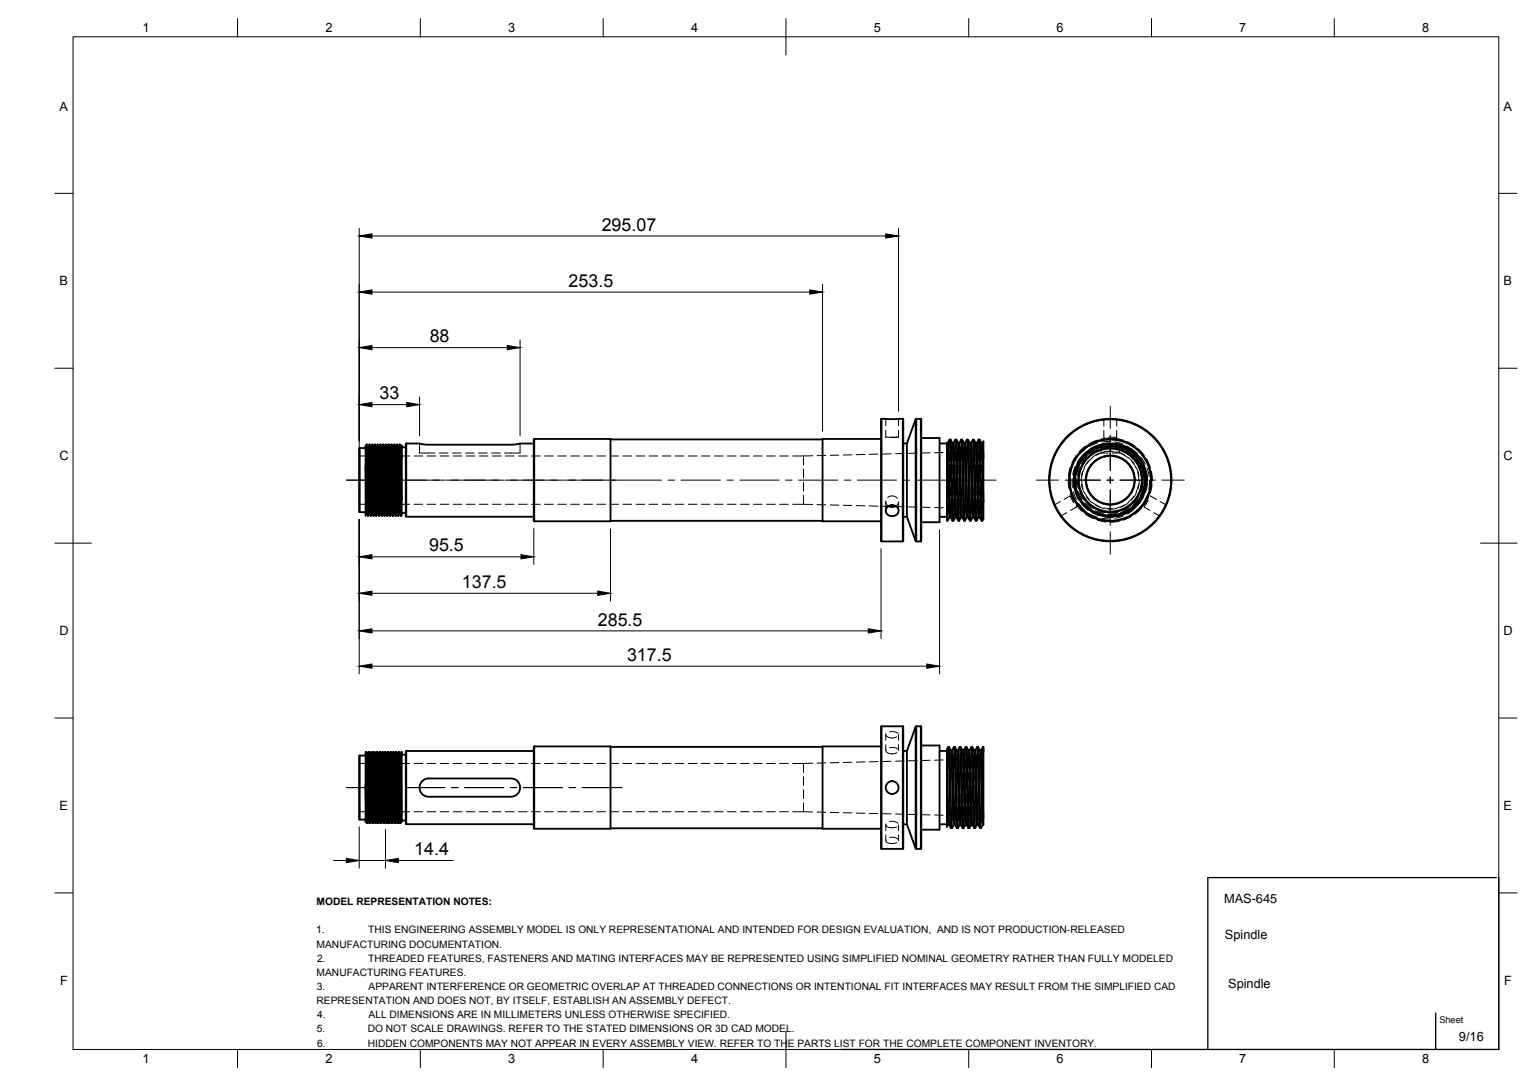
ISO-10303-21;
HEADER;
FILE_DESCRIPTION((''),'2;1');
FILE_NAME('Spindle.step','2026-10-09T10:54:55-07:00',(''),(''),'','','');
FILE_SCHEMA (('AUTOMOTIVE_DESIGN { 1 0 10303 214 3 1 1 }'));
ENDSEC;
DATA;
#10=MECHANICAL_DESIGN_GEOMETRIC_PRESENTATION_REPRESENTATION('',(#600),#63824);
#215=B_SPLINE_SURFACE_WITH_KNOTS('',3,1,((#48544,#48545),(#48546,#48547),
(#48548,#48549),(#48550,#48551),(#48552,#48553),(#48554,#48555),(#48556,
#48557),(#48558,#48559),(#48560,#48561),(#48562,#48563),(#48564,#48565),
(#48566,#48567),(#48568,#48569),(#48570,#48571),(#48572,#48573),(#48574,
#48575),(#48576,#48577),(#48578,#48579),(#48580,#48581),(#48582,#48583),
(#48584,#48585),(#48586,#48587),(#48588,#48589),(#48590,#48591),(#48592,
#48593),(#48594,#48595),(#48596,#48597),(#48598,#48599),(#48600,#48601),
(#48602,#48603),(#48604,#48605),(#48606,#48607),(#48608,#48609),(#48610,
#48611)),.UNSPECIFIED.,.T.,.F.,.F.,(4,2,2,2,2,2,2,2,2,2,2,2,2,2,2,2,4),
(2,2),(0.,0.131943994423176,0.263887988846351,0.395831447701094,0.527774906555838,
0.659718365410582,0.791661824265325,0.9236058186885,1.05554981311168,1.18749380753485,
1.31943780195803,1.45138126081277,1.58332471966751,1.71526817852226,1.847211637377,
1.97915563180018,2.11109962622335),(0.,1.00001320870816),.UNSPECIFIED.) ;
#216=B_SPLINE_SURFACE_WITH_KNOTS('',3,1,((#48671,#48672),(#48673,#48674),
(#48675,#48676),(#48677,#48678),(#48679,#48680),(#48681,#48682),(#48683,
#48684),(#48685,#48686),(#48687,#48688),(#48689,#48690),(#48691,#48692),
(#48693,#48694),(#48695,#48696),(#48697,#48698),(#48699,#48700),(#48701,
#48702),(#48703,#48704),(#48705,#48706),(#48707,#48708),(#48709,#48710),
(#48711,#48712),(#48713,#48714),(#48715,#48716),(#48717,#48718),(#48719,
#48720),(#48721,#48722),(#48723,#48724),(#48725,#48726),(#48727,#48728),
(#48729,#48730),(#48731,#48732),(#48733,#48734),(#48735,#48736),(#48737,
#48738)),.UNSPECIFIED.,.T.,.F.,.F.,(4,2,2,2,2,2,2,2,2,2,2,2,2,2,2,2,4),
(2,2),(0.,0.131943994423175,0.263887988846351,0.395831447701094,0.527774906555838,
0.659718365410582,0.791661824265325,0.923605818688501,1.05554981311168,
1.18749380753485,1.31943780195803,1.45138126081277,1.58332471966751,1.71526817852226,
1.847211637377,1.97915563180018,2.11109962622335),(0.,1.00001320870815),
 .UNSPECIFIED.) ;
#217=B_SPLINE_SURFACE_WITH_KNOTS('',3,1,((#48798,#48799),(#48800,#48801),
(#48802,#48803),(#48804,#48805),(#48806,#48807),(#48808,#48809),(#48810,
#48811),(#48812,#48813),(#48814,#48815),(#48816,#48817),(#48818,#48819),
(#48820,#48821),(#48822,#48823),(#48824,#48825),(#48826,#48827),(#48828,
#48829),(#48830,#48831),(#48832,#48833),(#48834,#48835),(#48836,#48837),
(#48838,#48839),(#48840,#48841),(#48842,#48843),(#48844,#48845),(#48846,
#48847),(#48848,#48849),(#48850,#48851),(#48852,#48853),(#48854,#48855),
(#48856,#48857),(#48858,#48859),(#48860,#48861),(#48862,#48863),(#48864,
#48865)),.UNSPECIFIED.,.T.,.F.,.F.,(4,2,2,2,2,2,2,2,2,2,2,2,2,2,2,2,4),
(2,2),(0.,0.131943994423175,0.26388798884635,0.395831447701094,0.527774906555837,
0.659718365410581,0.791661824265324,0.9236058186885,1.05554981311168,1.18749380753485,
1.31943780195803,1.45138126081277,1.58332471966751,1.71526817852226,1.847211637377,
1.97915563180018,2.11109962622335),(0.,1.00001320870816),.UNSPECIFIED.) ;
#218=B_SPLINE_SURFACE_WITH_KNOTS('',3,3,((#48925,#48926,#48927,#48928,#48929,
#48930,#48931,#48932,#48933,#48934,#48935,#48936,#48937,#48938,#48939,#48940,
#48941,#48942,#48943,#48944,#48945,#48946,#48947,#48948,#48949,#48950,#48951,
#48952,#48953,#48954,#48955,#48956,#48957,#48958,#48959,#48960,#48961,#48962,
#48963,#48964,#48965,#48966,#48967,#48968,#48969,#48970,#48971,#48972,#48973,
#48974,#48975,#48976,#48977,#48978,#48979,#48980,#48981,#48982,#48983,#48984,
#48985,#48986,#48987,#48988,#48989,#48990,#48991,#48992,#48993,#48994,#48995,
#48996,#48997,#48998,#48999,#49000,#49001,#49002,#49003,#49004,#49005,#49006,
#49007,#49008,#49009,#49010,#49011,#49012,#49013,#49014,#49015,#49016,#49017,
#49018,#49019,#49020,#49021,#49022,#49023,#49024,#49025,#49026,#49027,#49028,
#49029,#49030,#49031,#49032,#49033,#49034,#49035,#49036,#49037,#49038,#49039,
#49040,#49041,#49042,#49043,#49044,#49045,#49046,#49047,#49048,#49049,#49050,
#49051,#49052,#49053,#49054,#49055,#49056,#49057,#49058,#49059,#49060,#49061,
#49062,#49063,#49064,#49065,#49066,#49067,#49068,#49069,#49070,#49071,#49072,
#49073,#49074,#49075,#49076,#49077,#49078,#49079,#49080,#49081,#49082,#49083,
#49084,#49085,#49086,#49087,#49088,#49089,#49090,#49091,#49092,#49093,#49094,
#49095,#49096,#49097),(#49098,#49099,#49100,#49101,#49102,#49103,#49104,
#49105,#49106,#49107,#49108,#49109,#49110,#49111,#49112,#49113,#49114,#49115,
#49116,#49117,#49118,#49119,#49120,#49121,#49122,#49123,#49124,#49125,#49126,
#49127,#49128,#49129,#49130,#49131,#49132,#49133,#49134,#49135,#49136,#49137,
#49138,#49139,#49140,#49141,#49142,#49143,#49144,#49145,#49146,#49147,#49148,
#49149,#49150,#49151,#49152,#49153,#49154,#49155,#49156,#49157,#49158,#49159,
#49160,#49161,#49162,#49163,#49164,#49165,#49166,#49167,#49168,#49169,#49170,
#49171,#49172,#49173,#49174,#49175,#49176,#49177,#49178,#49179,#49180,#49181,
#49182,#49183,#49184,#49185,#49186,#49187,#49188,#49189,#49190,#49191,#49192,
#49193,#49194,#49195,#49196,#49197,#49198,#49199,#49200,#49201,#49202,#49203,
#49204,#49205,#49206,#49207,#49208,#49209,#49210,#49211,#49212,#49213,#49214,
#49215,#49216,#49217,#49218,#49219,#49220,#49221,#49222,#49223,#49224,#49225,
#49226,#49227,#49228,#49229,#49230,#49231,#49232,#49233,#49234,#49235,#49236,
#49237,#49238,#49239,#49240,#49241,#49242,#49243,#49244,#49245,#49246,#49247,
#49248,#49249,#49250,#49251,#49252,#49253,#49254,#49255,#49256,#49257,#49258,
#49259,#49260,#49261,#49262,#49263,#49264,#49265,#49266,#49267,#49268,#49269,
#49270),(#49271,#49272,#49273,#49274,#49275,#49276,#49277,#49278,#49279,
#49280,#49281,#49282,#49283,#49284,#49285,#49286,#49287,#49288,#49289,#49290,
#49291,#49292,#49293,#49294,#49295,#49296,#49297,#49298,#49299,#49300,#49301,
#49302,#49303,#49304,#49305,#49306,#49307,#49308,#49309,#49310,#49311,#49312,
#49313,#49314,#49315,#49316,#49317,#49318,#49319,#49320,#49321,#49322,#49323,
#49324,#49325,#49326,#49327,#49328,#49329,#49330,#49331,#49332,#49333,#49334,
#49335,#49336,#49337,#49338,#49339,#49340,#49341,#49342,#49343,#49344,#49345,
#49346,#49347,#49348,#49349,#49350,#49351,#49352,#49353,#49354,#49355,#49356,
#49357,#49358,#49359,#49360,#49361,#49362,#49363,#49364,#49365,#49366,#49367,
#49368,#49369,#49370,#49371,#49372,#49373,#49374,#49375,#49376,#49377,#49378,
#49379,#49380,#49381,#49382,#49383,#49384,#49385,#49386,#49387,#49388,#49389,
#49390,#49391,#49392,#49393,#49394,#49395,#49396,#49397,#49398,#49399,#49400,
#49401,#49402,#49403,#49404,#49405,#49406,#49407,#49408,#49409,#49410,#49411,
#49412,#49413,#49414,#49415,#49416,#49417,#49418,#49419,#49420,#49421,#49422,
#49423,#49424,#49425,#49426,#49427,#49428,#49429,#49430,#49431,#49432,#49433,
#49434,#49435,#49436,#49437,#49438,#49439,#49440,#49441,#49442,#49443),
(#49444,#49445,#49446,#49447,#49448,#49449,#49450,#49451,#49452,#49453,
#49454,#49455,#49456,#49457,#49458,#49459,#49460,#49461,#49462,#49463,#49464,
#49465,#49466,#49467,#49468,#49469,#49470,#49471,#49472,#49473,#49474,#49475,
#49476,#49477,#49478,#49479,#49480,#49481,#49482,#49483,#49484,#49485,#49486,
#49487,#49488,#49489,#49490,#49491,#49492,#49493,#49494,#49495,#49496,#49497,
#49498,#49499,#49500,#49501,#49502,#49503,#49504,#49505,#49506,#49507,#49508,
#49509,#49510,#49511,#49512,#49513,#49514,#49515,#49516,#49517,#49518,#49519,
#49520,#49521,#49522,#49523,#49524,#49525,#49526,#49527,#49528,#49529,#49530,
#49531,#49532,#49533,#49534,#49535,#49536,#49537,#49538,#49539,#49540,#49541,
#49542,#49543,#49544,#49545,#49546,#49547,#49548,#49549,#49550,#49551,#49552,
#49553,#49554,#49555,#49556,#49557,#49558,#49559,#49560,#49561,#49562,#49563,
#49564,#49565,#49566,#49567,#49568,#49569,#49570,#49571,#49572,#49573,#49574,
#49575,#49576,#49577,#49578,#49579,#49580,#49581,#49582,#49583,#49584,#49585,
#49586,#49587,#49588,#49589,#49590,#49591,#49592,#49593,#49594,#49595,#49596,
#49597,#49598,#49599,#49600,#49601,#49602,#49603,#49604,#49605,#49606,#49607,
#49608,#49609,#49610,#49611,#49612,#49613,#49614,#49615,#49616)),
 .UNSPECIFIED.,.F.,.F.,.F.,(4,4),(4,1,1,1,1,1,1,1,1,1,1,1,1,1,1,1,1,1,1,
1,1,1,1,1,1,1,1,1,1,1,1,1,1,1,1,1,1,1,1,1,1,1,1,1,1,1,1,1,1,1,1,1,1,1,1,
1,1,1,1,1,1,1,1,1,1,1,1,1,1,1,1,1,1,1,1,1,1,1,1,1,1,1,1,1,1,1,1,1,1,1,1,
1,1,1,1,1,1,1,1,1,1,1,1,1,1,1,1,1,1,1,1,1,1,1,1,1,1,1,1,1,1,1,1,1,1,1,1,
1,1,1,1,1,1,1,1,1,1,1,1,1,1,1,1,1,1,1,1,1,1,1,1,1,1,1,1,1,1,1,1,1,1,1,1,
1,1,1,1,1,1,1,4),(-0.000231965532648874,0.0996290022117273),(8.29836425792185,
8.79750999747347,9.29636959945186,9.79522920143024,10.2940888034086,10.792948405387,
11.2918080073654,11.7906676093438,12.2895272113222,12.7883868133005,13.2872464152789,
13.7861060172573,14.2849656192357,14.7838252212141,15.2826848231925,15.7815444251708,
16.2804040271492,16.7792636291276,17.278123231106,17.7769828330844,18.2758424350628,
18.7747020370411,19.2735616390195,19.7724212409979,20.2712808429763,20.7701404449547,
21.2690000469331,21.7678596489115,22.2667192508898,22.7655788528682,23.2644384548466,
23.763298056825,24.2621576588034,24.7610172607818,25.2598768627601,25.7587364647385,
26.2575960667169,26.7564556686953,27.2553152706737,27.7541748726521,28.2530344746304,
28.7518940766088,29.2507536785872,29.7496132805656,30.248472882544,30.7473324845224,
31.2461920865007,31.7450516884791,32.2439112904575,32.7427708924359,33.2416304944143,
33.7404900963927,34.239349698371,34.7382093003494,35.2370689023278,35.7359285043062,
36.2347881062846,36.733647708263,37.2325073102413,37.7313669122197,38.2302265141981,
38.7290861161765,39.2279457181549,39.7268053201333,40.2256649221116,40.72452452409,
41.2233841260684,41.7222437280468,42.2211033300252,42.7199629320036,43.218822533982,
43.7176821359603,44.2165417379387,44.7154013399171,45.2142609418955,45.7131205438739,
46.2119801458523,46.7108397478306,47.209699349809,47.7085589517874,48.2074185537658,
48.7062781557442,49.2051377577226,49.7039973597009,50.2028569616793,50.7017165636577,
51.2005761656361,51.6994357676145,52.1982953695929,52.6971549715713,53.1960145735496,
53.694874175528,54.1937337775064,54.6925933794848,55.1914529814632,55.6903125834416,
56.1891721854199,56.6880317873983,57.1868913893767,57.6857509913551,58.1846105933335,
58.6834701953119,59.1823297972902,59.6811893992686,60.180049001247,60.6789086032254,
61.1777682052038,61.6766278071822,62.1754874091605,62.6743470111389,63.1732066131173,
63.6720662150957,64.1709258170741,64.6697854190525,65.1686450210308,65.6675046230092,
66.1663642249876,66.665223826966,67.1640834289444,67.6629430309227,68.1618026329011,
68.6606622348795,69.1595218368579,69.6583814388363,70.1572410408147,70.6561006427931,
71.1549602447714,71.6538198467498,72.1526794487282,72.6515390507066,73.150398652685,
73.6492582546634,74.1481178566417,74.6469774586201,75.1458370605985,75.6446966625769,
76.1435562645553,76.6424158665337,77.141275468512,77.6401350704904,78.1389946724688,
78.6378542744472,79.1367138764256,79.635573478404,80.1344330803824,80.6332926823607,
81.1321522843391,81.6310118863175,82.1298714882959,82.6287310902743,83.1275906922527,
83.626450294231,84.1253098962094,84.6241694981878,85.1230291001662,85.6218887021446,
86.120748304123,86.6196079061014,87.1184675080797,87.6173271100581,88.1161867120365,
88.6150463140149,89.1139059159933,89.6127655179716,90.11162511995,90.6104847219284,
91.1093443239068,91.6082039258852,92.1070635278636,92.605923129842,93.1050146973529),
 .UNSPECIFIED.) ;
#219=B_SPLINE_SURFACE_WITH_KNOTS('',3,3,((#49897,#49898,#49899,#49900,#49901,
#49902,#49903,#49904,#49905,#49906,#49907,#49908,#49909,#49910,#49911,#49912,
#49913,#49914,#49915,#49916,#49917,#49918,#49919,#49920,#49921,#49922,#49923,
#49924,#49925,#49926,#49927,#49928,#49929,#49930,#49931,#49932,#49933,#49934,
#49935,#49936,#49937,#49938,#49939,#49940,#49941,#49942,#49943,#49944,#49945,
#49946,#49947,#49948,#49949,#49950,#49951,#49952,#49953,#49954,#49955,#49956,
#49957,#49958,#49959,#49960,#49961,#49962,#49963,#49964,#49965,#49966,#49967,
#49968,#49969,#49970,#49971,#49972,#49973,#49974,#49975,#49976,#49977,#49978,
#49979,#49980,#49981,#49982,#49983,#49984,#49985,#49986,#49987,#49988,#49989,
#49990,#49991,#49992,#49993,#49994,#49995,#49996,#49997,#49998,#49999,#50000,
#50001,#50002,#50003,#50004,#50005,#50006,#50007,#50008,#50009,#50010,#50011,
#50012,#50013,#50014,#50015,#50016,#50017,#50018,#50019,#50020,#50021,#50022,
#50023,#50024,#50025,#50026,#50027,#50028,#50029,#50030,#50031,#50032,#50033,
#50034,#50035,#50036,#50037,#50038,#50039,#50040,#50041,#50042,#50043,#50044,
#50045,#50046,#50047,#50048,#50049,#50050,#50051,#50052,#50053,#50054,#50055,
#50056,#50057,#50058,#50059,#50060,#50061,#50062,#50063,#50064,#50065,#50066,
#50067,#50068,#50069),(#50070,#50071,#50072,#50073,#50074,#50075,#50076,
#50077,#50078,#50079,#50080,#50081,#50082,#50083,#50084,#50085,#50086,#50087,
#50088,#50089,#50090,#50091,#50092,#50093,#50094,#50095,#50096,#50097,#50098,
#50099,#50100,#50101,#50102,#50103,#50104,#50105,#50106,#50107,#50108,#50109,
#50110,#50111,#50112,#50113,#50114,#50115,#50116,#50117,#50118,#50119,#50120,
#50121,#50122,#50123,#50124,#50125,#50126,#50127,#50128,#50129,#50130,#50131,
#50132,#50133,#50134,#50135,#50136,#50137,#50138,#50139,#50140,#50141,#50142,
#50143,#50144,#50145,#50146,#50147,#50148,#50149,#50150,#50151,#50152,#50153,
#50154,#50155,#50156,#50157,#50158,#50159,#50160,#50161,#50162,#50163,#50164,
#50165,#50166,#50167,#50168,#50169,#50170,#50171,#50172,#50173,#50174,#50175,
#50176,#50177,#50178,#50179,#50180,#50181,#50182,#50183,#50184,#50185,#50186,
#50187,#50188,#50189,#50190,#50191,#50192,#50193,#50194,#50195,#50196,#50197,
#50198,#50199,#50200,#50201,#50202,#50203,#50204,#50205,#50206,#50207,#50208,
#50209,#50210,#50211,#50212,#50213,#50214,#50215,#50216,#50217,#50218,#50219,
#50220,#50221,#50222,#50223,#50224,#50225,#50226,#50227,#50228,#50229,#50230,
#50231,#50232,#50233,#50234,#50235,#50236,#50237,#50238,#50239,#50240,#50241,
#50242),(#50243,#50244,#50245,#50246,#50247,#50248,#50249,#50250,#50251,
#50252,#50253,#50254,#50255,#50256,#50257,#50258,#50259,#50260,#50261,#50262,
#50263,#50264,#50265,#50266,#50267,#50268,#50269,#50270,#50271,#50272,#50273,
#50274,#50275,#50276,#50277,#50278,#50279,#50280,#50281,#50282,#50283,#50284,
#50285,#50286,#50287,#50288,#50289,#50290,#50291,#50292,#50293,#50294,#50295,
#50296,#50297,#50298,#50299,#50300,#50301,#50302,#50303,#50304,#50305,#50306,
#50307,#50308,#50309,#50310,#50311,#50312,#50313,#50314,#50315,#50316,#50317,
#50318,#50319,#50320,#50321,#50322,#50323,#50324,#50325,#50326,#50327,#50328,
#50329,#50330,#50331,#50332,#50333,#50334,#50335,#50336,#50337,#50338,#50339,
#50340,#50341,#50342,#50343,#50344,#50345,#50346,#50347,#50348,#50349,#50350,
#50351,#50352,#50353,#50354,#50355,#50356,#50357,#50358,#50359,#50360,#50361,
#50362,#50363,#50364,#50365,#50366,#50367,#50368,#50369,#50370,#50371,#50372,
#50373,#50374,#50375,#50376,#50377,#50378,#50379,#50380,#50381,#50382,#50383,
#50384,#50385,#50386,#50387,#50388,#50389,#50390,#50391,#50392,#50393,#50394,
#50395,#50396,#50397,#50398,#50399,#50400,#50401,#50402,#50403,#50404,#50405,
#50406,#50407,#50408,#50409,#50410,#50411,#50412,#50413,#50414,#50415),
(#50416,#50417,#50418,#50419,#50420,#50421,#50422,#50423,#50424,#50425,
#50426,#50427,#50428,#50429,#50430,#50431,#50432,#50433,#50434,#50435,#50436,
#50437,#50438,#50439,#50440,#50441,#50442,#50443,#50444,#50445,#50446,#50447,
#50448,#50449,#50450,#50451,#50452,#50453,#50454,#50455,#50456,#50457,#50458,
#50459,#50460,#50461,#50462,#50463,#50464,#50465,#50466,#50467,#50468,#50469,
#50470,#50471,#50472,#50473,#50474,#50475,#50476,#50477,#50478,#50479,#50480,
#50481,#50482,#50483,#50484,#50485,#50486,#50487,#50488,#50489,#50490,#50491,
#50492,#50493,#50494,#50495,#50496,#50497,#50498,#50499,#50500,#50501,#50502,
#50503,#50504,#50505,#50506,#50507,#50508,#50509,#50510,#50511,#50512,#50513,
#50514,#50515,#50516,#50517,#50518,#50519,#50520,#50521,#50522,#50523,#50524,
#50525,#50526,#50527,#50528,#50529,#50530,#50531,#50532,#50533,#50534,#50535,
#50536,#50537,#50538,#50539,#50540,#50541,#50542,#50543,#50544,#50545,#50546,
#50547,#50548,#50549,#50550,#50551,#50552,#50553,#50554,#50555,#50556,#50557,
#50558,#50559,#50560,#50561,#50562,#50563,#50564,#50565,#50566,#50567,#50568,
#50569,#50570,#50571,#50572,#50573,#50574,#50575,#50576,#50577,#50578,#50579,
#50580,#50581,#50582,#50583,#50584,#50585,#50586,#50587,#50588)),
 .UNSPECIFIED.,.F.,.F.,.F.,(4,4),(4,1,1,1,1,1,1,1,1,1,1,1,1,1,1,1,1,1,1,
1,1,1,1,1,1,1,1,1,1,1,1,1,1,1,1,1,1,1,1,1,1,1,1,1,1,1,1,1,1,1,1,1,1,1,1,
1,1,1,1,1,1,1,1,1,1,1,1,1,1,1,1,1,1,1,1,1,1,1,1,1,1,1,1,1,1,1,1,1,1,1,1,
1,1,1,1,1,1,1,1,1,1,1,1,1,1,1,1,1,1,1,1,1,1,1,1,1,1,1,1,1,1,1,1,1,1,1,1,
1,1,1,1,1,1,1,1,1,1,1,1,1,1,1,1,1,1,1,1,1,1,1,1,1,1,1,1,1,1,1,1,1,1,1,1,
1,1,1,1,1,1,1,4),(-0.000434450397776735,0.0994265044407978),(11.614740433148,
12.1138319898177,12.6126915917961,13.1115511937745,13.6104107957528,14.1092703977312,
14.6081299997096,15.106989601688,15.6058492036664,16.1047088056448,16.6035684076232,
17.1024280096015,17.6012876115799,18.1001472135583,18.5990068155367,19.0978664175151,
19.5967260194935,20.0955856214718,20.5944452234502,21.0933048254286,21.592164427407,
22.0910240293854,22.5898836313638,23.0887432333421,23.5876028353205,24.0864624372989,
24.5853220392773,25.0841816412557,25.5830412432341,26.0819008452124,26.5807604471908,
27.0796200491692,27.5784796511476,28.077339253126,28.5761988551044,29.0750584570828,
29.5739180590611,30.0727776610395,30.5716372630179,31.0704968649963,31.5693564669747,
32.0682160689531,32.5670756709314,33.0659352729098,33.5647948748882,34.0636544768666,
34.562514078845,35.0613736808234,35.5602332828017,36.0590928847801,36.5579524867585,
37.0568120887369,37.5556716907153,38.0545312926937,38.553390894672,39.0522504966504,
39.5511100986288,40.0499697006072,40.5488293025856,41.047688904564,41.5465485065424,
42.0454081085207,42.5442677104991,43.0431273124775,43.5419869144559,44.0408465164343,
44.5397061184127,45.038565720391,45.5374253223694,46.0362849243478,46.5351445263262,
47.0340041283046,47.532863730283,48.0317233322614,48.5305829342397,49.0294425362181,
49.5283021381965,50.0271617401749,50.5260213421533,51.0248809441317,51.52374054611,
52.0226001480884,52.5214597500668,53.0203193520452,53.5191789540236,54.018038556002,
54.5168981579803,55.0157577599587,55.5146173619371,56.0134769639155,56.5123365658939,
57.0111961678723,57.5100557698507,58.008915371829,58.5077749738074,59.0066345757858,
59.5054941777642,60.0043537797426,60.503213381721,61.0020729836993,61.5009325856777,
61.9997921876561,62.4986517896345,62.9975113916129,63.4963709935913,63.9952305955696,
64.494090197548,64.9929497995264,65.4918094015048,65.9906690034832,66.4895286054616,
66.98838820744,67.4872478094183,67.9861074113967,68.4849670133751,68.9838266153535,
69.4826862173319,69.9815458193102,70.4804054212886,70.979265023267,71.4781246252454,
71.9769842272238,72.4758438292022,72.9747034311806,73.4735630331589,73.9724226351373,
74.4712822371157,74.9701418390941,75.4690014410725,75.9678610430509,76.4667206450292,
76.9655802470076,77.464439848986,77.9632994509644,78.4621590529428,78.9610186549212,
79.4598782568995,79.9587378588779,80.4575974608563,80.9564570628347,81.4553166648131,
81.9541762667915,82.4530358687698,82.9518954707482,83.4507550727266,83.949614674705,
84.4484742766834,84.9473338786618,85.4461934806401,85.9450530826185,86.4439126845969,
86.9427722865753,87.4416318885537,87.9404914905321,88.4393510925105,88.9382106944888,
89.4370702964672,89.9359298984456,90.434789500424,90.9336491024024,91.4325087043808,
91.9313683063591,92.4302279083375,92.9290875103159,93.4279471122943,93.9268067142727,
94.4256663162511,94.9245259182294,95.4233855202078,95.9222451221862,96.421393347443),
 .UNSPECIFIED.) ;
#220=B_SPLINE_SURFACE_WITH_KNOTS('',3,3,((#50861,#50862,#50863,#50864,#50865,
#50866,#50867,#50868,#50869,#50870,#50871,#50872,#50873,#50874,#50875,#50876,
#50877,#50878,#50879,#50880,#50881,#50882,#50883,#50884,#50885,#50886,#50887,
#50888,#50889,#50890,#50891,#50892,#50893,#50894,#50895,#50896,#50897,#50898,
#50899,#50900,#50901,#50902,#50903,#50904,#50905,#50906,#50907,#50908,#50909,
#50910,#50911,#50912,#50913,#50914,#50915,#50916,#50917,#50918,#50919,#50920,
#50921,#50922,#50923,#50924,#50925,#50926,#50927,#50928,#50929,#50930,#50931,
#50932,#50933,#50934,#50935,#50936,#50937,#50938,#50939,#50940,#50941,#50942,
#50943,#50944,#50945,#50946,#50947),(#50948,#50949,#50950,#50951,#50952,
#50953,#50954,#50955,#50956,#50957,#50958,#50959,#50960,#50961,#50962,#50963,
#50964,#50965,#50966,#50967,#50968,#50969,#50970,#50971,#50972,#50973,#50974,
#50975,#50976,#50977,#50978,#50979,#50980,#50981,#50982,#50983,#50984,#50985,
#50986,#50987,#50988,#50989,#50990,#50991,#50992,#50993,#50994,#50995,#50996,
#50997,#50998,#50999,#51000,#51001,#51002,#51003,#51004,#51005,#51006,#51007,
#51008,#51009,#51010,#51011,#51012,#51013,#51014,#51015,#51016,#51017,#51018,
#51019,#51020,#51021,#51022,#51023,#51024,#51025,#51026,#51027,#51028,#51029,
#51030,#51031,#51032,#51033,#51034),(#51035,#51036,#51037,#51038,#51039,
#51040,#51041,#51042,#51043,#51044,#51045,#51046,#51047,#51048,#51049,#51050,
#51051,#51052,#51053,#51054,#51055,#51056,#51057,#51058,#51059,#51060,#51061,
#51062,#51063,#51064,#51065,#51066,#51067,#51068,#51069,#51070,#51071,#51072,
#51073,#51074,#51075,#51076,#51077,#51078,#51079,#51080,#51081,#51082,#51083,
#51084,#51085,#51086,#51087,#51088,#51089,#51090,#51091,#51092,#51093,#51094,
#51095,#51096,#51097,#51098,#51099,#51100,#51101,#51102,#51103,#51104,#51105,
#51106,#51107,#51108,#51109,#51110,#51111,#51112,#51113,#51114,#51115,#51116,
#51117,#51118,#51119,#51120,#51121),(#51122,#51123,#51124,#51125,#51126,
#51127,#51128,#51129,#51130,#51131,#51132,#51133,#51134,#51135,#51136,#51137,
#51138,#51139,#51140,#51141,#51142,#51143,#51144,#51145,#51146,#51147,#51148,
#51149,#51150,#51151,#51152,#51153,#51154,#51155,#51156,#51157,#51158,#51159,
#51160,#51161,#51162,#51163,#51164,#51165,#51166,#51167,#51168,#51169,#51170,
#51171,#51172,#51173,#51174,#51175,#51176,#51177,#51178,#51179,#51180,#51181,
#51182,#51183,#51184,#51185,#51186,#51187,#51188,#51189,#51190,#51191,#51192,
#51193,#51194,#51195,#51196,#51197,#51198,#51199,#51200,#51201,#51202,#51203,
#51204,#51205,#51206,#51207,#51208)),.UNSPECIFIED.,.F.,.F.,.F.,(4,4),(4,
1,1,1,1,1,1,1,1,1,1,1,1,1,1,1,1,1,1,1,1,1,1,1,1,1,1,1,1,1,1,1,1,1,1,1,1,
1,1,1,1,1,1,1,1,1,1,1,1,1,1,1,1,1,1,1,1,1,1,1,1,1,1,1,1,1,1,1,1,1,1,1,1,
1,1,1,1,1,1,1,1,1,1,1,4),(-0.000240669354260341,0.207692603139416),(8.31441726003343,
8.81032130755511,9.30590986525221,9.8014984229493,10.2970869806464,10.7926755383435,
11.2882640960406,11.7838526537377,12.2794412114348,12.7750297691319,13.270618326829,
13.7662068845261,14.2617954422232,14.7573839999203,15.2529725576174,15.7485611153145,
16.2441496730116,16.7397382307087,17.2353267884057,17.7309153461028,18.2265039037999,
18.722092461497,19.2176810191941,19.7132695768912,20.2088581345883,20.7044466922854,
21.2000352499825,21.6956238076796,22.1912123653767,22.6868009230738,23.1823894807709,
23.677978038468,24.1735665961651,24.6691551538622,25.1647437115593,25.6603322692564,
26.1559208269535,26.6515093846506,27.1470979423477,27.6426865000448,28.1382750577419,
28.633863615439,29.1294521731361,29.6250407308331,30.1206292885302,30.6162178462273,
31.1118064039244,31.6073949616215,32.1029835193186,32.5985720770157,33.0941606347128,
33.5897491924099,34.085337750107,34.5809263078041,35.0765148655012,35.5721034231983,
36.0676919808954,36.5632805385925,37.0588690962896,37.5544576539867,38.0500462116838,
38.5456347693809,39.041223327078,39.5368118847751,40.0324004424722,40.5279890001693,
41.0235775578664,41.5191661155635,42.0147546732606,42.5103432309577,43.0059317886547,
43.5015203463518,43.9971089040489,44.492697461746,44.9882860194431,45.4838745771402,
45.9794631348373,46.4750516925344,46.9706402502315,47.4662288079286,47.9618173656257,
48.4574059233228,48.9529944810199,49.448583038717,49.9444122657684),
 .UNSPECIFIED.) ;
#221=B_SPLINE_SURFACE_WITH_KNOTS('',3,3,((#51336,#51337,#51338,#51339,#51340,
#51341,#51342,#51343,#51344,#51345,#51346,#51347,#51348,#51349,#51350,#51351,
#51352,#51353,#51354,#51355,#51356,#51357,#51358,#51359,#51360,#51361,#51362,
#51363,#51364,#51365,#51366,#51367,#51368,#51369,#51370,#51371,#51372,#51373,
#51374,#51375,#51376,#51377,#51378,#51379,#51380,#51381,#51382,#51383,#51384,
#51385,#51386,#51387,#51388,#51389,#51390,#51391,#51392,#51393,#51394,#51395,
#51396,#51397,#51398,#51399,#51400,#51401,#51402,#51403,#51404,#51405,#51406,
#51407,#51408,#51409,#51410,#51411,#51412,#51413,#51414,#51415,#51416,#51417,
#51418,#51419,#51420,#51421,#51422),(#51423,#51424,#51425,#51426,#51427,
#51428,#51429,#51430,#51431,#51432,#51433,#51434,#51435,#51436,#51437,#51438,
#51439,#51440,#51441,#51442,#51443,#51444,#51445,#51446,#51447,#51448,#51449,
#51450,#51451,#51452,#51453,#51454,#51455,#51456,#51457,#51458,#51459,#51460,
#51461,#51462,#51463,#51464,#51465,#51466,#51467,#51468,#51469,#51470,#51471,
#51472,#51473,#51474,#51475,#51476,#51477,#51478,#51479,#51480,#51481,#51482,
#51483,#51484,#51485,#51486,#51487,#51488,#51489,#51490,#51491,#51492,#51493,
#51494,#51495,#51496,#51497,#51498,#51499,#51500,#51501,#51502,#51503,#51504,
#51505,#51506,#51507,#51508,#51509),(#51510,#51511,#51512,#51513,#51514,
#51515,#51516,#51517,#51518,#51519,#51520,#51521,#51522,#51523,#51524,#51525,
#51526,#51527,#51528,#51529,#51530,#51531,#51532,#51533,#51534,#51535,#51536,
#51537,#51538,#51539,#51540,#51541,#51542,#51543,#51544,#51545,#51546,#51547,
#51548,#51549,#51550,#51551,#51552,#51553,#51554,#51555,#51556,#51557,#51558,
#51559,#51560,#51561,#51562,#51563,#51564,#51565,#51566,#51567,#51568,#51569,
#51570,#51571,#51572,#51573,#51574,#51575,#51576,#51577,#51578,#51579,#51580,
#51581,#51582,#51583,#51584,#51585,#51586,#51587,#51588,#51589,#51590,#51591,
#51592,#51593,#51594,#51595,#51596),(#51597,#51598,#51599,#51600,#51601,
#51602,#51603,#51604,#51605,#51606,#51607,#51608,#51609,#51610,#51611,#51612,
#51613,#51614,#51615,#51616,#51617,#51618,#51619,#51620,#51621,#51622,#51623,
#51624,#51625,#51626,#51627,#51628,#51629,#51630,#51631,#51632,#51633,#51634,
#51635,#51636,#51637,#51638,#51639,#51640,#51641,#51642,#51643,#51644,#51645,
#51646,#51647,#51648,#51649,#51650,#51651,#51652,#51653,#51654,#51655,#51656,
#51657,#51658,#51659,#51660,#51661,#51662,#51663,#51664,#51665,#51666,#51667,
#51668,#51669,#51670,#51671,#51672,#51673,#51674,#51675,#51676,#51677,#51678,
#51679,#51680,#51681,#51682,#51683)),.UNSPECIFIED.,.F.,.F.,.F.,(4,4),(4,
1,1,1,1,1,1,1,1,1,1,1,1,1,1,1,1,1,1,1,1,1,1,1,1,1,1,1,1,1,1,1,1,1,1,1,1,
1,1,1,1,1,1,1,1,1,1,1,1,1,1,1,1,1,1,1,1,1,1,1,1,1,1,1,1,1,1,1,1,1,1,1,1,
1,1,1,1,1,1,1,1,1,1,1,4),(-0.000480856812830276,0.207452754717094),(11.6258564355357,
12.1216855816372,12.6172741393343,13.1128626970314,13.6084512547285,14.1040398124256,
14.5996283701227,15.0952169278198,15.5908054855169,16.086394043214,16.5819826009111,
17.0775711586082,17.5731597163053,18.0687482740024,18.5643368316995,19.0599253893966,
19.5555139470937,20.0511025047908,20.5466910624879,21.042279620185,21.5378681778821,
22.0334567355792,22.5290452932763,23.0246338509733,23.5202224086704,24.0158109663675,
24.5113995240646,25.0069880817617,25.5025766394588,25.9981651971559,26.493753754853,
26.9893423125501,27.4849308702472,27.9805194279443,28.4761079856414,28.9716965433385,
29.4672851010356,29.9628736587327,30.4584622164298,30.9540507741269,31.449639331824,
31.9452278895211,32.4408164472182,32.9364050049153,33.4319935626124,33.9275821203095,
34.4231706780066,34.9187592357037,35.4143477934008,35.9099363510978,36.4055249087949,
36.901113466492,37.3967020241891,37.8922905818862,38.3878791395833,38.8834676972804,
39.3790562549775,39.8746448126746,40.3702333703717,40.8658219280688,41.3614104857659,
41.856999043463,42.3525876011601,42.8481761588572,43.3437647165543,43.8393532742514,
44.3349418319485,44.8305303896456,45.3261189473427,45.8217075050398,46.3172960627369,
46.812884620434,47.3084731781311,47.8040617358281,48.2996502935252,48.7952388512223,
49.2908274089194,49.7864159666165,50.2820045243136,50.7775930820107,51.2731816397078,
51.7687701974049,52.264358755102,52.7599473127991,53.2558559415817),
 .UNSPECIFIED.) ;
#222=B_SPLINE_CURVE_WITH_KNOTS('',3,(#23804,#23805,#23806,#23807,#23808,
#23809,#23810,#23811,#23812,#23813,#23814,#23815,#23816,#23817,#23818,#23819,
#23820,#23821,#23822,#23823,#23824,#23825,#23826,#23827,#23828,#23829,#23830,
#23831,#23832,#23833,#23834,#23835,#23836,#23837,#23838,#23839,#23840,#23841,
#23842,#23843,#23844,#23845,#23846,#23847,#23848,#23849,#23850,#23851,#23852,
#23853,#23854,#23855,#23856,#23857,#23858,#23859,#23860,#23861,#23862,#23863,
#23864,#23865,#23866,#23867,#23868,#23869,#23870,#23871,#23872,#23873,#23874,
#23875,#23876,#23877,#23878,#23879,#23880,#23881,#23882,#23883,#23884,#23885,
#23886,#23887,#23888,#23889,#23890,#23891,#23892,#23893,#23894,#23895,#23896,
#23897,#23898,#23899,#23900,#23901,#23902,#23903,#23904,#23905,#23906,#23907,
#23908,#23909,#23910,#23911,#23912,#23913,#23914,#23915,#23916,#23917,#23918,
#23919,#23920,#23921,#23922,#23923,#23924,#23925,#23926,#23927,#23928,#23929,
#23930,#23931,#23932,#23933,#23934,#23935),.UNSPECIFIED.,.F.,.F.,(4,2,2,
2,2,2,2,2,2,2,2,2,2,2,2,2,2,2,2,2,2,2,2,2,2,2,2,2,2,2,2,2,2,2,2,2,2,2,2,
2,2,2,2,2,2,2,2,2,2,2,2,2,2,2,2,2,2,2,2,2,2,2,2,2,2,4),(-16.1229693507328,
-15.9135799066995,-15.8630188232808,-15.8258339769541,-15.7900643273633,
-15.7493447314678,-15.6804351503378,-15.4438875959545,-15.382716929369,
-15.3511867583258,-15.3490515343236,-15.3474738962906,-15.3462861030307,
-15.3453772206255,-15.3446721805859,-15.3422209639646,-15.3399838267774,
-15.3379087228275,-15.335949913756,-15.3340653838625,-15.3322140707189,
-15.312299721018,-15.2933483093209,-15.2575988936463,-15.1101303960858,
-14.9770661832259,-14.9147347649729,-14.8645510943747,-14.8321428783299,
-14.7941984330884,-14.7474930119732,-14.5824427622385,-14.4236499865968,
-14.3733286233332,-14.3496260871508,-14.3296916779127,-14.3001338022836,
-14.205790025479,-14.1493019577269,-14.0104112561113,-13.9672600709325,
-13.902906436049,-13.8630630143224,-13.8252061120945,-13.7790024342338,
-13.6144737469252,-13.4558833048607,-13.4046920450664,-13.3808187973035,
-13.360892241764,-13.3315240504932,-13.239398973681,-13.112513364983,-12.9674714651803,
-12.9174417478242,-12.8799279430778,-12.838125864583,-12.7648688910664,
-12.7000821654783,-12.5248339492791,-12.4451057288507,-12.4174885325345,
-12.399593032763,-12.3756627482975,-12.3240898597893,-12.2072680143011),
 .UNSPECIFIED.) ;
#223=B_SPLINE_CURVE_WITH_KNOTS('',3,(#23938,#23939,#23940,#23941,#23942,
#23943,#23944,#23945,#23946,#23947,#23948,#23949,#23950,#23951,#23952,#23953,
#23954,#23955,#23956,#23957,#23958,#23959,#23960,#23961,#23962,#23963,#23964,
#23965,#23966,#23967,#23968,#23969,#23970,#23971,#23972,#23973,#23974,#23975,
#23976,#23977,#23978,#23979,#23980,#23981,#23982,#23983,#23984,#23985,#23986,
#23987,#23988,#23989,#23990,#23991,#23992,#23993,#23994,#23995,#23996,#23997,
#23998,#23999,#24000,#24001,#24002,#24003,#24004,#24005,#24006,#24007,#24008,
#24009),.UNSPECIFIED.,.F.,.F.,(4,2,2,2,2,2,2,2,2,2,2,2,2,2,2,2,2,2,2,2,
2,2,2,2,2,2,2,2,2,2,2,2,2,2,2,4),(0.000310445151374366,0.0115408935467113,
0.0246665289368376,0.0621056912317256,0.260884109848728,0.378907191384278,
0.417457177688961,0.45359225385393,0.489222506445489,0.54948956411632,0.725511782450542,
0.865407477841949,0.915570228192533,0.936508372302185,0.957197100440422,
0.975194107826528,0.99626310266181,1.0317648914341,1.16397106478206,1.30320971966519,
1.36670318110169,1.40294750827005,1.41439432286191,1.44931608805952,1.48713481040049,
1.5418368243862,1.75235977753755,1.88243028398069,1.91902241857432,1.94008923532906,
1.9615202035756,1.99897338198793,2.08917556360275,2.10566915491795,2.13232522116834,
2.18817716271853),.UNSPECIFIED.) ;
#224=B_SPLINE_CURVE_WITH_KNOTS('',3,(#24014,#24015,#24016,#24017,#24018,
#24019,#24020,#24021,#24022,#24023,#24024,#24025,#24026,#24027,#24028,#24029,
#24030,#24031,#24032,#24033,#24034,#24035,#24036,#24037,#24038,#24039,#24040,
#24041,#24042,#24043,#24044,#24045,#24046,#24047,#24048,#24049,#24050,#24051,
#24052,#24053,#24054,#24055,#24056,#24057,#24058,#24059,#24060,#24061,#24062,
#24063,#24064,#24065,#24066,#24067,#24068,#24069,#24070,#24071,#24072,#24073,
#24074,#24075,#24076,#24077,#24078,#24079,#24080,#24081,#24082,#24083,#24084,
#24085,#24086,#24087,#24088,#24089,#24090,#24091,#24092,#24093,#24094,#24095,
#24096,#24097,#24098,#24099,#24100,#24101,#24102,#24103,#24104,#24105,#24106,
#24107,#24108,#24109,#24110,#24111,#24112,#24113,#24114,#24115,#24116,#24117,
#24118,#24119,#24120,#24121,#24122,#24123,#24124,#24125,#24126,#24127,#24128,
#24129,#24130,#24131,#24132,#24133,#24134,#24135,#24136,#24137,#24138,#24139,
#24140,#24141,#24142,#24143,#24144,#24145,#24146,#24147,#24148,#24149,#24150,
#24151,#24152,#24153,#24154,#24155,#24156,#24157,#24158,#24159,#24160,#24161,
#24162,#24163,#24164,#24165,#24166,#24167,#24168,#24169,#24170,#24171,#24172,
#24173,#24174,#24175,#24176,#24177,#24178,#24179,#24180,#24181,#24182,#24183,
#24184,#24185,#24186,#24187,#24188,#24189,#24190,#24191,#24192,#24193,#24194,
#24195,#24196,#24197,#24198,#24199,#24200,#24201,#24202,#24203,#24204,#24205,
#24206,#24207,#24208,#24209,#24210,#24211,#24212,#24213,#24214,#24215,#24216,
#24217,#24218,#24219,#24220,#24221,#24222,#24223,#24224,#24225,#24226,#24227,
#24228,#24229,#24230,#24231,#24232,#24233,#24234,#24235,#24236,#24237,#24238,
#24239,#24240,#24241,#24242,#24243,#24244,#24245,#24246,#24247,#24248,#24249,
#24250,#24251,#24252,#24253,#24254,#24255,#24256,#24257,#24258,#24259,#24260,
#24261,#24262,#24263,#24264,#24265,#24266,#24267,#24268,#24269,#24270,#24271,
#24272,#24273,#24274,#24275,#24276,#24277,#24278,#24279,#24280,#24281,#24282,
#24283,#24284,#24285,#24286,#24287,#24288,#24289,#24290,#24291,#24292,#24293,
#24294,#24295,#24296,#24297,#24298,#24299,#24300,#24301,#24302,#24303,#24304,
#24305,#24306,#24307,#24308,#24309,#24310,#24311,#24312,#24313,#24314,#24315,
#24316,#24317,#24318,#24319,#24320,#24321,#24322,#24323,#24324,#24325,#24326,
#24327,#24328,#24329,#24330,#24331,#24332,#24333,#24334,#24335,#24336,#24337,
#24338,#24339,#24340,#24341,#24342,#24343,#24344,#24345,#24346,#24347,#24348,
#24349,#24350,#24351,#24352,#24353,#24354,#24355),.UNSPECIFIED.,.F.,.F.,
(4,2,2,2,2,2,2,2,2,2,2,2,2,2,2,2,2,2,2,2,2,2,2,2,2,2,2,2,2,2,2,2,2,2,2,
2,2,2,2,2,2,2,2,2,2,2,2,2,2,2,2,2,2,2,2,2,2,2,2,2,2,2,2,2,2,2,2,2,2,2,2,
2,2,2,2,2,2,2,2,2,2,2,2,2,2,2,2,2,2,2,2,2,2,2,2,2,2,2,2,2,2,2,2,2,2,2,2,
2,2,2,2,2,2,2,2,2,2,2,2,2,2,2,2,2,2,2,2,2,2,2,2,2,2,2,2,2,2,2,2,2,2,2,2,
2,2,2,2,2,2,2,2,2,2,2,2,2,2,2,2,2,2,2,2,2,2,2,2,2,2,2,4),(-12.2072680143011,
-12.1214316325864,-12.0348137295484,-11.9673727988363,-11.9269792152918,
-11.8889951798646,-11.8354617297945,-11.615155934698,-11.4926371450886,
-11.4567462368015,-11.4357130176028,-11.4169088168123,-11.3819692573798,
-11.2753908522613,-11.0659613648654,-10.9982933482017,-10.9578545775686,
-10.919881999828,-10.866456417054,-10.7484568701481,-10.5837678213848,-10.5450462648772,
-10.4960146050613,-10.4725095334352,-10.4524974952048,-10.4224502327544,
-10.3093369784509,-10.2224431927978,-10.1144447738829,-10.0365217618984,
-9.99428594351171,-9.95687012854156,-9.90853845623905,-9.7794505566006,
-9.61462525448062,-9.57588749294409,-9.52684296406612,-9.50333752228509,
-9.48332735686028,-9.45328875884435,-9.34062140172601,-9.21399657064198,
-9.12730295634282,-9.05982032737858,-9.01941609794039,-8.98143018783511,
-8.93636895026983,-8.80735611467015,-8.64484772170618,-8.60637781831352,
-8.55756026874535,-8.53409283329303,-8.51407078986009,-8.48395034743693,
-8.37518456547857,-8.34399557902459,-8.19873504568114,-8.10613967829615,
-8.06157709065096,-8.02810934960208,-7.98401608757255,-7.89456466392264,
-7.7582671599074,-7.61585865112676,-7.58000855002441,-7.56104370400703,
-7.5401903997776,-7.50523201263521,-7.26025892497224,-7.14755908688535,
-7.09984468888507,-7.06249093535267,-7.01988569946944,-6.93977085594752,
-6.69088410769133,-6.62674460165974,-6.60070971340099,-6.58101006716034,
-6.55508595815767,-6.49001828517347,-6.37409284031265,-6.31557441951567,
-6.18244765878282,-6.13318015851525,-6.09565470845379,-6.05391590447638,
-5.97889669698792,-5.8771619883261,-5.67448067858958,-5.64019149258949,
-5.62150014994861,-5.60031687680764,-5.56367573660035,-5.43426584477831,
-5.22452145485842,-5.16997775976138,-5.13221214200042,-5.0922198482054,
-5.02702365776805,-4.9830435683078,-4.83945447753678,-4.70766533110664,
-4.67208618909627,-4.65316940855279,-4.63226428501289,-4.59703789099837,
-4.42032405949409,-4.34154390172734,-4.23761631495814,-4.19022786076316,
-4.15296687672001,-4.10961863244128,-4.02495046492125,-3.82755257418756,
-3.7266387684387,-3.6970509612286,-3.67710061387468,-3.65336156746934,-3.60294539519532,
-3.44449865278867,-3.27845839873617,-3.23226040626606,-3.19440753104968,
-3.15456903235772,-3.09022638220154,-3.0470830704392,-2.90822062929407,
-2.84901726335752,-2.75694936493455,-2.72759521858757,-2.70767440564304,
-2.68380864659361,-2.63263287327469,-2.47402511406729,-2.30942096653791,
-2.26316889515377,-2.2253042136077,-2.18548599498706,-2.12125537850627,
-2.07822126784755,-1.93996303018653,-1.88739961108352,-1.78860071682233,
-1.75885926938661,-1.73888901059928,-1.71523115206963,-1.66529595529032,
-1.62550000660333,-1.45109008988929,-1.33257085340842,-1.2847708639072,
-1.2474088803859,-1.23704712794801,-1.23271077082133,-1.22810693380001,
-1.18084215915745,-1.12292612799538,-1.00764929421452,-0.825471155663644,
-0.792760620363109,-0.774333300655851,-0.759230550740772,-0.73650450015082,
-0.6598266807045,-0.49922070704633,-0.366888604665163,-0.317766506712928,
-0.280259080447408,-0.245357825619976,-0.203857388925526,-4.21440357605785E-5),
 .UNSPECIFIED.) ;
#225=B_SPLINE_CURVE_WITH_KNOTS('',3,(#24356,#24357,#24358,#24359,#24360,
#24361,#24362,#24363,#24364,#24365,#24366,#24367,#24368,#24369,#24370,#24371,
#24372,#24373,#24374,#24375,#24376,#24377,#24378,#24379,#24380,#24381,#24382,
#24383,#24384,#24385,#24386,#24387,#24388,#24389,#24390,#24391,#24392,#24393,
#24394,#24395,#24396,#24397,#24398,#24399,#24400,#24401,#24402,#24403,#24404,
#24405,#24406,#24407,#24408,#24409,#24410,#24411,#24412,#24413,#24414,#24415,
#24416,#24417,#24418,#24419,#24420,#24421,#24422,#24423,#24424,#24425,#24426,
#24427,#24428,#24429,#24430,#24431,#24432,#24433,#24434,#24435,#24436,#24437,
#24438,#24439,#24440,#24441,#24442,#24443,#24444,#24445,#24446,#24447,#24448,
#24449,#24450,#24451,#24452,#24453,#24454,#24455,#24456,#24457,#24458,#24459,
#24460,#24461,#24462,#24463,#24464,#24465,#24466,#24467,#24468,#24469,#24470,
#24471,#24472,#24473,#24474,#24475,#24476,#24477,#24478,#24479,#24480,#24481,
#24482,#24483,#24484,#24485,#24486,#24487,#24488,#24489,#24490,#24491,#24492,
#24493,#24494,#24495,#24496,#24497,#24498,#24499,#24500,#24501,#24502,#24503,
#24504,#24505,#24506,#24507,#24508,#24509,#24510,#24511,#24512,#24513,#24514,
#24515,#24516,#24517,#24518,#24519,#24520,#24521,#24522,#24523,#24524,#24525,
#24526,#24527,#24528,#24529,#24530,#24531,#24532,#24533,#24534,#24535,#24536,
#24537,#24538,#24539,#24540,#24541,#24542,#24543,#24544,#24545,#24546,#24547,
#24548,#24549,#24550,#24551,#24552,#24553,#24554,#24555,#24556,#24557,#24558,
#24559,#24560,#24561,#24562,#24563,#24564,#24565,#24566,#24567,#24568,#24569,
#24570,#24571,#24572,#24573,#24574,#24575,#24576,#24577,#24578,#24579,#24580,
#24581,#24582,#24583,#24584,#24585,#24586,#24587,#24588,#24589,#24590,#24591,
#24592,#24593,#24594,#24595,#24596,#24597,#24598,#24599,#24600,#24601,#24602,
#24603,#24604,#24605,#24606,#24607,#24608,#24609,#24610,#24611,#24612,#24613,
#24614,#24615,#24616,#24617,#24618,#24619,#24620,#24621,#24622,#24623,#24624,
#24625,#24626,#24627,#24628,#24629,#24630,#24631,#24632,#24633,#24634,#24635,
#24636,#24637,#24638,#24639,#24640,#24641,#24642,#24643,#24644,#24645,#24646,
#24647,#24648,#24649,#24650,#24651,#24652,#24653,#24654,#24655,#24656,#24657,
#24658,#24659,#24660,#24661,#24662,#24663,#24664,#24665,#24666,#24667,#24668,
#24669,#24670,#24671,#24672,#24673,#24674,#24675,#24676,#24677,#24678,#24679,
#24680,#24681,#24682,#24683,#24684,#24685,#24686,#24687,#24688,#24689,#24690,
#24691,#24692,#24693,#24694,#24695,#24696,#24697,#24698,#24699,#24700,#24701,
#24702,#24703,#24704,#24705,#24706,#24707),.UNSPECIFIED.,.F.,.F.,(4,2,2,
2,2,2,2,2,2,2,2,2,2,2,2,2,2,2,2,2,2,2,2,2,2,2,2,2,2,2,2,2,2,2,2,2,2,2,2,
2,2,2,2,2,2,2,2,2,2,2,2,2,2,2,2,2,2,2,2,2,2,2,2,2,2,2,2,2,2,2,2,2,2,2,2,
2,2,2,2,2,2,2,2,2,2,2,2,2,2,2,2,2,2,2,2,2,2,2,2,2,2,2,2,2,2,2,2,2,2,2,2,
2,2,2,2,2,2,2,2,2,2,2,2,2,2,2,2,2,2,2,2,2,2,2,2,2,2,2,2,2,2,2,2,2,2,2,2,
2,2,2,2,2,2,2,2,2,2,2,2,2,2,2,2,2,2,2,2,2,2,2,2,2,2,2,2,4),(2.18817716271853,
2.27258985578313,2.31604363060642,2.38083993956034,2.42101112656157,2.45925672133389,
2.50608966252046,2.67030192185054,2.80070882856306,2.84896253681468,2.88582472444221,
2.90720085914843,2.92594015309928,2.96052122729631,3.13558019513664,3.29691169508635,
3.35412793258946,3.39256123443125,3.42709759077454,3.48388809280466,3.63441718908193,
3.76995307059931,3.84067309963547,3.86719537629394,3.88681756102699,3.9120457363662,
3.96990045621053,4.22743789373958,4.30759701363214,4.35027338084236,4.38772330967091,
4.43562518983659,4.5500003783448,4.72657464056413,4.7665750812795,4.81670405179479,
4.84044726256082,4.86045284261538,4.89026606925306,4.98883636689778,5.18495913352847,
5.2462668736371,5.29914506260869,5.33701066629752,5.37757909946605,5.44608794428359,
5.68485825800973,5.74625569619831,5.78987912174619,5.81239607270393,5.83250681328118,
5.86453556595654,6.0535504441511,6.1656218068973,6.24536847052205,6.28791548716059,
6.32528363131567,6.37310775308717,6.49117238849288,6.66574065634653,6.70554889136079,
6.75549574276886,6.77916055802478,6.79913681140632,6.82889398711347,6.92755915224754,
6.9646146930374,7.07893349649339,7.19783297962598,7.24568051399259,7.28297798784249,
7.32602002229107,7.40877437224083,7.61642909110148,7.71021325152551,7.73974802479294,
7.75969129539594,7.78345667537042,7.83403679037394,7.99229976566751,8.15831221921274,
8.20449621568462,8.24234309080218,8.28218038007358,8.34653217890775,8.38968559157436,
8.52860532650486,8.58521464561437,8.679350844392,8.70891274535028,8.72885850696504,
8.75260920747026,8.80309335979099,8.96146589839134,9.12751138397173,9.17369993230231,
9.21155217066301,9.25139742988831,9.31577013706904,9.35894245804052,9.49796962270571,
9.54934695754393,9.64811878745205,9.67786314318781,9.69783460214745,9.72149243353714,
9.77142886870925,9.81122661178085,9.98565408529672,10.1041854649933,10.1519711614567,
10.189330449529,10.2318884386356,10.3117264710507,10.4240185480195,10.612574726657,
10.644619733548,10.6647404808281,10.6872974545491,10.7310286658147,10.7637600340689,
10.8843189994301,10.9390691633499,11.0698512951672,11.1189664111175,11.1564731071566,
11.1982887945662,11.273753523903,11.3764315412984,11.5759792595209,11.6110296504896,
11.6298532425524,11.6508654825314,11.6866422059215,11.8081309959872,12.030510862482,
12.0836747704508,12.1216061472386,12.1621272563688,12.2302642106318,12.2771873613173,
12.4389310397248,12.5454060943917,12.5803373501216,12.599139745995,12.6201769173334,
12.6560810550213,12.7787069726977,12.9987615041652,13.0523392943701,13.0903327787884,
13.125102134132,13.179271971074,13.2485400062385,13.4155621854189,13.5241216925213,
13.5542315609061,13.573930635645,13.5888938238053,13.5907128182226,13.5925919389256,
13.5945711446099,13.5966932123652,13.5990062508306,13.6015661956319,13.602590316265,
13.6039528520496,13.6336689090568,13.6892734768506,13.8691088931611,13.9813352653587,
14.0289878310402,14.0663352143452,14.1013385267474,14.143671946755,14.3953830185734),
 .UNSPECIFIED.) ;
#226=B_SPLINE_CURVE_WITH_KNOTS('',3,(#24712,#24713,#24714,#24715,#24716,
#24717,#24718,#24719,#24720,#24721,#24722,#24723,#24724,#24725,#24726,#24727,
#24728,#24729,#24730,#24731,#24732,#24733,#24734,#24735,#24736,#24737,#24738,
#24739,#24740,#24741,#24742,#24743,#24744,#24745,#24746,#24747,#24748,#24749,
#24750,#24751,#24752,#24753,#24754,#24755,#24756,#24757,#24758,#24759,#24760,
#24761,#24762,#24763,#24764,#24765,#24766,#24767,#24768,#24769,#24770,#24771,
#24772,#24773,#24774,#24775,#24776,#24777,#24778,#24779,#24780,#24781,#24782,
#24783,#24784,#24785,#24786,#24787,#24788,#24789,#24790,#24791,#24792,#24793,
#24794,#24795,#24796,#24797,#24798,#24799,#24800,#24801,#24802,#24803,#24804,
#24805,#24806,#24807,#24808,#24809,#24810,#24811,#24812,#24813,#24814,#24815,
#24816,#24817,#24818,#24819,#24820,#24821,#24822,#24823,#24824,#24825,#24826,
#24827,#24828,#24829,#24830,#24831,#24832,#24833,#24834,#24835,#24836,#24837,
#24838,#24839,#24840,#24841,#24842,#24843,#24844,#24845,#24846,#24847,#24848,
#24849,#24850,#24851,#24852,#24853,#24854,#24855,#24856,#24857,#24858,#24859,
#24860,#24861,#24862,#24863,#24864,#24865,#24866,#24867,#24868,#24869,#24870,
#24871,#24872,#24873,#24874,#24875,#24876,#24877,#24878,#24879,#24880,#24881,
#24882,#24883,#24884,#24885,#24886,#24887,#24888,#24889,#24890,#24891,#24892,
#24893,#24894,#24895,#24896,#24897,#24898,#24899,#24900,#24901,#24902,#24903,
#24904,#24905,#24906,#24907,#24908,#24909,#24910,#24911,#24912,#24913,#24914,
#24915,#24916,#24917,#24918,#24919,#24920,#24921,#24922,#24923,#24924,#24925,
#24926,#24927,#24928,#24929,#24930,#24931,#24932,#24933,#24934,#24935,#24936,
#24937,#24938,#24939,#24940,#24941,#24942,#24943,#24944,#24945,#24946,#24947,
#24948,#24949,#24950,#24951,#24952,#24953,#24954,#24955,#24956,#24957,#24958,
#24959,#24960,#24961,#24962,#24963,#24964,#24965,#24966,#24967,#24968,#24969,
#24970,#24971,#24972,#24973,#24974,#24975,#24976,#24977,#24978,#24979,#24980,
#24981,#24982,#24983,#24984,#24985,#24986,#24987,#24988,#24989,#24990,#24991,
#24992,#24993,#24994,#24995,#24996,#24997,#24998,#24999,#25000,#25001,#25002,
#25003,#25004,#25005,#25006,#25007,#25008,#25009,#25010,#25011,#25012,#25013,
#25014,#25015),.UNSPECIFIED.,.F.,.F.,(4,3,3,3,3,3,3,3,3,3,3,3,3,3,3,3,3,
3,3,3,3,3,3,3,3,3,3,3,3,3,3,3,3,3,3,3,3,3,3,3,3,3,3,3,3,3,3,3,3,3,3,3,3,
3,3,3,3,3,3,3,3,3,3,3,3,3,3,3,3,3,3,3,3,3,3,3,3,3,3,3,3,3,3,3,3,3,3,3,3,
3,3,3,3,3,3,3,3,3,3,3,3,4),(-16.6593614944316,-16.5954782572781,-16.5289225612824,
-16.4623668652867,-16.4000094150394,-16.3376992006281,-16.2753956730767,
-16.2130959318694,-16.1506987647291,-16.0883926326437,-16.025949947976,
-15.9635072633083,-15.901149813061,-15.8388395986498,-15.7765360710986,
-15.7142363298915,-15.6518391627511,-15.5895330306658,-15.5270903459979,
-15.4646476613299,-15.4022902110826,-15.3399799966714,-15.2776764691201,
-15.2153767279131,-15.1529795607727,-15.0906734286873,-15.0282307440194,
-14.9657880593515,-14.9034306091042,-14.841120394693,-14.7788168671418,
-14.7165171259347,-14.6541199587943,-14.5918138267091,-14.5293711420411,
-14.4669284573731,-14.4045710071258,-14.3422607927144,-14.2799572651628,
-14.2176575239555,-14.1552603568154,-14.0929542247299,-14.0305115400623,
-13.9680688553948,-13.9057114051475,-13.8434011907372,-13.7810976631868,
-13.7187979219806,-13.6564007548396,-13.5940946227552,-13.5316519380858,
-13.4692092534164,-13.4068518031691,-13.3445415887561,-13.282238061203,
-13.2199383199941,-13.1575411528551,-13.0952350207681,-13.0327923361031,
-12.970349651438,-12.9079922011907,-12.8456819867821,-12.7833784592334,
-12.7210787180288,-12.6586815508865,-12.5963754188038,-12.5339327341317,
-12.4714900494596,-12.4091325992123,-12.3468223847994,-12.2845188572466,
-12.2222191160378,-12.1598219488986,-12.0975158168117,-12.0350731321465,
-11.9726304474812,-11.9102729972339,-11.8479627828177,-11.7856592552614,
-11.7233595140491,-11.6609623469126,-11.5986562148222,-11.5362135301625,
-11.4737708455028,-11.4114133952555,-11.3491031808696,-11.2867996533438,
-11.2244999121623,-11.1621027450028,-11.0997966129428,-11.0373539282336,
-10.9749112435245,-10.9125537932772,-10.8502435787957,-10.7879400511739,
-10.7256403098962,-10.6632431428086,-10.6009370106539,-10.5384943261,-10.4760516415461,
-10.4098345567239,-10.3761761872893),.UNSPECIFIED.) ;
#227=B_SPLINE_CURVE_WITH_KNOTS('',3,(#25016,#25017,#25018,#25019,#25020,
#25021,#25022,#25023,#25024,#25025,#25026,#25027,#25028,#25029,#25030,#25031,
#25032,#25033,#25034,#25035,#25036,#25037,#25038,#25039,#25040,#25041,#25042,
#25043,#25044,#25045,#25046,#25047,#25048,#25049,#25050,#25051,#25052,#25053,
#25054,#25055,#25056,#25057,#25058,#25059,#25060,#25061,#25062,#25063,#25064,
#25065,#25066,#25067,#25068,#25069,#25070,#25071,#25072,#25073,#25074,#25075,
#25076,#25077,#25078,#25079,#25080,#25081,#25082,#25083,#25084,#25085,#25086,
#25087,#25088,#25089,#25090,#25091,#25092,#25093,#25094,#25095,#25096,#25097,
#25098,#25099,#25100,#25101,#25102,#25103,#25104,#25105,#25106,#25107,#25108,
#25109,#25110,#25111,#25112,#25113,#25114,#25115,#25116,#25117,#25118,#25119,
#25120,#25121,#25122,#25123,#25124,#25125,#25126,#25127,#25128,#25129,#25130,
#25131,#25132,#25133,#25134,#25135,#25136,#25137,#25138,#25139,#25140,#25141,
#25142,#25143,#25144,#25145,#25146,#25147,#25148,#25149,#25150,#25151,#25152,
#25153,#25154,#25155,#25156,#25157,#25158,#25159,#25160,#25161,#25162,#25163,
#25164,#25165,#25166,#25167,#25168,#25169,#25170,#25171,#25172,#25173,#25174,
#25175,#25176,#25177,#25178,#25179,#25180,#25181,#25182,#25183,#25184,#25185,
#25186,#25187,#25188,#25189,#25190,#25191,#25192,#25193,#25194,#25195,#25196,
#25197,#25198,#25199,#25200,#25201,#25202,#25203,#25204,#25205,#25206,#25207,
#25208,#25209,#25210,#25211,#25212,#25213,#25214,#25215,#25216,#25217,#25218,
#25219,#25220,#25221,#25222,#25223,#25224,#25225,#25226,#25227,#25228,#25229,
#25230,#25231,#25232,#25233,#25234,#25235,#25236,#25237,#25238,#25239,#25240,
#25241,#25242,#25243,#25244,#25245,#25246,#25247,#25248,#25249,#25250,#25251,
#25252,#25253,#25254,#25255,#25256,#25257,#25258,#25259,#25260,#25261,#25262,
#25263,#25264,#25265,#25266,#25267,#25268,#25269,#25270,#25271,#25272,#25273,
#25274,#25275,#25276,#25277,#25278,#25279,#25280,#25281,#25282,#25283,#25284,
#25285,#25286,#25287,#25288,#25289,#25290,#25291,#25292,#25293,#25294,#25295,
#25296,#25297,#25298,#25299,#25300,#25301,#25302,#25303,#25304,#25305,#25306,
#25307,#25308,#25309,#25310,#25311,#25312,#25313,#25314,#25315,#25316,#25317,
#25318,#25319,#25320,#25321,#25322,#25323,#25324,#25325,#25326,#25327,#25328,
#25329,#25330,#25331,#25332,#25333,#25334,#25335,#25336,#25337,#25338,#25339,
#25340,#25341,#25342,#25343,#25344,#25345,#25346,#25347,#25348,#25349,#25350,
#25351,#25352,#25353,#25354,#25355,#25356,#25357,#25358,#25359,#25360,#25361,
#25362,#25363,#25364,#25365,#25366,#25367,#25368,#25369,#25370,#25371,#25372,
#25373,#25374,#25375,#25376,#25377,#25378,#25379,#25380,#25381,#25382,#25383,
#25384,#25385,#25386,#25387,#25388,#25389,#25390,#25391,#25392,#25393,#25394,
#25395,#25396,#25397,#25398,#25399,#25400,#25401,#25402,#25403,#25404,#25405),
 .UNSPECIFIED.,.F.,.F.,(4,2,2,2,2,2,2,2,2,2,2,2,2,2,2,2,2,2,2,2,2,2,2,2,
2,2,2,2,2,2,2,2,2,2,2,2,2,2,2,2,2,2,2,2,2,2,2,2,2,2,2,2,2,2,2,2,2,2,2,2,
2,2,2,2,2,2,2,2,2,2,2,2,2,2,2,2,2,2,2,2,2,2,2,2,2,2,2,2,2,2,2,2,2,2,2,2,
2,2,2,2,2,2,2,2,2,2,2,2,2,2,2,2,2,2,2,2,2,2,2,2,2,2,2,2,2,2,2,2,2,2,2,2,
2,2,2,2,2,2,2,2,2,2,2,2,2,2,2,2,2,2,2,2,2,2,2,2,2,2,2,2,2,2,2,2,2,2,2,2,
2,2,2,2,2,2,2,2,2,2,2,2,2,2,2,2,2,2,2,2,2,2,2,2,2,2,4),(6.54590052552168E-5,
0.0660743354571956,0.103646198129629,0.1252023219725,0.143355746835144,
0.16207812232254,0.196548198026947,0.364599260483942,0.530414938452012,
0.563373596596461,0.589086313045187,0.623967302147303,0.661850038598023,
0.708184547062534,0.96964444084449,1.03777847100332,1.07140718005652,1.09885832328466,
1.11306927385535,1.13190624320692,1.16703366806672,1.33681292915678,1.45677425094401,
1.51591602316336,1.52067111789573,1.52476468859033,1.52832269269611,1.53144559951978,
1.53421362971229,1.53669108928998,1.5389298436005,1.54097205554933,1.54285232749387,
1.54459937456026,1.54623733703716,1.54778681886104,1.54926572133688,1.55068992711668,
1.55207387897404,1.55343109095958,1.55477462589866,1.55611757297875,1.55747356314925,
1.5588573698539,1.59408144255242,1.63209985338781,1.67903832309788,1.84154000799963,
2.00028928923424,2.05155362069965,2.07543402909437,2.09535154223313,2.12467914335601,
2.21652710044626,2.24569141154283,2.4050812360259,2.45164657977742,2.51943120454188,
2.55988944332175,2.59784982310284,2.65120519507239,2.87248814984226,2.99452113975738,
3.03035923015238,3.05138364080831,3.07019711407189,3.10519029423227,3.2124988329447,
3.22937708618387,3.37879241285159,3.42376313105816,3.48995977422986,3.53013228964512,
3.56780382128332,3.62173376307465,3.83971854740559,3.96339735836579,3.99941880927593,
4.0204793111109,4.03926364197498,4.07408997537889,4.17913571272868,4.21352263299063,
4.35297971909989,4.39622995004449,4.46068209329239,4.50054032269965,4.53838163473991,
4.59340962187226,4.7035779351548,4.77050878541039,4.88795941750521,4.95349857385879,
4.97948430158276,4.99918292756109,5.02515497019942,5.08560122530602,5.17513098832738,
5.31957831295779,5.36370711060574,5.42905416069796,5.46907362879258,5.50682450200796,
5.55255303132238,5.6790786642144,5.84209677309376,5.88062597494018,5.92949393068853,
5.95296982544281,5.97298923678071,6.00309139095167,6.1069188961213,6.24168575063817,
6.3286708128752,6.39630705601036,6.43673881669355,6.47471170407527,6.52814902418533,
6.74898021993785,6.87123375025607,6.90709669588237,6.92812608271242,6.94693571741768,
6.98190649947664,7.08890827239652,7.25023590060713,7.29709675142791,7.36517279691773,
7.40568360148085,7.44362079455436,7.49681933001752,7.7190028270069,7.84059300385476,
7.87638152186083,7.89739631457088,7.9162180052221,7.95125752430234,8.1508609250141,
8.25353079054083,8.328992286189,8.37080771702598,8.40831483255875,8.45743136325945,
8.58895408285465,8.64289928696326,8.76350317435513,8.80985943264742,8.84560889744294,
8.86661597948867,8.88544394006687,8.9205194826862,9.10716755185701,9.12225749881739,
9.2236941365127,9.29857174501226,9.3402859599525,9.37781742511362,9.42713395574194,
9.5644409129488,9.72075816499905,9.75848990013041,9.80667613990164,9.83003414494448,
9.85008828593659,9.88043509359002,9.99059322055077,10.156125442796,10.2036112691254,
10.2359891066826,10.2886633017569,10.3265234965363,10.3672152888013,10.4363011155497,
10.6736725170651,10.734943384144,10.7785105700521,10.8010374018716,10.8211737117607,
10.8533063210872,11.0415303876383,11.18253517616,11.2460005498542,11.2856813892659,
11.3236317291432,11.3702673983871,11.533682275802,11.6923778519106,11.743607978469,
11.7674829130203,11.7874019596289,11.8167403325837,11.9086749671978,12.0355647832628,
12.1338726876243,12.2072456703103),.UNSPECIFIED.) ;
#228=B_SPLINE_CURVE_WITH_KNOTS('',3,(#25410,#25411,#25412,#25413,#25414,
#25415,#25416,#25417,#25418,#25419,#25420,#25421,#25422,#25423,#25424,#25425,
#25426,#25427,#25428,#25429,#25430,#25431,#25432,#25433,#25434,#25435,#25436,
#25437,#25438,#25439,#25440,#25441,#25442,#25443,#25444,#25445,#25446,#25447,
#25448,#25449,#25450,#25451,#25452,#25453,#25454,#25455,#25456,#25457,#25458,
#25459,#25460,#25461,#25462,#25463,#25464,#25465,#25466,#25467,#25468,#25469,
#25470,#25471,#25472,#25473,#25474,#25475,#25476,#25477,#25478,#25479,#25480,
#25481,#25482,#25483,#25484,#25485,#25486,#25487,#25488,#25489,#25490,#25491,
#25492,#25493,#25494,#25495,#25496,#25497,#25498,#25499,#25500,#25501,#25502,
#25503,#25504,#25505,#25506,#25507,#25508,#25509,#25510,#25511,#25512,#25513,
#25514,#25515,#25516,#25517,#25518,#25519,#25520,#25521,#25522,#25523,#25524,
#25525,#25526,#25527,#25528,#25529,#25530,#25531,#25532,#25533,#25534,#25535,
#25536,#25537,#25538,#25539,#25540,#25541,#25542,#25543,#25544,#25545,#25546,
#25547,#25548,#25549,#25550,#25551,#25552,#25553,#25554,#25555,#25556,#25557,
#25558,#25559,#25560,#25561,#25562,#25563,#25564,#25565,#25566,#25567,#25568,
#25569,#25570,#25571,#25572,#25573,#25574,#25575,#25576,#25577,#25578,#25579,
#25580,#25581,#25582,#25583,#25584,#25585,#25586,#25587,#25588,#25589,#25590,
#25591,#25592,#25593,#25594,#25595,#25596,#25597,#25598,#25599,#25600,#25601,
#25602,#25603,#25604,#25605,#25606,#25607,#25608,#25609,#25610,#25611,#25612,
#25613,#25614,#25615,#25616,#25617,#25618,#25619,#25620,#25621,#25622,#25623,
#25624,#25625,#25626,#25627,#25628,#25629,#25630,#25631,#25632,#25633,#25634,
#25635,#25636,#25637,#25638,#25639,#25640,#25641,#25642,#25643,#25644,#25645,
#25646,#25647,#25648,#25649,#25650,#25651,#25652,#25653,#25654,#25655,#25656,
#25657,#25658,#25659,#25660,#25661,#25662,#25663,#25664,#25665,#25666,#25667,
#25668,#25669,#25670,#25671,#25672,#25673,#25674,#25675,#25676,#25677,#25678,
#25679,#25680,#25681,#25682,#25683,#25684,#25685,#25686,#25687,#25688,#25689,
#25690,#25691,#25692,#25693,#25694,#25695,#25696,#25697,#25698,#25699,#25700,
#25701,#25702,#25703,#25704,#25705,#25706,#25707,#25708,#25709,#25710,#25711,
#25712,#25713,#25714,#25715,#25716,#25717,#25718,#25719,#25720,#25721,#25722,
#25723,#25724,#25725,#25726,#25727,#25728,#25729,#25730,#25731,#25732,#25733,
#25734,#25735,#25736,#25737,#25738,#25739,#25740,#25741,#25742,#25743,#25744,
#25745,#25746,#25747,#25748,#25749,#25750,#25751,#25752,#25753,#25754,#25755,
#25756,#25757,#25758,#25759,#25760,#25761,#25762,#25763,#25764,#25765,#25766,
#25767,#25768,#25769,#25770,#25771,#25772,#25773,#25774,#25775,#25776,#25777,
#25778,#25779,#25780,#25781,#25782,#25783,#25784,#25785,#25786,#25787,#25788,
#25789,#25790,#25791,#25792,#25793,#25794,#25795,#25796,#25797,#25798,#25799,
#25800,#25801,#25802,#25803,#25804,#25805,#25806,#25807,#25808,#25809,#25810,
#25811,#25812,#25813,#25814,#25815,#25816,#25817,#25818,#25819,#25820,#25821,
#25822,#25823,#25824,#25825,#25826,#25827,#25828,#25829,#25830,#25831,#25832,
#25833,#25834,#25835,#25836,#25837,#25838,#25839,#25840,#25841,#25842,#25843,
#25844,#25845,#25846,#25847,#25848,#25849,#25850,#25851,#25852,#25853,#25854,
#25855,#25856,#25857,#25858,#25859,#25860,#25861,#25862,#25863,#25864,#25865,
#25866,#25867,#25868,#25869,#25870,#25871,#25872,#25873,#25874,#25875,#25876,
#25877,#25878,#25879,#25880,#25881),.UNSPECIFIED.,.F.,.F.,(4,2,2,2,2,2,
2,2,2,2,2,2,2,2,2,2,2,2,2,2,2,2,2,2,2,2,2,2,2,2,2,2,2,2,2,2,2,2,2,2,2,2,
2,2,2,2,2,2,2,2,2,2,2,2,2,2,2,2,2,2,2,2,2,2,2,2,2,2,2,2,2,2,2,2,2,2,2,2,
2,2,2,2,2,2,2,2,2,2,2,2,2,2,2,2,2,2,2,2,2,2,2,2,2,2,2,2,2,2,2,2,2,2,2,2,
2,2,2,2,2,2,2,2,2,2,2,2,2,2,2,2,2,2,2,2,2,2,2,2,2,2,2,2,2,2,2,2,2,2,2,2,
2,2,2,2,2,2,2,2,2,2,2,2,2,2,2,2,2,2,2,2,2,2,2,2,2,2,2,2,2,2,2,2,2,2,2,2,
2,2,2,2,2,2,2,2,2,2,2,2,2,2,2,2,2,2,2,2,2,2,2,2,2,2,2,2,2,2,2,2,2,2,2,2,
2,2,2,2,2,2,2,2,2,2,2,2,2,4),(12.2072906505637,12.2333995230658,12.2998920652981,
12.4204853076344,12.4746294858109,12.6059734111218,12.6550894061824,12.6925963981913,
12.7344119738802,12.8098747078753,12.9125471786017,13.1121343210669,13.1471771244674,
13.1659993677865,13.1870133994815,13.2227982146858,13.3443555734894,13.5666085535278,
13.619795761001,13.6577312089582,13.6982456861688,13.7663425696405,13.8132246011097,
13.9746937416869,14.0815144599795,14.1164717439445,14.1352789917533,14.1563111994805,
14.1921886888268,14.3145723171371,14.5351379620659,14.5886240749683,14.6266042491524,
14.6670199966474,14.7345675613066,14.8213843933541,14.9480065971356,15.0604443260453,
15.0904788517653,15.1104888354367,15.1339980265039,15.18306001687,15.2218179084713,
15.3868202369665,15.5148871547583,15.5635152706309,15.6009650600216,15.6430383627059,
15.7200011187959,15.8258947711875,15.8926597645677,15.9399753637726,16.0312743658349,
16.0605325499453,16.0804416019661,16.1043607935269,16.1558597319316,16.3149858635752,
16.4701698017627,16.5251213385783,16.562950421573,16.6028289716119,16.6673950459589,
16.7107567540235,16.8508379093865,16.8761607749545,16.906370006885,16.9999039644488,
17.0294141907173,17.0493544398992,17.0731346433331,17.1237973782612,17.2819685123973,
17.4479777167766,17.4941531132684,17.5320007288664,17.571847058112,17.6362348917337,
17.6794224762023,17.8185324364809,17.8665906361654,17.9370164162362,17.9846775334201,
18.0079436938594,18.0280262756519,18.0585692200623,18.1838462680258,18.4180055990733,
18.4638778223217,18.501659307889,18.5416213709074,18.6066518327291,18.6504690683125,
18.7931269099642,18.823958030315,18.9278349860858,18.9625848584942,18.9813557107571,
19.0024326816713,19.0385385652653,19.1629850145529,19.3799199640003,19.4339055464632,
19.471585145455,19.5117401022612,19.5778412768407,19.6227172196298,19.7715658839122,
19.8021551667263,19.9062357434439,19.9363309993209,19.9563491777512,19.9798277948077,
20.0287130877471,20.0672630437681,20.2304614994038,20.3560953414037,20.4020660760878,
20.4398687809886,20.4797923610338,20.5446100498309,20.7116044997462,20.7573909757551,
20.865623977585,20.9006842262204,20.9195092636372,20.9405190157294,20.9762835009882,
21.0008894822945,21.1590469701795,21.3248235295797,21.3709615298301,21.4088007590458,
21.4486607337168,21.5131253400588,21.5563880460295,21.695916972558,21.727860631611,
21.8349492965941,21.8699257819381,21.8887361337303,21.9097636543885,21.9456187257387,
22.0678060336367,22.2887686798031,22.3421808380487,22.380149271758,22.4205879504804,
22.4882662660198,22.575331937019,22.7019456534822,22.8139126481655,22.8439389453787,
22.8639474710601,22.8796255428054,22.8798710868697,22.8801208893376,22.8803751977609,
22.8806342700849,22.8808983754389,22.8811677948888,22.8814428223748,22.8817237656049,
22.8820109469831,22.8823047046758,22.882605393669,22.8829133869871,22.8832290768713,
22.8835528761049,22.8838852194455,22.8842265651085,22.8845773963741,22.8849382232655,
22.8853095843748,22.8856920488534,22.8860862184288,22.8864927296133,22.8869122561194,
22.8873455113299,22.8877932510179,22.8882562762144,22.8887354362864,22.8892316322082,
22.8897458200612,22.8902790147546,22.8908322940296,22.8914068027022,22.8920037571857,
22.8926244503446,22.893270256656,22.8939426377042,22.8946431480831,22.8953734416365,
22.8961352781657,22.8963728185666,22.8966383520258,22.8969353318644,22.8972676697636,
22.8976398025119,22.8980567694588,22.8985243020402,22.8990489274648,22.8996380885287,
22.9003002817726,22.901045216305,22.9018839955778,22.9028293242095,22.9038957414864,
22.9050998824483,22.9064607661696,22.9080001089037,22.9097426571472,22.9117165315429,
22.9553119449238,23.0625266937836,23.2514205529398,23.3077527107458,23.3454329646705,
23.3777691992466,23.4269424204246,23.4879482197223,23.5553218510742,23.6819455263177,
23.7834993556504,23.8133239900265,23.8333050193339,23.8519007961556,23.8816510206883,
23.8896786880865,23.9833988046422,24.1196332017496,24.2390329191062,24.2870761464822,
24.3229922517165,24.3578991392153,24.4142930285787),.UNSPECIFIED.) ;
#229=B_SPLINE_CURVE_WITH_KNOTS('',3,(#25882,#25883,#25884,#25885,#25886,
#25887,#25888,#25889,#25890,#25891,#25892,#25893,#25894,#25895,#25896,#25897,
#25898,#25899,#25900,#25901,#25902,#25903,#25904,#25905,#25906,#25907,#25908,
#25909,#25910,#25911,#25912,#25913,#25914,#25915,#25916,#25917,#25918,#25919,
#25920,#25921,#25922,#25923,#25924,#25925,#25926,#25927,#25928,#25929,#25930,
#25931,#25932,#25933,#25934,#25935,#25936,#25937,#25938,#25939,#25940,#25941,
#25942,#25943,#25944,#25945,#25946,#25947,#25948,#25949,#25950,#25951,#25952,
#25953,#25954,#25955,#25956,#25957,#25958,#25959,#25960,#25961,#25962,#25963,
#25964,#25965,#25966,#25967,#25968,#25969,#25970,#25971,#25972,#25973,#25974,
#25975,#25976,#25977,#25978,#25979,#25980,#25981,#25982,#25983,#25984,#25985,
#25986,#25987,#25988,#25989,#25990,#25991,#25992,#25993,#25994,#25995,#25996,
#25997,#25998,#25999,#26000,#26001,#26002,#26003,#26004,#26005,#26006,#26007,
#26008,#26009,#26010,#26011,#26012,#26013,#26014,#26015,#26016,#26017,#26018,
#26019,#26020,#26021,#26022,#26023,#26024,#26025,#26026,#26027,#26028,#26029,
#26030,#26031,#26032,#26033,#26034,#26035,#26036,#26037,#26038,#26039,#26040,
#26041,#26042,#26043,#26044,#26045,#26046,#26047,#26048,#26049,#26050,#26051,
#26052,#26053,#26054,#26055,#26056,#26057,#26058,#26059,#26060,#26061,#26062,
#26063,#26064,#26065,#26066,#26067,#26068,#26069,#26070,#26071,#26072,#26073,
#26074,#26075,#26076,#26077,#26078,#26079,#26080,#26081,#26082,#26083,#26084,
#26085,#26086,#26087,#26088,#26089,#26090,#26091,#26092,#26093,#26094,#26095,
#26096,#26097,#26098,#26099,#26100,#26101,#26102,#26103,#26104,#26105,#26106,
#26107,#26108,#26109,#26110,#26111,#26112,#26113,#26114,#26115,#26116,#26117,
#26118,#26119,#26120,#26121,#26122,#26123,#26124,#26125,#26126,#26127,#26128,
#26129,#26130,#26131,#26132,#26133,#26134,#26135,#26136,#26137,#26138,#26139,
#26140,#26141,#26142,#26143,#26144,#26145,#26146,#26147,#26148,#26149,#26150,
#26151,#26152,#26153,#26154,#26155,#26156,#26157,#26158,#26159,#26160,#26161,
#26162,#26163,#26164,#26165,#26166,#26167,#26168,#26169,#26170,#26171,#26172,
#26173,#26174,#26175,#26176,#26177,#26178,#26179,#26180,#26181,#26182,#26183,
#26184,#26185,#26186,#26187,#26188,#26189,#26190,#26191,#26192,#26193,#26194,
#26195,#26196,#26197,#26198,#26199,#26200,#26201,#26202,#26203,#26204,#26205,
#26206,#26207,#26208,#26209,#26210,#26211,#26212,#26213,#26214,#26215,#26216,
#26217,#26218,#26219,#26220,#26221,#26222,#26223,#26224,#26225,#26226,#26227,
#26228,#26229,#26230,#26231,#26232,#26233,#26234,#26235),.UNSPECIFIED.,
 .F.,.F.,(4,2,2,2,2,2,2,2,2,2,2,2,2,2,2,2,2,2,2,2,2,2,2,2,2,2,2,2,2,2,2,
2,2,2,2,2,2,2,2,2,2,2,2,2,2,2,2,2,2,2,2,2,2,2,2,2,2,2,2,2,2,2,2,2,2,2,2,
2,2,2,2,2,2,2,2,2,2,2,2,2,2,2,2,2,2,2,2,2,2,2,2,2,2,2,2,2,2,2,2,2,2,2,2,
2,2,2,2,2,2,2,2,2,2,2,2,2,2,2,2,2,2,2,2,2,2,2,2,2,2,2,2,2,2,2,2,2,2,2,2,
2,2,2,2,2,2,2,2,2,2,2,2,2,2,2,2,2,2,2,2,2,2,2,2,2,2,2,2,2,2,2,2,2,2,2,2,
2,4),(12.2072456703103,12.2486977382348,12.2862991346331,12.3370675853609,
12.4955056945959,12.6723064111662,12.7165364236069,12.7391860550326,12.7595074682699,
12.7915485636307,12.8314569706321,12.9227553177696,13.1407849364068,13.1947105076481,
13.2323818102843,13.2725564714223,13.3387627942662,13.4561514293095,13.6585370836615,
13.6928946928717,13.7115979590741,13.7327653686174,13.7693258959595,13.8979719074965,
14.108548001842,14.1631311423434,14.2009032660361,14.2408851037059,14.3060212698353,
14.3499419636041,14.4931891857176,14.5541961935573,14.6395264434425,14.6680975226309,
14.6879299393261,14.7122594485561,14.7662943566752,14.8510953181161,15.0865196191968,
15.1323492953002,15.1701221666306,15.2101020929185,15.2752284435875,15.3191395794418,
15.4623325335554,15.4979301920437,15.6054949295739,15.6355678551499,15.6555832804525,
15.6790737572924,15.7280260735791,15.7666545126145,15.9305281011558,16.0528048640956,
16.0997150011174,16.1377272874295,16.1773138358134,16.2402544764528,16.2820392513916,
16.4135664983527,16.4593764288642,16.56517460133,16.6000563850533,16.6188504597195,
16.6398990102012,16.6758594576763,16.7989868423694,17.01802376967,17.0717863210419,
17.1094327589452,17.1496568773599,17.2161392823434,17.30095135273,17.4123212286938,
17.5329590784149,17.5686136285624,17.5875438179729,17.6084343884826,17.6435855486997,
17.6676047878321,17.707172586896,17.8794535122686,17.9648471064293,18.0294516412634,
18.0693374199954,18.107599066136,18.1628843422288,18.2280923016221,18.3740617889961,
18.4108101264105,18.5134536822447,18.5433407488112,18.5633306086471,18.5869139438179,
18.6364094567011,18.6756807452355,18.8452506629214,18.9464257791202,19.0047585507113,
19.039664322051,19.0781107971785,19.13452402533,19.2884483576653,19.4776528089821,
19.5099864957067,19.5301567007405,19.552611715689,19.5957942459034,19.6279335709638,
19.7448230752108,19.8090063387367,19.9357316367902,19.9847596060258,20.0222559995674,
20.0641168322337,20.139841803154,20.2430719388833,20.4191025263796,20.467737281041,
20.491173005453,20.5112040083972,20.5413885849518,20.6574709219083,20.9027636167975,
20.9482081267957,20.9858985819515,21.0260337314445,21.0920226627224,21.1759153590753,
21.2884491584225,21.3908037678933,21.4378195218731,21.4609722025259,21.4810928752659,
21.5118887521058,21.6459575211512,21.8635283825155,21.9175082296144,21.9551873756986,
21.9953448636759,22.0614578718175,22.106345289338,22.2552610128412,22.2839220264468,
22.3903933354499,22.4202267376629,22.4402093140805,22.4638198895315,22.513475814836,
22.5529380950516,22.7242489607561,22.8152070971007,22.8775374852681,22.9170144222158,
22.9555507746083,23.0081366376917,23.2596158863234,23.3598101309815,23.3890076525042,
23.4041051946206,23.4185004054957,23.4390365433674,23.4688488899205,23.5247468046023,
23.706992854538,23.817547422462,23.8652438975169,23.9025270406034,23.9376075996493,
23.9804287313472,24.1651712231583,24.2505805506159,24.3322618369051,24.3577837539985,
24.3775616024521,24.3948373796966,24.414543948155),.UNSPECIFIED.) ;
#230=B_SPLINE_CURVE_WITH_KNOTS('',3,(#26240,#26241,#26242,#26243,#26244,
#26245,#26246,#26247,#26248,#26249,#26250,#26251,#26252,#26253,#26254,#26255,
#26256,#26257,#26258,#26259,#26260,#26261,#26262,#26263,#26264,#26265,#26266,
#26267,#26268,#26269,#26270,#26271,#26272,#26273,#26274,#26275,#26276,#26277,
#26278,#26279,#26280,#26281,#26282,#26283,#26284,#26285,#26286,#26287,#26288,
#26289,#26290,#26291,#26292,#26293,#26294,#26295,#26296,#26297,#26298,#26299,
#26300,#26301,#26302,#26303,#26304,#26305,#26306,#26307,#26308,#26309,#26310,
#26311,#26312,#26313,#26314,#26315,#26316,#26317,#26318,#26319,#26320,#26321,
#26322,#26323,#26324,#26325,#26326,#26327,#26328,#26329,#26330,#26331,#26332,
#26333,#26334,#26335,#26336,#26337,#26338,#26339,#26340,#26341,#26342,#26343,
#26344,#26345,#26346,#26347,#26348,#26349,#26350,#26351,#26352,#26353,#26354,
#26355,#26356,#26357,#26358,#26359,#26360,#26361,#26362,#26363,#26364,#26365,
#26366,#26367,#26368,#26369,#26370,#26371,#26372,#26373,#26374,#26375,#26376,
#26377,#26378,#26379,#26380,#26381,#26382,#26383,#26384,#26385,#26386,#26387,
#26388,#26389,#26390,#26391,#26392,#26393,#26394,#26395,#26396,#26397,#26398,
#26399,#26400,#26401,#26402,#26403,#26404,#26405,#26406,#26407,#26408,#26409,
#26410,#26411,#26412,#26413,#26414,#26415,#26416,#26417,#26418,#26419,#26420,
#26421,#26422,#26423,#26424,#26425,#26426,#26427,#26428,#26429,#26430,#26431,
#26432,#26433,#26434,#26435,#26436,#26437,#26438,#26439,#26440,#26441,#26442,
#26443,#26444,#26445,#26446,#26447,#26448,#26449,#26450,#26451,#26452,#26453,
#26454,#26455,#26456,#26457,#26458,#26459,#26460,#26461,#26462,#26463,#26464,
#26465,#26466,#26467,#26468,#26469,#26470,#26471,#26472,#26473,#26474,#26475,
#26476,#26477,#26478,#26479,#26480,#26481,#26482,#26483,#26484,#26485,#26486,
#26487,#26488,#26489,#26490,#26491,#26492,#26493,#26494,#26495,#26496,#26497,
#26498,#26499,#26500,#26501,#26502,#26503,#26504,#26505,#26506,#26507,#26508,
#26509,#26510,#26511,#26512,#26513,#26514,#26515,#26516,#26517,#26518,#26519,
#26520,#26521,#26522,#26523,#26524,#26525,#26526,#26527,#26528,#26529,#26530,
#26531,#26532,#26533,#26534,#26535,#26536,#26537,#26538,#26539,#26540,#26541,
#26542,#26543,#26544,#26545,#26546,#26547,#26548,#26549,#26550,#26551,#26552,
#26553,#26554,#26555,#26556,#26557,#26558,#26559,#26560,#26561,#26562,#26563,
#26564,#26565,#26566,#26567,#26568,#26569,#26570,#26571,#26572,#26573,#26574,
#26575,#26576,#26577,#26578,#26579,#26580,#26581,#26582,#26583,#26584,#26585,
#26586,#26587,#26588,#26589,#26590,#26591,#26592,#26593,#26594,#26595,#26596,
#26597,#26598,#26599,#26600,#26601,#26602,#26603,#26604,#26605,#26606,#26607,
#26608,#26609,#26610,#26611,#26612,#26613,#26614,#26615,#26616,#26617,#26618,
#26619,#26620,#26621,#26622,#26623,#26624,#26625,#26626,#26627,#26628,#26629,
#26630,#26631,#26632,#26633,#26634,#26635,#26636,#26637,#26638,#26639,#26640,
#26641,#26642,#26643,#26644,#26645,#26646,#26647,#26648,#26649,#26650,#26651,
#26652,#26653),.UNSPECIFIED.,.F.,.F.,(4,2,2,2,2,2,2,2,2,2,2,2,2,2,2,2,2,
2,2,2,2,2,2,2,2,2,2,2,2,2,2,2,2,2,2,2,2,2,2,2,2,2,2,2,2,2,2,2,2,2,2,2,2,
2,2,2,2,2,2,2,2,2,2,2,2,2,2,2,2,2,2,2,2,2,2,2,2,2,2,2,2,2,2,2,2,2,2,2,2,
2,2,2,2,2,2,2,2,2,2,2,2,2,2,2,2,2,2,2,2,2,2,2,2,2,2,2,2,2,2,2,2,2,2,2,2,
2,2,2,2,2,2,2,2,2,2,2,2,2,2,2,2,2,2,2,2,2,2,2,2,2,2,2,2,2,2,2,2,2,2,2,2,
2,2,2,2,2,2,2,2,2,2,2,2,2,2,2,2,2,2,2,2,2,2,2,2,2,2,2,2,2,2,2,2,2,2,2,2,
2,2,2,2,2,2,2,2,2,4),(8.33097403985845E-5,0.037924742923994,0.0723184899431885,
0.108380290041682,0.156714991299736,0.280103304901921,0.417705952640096,
0.420982404833398,0.425206806614123,0.430689472612384,0.454416149801046,
0.52869592538976,0.550033669237741,0.570400687153203,0.592952016895259,
0.636652157922749,0.813935734611086,0.920813221386165,0.97642504527676,
1.02383562632131,1.05434606689617,1.08921156671304,1.1453040955072,1.32097494979816,
1.43620600469129,1.4814893668784,1.48269234458807,1.48354804559005,1.4841557118606,
1.48458676224817,1.48655803406899,1.48830150331304,1.48984406973238,1.4912095796305,
1.49241909838386,1.49349118516626,1.49444215930972,1.49528635161025,1.49603633674722,
1.49670314481816,1.49729645157753,1.49782474777846,1.498295488897,1.49871522661799,
1.49908972385428,1.49942405501724,1.49972269326349,1.49998958623333,1.50022822184291,
1.50096734386075,1.50167606978337,1.52202439888614,1.53644654344062,1.55510281038928,
1.58918819506854,1.75838878910648,1.87988919515148,1.96362838272971,2.00682733499522,
2.04410319658965,2.09170609555358,2.20196652287321,2.21156263283878,2.38645095865376,
2.4262977436429,2.47627536272184,2.49994037767516,2.51990878827355,2.54963638925063,
2.64660470158102,2.70100888497496,2.83927934713902,2.88231565042999,2.94654849259009,
2.98636707769959,3.02423146550515,3.07048235755101,3.2350934482223,3.39369887739012,
3.44487325321878,3.46873876266709,3.48865960655727,3.51801413236063,3.61008539349427,
3.63884740392259,3.79832223152826,3.84490066303349,3.9126982415971,3.95315885195754,
3.9911182407047,4.04446668963585,4.26578912901904,4.38780317245995,4.42363917301473,
4.44466319658567,4.46347704422078,4.4984722576448,4.60580792659009,4.64956654788277,
4.78128857765866,4.84332530544383,4.89666764583297,4.93462618020398,4.97508891347651,
5.04289805390158,5.12067555119254,5.29431532066301,5.3340291652571,5.35811064851171,
5.39332715136781,5.41423032493115,5.43314881398654,5.46873769315376,5.60051985904766,
5.74410091778763,5.78807956191048,5.85327424280867,5.89326621779936,5.9310319155375,
5.98557643098345,6.19521783291394,6.32471181045928,6.36136178221986,6.38254678536875,
6.4012367865757,6.43551841279528,6.63823198419296,6.73995614476405,6.81497027405884,
6.85670810204116,6.89423362662374,6.94350260917837,7.07638563387608,7.13509845021154,
7.29555995338409,7.33130216692823,7.35230776716117,7.37113680573451,7.40621880436233,
7.51474489469923,7.67485389935436,7.72152941057088,7.78942274470131,7.82990053763285,
7.86785210557337,7.92114844542685,8.14276439872491,8.26463458314003,8.30045442391829,
8.32147526494929,8.3402917050924,8.37530177149167,8.48284009898151,8.52633597229078,
8.6580785394766,8.69990422582333,8.76288722725818,8.80248121932488,8.84048811415104,
8.89655058126913,9.00383877176518,9.17237633495223,9.21153292551815,9.26093187098583,
9.28449872510489,9.30449296336996,9.33441247871471,9.43774001426987,9.60883250797868,
9.65711220598767,9.72657348511125,9.76733241057447,9.80516566371884,9.85765296710003,
10.1191234071707,10.1857677606014,10.2319131742954,10.2549109195941,10.2748552302506,
10.3057903605918,10.3801341012346,10.6562804474052,10.710663549089,10.7487816986966,
10.7889203435939,10.8549283417174,10.9369559331857,11.1098303728143,11.1494620486647,
11.1735085210119,11.2086883037301,11.2295844051551,11.2485094706637,11.2841352330492,
11.4158790133166,11.5594414126286,11.6034168628817,11.6686083556248,11.708599831746,
11.7463659613795,11.7921652693021,11.9369634128778,11.967222552164,12.0932113976351,
12.1612847697981,12.1875932308972,12.2072906505637),.UNSPECIFIED.) ;
#231=B_SPLINE_CURVE_WITH_KNOTS('',3,(#26654,#26655,#26656,#26657,#26658,
#26659,#26660,#26661,#26662,#26663,#26664,#26665,#26666,#26667,#26668,#26669,
#26670,#26671,#26672,#26673,#26674,#26675,#26676,#26677,#26678,#26679,#26680,
#26681,#26682,#26683,#26684,#26685,#26686,#26687,#26688,#26689,#26690,#26691,
#26692,#26693,#26694,#26695,#26696,#26697,#26698,#26699,#26700,#26701,#26702,
#26703,#26704,#26705,#26706,#26707,#26708,#26709,#26710,#26711,#26712,#26713,
#26714,#26715,#26716,#26717,#26718,#26719,#26720,#26721,#26722,#26723,#26724,
#26725,#26726,#26727,#26728,#26729,#26730,#26731,#26732,#26733,#26734,#26735,
#26736,#26737,#26738,#26739,#26740,#26741,#26742,#26743,#26744,#26745,#26746,
#26747,#26748,#26749,#26750,#26751,#26752,#26753,#26754,#26755,#26756,#26757,
#26758,#26759,#26760,#26761,#26762,#26763,#26764,#26765,#26766,#26767,#26768,
#26769,#26770,#26771,#26772,#26773,#26774,#26775,#26776,#26777,#26778,#26779,
#26780,#26781,#26782,#26783,#26784,#26785,#26786,#26787,#26788,#26789,#26790,
#26791,#26792,#26793,#26794,#26795,#26796,#26797,#26798,#26799,#26800,#26801,
#26802,#26803,#26804,#26805,#26806,#26807,#26808,#26809,#26810,#26811,#26812,
#26813,#26814,#26815,#26816,#26817,#26818,#26819,#26820,#26821,#26822,#26823,
#26824,#26825,#26826,#26827,#26828,#26829,#26830,#26831,#26832,#26833,#26834,
#26835,#26836,#26837,#26838,#26839,#26840,#26841,#26842,#26843,#26844,#26845,
#26846,#26847,#26848,#26849,#26850,#26851,#26852,#26853,#26854,#26855,#26856,
#26857,#26858,#26859,#26860,#26861,#26862,#26863,#26864,#26865,#26866,#26867,
#26868,#26869,#26870,#26871,#26872,#26873,#26874,#26875,#26876,#26877,#26878,
#26879,#26880,#26881,#26882,#26883,#26884,#26885,#26886,#26887,#26888,#26889,
#26890,#26891,#26892,#26893,#26894,#26895,#26896,#26897,#26898,#26899,#26900,
#26901,#26902,#26903,#26904,#26905,#26906,#26907,#26908,#26909,#26910,#26911,
#26912,#26913,#26914,#26915,#26916,#26917,#26918,#26919,#26920,#26921,#26922,
#26923,#26924,#26925,#26926,#26927,#26928,#26929,#26930,#26931,#26932,#26933,
#26934,#26935,#26936,#26937,#26938,#26939,#26940,#26941,#26942,#26943,#26944,
#26945,#26946,#26947,#26948,#26949,#26950,#26951,#26952,#26953,#26954,#26955,
#26956,#26957,#26958,#26959,#26960,#26961,#26962,#26963,#26964,#26965,#26966,
#26967,#26968,#26969,#26970,#26971,#26972,#26973,#26974,#26975,#26976,#26977,
#26978,#26979,#26980,#26981,#26982,#26983,#26984,#26985,#26986,#26987,#26988,
#26989,#26990,#26991,#26992,#26993,#26994,#26995,#26996,#26997,#26998,#26999,
#27000,#27001,#27002,#27003),.UNSPECIFIED.,.F.,.F.,(4,2,2,2,2,2,2,2,2,2,
2,2,2,2,2,2,2,2,2,2,2,2,2,2,2,2,2,2,2,2,2,2,2,2,2,2,2,2,2,2,2,2,2,2,2,2,
2,2,2,2,2,2,2,2,2,2,2,2,2,2,2,2,2,2,2,2,2,2,2,2,2,2,2,2,2,2,2,2,2,2,2,2,
2,2,2,2,2,2,2,2,2,2,2,2,2,2,2,2,2,2,2,2,2,2,2,2,2,2,2,2,2,2,2,2,2,2,2,2,
2,2,2,2,2,2,2,2,2,2,2,2,2,2,2,2,2,2,2,2,2,2,2,2,2,2,2,2,2,2,2,2,2,2,2,2,
2,2,2,2,2,2,2,2,2,2,2,2,2,2,2,2,2,2,2,2,4),(8.71340497090936E-5,0.0431462393397145,
0.181910412010808,0.302714611116052,0.362072461948706,0.402214388992738,
0.437051944320088,0.474994746927191,0.528233256846255,0.75017799640711,
0.839953070808968,0.879482969901102,0.903609086629516,0.906634849381504,
0.909353999597516,0.912022049628397,0.915012628127877,0.934015672618608,
0.957952767559258,1.00558432627594,1.19433084553241,1.29030967439327,1.34272491498296,
1.38047054742223,1.39814501856307,1.43540911818344,1.48284794697211,1.58893166624209,
1.6654774828848,1.84253608693549,1.87753985098077,1.89840180679442,1.9173582960463,
1.95316163448382,2.08463940622617,2.22815983867,2.27212777975579,2.33731142170937,
2.37730117437565,2.41506759426198,2.46961832702716,2.67980497491144,2.80882575826391,
2.84542549106478,2.86660038316869,2.88529741711737,2.91962055116382,3.11215955905958,
3.21958255490145,3.2972448655286,3.3394372176361,3.37686277535162,3.42527526889042,
3.55407063353732,3.71894157041404,3.75768410043355,3.80673297543037,3.83023980332077,
3.85025024582739,3.88028896781445,3.99296148202705,4.1195876398833,4.20627884229904,
4.27375983542273,4.31416341062241,4.35214883047807,4.40567119924325,4.62603025926647,
4.7485091963076,4.78439713372531,4.80543129520775,4.82423668190984,4.85918389276147,
4.96586967618732,5.12744806913989,5.17434658198585,5.24245946577088,5.28297660984649,
5.32091045160027,5.37408840784635,5.59638784963516,5.71791751129297,5.75369900268019,
5.77471228137251,5.79353487511399,5.82858024712498,6.02815762939676,6.13083354153618,
6.20629762365978,6.24811322208642,6.28561983795941,6.33473477056653,6.46581316357391,
6.62742172267578,6.66578636547734,6.7145141712988,6.73796583700825,6.75799201983952,
6.78814321635514,6.89738942528884,7.06386478617193,7.1114877160055,7.18031033146228,
7.22095481272212,7.25883410989398,7.31164121235167,7.53638617710364,7.62500520997337,
7.66424512477582,7.69588958143311,7.71614459764995,7.73894444327569,7.78399561338899,
7.96463276113703,8.08637008875333,8.15208915214763,8.19217549882729,8.22989065090505,
8.27545264837787,8.51791709249546,8.59875626306783,8.65117096721831,8.67524022380368,
8.69511861441865,8.72411589629726,8.81249850409033,8.87080148252813,9.01319238265485,
9.05696315441157,9.12194654049746,9.16190046891161,9.19968719212972,9.2543668302558,
9.36551960605822,9.53340711272466,9.57249116503908,9.62182896216429,9.64538538638823,
9.66538245307504,9.69532268345045,9.79911773625038,9.99818357310984,10.0794701347149,
10.1222696918792,10.1595951438513,10.2070039239542,10.318236627621,10.3720808854931,
10.5110095745858,10.5606997473462,10.5982860122506,10.6196580071804,10.6382222380849,
10.6717632605593,10.877981421532,10.9785429751086,11.0137461608897,11.0696045947159,
11.1079593650195,11.1429607274567,11.2019041813594,11.3217285549136,11.4755952362156,
11.5276685515026,11.5665353112394,11.5881610618419,11.6065771347512,11.6392174588903,
11.7096407439587,11.9011260415366,12.00661533188,12.0529301905531,12.0865352830313,
12.1292147869275,12.207327736701),.UNSPECIFIED.) ;
#232=B_SPLINE_CURVE_WITH_KNOTS('',3,(#27008,#27009,#27010,#27011,#27012,
#27013,#27014,#27015,#27016,#27017,#27018,#27019,#27020,#27021,#27022,#27023,
#27024,#27025,#27026,#27027,#27028,#27029,#27030,#27031,#27032,#27033,#27034,
#27035,#27036,#27037,#27038,#27039,#27040,#27041,#27042,#27043,#27044,#27045,
#27046,#27047,#27048,#27049,#27050,#27051,#27052,#27053,#27054,#27055,#27056,
#27057,#27058,#27059,#27060,#27061,#27062,#27063,#27064,#27065,#27066,#27067,
#27068,#27069,#27070,#27071,#27072,#27073,#27074,#27075,#27076,#27077,#27078,
#27079,#27080,#27081,#27082,#27083,#27084,#27085,#27086,#27087,#27088,#27089,
#27090,#27091,#27092,#27093,#27094,#27095,#27096,#27097,#27098,#27099,#27100,
#27101,#27102,#27103,#27104,#27105,#27106,#27107,#27108,#27109,#27110,#27111,
#27112,#27113,#27114,#27115,#27116,#27117,#27118,#27119,#27120,#27121,#27122,
#27123,#27124,#27125,#27126,#27127,#27128,#27129,#27130,#27131,#27132,#27133,
#27134,#27135,#27136,#27137,#27138,#27139,#27140,#27141,#27142,#27143,#27144,
#27145,#27146,#27147,#27148,#27149,#27150,#27151,#27152,#27153,#27154,#27155,
#27156,#27157,#27158,#27159,#27160,#27161,#27162,#27163,#27164,#27165,#27166,
#27167,#27168,#27169,#27170,#27171,#27172,#27173,#27174,#27175,#27176,#27177,
#27178,#27179,#27180,#27181,#27182,#27183,#27184,#27185,#27186,#27187,#27188,
#27189,#27190,#27191,#27192,#27193,#27194,#27195,#27196,#27197,#27198,#27199,
#27200,#27201,#27202,#27203,#27204,#27205,#27206,#27207,#27208,#27209,#27210,
#27211,#27212,#27213,#27214,#27215,#27216,#27217,#27218,#27219,#27220,#27221,
#27222,#27223,#27224,#27225,#27226,#27227,#27228,#27229,#27230,#27231,#27232,
#27233,#27234,#27235,#27236,#27237,#27238,#27239,#27240,#27241,#27242,#27243,
#27244,#27245,#27246,#27247,#27248,#27249,#27250,#27251,#27252,#27253,#27254,
#27255,#27256,#27257,#27258,#27259,#27260,#27261,#27262,#27263,#27264,#27265,
#27266,#27267,#27268,#27269,#27270,#27271,#27272,#27273,#27274,#27275,#27276,
#27277,#27278,#27279,#27280,#27281,#27282,#27283,#27284,#27285,#27286,#27287,
#27288,#27289,#27290,#27291,#27292,#27293,#27294,#27295,#27296,#27297,#27298,
#27299,#27300,#27301,#27302,#27303,#27304,#27305,#27306,#27307,#27308,#27309,
#27310,#27311,#27312,#27313,#27314,#27315,#27316,#27317,#27318,#27319,#27320,
#27321,#27322,#27323,#27324,#27325,#27326,#27327,#27328,#27329,#27330,#27331,
#27332,#27333,#27334,#27335,#27336,#27337,#27338,#27339,#27340,#27341,#27342,
#27343,#27344,#27345,#27346,#27347,#27348,#27349,#27350,#27351,#27352,#27353,
#27354,#27355,#27356,#27357,#27358,#27359,#27360,#27361,#27362,#27363,#27364,
#27365,#27366,#27367),.UNSPECIFIED.,.F.,.F.,(4,2,2,2,2,2,2,2,2,2,2,2,2,
2,2,2,2,2,2,2,2,2,2,2,2,2,2,2,2,2,2,2,2,2,2,2,2,2,2,2,2,2,2,2,2,2,2,2,2,
2,2,2,2,2,2,2,2,2,2,2,2,2,2,2,2,2,2,2,2,2,2,2,2,2,2,2,2,2,2,2,2,2,2,2,2,
2,2,2,2,2,2,2,2,2,2,2,2,2,2,2,2,2,2,2,2,2,2,2,2,2,2,2,2,2,2,2,2,2,2,2,2,
2,2,2,2,2,2,2,2,2,2,2,2,2,2,2,2,2,2,2,2,2,2,2,2,2,2,2,2,2,2,2,2,2,2,2,2,
2,2,2,2,2,2,2,2,2,2,2,2,2,2,2,2,2,2,2,2,2,2,4),(12.2075745498797,12.3262656338311,
12.3619799132888,12.3809205220066,12.40179923522,12.4368901463382,12.4608521887084,
12.5002863457929,12.6713410935888,12.7637780156581,12.8255142107852,12.8648847006477,
12.9035025005532,12.9609363993553,13.0297220988503,13.1940375782104,13.3065495849622,
13.3365851096342,13.3565950453348,13.380103289859,13.4291607943439,13.467913616835,
13.6328736557849,13.7611697099932,13.8097291715017,13.8471708606928,13.8892810420357,
13.9664617258692,14.0728304943579,14.2488431086171,14.2938968453501,14.3166970330802,
14.3369516420502,14.3685944472407,14.5180413907856,14.7142330118598,14.7701250277482,
14.8081039637735,14.8477388963176,14.9109518103223,14.9529991818009,15.0859152238612,
15.1049128584893,15.1375766918174,15.2448629786792,15.274923039628,15.2949363417486,
15.3184323560644,15.3674187760068,15.5294021536682,15.6932977991888,15.7397747005401,
15.7776888813061,15.8174246025427,15.8811988808129,15.9610349670388,16.0916551067236,
16.1219689559579,16.2152561674053,16.2447424284249,16.2646794758532,16.2884722309518,
16.3392109897658,16.4972951791983,16.6632894705936,16.7094587940107,16.7473047942463,
16.7871528141012,16.8515516277932,16.8947501342632,17.033921858492,17.0793243534708,
17.1831088277998,17.2132110703781,17.2332301097813,17.2567050186198,17.3055693841273,
17.3440948555309,17.5070834158003,17.6337430137899,17.6794338420895,17.7171759490474,
17.757209060919,17.8226357099702,17.8668435123017,18.0117523825704,18.0534922684096,
18.1530689629708,18.1827909262348,18.2027582911727,18.226425495008,18.2764177677676,
18.316282522179,18.4913421604818,18.510414580487,18.6123123496834,18.659436163935,
18.6966788096134,18.7402145210129,18.8260699123708,18.8931276785117,19.0197420309939,
19.1219162354014,19.1517788528257,19.1717649053111,19.1953594498315,19.2449236235016,
19.2842771920227,19.4545999815899,19.5512977124525,19.6113494801581,19.6465255305553,
19.6847274228018,19.7396467257866,19.905489994391,20.0840613813005,20.1174047867361,
20.1359356258587,20.1573598092236,20.1952103209491,20.2453889442275,20.387243261883,
20.4033374639141,20.5369441268338,20.58941456322,20.6272444503295,20.6680076236605,
20.7374977202671,20.7858078662379,20.9571258856279,21.0601566271548,21.0900615246835,
21.1100532790556,21.1336263041982,21.183064223829,21.2222677242819,21.3912314081192,
21.4959662401701,21.5529624231092,21.5876612035588,21.6263293809405,21.6840624487702,
21.7533530491582,21.9205065892055,22.0288939434272,22.0589958410839,22.0790146702706,
22.1024893564889,22.1513533254384,22.1898785245784,22.3528664700775,22.4795196019357,
22.5252113609124,22.5629533806562,22.602985521628,22.6684083890041,22.7126126667274,
22.8575022074562,22.9004294695854,22.9987949696125,23.028539523143,23.0485097053532,
23.0679043092712,23.0923169440898,23.1326322607895,23.2255946490421,23.4407720122268,
23.4938299072249,23.5312696663016,23.5658907766766,23.6114338851711,23.792588410267,
23.9590681836148,23.9932717857122,24.0119479115602,24.0300697997594,24.0516791077489,
24.0844064158757,24.1495428583943,24.4143137504503),.UNSPECIFIED.) ;
#233=B_SPLINE_CURVE_WITH_KNOTS('',3,(#27368,#27369,#27370,#27371,#27372,
#27373,#27374,#27375,#27376,#27377,#27378,#27379,#27380,#27381,#27382,#27383,
#27384,#27385,#27386,#27387,#27388,#27389,#27390,#27391,#27392,#27393,#27394,
#27395,#27396,#27397,#27398,#27399,#27400,#27401,#27402,#27403,#27404,#27405,
#27406,#27407,#27408,#27409,#27410,#27411,#27412,#27413,#27414,#27415,#27416,
#27417,#27418,#27419,#27420,#27421,#27422,#27423,#27424,#27425,#27426,#27427,
#27428,#27429,#27430,#27431,#27432,#27433,#27434,#27435,#27436,#27437,#27438,
#27439,#27440,#27441,#27442,#27443,#27444,#27445,#27446,#27447,#27448,#27449,
#27450,#27451,#27452,#27453,#27454,#27455,#27456,#27457,#27458,#27459,#27460,
#27461,#27462,#27463,#27464,#27465,#27466,#27467,#27468,#27469,#27470,#27471,
#27472,#27473,#27474,#27475,#27476,#27477,#27478,#27479,#27480,#27481,#27482,
#27483,#27484,#27485,#27486,#27487,#27488,#27489,#27490,#27491,#27492,#27493,
#27494,#27495,#27496,#27497,#27498,#27499,#27500,#27501,#27502,#27503,#27504,
#27505,#27506,#27507,#27508,#27509,#27510,#27511,#27512,#27513,#27514,#27515,
#27516,#27517,#27518,#27519,#27520,#27521,#27522,#27523,#27524,#27525,#27526,
#27527,#27528,#27529,#27530,#27531,#27532,#27533,#27534,#27535,#27536,#27537,
#27538,#27539,#27540,#27541,#27542,#27543,#27544,#27545,#27546,#27547,#27548,
#27549,#27550,#27551,#27552,#27553,#27554,#27555,#27556,#27557,#27558,#27559,
#27560,#27561,#27562,#27563,#27564,#27565,#27566,#27567,#27568,#27569,#27570,
#27571,#27572,#27573,#27574,#27575,#27576,#27577,#27578,#27579,#27580,#27581,
#27582,#27583,#27584,#27585,#27586,#27587,#27588,#27589,#27590,#27591,#27592,
#27593,#27594,#27595,#27596,#27597,#27598,#27599,#27600,#27601,#27602,#27603,
#27604,#27605,#27606,#27607,#27608,#27609,#27610,#27611,#27612,#27613,#27614,
#27615,#27616,#27617,#27618,#27619,#27620,#27621,#27622,#27623,#27624,#27625,
#27626,#27627,#27628,#27629,#27630,#27631,#27632,#27633,#27634,#27635,#27636,
#27637,#27638,#27639,#27640,#27641,#27642,#27643,#27644,#27645,#27646,#27647,
#27648,#27649,#27650,#27651,#27652,#27653,#27654,#27655,#27656,#27657,#27658,
#27659,#27660,#27661,#27662,#27663,#27664,#27665,#27666,#27667,#27668,#27669,
#27670,#27671,#27672,#27673,#27674,#27675,#27676,#27677,#27678,#27679,#27680,
#27681,#27682,#27683,#27684,#27685,#27686,#27687,#27688,#27689,#27690,#27691,
#27692,#27693,#27694,#27695,#27696,#27697,#27698,#27699,#27700,#27701,#27702,
#27703,#27704,#27705,#27706,#27707,#27708,#27709,#27710,#27711,#27712,#27713,
#27714,#27715,#27716,#27717,#27718,#27719,#27720,#27721,#27722,#27723,#27724,
#27725,#27726,#27727,#27728,#27729,#27730,#27731,#27732,#27733),
 .UNSPECIFIED.,.F.,.F.,(4,2,2,2,2,2,2,2,2,2,2,2,2,2,2,2,2,2,2,2,2,2,2,2,
2,2,2,2,2,2,2,2,2,2,2,2,2,2,2,2,2,2,2,2,2,2,2,2,2,2,2,2,2,2,2,2,2,2,2,2,
2,2,2,2,2,2,2,2,2,2,2,2,2,2,2,2,2,2,2,2,2,2,2,2,2,2,2,2,2,2,2,2,2,2,2,2,
2,2,2,2,2,2,2,2,2,2,2,2,2,2,2,2,2,2,2,2,2,2,2,2,2,2,2,2,2,2,2,2,2,2,2,2,
2,2,2,2,2,2,2,2,2,2,2,2,2,2,2,2,2,2,2,2,2,2,2,2,2,2,2,2,2,2,2,2,2,2,2,2,
2,2,2,2,2,2,2,2,2,2,2,2,2,2,4),(12.207327736701,12.3178091535815,12.5100743794467,
12.5418117813965,12.5618825409038,12.5845557468051,12.6289149326578,12.6918105994009,
12.9520503301033,13.0079775049734,13.0459622936337,13.085588895521,13.1487545277891,
13.1907561957183,13.3234292736677,13.3484659519424,13.37024182797,13.4828099779603,
13.5128466304612,13.5328567817399,13.5563646121386,13.6054193728659,13.6441688869385,
13.8090993676656,13.9375679680787,13.9860769341604,14.0235131123492,14.0656514968094,
14.1429969316421,14.2497252201926,14.4266607863629,14.4707378225575,14.4933589249592,
14.5136928400826,14.5458095020569,14.6954878462602,14.8901329126284,14.9461938982554,
14.984200324635,15.0237942440784,15.0867781451114,15.1286048024763,15.2603535862527,
15.3037427392678,15.4113596570535,15.4463751684567,15.4651924629181,15.4862119103093,
15.5220252580706,15.6438389155786,15.8655708085405,15.9188467216112,15.9567949966148,
15.9972790931677,16.0652088532836,16.111921452303,16.2722757918865,16.3804874319662,
16.415546306964,16.4343711876278,16.4553814189954,16.4911478746352,16.6068788644865,
16.8368836909677,16.8892617473599,16.9270789901272,16.9678770350268,17.0375595302559,
17.0860681619753,17.258817442158,17.3025004445771,17.3677833610841,17.3939329753429,
17.4136347980508,17.4394477574176,17.5036765935167,17.6169356864953,17.6615704496211,
17.8084344473779,17.8547379396401,17.8926137546589,17.9324125853187,17.9965368067468,
18.039467367389,18.1771560689096,18.3176876765218,18.3533854613398,18.3723231472201,
18.3932050273094,18.4283122853703,18.6052107732637,18.682904262808,18.7877998404064,
18.8352429535751,18.8725072571318,18.9158161638107,19.0002408803156,19.1234292203653,
19.289575381956,19.3238163707776,19.3424992520199,19.3636936472215,19.40039159649,
19.4484575823164,19.5781284894148,19.6060531490213,19.7475213408503,19.7935510376247,
19.831366781637,19.8712681793573,19.9359616162522,19.9794480723337,20.1202300879615,
20.1576768412232,20.2668746076173,20.2970218335619,20.3170473471543,20.3405006672809,
20.389238701331,20.4276155161417,20.5893276240276,20.720276259877,20.7693910090018,
20.8068973726441,20.8487125732679,20.9241756589133,21.0268497502248,21.2264229268091,
21.2614680033038,21.2802904532003,21.3013035745517,21.3370848289635,21.4586135417284,
21.6809163642699,21.7340937384932,21.7720272702546,21.8125441664727,21.8806569094721,
21.9275554030667,22.0891358617711,22.1958129621524,22.230759234421,22.2495643634196,
22.2705985026272,22.3064868979792,22.4289711190001,22.6493206586609,22.702844768519,
22.7408302258397,22.7812327937582,22.7825642676513,22.7839416949544,22.7853787528071,
22.7868907252314,22.7884950545104,22.790212008366,22.7920655063888,22.7940841609254,
22.7963026032125,22.8443807907027,22.9266898391829,23.0405125053488,23.0594391175267,
23.165137508115,23.2000113966874,23.2188038453493,23.2330053580524,23.2596792309956,
23.3346895057409,23.4944949105014,23.6274693338759,23.6767372189328,23.714262211541,
23.7520563198239,23.7760108174523,23.8855779476864,24.1118905529006,24.1596988100813,
24.1832773027337,24.2025205472974,24.2228626976231,24.2521404093967,24.4143563453461),
 .UNSPECIFIED.) ;
#234=B_SPLINE_CURVE_WITH_KNOTS('',3,(#27738,#27739,#27740,#27741,#27742,
#27743,#27744,#27745,#27746,#27747,#27748,#27749,#27750,#27751,#27752,#27753,
#27754,#27755,#27756,#27757,#27758,#27759,#27760,#27761,#27762,#27763,#27764,
#27765,#27766,#27767,#27768,#27769,#27770,#27771,#27772,#27773,#27774,#27775,
#27776,#27777,#27778,#27779,#27780,#27781,#27782,#27783,#27784,#27785,#27786,
#27787,#27788,#27789,#27790,#27791,#27792,#27793,#27794,#27795,#27796,#27797,
#27798,#27799,#27800,#27801,#27802,#27803,#27804,#27805,#27806,#27807,#27808,
#27809,#27810,#27811,#27812,#27813,#27814,#27815,#27816,#27817,#27818,#27819,
#27820,#27821,#27822,#27823,#27824,#27825,#27826,#27827,#27828,#27829,#27830,
#27831,#27832,#27833,#27834,#27835,#27836,#27837,#27838,#27839,#27840,#27841,
#27842,#27843,#27844,#27845,#27846,#27847,#27848,#27849,#27850,#27851,#27852,
#27853,#27854,#27855,#27856,#27857,#27858,#27859,#27860,#27861,#27862,#27863,
#27864,#27865,#27866,#27867,#27868,#27869,#27870,#27871,#27872,#27873,#27874,
#27875,#27876,#27877,#27878,#27879,#27880,#27881,#27882,#27883,#27884,#27885,
#27886,#27887,#27888,#27889,#27890,#27891,#27892,#27893,#27894,#27895,#27896,
#27897,#27898,#27899,#27900,#27901,#27902,#27903,#27904,#27905,#27906,#27907,
#27908,#27909,#27910,#27911,#27912,#27913,#27914,#27915,#27916,#27917,#27918,
#27919,#27920,#27921,#27922,#27923,#27924,#27925,#27926,#27927,#27928,#27929,
#27930,#27931,#27932,#27933,#27934,#27935,#27936,#27937,#27938,#27939,#27940,
#27941,#27942,#27943,#27944,#27945,#27946,#27947,#27948,#27949,#27950,#27951,
#27952,#27953,#27954,#27955,#27956,#27957,#27958,#27959,#27960,#27961,#27962,
#27963,#27964,#27965,#27966,#27967,#27968,#27969,#27970,#27971,#27972,#27973,
#27974,#27975,#27976,#27977,#27978,#27979,#27980,#27981,#27982,#27983,#27984,
#27985,#27986,#27987,#27988,#27989,#27990,#27991,#27992,#27993,#27994,#27995,
#27996,#27997,#27998,#27999,#28000,#28001,#28002,#28003,#28004,#28005,#28006,
#28007,#28008,#28009,#28010,#28011,#28012,#28013,#28014,#28015,#28016,#28017,
#28018,#28019,#28020,#28021,#28022,#28023,#28024,#28025,#28026,#28027,#28028,
#28029,#28030,#28031,#28032,#28033,#28034,#28035,#28036,#28037,#28038,#28039,
#28040,#28041,#28042,#28043,#28044,#28045,#28046,#28047,#28048,#28049,#28050,
#28051,#28052,#28053,#28054,#28055,#28056,#28057,#28058,#28059,#28060,#28061,
#28062,#28063,#28064,#28065,#28066,#28067,#28068,#28069,#28070,#28071,#28072,
#28073,#28074,#28075,#28076,#28077),.UNSPECIFIED.,.F.,.F.,(4,2,2,2,2,2,
2,2,2,2,2,2,2,2,2,2,2,2,2,2,2,2,2,2,2,2,2,2,2,2,2,2,2,2,2,2,2,2,2,2,2,2,
2,2,2,2,2,2,2,2,2,2,2,2,2,2,2,2,2,2,2,2,2,2,2,2,2,2,2,2,2,2,2,2,2,2,2,2,
2,2,2,2,2,2,2,2,2,2,2,2,2,2,2,2,2,2,2,2,2,2,2,2,2,2,2,2,2,2,2,2,2,2,2,2,
2,2,2,2,2,2,2,2,2,2,2,2,2,2,2,2,2,2,2,2,2,2,2,2,2,2,2,2,2,2,2,2,2,2,2,2,
2,2,2,2,2,2,2,2,2,2,2,2,2,2,2,2,2,2,2,4),(0.000300129334749554,0.170465605201082,
0.214637287488896,0.249980507413532,0.283690260726543,0.327926523715331,
0.418325202517395,0.625914115324944,0.710601461913576,0.734601505583537,
0.75288144025282,0.771791205841507,0.807331235707942,0.922372580218292,
1.07735723027461,1.14439175336905,1.19718502406728,1.23119397558456,1.26885562888494,
1.32272110109602,1.5663565353341,1.64165365566064,1.66583171542758,1.70114944642875,
1.72207220203394,1.74097283993035,1.77646121213289,1.89073012681927,2.06011175954378,
2.10136034790645,2.16374171685343,2.20322772394761,2.24130902597476,2.29782783579101,
2.44545568475422,2.58202574778774,2.63131319296772,2.66868035420441,2.69000854808319,
2.70860064223467,2.74230781710601,2.94717425486887,3.04830685954465,3.08364420536323,
3.13965165022443,3.17803074202575,3.21300556545503,3.27178104262712,3.42241596180073,
3.55322533087405,3.60149741138596,3.63830885096753,3.65952591970968,3.67819284370369,
3.71234052207645,3.91564545314322,4.03249736151204,4.09870746168942,4.1388821666574,
4.17655212825755,4.23047331559905,4.44721933963644,4.57194332415861,4.60807974270388,
4.62916280319412,4.65063485526444,4.68872480648082,4.92902139295812,5.00763059519555,
5.07072319130099,5.11033650613542,5.14832968813457,5.20430984495815,5.40572489476059,
5.54326374723279,5.57826773895211,5.59912968855381,5.61808604561732,5.65388889218677,
5.78536681143262,5.92888681078269,5.9728546110497,6.03803803799565,6.07802765170954,
6.11579393536218,6.17034446111403,6.37968776190185,6.50941613108775,6.54609055206226,
6.56728025879866,6.58596647804041,6.62022697135088,6.82302906606593,6.92472319746984,
6.99972276014687,7.04145772361579,7.07898338791301,7.12825652116853,7.2634165000218,
7.42149409749689,7.45943896159524,7.50780792108265,7.53119743466352,7.55124167182216,
7.58152106393081,7.69155709053772,7.8572732465834,7.90478559705969,7.97350007778487,
8.01412496788776,8.05201203658566,8.1048739416702,8.22460674778463,8.25994604508097,
8.39706702613442,8.44644900246894,8.48386757826114,8.50520594649681,8.52379124003589,
8.55745857534416,8.76303535135153,8.87912816591802,8.94501396227604,8.98513011922795,
9.02282939732705,9.06831763163212,9.20844413813766,9.23043327241713,9.3665852366911,
9.41580029743774,9.45312790975155,9.47444807492814,9.4930450945367,9.52678216465161,
9.70430907774216,9.86525919965067,9.92256964739479,9.96116636547169,10.0005632205022,
10.0624478544322,10.1545107458112,10.3256265502277,10.3650670819695,10.3890318007783,
10.4241255136066,10.4450047085898,10.4639446937056,10.4996558087116,10.618226283471,
10.7705657941295,10.8370779122678,10.8931514127444,10.9315410977742,10.9712236694182,
11.0347024647697,11.122825319912,11.2946224940449,11.3341372028636,11.3838368902229,
11.4074546806538,11.4274349945917,11.457253245552,11.5634988816045,11.7326325700872,
11.7806363762068,11.8498296065167,11.890540121213,11.9283917584273,11.9810105037408,
12.2075745498797),.UNSPECIFIED.) ;
#235=B_SPLINE_CURVE_WITH_KNOTS('',3,(#28078,#28079,#28080,#28081,#28082,
#28083,#28084,#28085,#28086,#28087,#28088,#28089,#28090,#28091,#28092,#28093,
#28094,#28095,#28096,#28097,#28098,#28099,#28100,#28101,#28102,#28103,#28104,
#28105,#28106,#28107,#28108,#28109,#28110,#28111,#28112,#28113,#28114,#28115,
#28116,#28117,#28118,#28119,#28120,#28121,#28122,#28123,#28124,#28125,#28126,
#28127,#28128,#28129,#28130,#28131,#28132,#28133,#28134,#28135,#28136,#28137,
#28138,#28139,#28140,#28141,#28142,#28143,#28144,#28145,#28146,#28147,#28148,
#28149,#28150,#28151,#28152,#28153,#28154,#28155,#28156,#28157,#28158,#28159,
#28160,#28161,#28162,#28163,#28164,#28165,#28166,#28167,#28168,#28169,#28170,
#28171,#28172,#28173,#28174,#28175,#28176,#28177,#28178,#28179,#28180,#28181,
#28182,#28183,#28184,#28185,#28186,#28187,#28188,#28189,#28190,#28191,#28192,
#28193,#28194,#28195,#28196,#28197,#28198,#28199,#28200,#28201,#28202,#28203,
#28204,#28205,#28206,#28207,#28208,#28209,#28210,#28211,#28212,#28213,#28214,
#28215,#28216,#28217,#28218,#28219,#28220,#28221,#28222,#28223,#28224,#28225,
#28226,#28227,#28228,#28229,#28230,#28231,#28232,#28233,#28234,#28235,#28236,
#28237,#28238,#28239,#28240,#28241,#28242,#28243,#28244,#28245,#28246,#28247,
#28248,#28249,#28250,#28251,#28252,#28253,#28254,#28255,#28256,#28257,#28258,
#28259,#28260,#28261,#28262,#28263,#28264,#28265,#28266,#28267,#28268,#28269,
#28270,#28271,#28272,#28273,#28274,#28275,#28276,#28277,#28278,#28279,#28280,
#28281,#28282,#28283,#28284,#28285,#28286,#28287,#28288,#28289,#28290,#28291,
#28292,#28293,#28294,#28295,#28296,#28297,#28298,#28299,#28300,#28301,#28302,
#28303,#28304,#28305,#28306,#28307,#28308,#28309,#28310,#28311,#28312,#28313,
#28314,#28315,#28316,#28317,#28318,#28319,#28320,#28321,#28322,#28323,#28324,
#28325,#28326,#28327,#28328,#28329,#28330,#28331,#28332,#28333,#28334,#28335,
#28336,#28337,#28338,#28339,#28340,#28341,#28342,#28343,#28344,#28345,#28346,
#28347,#28348,#28349,#28350,#28351,#28352,#28353,#28354,#28355,#28356,#28357,
#28358,#28359,#28360,#28361,#28362,#28363,#28364,#28365,#28366,#28367,#28368,
#28369,#28370,#28371,#28372,#28373,#28374,#28375,#28376,#28377,#28378,#28379,
#28380,#28381,#28382,#28383,#28384,#28385,#28386,#28387,#28388,#28389,#28390,
#28391,#28392,#28393,#28394,#28395,#28396,#28397,#28398,#28399,#28400,#28401,
#28402,#28403,#28404,#28405,#28406,#28407,#28408,#28409,#28410,#28411,#28412,
#28413,#28414,#28415,#28416,#28417,#28418,#28419,#28420,#28421,#28422,#28423,
#28424,#28425,#28426,#28427,#28428,#28429,#28430,#28431,#28432,#28433,#28434,
#28435,#28436,#28437,#28438,#28439),.UNSPECIFIED.,.F.,.F.,(4,2,2,2,2,2,
2,2,2,2,2,2,2,2,2,2,2,2,2,2,2,2,2,2,2,2,2,2,2,2,2,2,2,2,2,2,2,2,2,2,2,2,
2,2,2,2,2,2,2,2,2,2,2,2,2,2,2,2,2,2,2,2,2,2,2,2,2,2,2,2,2,2,2,2,2,2,2,2,
2,2,2,2,2,2,2,2,2,2,2,2,2,2,2,2,2,2,2,2,2,2,2,2,2,2,2,2,2,2,2,2,2,2,2,2,
2,2,2,2,2,2,2,2,2,2,2,2,2,2,2,2,2,2,2,2,2,2,2,2,2,2,2,2,2,2,2,2,2,2,2,2,
2,2,2,2,2,2,2,2,2,2,2,2,2,2,2,2,2,2,2,2,2,2,2,2,2,2,2,2,2,2,4),(4.23208308298446E-5,
0.125359044082082,0.188807359086395,0.226619635936491,0.261894632939479,
0.301516669984305,0.364656721856589,0.61174494231358,0.701792257972909,
0.726120374666445,0.7443308594801,0.763137486151525,0.798091618841933,0.904870341165865,
1.06637480891283,1.1346478809672,1.18801517880547,1.22249963161744,1.26051544834448,
1.31423745572013,1.55868437822124,1.63369005301111,1.68361916086748,1.7072760983078,
1.72724677703,1.75699053571378,1.85474710861021,1.87800506345815,1.92125906900328,
2.08751035155991,2.1528800725541,2.19290369839278,2.23065248806155,2.27637097063721,
2.41948400187062,2.56957920845577,2.62107711579589,2.65963718064942,2.68120248947268,
2.69965185280298,2.73249751267298,2.91344854070258,3.07305960022707,3.13020302263844,
3.16877198440148,3.20820629324407,3.27029768947247,3.36184935782567,3.53305642683296,
3.57250728691684,3.59647654667502,3.63157520846381,3.65245561014531,3.67139515469671,
3.70710253008245,3.84781568567189,3.98538126159972,4.02828973948332,4.09239148125162,
4.13218662328738,4.17006543016343,4.21638090087466,4.36464709054382,4.40849224309567,
4.52130023446569,4.58538569184048,4.6111797275287,4.6308823001479,4.65705252053155,
4.72247211276768,4.79779163748163,4.91060303536709,4.99420300781514,5.0600341082905,
5.10014084484866,5.13784586064497,5.18335914962703,5.42701725234172,5.50720117219997,
5.55934285500671,5.58336772698827,5.60325506408137,5.63232890046331,5.72125832396878,
5.84828674542808,5.94848543588946,5.98360317020306,6.03936667202018,6.07770613764213,
6.1174675128258,6.18138062525257,6.26844950686896,6.44043502187367,6.47997068112303,
6.52968833490125,6.55330954558013,6.57328960624022,6.60310304900225,6.70924258213049,
6.76838856406456,6.89762208222835,6.93896693259228,7.00144919678329,7.04095371300572,
7.07902292296772,7.13546531115045,7.24171428897968,7.30926201508716,7.42686290205341,
7.45911835407648,7.47987746782347,7.51151874063607,7.53177340356168,7.55457489041168,
7.59963416754486,7.77566893744542,7.92260413226695,7.97807940928382,8.01637185866739,
8.05620748142914,8.12053330743185,8.20659960122973,8.37876032725485,8.41831494587016,
8.46804846269441,8.49167234136789,8.51165166613299,8.54145979676041,8.64720944667967,
8.66543450543302,8.6900939667173,8.83004828358448,8.87338770827212,8.93793126485065,
8.97780620088743,9.01563831209363,9.06174053721773,9.17318043634505,9.34743776759368,
9.38721780003057,9.43713997440076,9.46079587793659,9.48076705789845,9.5105134961185,
9.60872403283247,9.63158564408396,9.67396915947893,9.80444882423844,9.86619223250518,
9.91935329872147,9.95728516743988,9.99780902479776,10.0659565583404,10.1195530796605,
10.3124948241768,10.3954032270064,10.4233305459428,10.4431037317468,10.4678643137253,
10.5246840232667,10.7851174757713,10.8650978148507,10.907680974549,10.9450386874909,
10.9927901013387,11.1112053664767,11.2858111189896,11.3256282138407,11.3755813085676,
11.3992424135982,11.419212220799,11.4489485073966,11.5462389152137,11.5902958510401,
11.7351763810448,11.7793800795842,11.8448032398245,11.8848367095948,11.9225806732416,
11.9682756484446,12.2073821909332),.UNSPECIFIED.) ;
#236=B_SPLINE_CURVE_WITH_KNOTS('',3,(#28444,#28445,#28446,#28447,#28448,
#28449,#28450,#28451,#28452,#28453,#28454,#28455,#28456,#28457,#28458,#28459,
#28460,#28461,#28462,#28463,#28464,#28465,#28466,#28467,#28468,#28469,#28470,
#28471,#28472,#28473,#28474,#28475,#28476,#28477,#28478,#28479,#28480,#28481,
#28482,#28483,#28484,#28485,#28486,#28487,#28488,#28489,#28490,#28491,#28492,
#28493,#28494,#28495,#28496,#28497,#28498,#28499,#28500,#28501,#28502,#28503,
#28504,#28505,#28506,#28507,#28508,#28509,#28510,#28511,#28512,#28513,#28514,
#28515,#28516,#28517,#28518,#28519,#28520,#28521,#28522,#28523,#28524,#28525,
#28526,#28527,#28528,#28529,#28530,#28531,#28532,#28533,#28534,#28535,#28536,
#28537,#28538,#28539,#28540,#28541,#28542,#28543,#28544,#28545,#28546,#28547,
#28548,#28549,#28550,#28551,#28552,#28553,#28554,#28555,#28556,#28557,#28558,
#28559,#28560,#28561,#28562,#28563,#28564,#28565,#28566,#28567,#28568,#28569,
#28570,#28571,#28572,#28573,#28574,#28575,#28576,#28577,#28578,#28579,#28580,
#28581,#28582,#28583,#28584,#28585,#28586,#28587,#28588,#28589,#28590,#28591,
#28592,#28593,#28594,#28595,#28596,#28597,#28598,#28599,#28600,#28601,#28602,
#28603,#28604,#28605,#28606,#28607,#28608,#28609,#28610,#28611,#28612,#28613,
#28614,#28615,#28616,#28617,#28618,#28619,#28620,#28621,#28622,#28623,#28624,
#28625,#28626,#28627,#28628,#28629,#28630,#28631,#28632,#28633,#28634,#28635,
#28636,#28637,#28638,#28639,#28640,#28641,#28642,#28643,#28644,#28645,#28646,
#28647,#28648,#28649,#28650,#28651,#28652,#28653,#28654,#28655,#28656,#28657,
#28658,#28659,#28660,#28661,#28662,#28663,#28664,#28665,#28666,#28667,#28668,
#28669,#28670,#28671,#28672,#28673,#28674,#28675,#28676,#28677,#28678,#28679,
#28680,#28681,#28682,#28683,#28684,#28685,#28686,#28687,#28688,#28689,#28690,
#28691,#28692,#28693,#28694,#28695,#28696,#28697,#28698,#28699,#28700,#28701,
#28702,#28703,#28704,#28705,#28706,#28707,#28708,#28709,#28710,#28711,#28712,
#28713,#28714,#28715,#28716,#28717,#28718,#28719,#28720,#28721,#28722,#28723,
#28724,#28725,#28726,#28727,#28728,#28729,#28730,#28731,#28732,#28733,#28734,
#28735,#28736,#28737,#28738,#28739,#28740,#28741,#28742,#28743,#28744,#28745,
#28746,#28747),.UNSPECIFIED.,.F.,.F.,(4,3,3,3,3,3,3,3,3,3,3,3,3,3,3,3,3,
3,3,3,3,3,3,3,3,3,3,3,3,3,3,3,3,3,3,3,3,3,3,3,3,3,3,3,3,3,3,3,3,3,3,3,3,
3,3,3,3,3,3,3,3,3,3,3,3,3,3,3,3,3,3,3,3,3,3,3,3,3,3,3,3,3,3,3,3,3,3,3,3,
3,3,3,3,3,3,3,3,3,3,3,3,4),(-48.0752879938944,-48.0111765274951,-47.9470448098061,
-47.8905217899249,-47.8281643396776,-47.7658541252663,-47.7035505977148,
-47.6412508565077,-47.5788536893674,-47.5165475572819,-47.4541048726142,
-47.3916621879465,-47.3293047376992,-47.266994523288,-47.2046909957368,
-47.1423912545299,-47.0799940873895,-47.0176879553043,-46.9552452706362,
-46.8928025859681,-46.8304451357208,-46.7681349213095,-46.7058313937583,
-46.643531652551,-46.5811344854107,-46.5188283533254,-46.4563856686576,
-46.3939429839897,-46.3315855337424,-46.2692753193313,-46.2069717917801,
-46.144672050573,-46.0822748834326,-46.0199687513474,-45.9575260666794,
-45.8950833820114,-45.8327259317641,-45.7704157173528,-45.7081121898015,
-45.6458124485943,-45.583415281454,-45.5211091493687,-45.4586664647008,
-45.396223780033,-45.3338663297857,-45.2715561153745,-45.2092525878232,
-45.1469528466161,-45.0845556794757,-45.0222495473905,-44.9598068627226,
-44.8973641780546,-44.8350067278073,-44.7726965133961,-44.7103929858449,
-44.6480932446378,-44.5856960774974,-44.5233899454122,-44.4609472607442,
-44.3985045760762,-44.3361471258289,-44.2738369114177,-44.2115333838663,
-44.1492336426592,-44.0868364755189,-44.0245303434336,-43.9620876587657,
-43.8996449740978,-43.8372875238505,-43.7749773094393,-43.712673781888,
-43.6503740406809,-43.5879768735405,-43.5256707414552,-43.4632280567873,
-43.4007853721194,-43.3384279218721,-43.2761177074608,-43.2138141799096,
-43.1515144387025,-43.0891172715621,-43.0268111394768,-42.9643684548089,
-42.901925770141,-42.8395683198937,-42.7772581054827,-42.7149545779317,
-42.6526548367248,-42.5902576695843,-42.527951537499,-42.4655088528309,
-42.4030661681627,-42.3407087179154,-42.2783985035042,-42.2160949759529,
-42.153795234746,-42.0913980676056,-42.0290919355203,-41.9666492508523,
-41.9042065661843,-41.8383523791251,-41.7921027231872),.UNSPECIFIED.) ;
#237=B_SPLINE_CURVE_WITH_KNOTS('',3,(#28748,#28749,#28750,#28751,#28752,
#28753,#28754,#28755,#28756,#28757,#28758,#28759,#28760,#28761,#28762,#28763,
#28764,#28765,#28766,#28767,#28768,#28769,#28770,#28771,#28772,#28773,#28774,
#28775,#28776,#28777,#28778,#28779,#28780,#28781,#28782,#28783,#28784,#28785,
#28786,#28787,#28788,#28789,#28790,#28791,#28792,#28793,#28794,#28795,#28796,
#28797,#28798,#28799,#28800,#28801,#28802,#28803,#28804,#28805,#28806,#28807,
#28808,#28809,#28810,#28811,#28812,#28813,#28814,#28815,#28816,#28817,#28818,
#28819,#28820,#28821,#28822,#28823,#28824,#28825,#28826,#28827,#28828,#28829,
#28830,#28831,#28832,#28833,#28834,#28835,#28836,#28837,#28838,#28839,#28840,
#28841,#28842,#28843,#28844,#28845,#28846,#28847,#28848,#28849,#28850,#28851,
#28852,#28853,#28854,#28855,#28856,#28857,#28858,#28859,#28860,#28861,#28862,
#28863,#28864,#28865,#28866,#28867,#28868,#28869,#28870,#28871,#28872,#28873,
#28874,#28875,#28876,#28877,#28878,#28879,#28880,#28881,#28882,#28883,#28884,
#28885,#28886,#28887,#28888,#28889,#28890,#28891,#28892,#28893,#28894,#28895,
#28896,#28897,#28898,#28899,#28900,#28901,#28902,#28903,#28904,#28905,#28906,
#28907,#28908,#28909,#28910,#28911,#28912,#28913,#28914,#28915,#28916,#28917,
#28918,#28919,#28920,#28921,#28922,#28923,#28924,#28925,#28926,#28927,#28928,
#28929,#28930,#28931,#28932,#28933,#28934,#28935,#28936,#28937,#28938,#28939,
#28940,#28941,#28942,#28943,#28944,#28945,#28946,#28947,#28948,#28949,#28950,
#28951,#28952,#28953,#28954,#28955,#28956,#28957,#28958,#28959,#28960,#28961,
#28962,#28963,#28964,#28965,#28966,#28967,#28968,#28969,#28970,#28971,#28972,
#28973,#28974,#28975,#28976,#28977,#28978,#28979,#28980,#28981,#28982,#28983,
#28984,#28985,#28986,#28987,#28988,#28989,#28990,#28991,#28992,#28993,#28994,
#28995,#28996,#28997,#28998,#28999,#29000,#29001,#29002,#29003,#29004,#29005,
#29006,#29007,#29008,#29009,#29010,#29011,#29012,#29013,#29014,#29015,#29016,
#29017,#29018,#29019,#29020,#29021,#29022,#29023,#29024,#29025,#29026,#29027,
#29028,#29029,#29030,#29031,#29032,#29033,#29034,#29035,#29036,#29037,#29038,
#29039,#29040,#29041,#29042,#29043,#29044,#29045,#29046,#29047,#29048,#29049,
#29050,#29051,#29052,#29053,#29054,#29055,#29056,#29057,#29058,#29059,#29060,
#29061,#29062,#29063,#29064,#29065,#29066,#29067,#29068,#29069,#29070,#29071,
#29072,#29073,#29074,#29075,#29076,#29077,#29078,#29079,#29080,#29081,#29082,
#29083,#29084,#29085,#29086,#29087,#29088,#29089,#29090,#29091,#29092,#29093,
#29094,#29095,#29096,#29097,#29098,#29099,#29100,#29101,#29102,#29103,#29104,
#29105,#29106,#29107),.UNSPECIFIED.,.F.,.F.,(4,2,2,2,2,2,2,2,2,2,2,2,2,
2,2,2,2,2,2,2,2,2,2,2,2,2,2,2,2,2,2,2,2,2,2,2,2,2,2,2,2,2,2,2,2,2,2,2,2,
2,2,2,2,2,2,2,2,2,2,2,2,2,2,2,2,2,2,2,2,2,2,2,2,2,2,2,2,2,2,2,2,2,2,2,2,
2,2,2,2,2,2,2,2,2,2,2,2,2,2,2,2,2,2,2,2,2,2,2,2,2,2,2,2,2,2,2,2,2,2,2,2,
2,2,2,2,2,2,2,2,2,2,2,2,2,2,2,2,2,2,2,2,2,2,2,2,2,2,2,2,2,2,2,2,2,2,2,2,
2,2,2,2,2,2,2,2,2,2,2,2,2,2,2,2,2,2,2,2,2,2,4),(12.2073821909332,12.2335108175185,
12.3299598799027,12.359669725321,12.379636103873,12.4033111185916,12.4533462044853,
12.4932615289407,12.66879152795,12.6866512872709,12.7890113437492,12.8362015980871,
12.8734497250337,12.9169400247124,13.0025007637647,13.1285337363769,13.2892804868801,
13.3239529316366,13.3427106131057,13.3638055097289,13.4000005239578,13.6698456745913,
13.763805228594,13.8091048954636,13.846284188843,13.8913684087509,13.9875932290115,
14.1440986993087,14.1602490901029,14.2676653884496,14.2977332044632,14.3177478629965,
14.3412407243228,14.3902072356886,14.4288524664773,14.592872378819,14.7144029361213,
14.7666914242695,14.8044963844781,14.8453284056641,14.9151990047304,14.9639021863386,
15.1380718922427,15.2375839381707,15.2673088456427,15.2872770337817,15.3109437657025,
15.3609308073712,15.4007887503178,15.5757787134379,15.5801640021051,15.6932087792408,
15.7411479955948,15.7785240519513,15.8209922723131,15.9002867660881,16.0113452242571,
16.2016950323066,16.233895139588,16.2540426958676,16.2765450004068,16.3199810428799,
16.3523932020669,16.4709609251633,16.5407207889432,16.6301590977717,16.6931043977956,
16.7326916193452,16.7711479806587,16.8276208164989,16.9820013316163,17.1710067511695,
17.2031455466139,17.2232827939903,17.2458071437963,17.2893615554697,17.3506067208589,
17.5876451688366,17.6569439452046,17.6976736459204,17.735518169528,17.7880852689427,
17.9692824278461,18.1363571134062,18.1705080951362,18.1891756527205,18.210392060249,
18.247199862594,18.2954653410335,18.4262365426923,18.5742167558884,18.6343215100856,
18.6695067476063,18.7077031839726,18.7625828700015,18.7969096618638,18.8937932623165,
19.0205917530423,19.1147345320124,19.1442990317169,19.164246283408,19.1879975186905,
19.2384868622976,19.3968527023198,19.5628872508156,19.6090775458069,19.6469285652457,
19.6867696000186,19.7511273021494,19.7942853784863,19.9332309222493,19.9885447352403,
20.0837452695773,20.1133884240324,20.1333457652756,20.1570550352196,20.2072950257437,
20.2474569200636,20.4253465244089,20.5393278456696,20.5872168681035,20.624587592034,
20.6670854383346,20.7465582805782,20.8058214030132,20.9189734423972,20.952383185187,
21.0528086576659,21.0824986058953,21.1024619896055,21.1261464813385,21.1762398477189,
21.2162255841325,21.3924288319422,21.4236285255905,21.5174088990174,21.5626807125665,
21.5998592239767,21.6449692039608,21.7413815390771,21.8985009085148,21.9281635907577,
22.0222563778361,22.0518164267903,22.0717629267108,22.0955160994496,22.1460180188203,
22.3043673793578,22.4703984770611,22.5165870426842,22.5544373713324,22.5942784111169,
22.6586379002873,22.7017979415561,22.8407555262912,22.8954534513049,22.9911796912393,
23.0208541392432,23.0408153794863,23.0574552138452,23.0807058927684,23.1178562351819,
23.1984496194167,23.4275355100229,23.4830345879557,23.5208986404524,23.5544995671929,
23.6090937621864,23.6741041743715,23.8191415988856,23.8541325148862,23.9600830243459,
23.9898913709594,24.0098702272613,24.0284682795909,24.0524962523772,24.0917586445026,
24.1804682782649,24.3558152153503,24.41439747201),.UNSPECIFIED.) ;
#238=B_SPLINE_CURVE_WITH_KNOTS('',3,(#29112,#29113,#29114,#29115,#29116,
#29117,#29118,#29119,#29120,#29121,#29122,#29123,#29124,#29125,#29126,#29127,
#29128,#29129,#29130,#29131,#29132,#29133,#29134,#29135,#29136,#29137,#29138,
#29139,#29140,#29141,#29142,#29143,#29144,#29145,#29146,#29147,#29148,#29149,
#29150,#29151,#29152,#29153,#29154,#29155,#29156,#29157,#29158,#29159,#29160,
#29161,#29162,#29163,#29164,#29165,#29166,#29167,#29168,#29169,#29170,#29171,
#29172,#29173,#29174,#29175,#29176,#29177,#29178,#29179,#29180,#29181,#29182,
#29183,#29184,#29185,#29186,#29187,#29188,#29189,#29190,#29191,#29192,#29193,
#29194,#29195,#29196,#29197,#29198,#29199,#29200,#29201,#29202,#29203,#29204,
#29205,#29206,#29207,#29208,#29209,#29210,#29211,#29212,#29213,#29214,#29215,
#29216,#29217,#29218,#29219,#29220,#29221,#29222,#29223,#29224,#29225,#29226,
#29227,#29228,#29229,#29230,#29231,#29232,#29233,#29234,#29235,#29236,#29237,
#29238,#29239,#29240,#29241,#29242,#29243,#29244,#29245,#29246,#29247,#29248,
#29249,#29250,#29251,#29252,#29253,#29254,#29255,#29256,#29257,#29258,#29259,
#29260,#29261,#29262,#29263,#29264,#29265,#29266,#29267,#29268,#29269,#29270,
#29271,#29272,#29273,#29274,#29275,#29276,#29277,#29278,#29279,#29280,#29281,
#29282,#29283,#29284,#29285,#29286,#29287,#29288,#29289,#29290,#29291,#29292,
#29293,#29294,#29295,#29296,#29297,#29298,#29299,#29300,#29301,#29302,#29303,
#29304,#29305,#29306,#29307,#29308,#29309,#29310,#29311,#29312,#29313,#29314,
#29315,#29316,#29317,#29318,#29319,#29320,#29321,#29322,#29323,#29324,#29325,
#29326,#29327,#29328,#29329,#29330,#29331,#29332,#29333,#29334,#29335,#29336,
#29337,#29338,#29339,#29340,#29341,#29342,#29343,#29344,#29345,#29346,#29347,
#29348,#29349,#29350,#29351,#29352,#29353,#29354,#29355,#29356,#29357,#29358,
#29359,#29360,#29361,#29362,#29363,#29364,#29365,#29366,#29367,#29368,#29369,
#29370,#29371,#29372,#29373,#29374,#29375,#29376,#29377,#29378,#29379,#29380,
#29381,#29382,#29383,#29384,#29385,#29386,#29387,#29388,#29389,#29390,#29391,
#29392,#29393,#29394,#29395,#29396,#29397,#29398,#29399,#29400,#29401,#29402,
#29403,#29404,#29405,#29406,#29407,#29408,#29409,#29410,#29411,#29412,#29413,
#29414,#29415),.UNSPECIFIED.,.F.,.F.,(4,3,3,3,3,3,3,3,3,3,3,3,3,3,3,3,3,
3,3,3,3,3,3,3,3,3,3,3,3,3,3,3,3,3,3,3,3,3,3,3,3,3,3,3,3,3,3,3,3,3,3,3,3,
3,3,3,3,3,3,3,3,3,3,3,3,3,3,3,3,3,3,3,3,3,3,3,3,3,3,3,3,3,3,3,3,3,3,3,3,
3,3,3,3,3,3,3,3,3,3,3,3,4),(-54.3584733375017,-54.2962473358395,-54.2340310509242,
-54.1718213867751,-54.1096152496348,-54.0474030002711,-53.9851897965479,
-53.9229636429728,-53.8768370136655,-53.8144795634182,-53.752169349007,
-53.6898658214558,-53.6275660802489,-53.5651689131085,-53.5028627810232,
-53.4404200963551,-53.3779774116871,-53.3156199614398,-53.2533097470287,
-53.1910062194775,-53.1287064782702,-53.0663093111299,-53.0040031790443,
-52.9415604943765,-52.8791178097087,-52.8167603594614,-52.7544501450502,
-52.6921466174993,-52.6298468762923,-52.5674497091518,-52.5051435770666,
-52.4427008923984,-52.3802582077303,-52.317900757483,-52.2555905430719,
-52.1932870155204,-52.1309872743138,-52.0685901071733,-52.0062839750878,
-51.9438412904198,-51.8813986057519,-51.8190411555046,-51.7567309410938,
-51.6944274135426,-51.6321276723354,-51.569730505195,-51.5074243731099,
-51.4449816884418,-51.3825390037736,-51.3201815535263,-51.2578713391152,
-51.1955678115636,-51.1332680703565,-51.0708709032162,-51.0085647711309,
-50.9461220864631,-50.8836794017952,-50.8213219515479,-50.7590117371368,
-50.6967082095859,-50.6344084683787,-50.5720113012383,-50.5097051691533,
-50.447262484485,-50.3848197998168,-50.3224623495695,-50.2601521351584,
-50.1978486076073,-50.1355488664007,-50.0731516992601,-50.0108455671745,
-49.9484028825064,-49.8859601978384,-49.8236027475911,-49.7612925331797,
-49.6989890056283,-49.6366892644216,-49.5742920972812,-49.5119859651957,
-49.4495432805279,-49.38710059586,-49.3247431456127,-49.2624329312014,-49.2001294036503,
-49.1378296624429,-49.0754324953026,-49.0131263632179,-48.9506836785498,
-48.8882409938817,-48.8258835436344,-48.7635733292232,-48.7012698016721,
-48.6389700604652,-48.5765728933247,-48.5142667612395,-48.4518240765714,
-48.3893813919033,-48.3269379190192,-48.264025446856,-48.2015992973433,
-48.138443663855,-48.0752880303667),.UNSPECIFIED.) ;
#239=B_SPLINE_CURVE_WITH_KNOTS('',3,(#29416,#29417,#29418,#29419,#29420,
#29421,#29422,#29423,#29424,#29425,#29426,#29427,#29428,#29429,#29430,#29431,
#29432,#29433,#29434,#29435,#29436,#29437,#29438,#29439,#29440,#29441,#29442,
#29443,#29444,#29445,#29446,#29447,#29448,#29449,#29450,#29451,#29452,#29453,
#29454,#29455,#29456,#29457,#29458,#29459,#29460,#29461,#29462,#29463,#29464,
#29465,#29466,#29467,#29468,#29469,#29470,#29471,#29472,#29473,#29474,#29475,
#29476,#29477,#29478,#29479,#29480,#29481,#29482,#29483,#29484,#29485,#29486,
#29487,#29488,#29489,#29490,#29491,#29492,#29493,#29494,#29495,#29496,#29497,
#29498,#29499,#29500,#29501,#29502,#29503,#29504,#29505,#29506,#29507,#29508,
#29509,#29510,#29511,#29512,#29513,#29514,#29515,#29516,#29517,#29518,#29519,
#29520,#29521,#29522,#29523,#29524,#29525,#29526,#29527,#29528,#29529,#29530,
#29531,#29532,#29533,#29534,#29535,#29536,#29537,#29538,#29539,#29540,#29541,
#29542,#29543,#29544,#29545,#29546,#29547,#29548,#29549,#29550,#29551,#29552,
#29553,#29554,#29555,#29556,#29557,#29558,#29559,#29560,#29561,#29562,#29563,
#29564,#29565,#29566,#29567,#29568,#29569,#29570,#29571,#29572,#29573,#29574,
#29575,#29576,#29577,#29578,#29579,#29580,#29581,#29582,#29583,#29584,#29585,
#29586,#29587,#29588,#29589,#29590,#29591,#29592,#29593,#29594,#29595,#29596,
#29597,#29598,#29599,#29600,#29601,#29602,#29603,#29604,#29605,#29606,#29607,
#29608,#29609,#29610,#29611,#29612,#29613,#29614,#29615,#29616,#29617,#29618,
#29619,#29620,#29621,#29622,#29623,#29624,#29625,#29626,#29627,#29628,#29629,
#29630,#29631,#29632,#29633,#29634,#29635,#29636,#29637,#29638,#29639,#29640,
#29641,#29642,#29643,#29644,#29645,#29646,#29647,#29648,#29649,#29650,#29651,
#29652,#29653,#29654,#29655,#29656,#29657,#29658,#29659,#29660,#29661,#29662,
#29663,#29664,#29665,#29666,#29667,#29668,#29669,#29670,#29671,#29672,#29673,
#29674,#29675,#29676,#29677,#29678,#29679,#29680,#29681,#29682,#29683,#29684,
#29685,#29686,#29687,#29688,#29689,#29690,#29691,#29692,#29693,#29694,#29695,
#29696,#29697,#29698,#29699,#29700,#29701,#29702,#29703,#29704,#29705,#29706,
#29707,#29708,#29709,#29710,#29711,#29712,#29713,#29714,#29715,#29716,#29717,
#29718,#29719,#29720,#29721,#29722,#29723,#29724,#29725,#29726,#29727,#29728,
#29729,#29730,#29731,#29732,#29733,#29734,#29735,#29736,#29737,#29738,#29739,
#29740,#29741,#29742,#29743,#29744,#29745,#29746,#29747,#29748,#29749,#29750,
#29751,#29752,#29753,#29754,#29755,#29756,#29757,#29758,#29759,#29760,#29761,
#29762,#29763,#29764,#29765,#29766,#29767,#29768,#29769,#29770,#29771,#29772,
#29773,#29774,#29775,#29776,#29777,#29778,#29779,#29780,#29781,#29782,#29783,
#29784,#29785,#29786,#29787,#29788,#29789,#29790,#29791,#29792,#29793,#29794,
#29795,#29796,#29797,#29798,#29799,#29800,#29801,#29802,#29803,#29804,#29805,
#29806,#29807,#29808,#29809),.UNSPECIFIED.,.F.,.F.,(4,2,2,2,2,2,2,2,2,2,
2,2,2,2,2,2,2,2,2,2,2,2,2,2,2,2,2,2,2,2,2,2,2,2,2,2,2,2,2,2,2,2,2,2,2,2,
2,2,2,2,2,2,2,2,2,2,2,2,2,2,2,2,2,2,2,2,2,2,2,2,2,2,2,2,2,2,2,2,2,2,2,2,
2,2,2,2,2,2,2,2,2,2,2,2,2,2,2,2,2,2,2,2,2,2,2,2,2,2,2,2,2,2,2,2,2,2,2,2,
2,2,2,2,2,2,2,2,2,2,2,2,2,2,2,2,2,2,2,2,2,2,2,2,2,2,2,2,2,2,2,2,2,2,2,2,
2,2,2,2,2,2,2,2,2,2,2,2,2,2,2,2,2,2,2,2,2,2,2,2,2,2,2,2,2,2,2,2,2,2,2,2,
2,2,2,2,2,2,4),(8.42914463236037E-5,0.0379717091092616,0.0736004856464233,
0.111473526474535,0.167020001785984,0.317233552160938,0.505139405702036,
0.534949880889817,0.55357464234073,0.573529591958853,0.603153569578424,
0.698067353575928,0.824841874188393,0.921254879414346,0.973802149138873,
1.01159198463408,1.04328096525734,1.08124253197859,1.13727922809431,1.31362105569038,
1.42846726630663,1.47367222863448,1.475123949699,1.47616049958101,1.47826043255324,
1.48011910574621,1.48176445634631,1.48322140215602,1.48451207107788,1.4856560462315,
1.48667061299986,1.48757099891463,1.48837060052546,1.48908119374871,1.48971312584074,
1.49027548848422,1.49077627235489,1.49122250407503,1.49162036687352,1.49197530637639,
1.4922921231375,1.49257505325408,1.49282783861581,1.49356172595305,1.49426540413618,
1.51454008506316,1.52896115409072,1.54771820193755,1.58238781940073,1.743496899363,
1.92963920949245,1.98222828653364,2.02007603697584,2.06079794993105,2.13005292476935,
2.36715764379405,2.42840755269984,2.47196437793416,2.49448920784632,2.51462629013244,
2.54676395544301,2.73577335762321,2.89015668344801,2.94663001587642,2.98508651664267,
3.02467371278034,3.0876186215798,3.17705649078552,3.34862863024698,3.38811925433987,
3.43779904785868,3.46141373843161,3.48139534210748,3.51122103003068,3.61278413786048,
3.81457167343543,3.89570451511808,3.93847874779858,3.9758077862152,4.02325584262599,
4.13461652018255,4.14179323143894,4.31696781496736,4.35684517903941,4.40684849789668,
4.43051802538501,4.45048558308685,4.48020536235353,4.57988215993593,4.630397590054,
4.76945331042978,4.81263152939806,4.87701005759037,4.91685518757331,4.95470452532019,
5.0008856662727,5.16690394656811,5.32514240431074,5.37574589160291,5.3995164322811,
5.41945938440006,5.44898877434882,5.54272584624629,5.59981405266092,5.73872353145172,
5.78187549420257,5.84622720775365,5.88606762328978,5.92391998744518,5.97011438487237,
6.13615207424831,6.29455448153151,6.3450121274628,6.36875828692691,6.38870716422874,
6.41828234765136,6.51254958461194,6.56898841175525,6.7079126232618,6.75106731360748,
6.81542190354679,6.85526295200383,6.89311519239849,6.93930851464101,7.10534542211121,
7.2637337335032,7.28812340851755,7.3236626930908,7.34462883399883,7.36349196989876,
7.39876669505061,7.59746873301997,7.70040152346541,7.77598702393112,7.81782410906911,
7.85532652117246,7.90440190090633,8.03097055259366,8.19623428326075,8.23502212293775,
8.28410973392786,8.30762352669691,8.32763259646727,8.35765893967885,8.46955534934651,
8.59617419100339,8.68328405047701,8.75098629434154,8.79143024598732,8.82939818498459,
8.88280028053755,9.10383230051427,9.22599132024928,9.26184394033772,9.28287146140896,
9.30168304254138,9.33666410090269,9.44380113818884,9.60502335128768,9.65186851590099,
9.71992938011551,9.76043778765256,9.79837669551035,9.85158440980379,10.0737203701549,
10.1953370549295,10.2311288128344,10.2521444038105,10.2709658545005,10.3060031643562,
10.5056190625521,10.6082871429532,10.6837481119395,10.7255637860518,10.7630713946087,
10.812188969959,10.9438134631646,11.1049940917399,11.1433088797067,11.1919945336148,
11.2154392507245,11.235468013524,11.2656351550321,11.3750567230316,11.4127992358692,
11.553222914681,11.5966462616358,11.6612757849033,11.7011664832244,11.7389900921116,
11.7850521901086,11.9269428949954,12.0772646034911,12.1287980077517,12.1673772153281,
12.1889465269692,12.2073941385125),.UNSPECIFIED.) ;
#240=B_SPLINE_CURVE_WITH_KNOTS('',3,(#29814,#29815,#29816,#29817,#29818,
#29819,#29820,#29821,#29822,#29823,#29824,#29825,#29826,#29827,#29828,#29829,
#29830,#29831,#29832,#29833,#29834,#29835,#29836,#29837,#29838,#29839,#29840,
#29841,#29842,#29843,#29844,#29845,#29846,#29847,#29848,#29849,#29850,#29851,
#29852,#29853,#29854,#29855,#29856,#29857,#29858,#29859,#29860,#29861,#29862,
#29863,#29864,#29865,#29866,#29867,#29868,#29869,#29870,#29871,#29872,#29873,
#29874,#29875,#29876,#29877,#29878,#29879,#29880,#29881,#29882,#29883,#29884,
#29885,#29886,#29887,#29888,#29889,#29890,#29891,#29892,#29893,#29894,#29895,
#29896,#29897,#29898,#29899,#29900,#29901,#29902,#29903,#29904,#29905,#29906,
#29907,#29908,#29909,#29910,#29911,#29912,#29913,#29914,#29915,#29916,#29917,
#29918,#29919,#29920,#29921,#29922,#29923,#29924,#29925,#29926,#29927,#29928,
#29929,#29930,#29931,#29932,#29933,#29934,#29935,#29936,#29937,#29938,#29939,
#29940,#29941,#29942,#29943,#29944,#29945,#29946,#29947,#29948,#29949,#29950,
#29951,#29952,#29953,#29954,#29955,#29956,#29957,#29958,#29959,#29960,#29961,
#29962,#29963,#29964,#29965,#29966,#29967,#29968,#29969,#29970,#29971,#29972,
#29973,#29974,#29975,#29976,#29977,#29978,#29979,#29980,#29981,#29982,#29983,
#29984,#29985,#29986,#29987,#29988,#29989,#29990,#29991,#29992,#29993,#29994,
#29995,#29996,#29997,#29998,#29999,#30000,#30001,#30002,#30003,#30004,#30005,
#30006,#30007,#30008,#30009,#30010,#30011,#30012,#30013,#30014,#30015,#30016,
#30017,#30018,#30019,#30020,#30021,#30022,#30023,#30024,#30025,#30026,#30027,
#30028,#30029,#30030,#30031,#30032,#30033,#30034,#30035,#30036,#30037,#30038,
#30039,#30040,#30041,#30042,#30043,#30044,#30045,#30046,#30047,#30048,#30049,
#30050,#30051,#30052,#30053,#30054,#30055,#30056,#30057,#30058,#30059,#30060,
#30061,#30062,#30063,#30064,#30065,#30066,#30067,#30068,#30069,#30070,#30071,
#30072,#30073,#30074,#30075,#30076,#30077,#30078,#30079,#30080,#30081,#30082,
#30083,#30084,#30085,#30086,#30087,#30088,#30089,#30090,#30091,#30092,#30093,
#30094,#30095,#30096,#30097,#30098,#30099,#30100,#30101,#30102,#30103,#30104,
#30105,#30106,#30107,#30108,#30109,#30110,#30111,#30112,#30113,#30114,#30115,
#30116,#30117,#30118,#30119,#30120,#30121,#30122,#30123,#30124,#30125,#30126,
#30127,#30128,#30129,#30130,#30131,#30132,#30133,#30134,#30135,#30136,#30137,
#30138,#30139,#30140,#30141,#30142,#30143,#30144,#30145,#30146,#30147,#30148,
#30149,#30150,#30151,#30152,#30153,#30154,#30155,#30156,#30157,#30158,#30159,
#30160,#30161,#30162,#30163,#30164,#30165,#30166,#30167,#30168,#30169,#30170,
#30171,#30172,#30173,#30174,#30175,#30176,#30177,#30178,#30179,#30180,#30181,
#30182,#30183,#30184,#30185,#30186,#30187,#30188,#30189,#30190,#30191),
 .UNSPECIFIED.,.F.,.F.,(4,2,2,2,2,2,2,2,2,2,2,2,2,2,2,2,2,2,2,2,2,2,2,2,
2,2,2,2,2,2,2,2,2,2,2,2,2,2,2,2,2,2,2,2,2,2,2,2,2,2,2,2,2,2,2,2,2,2,2,2,
2,2,2,2,2,2,2,2,2,2,2,2,2,2,2,2,2,2,2,2,2,2,2,2,2,2,2,2,2,2,2,2,2,2,2,2,
2,2,2,2,2,2,2,2,2,2,2,2,2,2,2,2,2,2,2,2,2,2,2,2,2,2,2,2,2,2,2,2,2,2,2,2,
2,2,2,2,2,2,2,2,2,2,2,2,2,2,2,2,2,2,2,2,2,2,2,2,2,2,2,2,2,2,2,2,2,2,2,2,
2,2,2,2,2,2,2,2,2,2,2,2,2,2,2,2,2,2,2,2,4),(12.2074643523629,12.2510803881761,
12.2883180320074,12.3353371243011,12.4466774321583,12.6682126897982,12.7204788088286,
12.7445241480605,12.7624004881259,12.7898456193121,12.8678923586911,13.0347194994456,
13.1521854717311,13.2047004583025,13.2425381103645,13.2832878345502,13.3526954514402,
13.4009193969484,13.5716118896449,13.6758492046428,13.7056014738285,13.72557350327,
13.7492265568158,13.7991314627909,13.8388907598491,14.0129509107426,14.0976376388995,
14.1614522369843,14.2011960752979,14.2395472969524,14.2953814613993,14.3305625597964,
14.4310296607404,14.637522630409,14.6710105909773,14.6895661291709,14.7109526919714,
14.7486110615429,14.7984339371305,14.9381464093486,15.0815732664283,15.1381033189386,
15.1761870585934,15.2156715395401,15.2780412003025,15.3553589401022,15.5816945830979,
15.6294915144264,15.6530683724527,15.6730604222033,15.7029616079101,15.813172166321,
16.054776135241,16.1095205494218,16.1473178936361,16.1872547210646,16.252140473882,
16.295814959929,16.437656944076,16.5719371037958,16.6075966722555,16.6265279426321,
16.6474179656736,16.682565196325,16.7065805514402,16.7461389990475,16.9183306199123,
17.0042489247897,17.0686379592868,17.1084853493193,17.1467713642115,17.2022045788382,
17.2370257813654,17.5022201977551,17.5612904440889,17.5870846028357,17.6067822251668,
17.6329485882213,17.6998887355955,17.8219833864515,17.8374754768821,17.9940003069029,
18.0484104745623,18.0861561469217,18.1261879729017,18.1915998603211,18.2357920985166,
18.3806051357199,18.4299954355254,18.5227153760692,18.5521439148391,18.5720743712274,
18.5959001827515,18.6468333446375,18.805055771765,18.9707261747319,19.0168654435275,
19.0547059901497,19.0945676323238,19.1590356171313,19.202300884865,19.341840284446,
19.3736248368375,19.4808515432485,19.5158392026574,19.5346519865175,19.5556781893222,
19.5915238804521,19.7136200462538,19.9347883507604,19.9881669652328,20.0261314839503,
20.0665833334768,20.1343290372588,20.2215211384079,20.3481368979375,20.4573827572483,
20.488607745454,20.5085968812826,20.531473449926,20.5769455195891,20.6421622662813,
20.8944472580128,20.9521848115145,20.9869984733818,21.0255408652821,21.0825251729922,
21.2408749872914,21.4235403121264,21.4563279828499,21.4747680524404,21.4963505854128,
21.5349972264426,21.5866571617766,21.737799702797,21.8788098486998,21.9248047933719,
21.9626135807268,22.0025295478043,22.0673003824412,22.1108622458796,22.2520671713703,
22.2707721174684,22.3881315118216,22.4233417510973,22.4421935090534,22.4631728105367,
22.4987796572793,22.52323410308,22.6814825622351,22.847505797266,22.8936874985564,
22.9315371282327,22.9669806785719,22.9685774877449,22.9702809011894,22.9721163437289,
22.9741135066938,22.976307552976,22.978740559645,22.9814632409231,22.9845369755012,
22.9880361193795,22.9920504992698,22.996687822658,22.9987967732181,23.0019792913726,
23.1299912527637,23.237551300046,23.3568775224537,23.3916479673123,23.406909112261,
23.4214491618102,23.4406719877125,23.4667344349675,23.5116352457113,23.6250013681698,
23.6699341512628,23.8162833611432,23.8626152147707,23.9004979981165,23.9353795627966,
23.974761624626,24.1173917648754,24.3050605783251,24.3522425303142,24.3759138015097,
24.3947801408357,24.4149503713271),.UNSPECIFIED.) ;
#241=B_SPLINE_CURVE_WITH_KNOTS('',3,(#30192,#30193,#30194,#30195,#30196,
#30197,#30198,#30199,#30200,#30201,#30202,#30203,#30204,#30205,#30206,#30207,
#30208,#30209,#30210,#30211,#30212,#30213,#30214,#30215,#30216,#30217,#30218,
#30219,#30220,#30221,#30222,#30223,#30224,#30225,#30226,#30227,#30228,#30229,
#30230,#30231,#30232,#30233,#30234,#30235,#30236,#30237,#30238,#30239,#30240,
#30241,#30242,#30243,#30244,#30245,#30246,#30247,#30248,#30249,#30250,#30251,
#30252,#30253,#30254,#30255,#30256,#30257,#30258,#30259,#30260,#30261,#30262,
#30263,#30264,#30265,#30266,#30267,#30268,#30269,#30270,#30271,#30272,#30273,
#30274,#30275,#30276,#30277,#30278,#30279,#30280,#30281,#30282,#30283,#30284,
#30285,#30286,#30287,#30288,#30289,#30290,#30291,#30292,#30293,#30294,#30295,
#30296,#30297,#30298,#30299,#30300,#30301,#30302,#30303,#30304,#30305,#30306,
#30307,#30308,#30309,#30310,#30311,#30312,#30313,#30314,#30315,#30316,#30317,
#30318,#30319,#30320,#30321,#30322,#30323,#30324,#30325,#30326,#30327,#30328,
#30329,#30330,#30331,#30332,#30333,#30334,#30335,#30336,#30337,#30338,#30339,
#30340,#30341,#30342,#30343,#30344,#30345,#30346,#30347,#30348,#30349,#30350,
#30351,#30352,#30353,#30354,#30355,#30356,#30357,#30358,#30359,#30360,#30361,
#30362,#30363,#30364,#30365,#30366,#30367,#30368,#30369,#30370,#30371,#30372,
#30373,#30374,#30375,#30376,#30377,#30378,#30379,#30380,#30381,#30382,#30383,
#30384,#30385,#30386,#30387,#30388,#30389,#30390,#30391,#30392,#30393,#30394,
#30395,#30396,#30397,#30398,#30399,#30400,#30401,#30402,#30403,#30404,#30405,
#30406,#30407,#30408,#30409,#30410,#30411,#30412,#30413,#30414,#30415,#30416,
#30417,#30418,#30419,#30420,#30421,#30422,#30423,#30424,#30425,#30426,#30427,
#30428,#30429,#30430,#30431,#30432,#30433,#30434,#30435,#30436,#30437,#30438,
#30439,#30440,#30441,#30442,#30443,#30444,#30445,#30446,#30447,#30448,#30449,
#30450,#30451,#30452,#30453,#30454,#30455,#30456,#30457,#30458,#30459,#30460,
#30461,#30462,#30463,#30464,#30465,#30466,#30467,#30468,#30469,#30470,#30471,
#30472,#30473,#30474,#30475,#30476,#30477,#30478,#30479,#30480,#30481,#30482,
#30483,#30484,#30485,#30486,#30487,#30488,#30489,#30490,#30491,#30492,#30493,
#30494,#30495,#30496,#30497,#30498,#30499,#30500,#30501,#30502,#30503,#30504,
#30505,#30506,#30507,#30508,#30509,#30510,#30511,#30512,#30513,#30514,#30515,
#30516,#30517,#30518,#30519,#30520,#30521,#30522,#30523,#30524,#30525,#30526,
#30527,#30528,#30529,#30530,#30531,#30532,#30533,#30534,#30535,#30536,#30537,
#30538,#30539,#30540,#30541,#30542,#30543,#30544,#30545,#30546,#30547,#30548,
#30549,#30550,#30551,#30552,#30553,#30554,#30555,#30556,#30557,#30558,#30559,
#30560,#30561,#30562,#30563,#30564,#30565,#30566,#30567,#30568,#30569,#30570,
#30571,#30572,#30573,#30574,#30575,#30576,#30577,#30578,#30579,#30580,#30581,
#30582,#30583,#30584,#30585,#30586,#30587,#30588,#30589,#30590,#30591,#30592,
#30593,#30594,#30595),.UNSPECIFIED.,.F.,.F.,(4,2,2,2,2,2,2,2,2,2,2,2,2,
2,2,2,2,2,2,2,2,2,2,2,2,2,2,2,2,2,2,2,2,2,2,2,2,2,2,2,2,2,2,2,2,2,2,2,2,
2,2,2,2,2,2,2,2,2,2,2,2,2,2,2,2,2,2,2,2,2,2,2,2,2,2,2,2,2,2,2,2,2,2,2,2,
2,2,2,2,2,2,2,2,2,2,2,2,2,2,2,2,2,2,2,2,2,2,2,2,2,2,2,2,2,2,2,2,2,2,2,2,
2,2,2,2,2,2,2,2,2,2,2,2,2,2,2,2,2,2,2,2,2,2,2,2,2,2,2,2,2,2,2,2,2,2,2,2,
2,2,2,2,2,2,2,2,2,2,2,2,2,2,2,2,2,2,2,2,2,2,2,2,2,2,2,2,2,2,2,2,2,2,2,2,
2,2,2,2,2,2,2,2,4),(12.2073941385125,12.2402277463726,12.2620763310274,
12.3272670935593,12.5802781988266,12.6376944261202,12.672458709584,12.7110554746234,
12.7683607958391,12.929260864507,13.1070412498584,13.1406838558017,13.1592653645263,
13.1806110691908,13.2180644095471,13.2675098091101,13.4049956667988,13.4603376119083,
13.5718096540163,13.6192907211529,13.6566232879607,13.6993774303379,13.7803859555984,
13.985102861166,14.0841261389353,14.1138642469289,14.133834455417,14.1574949936934,
14.2074438455509,14.2472556898354,14.4218081857704,14.5402824015585,14.5880396880502,
14.6253982920502,14.6679785308719,14.7479397534326,15.0101718030228,15.0650846189291,
15.0898977721188,15.1094767154397,15.1371860434586,15.2178389622492,15.3979808805493,
15.5099669470672,15.557576848642,15.5949215325385,15.637594074765,15.7181090672836,
15.8319512896149,16.0170989026736,16.0495351425806,16.0697231547625,16.0921431083163,
16.1351367198853,16.1952448931677,16.4184621045062,16.4961897031074,16.5388011696546,
16.5724162675553,16.6188316749206,16.7251238282469,16.9202378288812,16.9373526937547,
16.9997737458706,17.0257826125564,17.0454821922326,17.0714327270402,17.1366993754574,
17.2532640785524,17.3156173902785,17.4401716471949,17.4864430803509,17.5243127165114,
17.5641251944169,17.6283200941376,17.6713188645151,17.8093800675466,17.8327271117422,
17.9498780016721,17.9852861878183,18.0041729606285,18.0251123281562,18.0605137665094,
18.0847715613042,18.1248997809032,18.3024587782809,18.4169858554173,18.4648290923152,
18.5021962697318,18.544724127103,18.6243709266633,18.6838364470958,18.8196312704273,
18.9292916969126,18.9594869148141,18.9795196804231,19.0029508627655,19.0515578999591,
19.0897805304463,19.2501783583851,19.3827794571685,19.4319061182526,19.4694148995634,
19.5112260819638,19.5866607633317,19.6892728136684,19.8890747185072,19.9240638087518,
19.9428768412877,19.9639027354199,19.9997468652963,20.1218291408583,20.3430258769336,
20.396399366038,20.4343631114911,20.4748166376966,20.5425716953716,20.6297815788976,
20.756396931293,20.8659003903521,20.8969824554747,20.9169494013343,20.9398852354991,
20.9856854428877,21.051595639326,21.2372716604169,21.3338551891554,21.3789900859218,
21.4161695752109,21.4614187244392,21.5588225609816,21.7192223136479,21.8273847351294,
21.8624407136265,21.8812654043188,21.902276959806,21.9380483773288,21.9626607089466,
22.1208406636643,22.2865907302731,22.3327294816639,22.3705697553468,22.4104312634578,
22.4748994070042,22.5181649442971,22.6577064435626,22.6894020266327,22.7967023059467,
22.8316952164351,22.8505088468344,22.8647992054061,22.8839837746901,22.8845685791001,
22.8851763591001,22.8858084486113,22.8864662668027,22.8871513239457,22.8878652276767,
22.8886096896721,22.8893865327876,22.8896415311894,22.8899266823925,22.8902457310949,
22.8906029244097,22.8910030861364,22.89145170288,22.8919550240197,22.8925201774645,
22.8931553036475,22.8938697102046,22.8946740498672,22.8955805241163,22.8966031147916,
22.8977578452999,22.8990630721213,22.9005398055998,22.9022120567559,22.9041072032384,
22.947517097388,23.0538776382587,23.2440538574769,23.3003757495573,23.3384253462907,
23.3709547725524,23.4205897152378,23.4823122802948,23.6127045873432,23.6546966511943,
23.6758343404169,23.7764285743187,23.8061122741945,23.8260752302238,23.8446917280693,
23.8747983291818,23.8838035469633,23.9768535759189,24.1132601416553,24.2318215601649,
24.2798122853754,24.3157026486367,24.3506131919194,24.4148629559983),
 .UNSPECIFIED.) ;
#242=B_SPLINE_CURVE_WITH_KNOTS('',3,(#30600,#30601,#30602,#30603,#30604,
#30605,#30606,#30607,#30608,#30609,#30610,#30611,#30612,#30613,#30614,#30615,
#30616,#30617,#30618,#30619,#30620,#30621,#30622,#30623,#30624,#30625,#30626,
#30627,#30628,#30629,#30630,#30631,#30632,#30633,#30634,#30635,#30636,#30637,
#30638,#30639,#30640,#30641,#30642,#30643,#30644,#30645,#30646,#30647,#30648,
#30649,#30650,#30651,#30652,#30653,#30654,#30655,#30656,#30657,#30658,#30659,
#30660,#30661,#30662,#30663,#30664,#30665,#30666,#30667,#30668,#30669,#30670,
#30671,#30672,#30673,#30674,#30675,#30676,#30677,#30678,#30679,#30680,#30681,
#30682,#30683,#30684,#30685,#30686,#30687,#30688,#30689,#30690,#30691,#30692,
#30693,#30694,#30695,#30696,#30697,#30698,#30699,#30700,#30701,#30702,#30703,
#30704,#30705,#30706,#30707,#30708,#30709,#30710,#30711,#30712,#30713,#30714,
#30715,#30716,#30717,#30718,#30719,#30720,#30721,#30722,#30723,#30724,#30725,
#30726,#30727,#30728,#30729,#30730,#30731,#30732,#30733,#30734,#30735,#30736,
#30737,#30738,#30739,#30740,#30741,#30742,#30743,#30744,#30745,#30746,#30747,
#30748,#30749,#30750,#30751,#30752,#30753,#30754,#30755,#30756,#30757,#30758,
#30759,#30760,#30761,#30762,#30763,#30764,#30765,#30766,#30767,#30768,#30769,
#30770,#30771,#30772,#30773,#30774,#30775,#30776,#30777,#30778,#30779,#30780,
#30781,#30782,#30783,#30784,#30785,#30786,#30787,#30788,#30789,#30790,#30791,
#30792,#30793,#30794,#30795,#30796,#30797,#30798,#30799,#30800,#30801,#30802,
#30803,#30804,#30805,#30806,#30807,#30808,#30809,#30810,#30811,#30812,#30813,
#30814,#30815,#30816,#30817,#30818,#30819,#30820,#30821,#30822,#30823,#30824,
#30825,#30826,#30827,#30828,#30829,#30830,#30831,#30832,#30833,#30834,#30835,
#30836,#30837,#30838,#30839,#30840,#30841,#30842,#30843,#30844,#30845,#30846,
#30847,#30848,#30849,#30850,#30851,#30852,#30853,#30854,#30855,#30856,#30857,
#30858,#30859,#30860,#30861,#30862,#30863,#30864,#30865,#30866,#30867,#30868,
#30869,#30870,#30871,#30872,#30873,#30874,#30875,#30876,#30877,#30878,#30879,
#30880,#30881,#30882,#30883,#30884,#30885,#30886,#30887,#30888,#30889,#30890,
#30891,#30892,#30893,#30894,#30895,#30896,#30897,#30898,#30899,#30900,#30901,
#30902,#30903,#30904,#30905,#30906,#30907,#30908,#30909,#30910,#30911,#30912,
#30913,#30914,#30915,#30916,#30917,#30918,#30919,#30920,#30921,#30922,#30923,
#30924,#30925,#30926,#30927,#30928,#30929,#30930,#30931,#30932,#30933,#30934,
#30935,#30936,#30937,#30938,#30939,#30940,#30941,#30942,#30943,#30944,#30945,
#30946,#30947,#30948,#30949,#30950,#30951,#30952,#30953,#30954,#30955,#30956,
#30957,#30958,#30959,#30960,#30961,#30962,#30963,#30964,#30965,#30966,#30967,
#30968,#30969,#30970,#30971,#30972,#30973,#30974,#30975,#30976,#30977,#30978,
#30979,#30980,#30981,#30982,#30983,#30984,#30985,#30986,#30987,#30988,#30989,
#30990,#30991,#30992,#30993,#30994,#30995,#30996,#30997,#30998,#30999,#31000,
#31001),.UNSPECIFIED.,.F.,.F.,(4,2,2,2,2,2,2,2,2,2,2,2,2,2,2,2,2,2,2,2,
2,2,2,2,2,2,2,2,2,2,2,2,2,2,2,2,2,2,2,2,2,2,2,2,2,2,2,2,2,2,2,2,2,2,2,2,
2,2,2,2,2,2,2,2,2,2,2,2,2,2,2,2,2,2,2,2,2,2,2,2,2,2,2,2,2,2,2,2,2,2,2,2,
2,2,2,2,2,2,2,2,2,2,2,2,2,2,2,2,2,2,2,2,2,2,2,2,2,2,2,2,2,2,2,2,2,2,2,2,
2,2,2,2,2,2,2,2,2,2,2,2,2,2,2,2,2,2,2,2,2,2,2,2,2,2,2,2,2,2,2,2,2,2,2,2,
2,2,2,2,2,2,2,2,2,2,2,2,2,2,2,2,2,2,2,2,2,2,2,2,2,2,2,2,2,2,2,2,2,2,2,2,
4),(0.000300064236370683,0.0723647523763316,0.111708964416556,0.133287846849445,
0.151427998569037,0.17013081821157,0.204487533123056,0.373915727662253,
0.537245797439023,0.570889420460193,0.596385588041295,0.631244919618651,
0.668999717700598,0.714747735427124,0.952409100978459,1.03593112393576,
1.07385966190513,1.10398883900008,1.11932044457847,1.13772612486928,1.17030222790595,
1.35876937254578,1.47049448971958,1.52745299964897,1.53168771270016,1.53535849172675,
1.53857162794452,1.54141187276103,1.5439470340794,1.54623167307539,1.54831002122938,
1.55021826097559,1.55198630429099,1.55363918342455,1.55519814630363,1.55668153004232,
1.55810547054093,1.559484494541,1.56083203232386,1.56216088437471,1.56348367356664,
1.56481331618967,1.56616355164705,1.60155322785786,1.63946693853557,1.68594048847265,
1.94848653822088,2.01577373849035,2.06221959112931,2.08527095315853,2.10519629497473,
2.13084457801574,2.21445944474567,2.23554690278583,2.3621746902663,2.42952807234498,
2.47051079859878,2.53261391621636,2.57205030529448,2.61016783628193,2.66690564154787,
2.81677996189875,2.97663844412068,3.0285960169111,3.05259073381019,3.07248411879497,
3.10161000549298,3.1919375061799,3.23252290104051,3.38535656667436,3.45196785765083,
3.50810142678944,3.54650165838166,3.58617065584388,3.64957052680161,3.73789184711398,
3.80749417098868,3.92634500745432,3.95880285775157,4.00228136249625,4.02479165207644,
4.04493560566148,4.07711391642218,4.26440509197348,4.40632405735721,4.46975103458349,
4.50942489693709,4.54737955021244,4.59403475245416,4.75738974052942,4.91941144723466,
4.96841971448581,4.99191978946321,5.01193249829625,5.04198595384655,5.14906647062526,
5.18878183592139,5.32960245465832,5.39370579429852,5.44831832084239,5.48647268635229,
5.52171219460949,5.58215554063168,5.67786011361571,5.84835696426342,5.88773025204314,
5.91166638340001,5.94673027626426,5.96760405128236,5.98655002035884,6.02229310404073,
6.16357791017453,6.16860445723978,6.30251128132899,6.34474497558316,6.40815118598117,
6.44782139163533,6.48577857146016,6.53244468854559,6.69576748855268,6.85779174181329,
6.90680135080787,6.93030169649483,6.95031440070281,6.98036751682532,7.08733849819573,
7.11498834189863,7.12643693941062,7.26773736289183,7.33194569648429,7.38662239240289,
7.42478697794578,7.46484105145289,7.53037852391577,7.61353026912302,7.78620615773346,
7.82581658647806,7.84985405055683,7.88502445212145,7.90591884726129,7.92484577643522,
7.96048149047412,8.09221411801463,8.23577394466106,8.27974909469319,8.34494044159996,
8.38493211014731,8.42269859623056,8.47724622664784,8.68674670184714,8.8163574987617,
8.85302003660045,8.8742076859909,8.89289613642419,8.92716796190361,9.09303206713614,
9.1304372160529,9.23185397379078,9.30672239106383,9.34843529249482,9.38596755269279,
9.4352880210662,9.57271885683992,9.59274033742292,9.73358572025248,9.78359783189059,
9.82135874652594,9.84276566457034,9.86130838133924,9.89471999765144,10.1016103456568,
10.201940253525,10.2370889597033,10.2928869478137,10.3312320888182,10.3709847738933,
10.4348494268077,10.522036558219,10.6940016560854,10.7335351245911,10.7832509602547,
10.8068718782516,10.8268520418335,10.8566661305089,10.9628188449026,10.9918644932046,
11.1407696282762,11.1856556229305,11.2517673867061,11.2919249703653,11.3296047038382,
11.3835863047801,11.6004953681049,11.7249773570164,11.7610876730576,11.7821658752364,
11.8009366502485,11.8356842599261,11.9930366547178,12.1211061577448,12.2074643523629),
 .UNSPECIFIED.) ;
#243=B_SPLINE_CURVE_WITH_KNOTS('',3,(#31002,#31003,#31004,#31005,#31006,
#31007,#31008,#31009,#31010,#31011,#31012,#31013,#31014,#31015,#31016,#31017,
#31018,#31019,#31020,#31021,#31022,#31023,#31024,#31025,#31026,#31027,#31028,
#31029,#31030,#31031,#31032,#31033,#31034,#31035,#31036,#31037,#31038,#31039,
#31040,#31041,#31042,#31043,#31044,#31045,#31046,#31047,#31048,#31049,#31050,
#31051,#31052,#31053,#31054,#31055,#31056,#31057,#31058,#31059,#31060,#31061,
#31062,#31063,#31064,#31065,#31066,#31067,#31068,#31069,#31070,#31071,#31072,
#31073,#31074,#31075,#31076,#31077,#31078,#31079,#31080,#31081,#31082,#31083,
#31084,#31085,#31086,#31087,#31088,#31089,#31090,#31091,#31092,#31093,#31094,
#31095,#31096,#31097,#31098,#31099,#31100,#31101,#31102,#31103,#31104,#31105,
#31106,#31107,#31108,#31109,#31110,#31111,#31112,#31113,#31114,#31115,#31116,
#31117,#31118,#31119,#31120,#31121,#31122,#31123,#31124,#31125,#31126,#31127,
#31128,#31129,#31130,#31131,#31132,#31133,#31134,#31135,#31136,#31137,#31138,
#31139,#31140,#31141,#31142,#31143,#31144,#31145,#31146,#31147,#31148,#31149,
#31150,#31151,#31152,#31153,#31154,#31155,#31156,#31157,#31158,#31159,#31160,
#31161,#31162,#31163,#31164,#31165,#31166,#31167,#31168,#31169,#31170,#31171,
#31172,#31173,#31174,#31175,#31176,#31177,#31178,#31179,#31180,#31181,#31182,
#31183,#31184,#31185,#31186,#31187,#31188,#31189,#31190,#31191,#31192,#31193,
#31194,#31195,#31196,#31197,#31198,#31199,#31200,#31201,#31202,#31203,#31204,
#31205,#31206,#31207,#31208,#31209,#31210,#31211,#31212,#31213,#31214,#31215,
#31216,#31217,#31218,#31219,#31220,#31221,#31222,#31223,#31224,#31225,#31226,
#31227,#31228,#31229,#31230,#31231,#31232,#31233,#31234,#31235,#31236,#31237,
#31238,#31239,#31240,#31241,#31242,#31243,#31244,#31245,#31246,#31247,#31248,
#31249,#31250,#31251,#31252,#31253,#31254,#31255,#31256,#31257,#31258,#31259,
#31260,#31261,#31262,#31263,#31264,#31265,#31266,#31267,#31268,#31269,#31270,
#31271,#31272,#31273,#31274,#31275,#31276,#31277,#31278,#31279,#31280,#31281,
#31282,#31283,#31284,#31285,#31286,#31287,#31288,#31289,#31290,#31291,#31292,
#31293,#31294,#31295,#31296,#31297,#31298,#31299,#31300,#31301,#31302,#31303,
#31304,#31305,#31306,#31307,#31308,#31309,#31310,#31311,#31312,#31313,#31314,
#31315,#31316,#31317,#31318,#31319,#31320,#31321,#31322,#31323,#31324,#31325,
#31326,#31327,#31328,#31329,#31330,#31331,#31332,#31333,#31334,#31335,#31336,
#31337,#31338,#31339,#31340,#31341,#31342,#31343,#31344,#31345,#31346,#31347,
#31348,#31349,#31350,#31351,#31352,#31353,#31354,#31355,#31356,#31357,#31358,
#31359,#31360,#31361,#31362,#31363,#31364,#31365,#31366,#31367,#31368,#31369,
#31370,#31371,#31372,#31373),.UNSPECIFIED.,.F.,.F.,(4,2,2,2,2,2,2,2,2,2,
2,2,2,2,2,2,2,2,2,2,2,2,2,2,2,2,2,2,2,2,2,2,2,2,2,2,2,2,2,2,2,2,2,2,2,2,
2,2,2,2,2,2,2,2,2,2,2,2,2,2,2,2,2,2,2,2,2,2,2,2,2,2,2,2,2,2,2,2,2,2,2,2,
2,2,2,2,2,2,2,2,2,2,2,2,2,2,2,2,2,2,2,2,2,2,2,2,2,2,2,2,2,2,2,2,2,2,2,2,
2,2,2,2,2,2,2,2,2,2,2,2,2,2,2,2,2,2,2,2,2,2,2,2,2,2,2,2,2,2,2,2,2,2,2,2,
2,2,2,2,2,2,2,2,2,2,2,2,2,2,2,2,2,2,2,2,2,2,2,2,2,2,2,2,2,2,2,4),(7.92263036594461E-5,
0.285439410797672,0.325676368230994,0.350060823789353,0.368760547286798,
0.388654969438788,0.417789629828308,0.507173101801483,0.689783397735617,
0.761619798396612,0.806150156115514,0.827146881759627,0.861764633508179,
0.896566139823352,0.954226345151844,1.13569588276715,1.24609044475653,1.29036866305543,
1.32257183830718,1.32300963011027,1.32346132062348,1.3239268511748,1.3244061461291,
1.32489911478138,1.32540565331693,1.32592564675978,1.32613706685496,1.32638366586913,
1.32667045895257,1.32700290726294,1.34528641022483,1.36420141855042,1.39977043093359,
1.51981062658116,1.62960186208969,1.71559627827994,1.7827085910791,1.82304611173117,
1.86106343668104,1.91479418490189,2.13400773413672,2.25704484647675,2.2929952128078,
2.31404178075911,2.3328374434696,2.36772835947233,2.47364901716055,2.50518289537555,
2.64586136325104,2.68932978949199,2.75400507063272,2.7939036207803,2.83172188411034,
2.87776125777176,3.01935189475744,3.07313293165803,3.18418266974929,3.22859936087,
3.26325525692269,3.28405066236122,3.30588196070914,3.34579788186677,3.4662822281287,
3.47076102233836,3.6138137466388,3.65770040213656,3.72280170143627,3.76277694874762,
3.80055202583491,3.85515631618018,4.06586733540959,4.16094638922756,4.20177335680755,
4.23435557358773,4.25477000579239,4.27722637779772,4.32041608244396,4.50351224128716,
4.60756120622037,4.68366923759432,4.7255960500385,4.76307743179355,4.8119789307011,
4.92772763216422,5.10200867745599,5.14179105332943,5.16590172698441,5.20114885299746,
5.22205796169431,5.24097105199415,5.27652947274814,5.39645726740062,5.50594777158999,
5.59216120249817,5.65938958444144,5.69974789728489,5.73775505200043,5.79141963594927,
6.01100098193801,6.1338570920963,6.16978724043466,6.19082978590478,6.20962858270671,
6.24453766784338,6.35070530251803,6.51270087106321,6.61057590871916,6.65588980040333,
6.69306901824452,6.73813895419844,6.83426310658243,7.03479453419374,7.1189348794266,
7.14697721537695,7.16675976898853,7.1914391192938,7.24772529496063,7.50892187453285,
7.58889300767342,7.63147429440938,7.66883179318164,7.71658489294355,7.83401819784822,
8.00940902891725,8.04930912411433,8.07346985049825,8.10876940680438,8.12968861911999,
8.14859240034251,8.18409860511552,8.378267319018,8.48350894297163,8.56017071346663,
8.60219237603552,8.63965275564109,8.68837534228286,8.81611979692329,8.98117508921895,
9.01993874606655,9.06900556021672,9.09251549839319,9.11252513281466,9.14255775762738,
9.25488838855663,9.38151021911214,9.46838523109454,9.53596328585282,9.57638437438618,
9.61436176961882,9.66783051638161,9.88848482264557,10.0108220173771,10.0466941582192,
10.0677252465313,10.0865332200554,10.121495054378,10.2283782003239,10.2589239251033,
10.3995307482353,10.4429863047724,10.5076483007207,10.5475442572115,10.5853635758931,
10.6314086883711,10.7730793282653,10.9235986574593,10.9606072834236,11.0081686762797,
11.0314174879324,11.0515059445415,11.0820875706546,11.1922514526446,11.3574293215483,
11.4263707271137,11.4838971873268,11.5225310618414,11.5572614879215,11.6144595637865,
11.7972060660193,11.9073918645691,11.9516257385787,11.9861775610999,12.0069530834011,
12.0259950927627,12.0622764357232,12.2072718274533),.UNSPECIFIED.) ;
#244=B_SPLINE_CURVE_WITH_KNOTS('',3,(#31378,#31379,#31380,#31381,#31382,
#31383,#31384,#31385,#31386,#31387,#31388,#31389,#31390,#31391,#31392,#31393,
#31394,#31395,#31396,#31397,#31398,#31399,#31400,#31401,#31402,#31403,#31404,
#31405,#31406,#31407,#31408,#31409,#31410,#31411,#31412,#31413,#31414,#31415,
#31416,#31417,#31418,#31419,#31420,#31421,#31422,#31423,#31424,#31425,#31426,
#31427,#31428,#31429,#31430,#31431,#31432,#31433,#31434,#31435,#31436,#31437,
#31438,#31439,#31440,#31441,#31442,#31443,#31444,#31445,#31446,#31447,#31448,
#31449,#31450,#31451,#31452,#31453,#31454,#31455,#31456,#31457,#31458,#31459,
#31460,#31461,#31462,#31463,#31464,#31465,#31466,#31467,#31468,#31469,#31470,
#31471,#31472,#31473,#31474,#31475,#31476,#31477,#31478,#31479,#31480,#31481,
#31482,#31483,#31484,#31485,#31486,#31487,#31488,#31489,#31490,#31491,#31492,
#31493,#31494,#31495,#31496,#31497,#31498,#31499,#31500,#31501,#31502,#31503,
#31504,#31505,#31506,#31507,#31508,#31509,#31510,#31511,#31512,#31513,#31514,
#31515,#31516,#31517,#31518,#31519,#31520,#31521,#31522,#31523,#31524,#31525,
#31526,#31527,#31528,#31529,#31530,#31531,#31532,#31533,#31534,#31535,#31536,
#31537,#31538,#31539,#31540,#31541,#31542,#31543,#31544,#31545,#31546,#31547,
#31548,#31549,#31550,#31551,#31552,#31553,#31554,#31555,#31556,#31557,#31558,
#31559,#31560,#31561,#31562,#31563,#31564,#31565,#31566,#31567,#31568,#31569,
#31570,#31571,#31572,#31573,#31574,#31575,#31576,#31577,#31578,#31579,#31580,
#31581,#31582,#31583,#31584,#31585,#31586,#31587,#31588,#31589,#31590,#31591,
#31592,#31593,#31594,#31595,#31596,#31597,#31598,#31599,#31600,#31601,#31602,
#31603,#31604,#31605,#31606,#31607,#31608,#31609,#31610,#31611,#31612,#31613,
#31614,#31615,#31616,#31617,#31618,#31619,#31620,#31621,#31622,#31623,#31624,
#31625,#31626,#31627,#31628,#31629,#31630,#31631,#31632,#31633,#31634,#31635,
#31636,#31637,#31638,#31639,#31640,#31641,#31642,#31643,#31644,#31645,#31646,
#31647,#31648,#31649,#31650,#31651,#31652,#31653,#31654,#31655,#31656,#31657,
#31658,#31659,#31660,#31661,#31662,#31663,#31664,#31665,#31666,#31667,#31668,
#31669,#31670,#31671,#31672,#31673,#31674,#31675,#31676,#31677,#31678,#31679,
#31680,#31681),.UNSPECIFIED.,.F.,.F.,(4,3,3,3,3,3,3,3,3,3,3,3,3,3,3,3,3,
3,3,3,3,3,3,3,3,3,3,3,3,3,3,3,3,3,3,3,3,3,3,3,3,3,3,3,3,3,3,3,3,3,3,3,3,
3,3,3,3,3,3,3,3,3,3,3,3,3,3,3,3,3,3,3,3,3,3,3,3,3,3,3,3,3,3,3,3,3,3,3,3,
3,3,3,3,3,3,3,3,3,3,3,3,4),(-73.2080292590851,-73.1459143162487,-73.083804333767,
-73.0212287225363,-72.9591134095751,-72.8963076492096,-72.8335018888441,
-72.7711444385968,-72.7088342241839,-72.6465306966311,-72.5842309554224,
-72.5218337882832,-72.4595276561961,-72.3970849715309,-72.3346422868657,
-72.2722848366184,-72.2099746222097,-72.147671094661,-72.0853713534566,
-72.0229741863143,-71.9606680542315,-71.8982253695594,-71.8357826848873,
-71.77342523464,-71.711115020227,-71.6488114926738,-71.5865117514652,-71.5241145843261,
-71.4618084522392,-71.399365767574,-71.3369230829089,-71.2745656326616,
-71.2122554182513,-71.1499518907003,-71.0876521494938,-71.025254982353,
-70.9629488502689,-70.9005061655997,-70.8380634809305,-70.7757060306832,
-70.7133958162715,-70.6510922887201,-70.5887925475126,-70.5263953803724,
-70.4640892482871,-70.4016465636196,-70.3392038789521,-70.2768464287048,
-70.2145362142939,-70.1522326867427,-70.0899329455366,-70.0275357783959,
-69.9652296463107,-69.9027869616422,-69.8403442769738,-69.7779868267265,
-69.7156766123153,-69.6533730847636,-69.5910733435567,-69.5286761764164,
-69.4663700443315,-69.4039273596635,-69.3414846749954,-69.2791272247481,
-69.2168170103367,-69.1545134827852,-69.0922137415786,-69.0298165744382,
-68.9675104423528,-68.9050677576849,-68.842625073017,-68.7802676227697,
-68.7179574083583,-68.6556538808074,-68.5933541396007,-68.5309569724601,
-68.4686508403746,-68.4062081557066,-68.3437654710386,-68.2814080207913,
-68.2190978063795,-68.1567942788276,-68.09449453762,-68.0320973704801,-67.9697912383952,
-67.9073485537277,-67.8449058690602,-67.7825484188129,-67.7202382044018,
-67.6579346768496,-67.5956349356414,-67.5332377685015,-67.4709316364168,
-67.4084889517493,-67.3460462670818,-67.2839762765568,-67.2219166211779,
-67.1598638956407,-67.0978094185812,-67.0357563242646,-66.9736929977926,
-66.9248439817473),.UNSPECIFIED.) ;
#245=B_SPLINE_CURVE_WITH_KNOTS('',3,(#31682,#31683,#31684,#31685,#31686,
#31687,#31688,#31689,#31690,#31691,#31692,#31693,#31694,#31695,#31696,#31697,
#31698,#31699,#31700,#31701,#31702,#31703,#31704,#31705,#31706,#31707,#31708,
#31709,#31710,#31711,#31712,#31713,#31714,#31715,#31716,#31717,#31718,#31719,
#31720,#31721,#31722,#31723,#31724,#31725,#31726,#31727,#31728,#31729,#31730,
#31731,#31732,#31733,#31734,#31735,#31736,#31737,#31738,#31739,#31740,#31741,
#31742,#31743,#31744,#31745,#31746,#31747,#31748,#31749,#31750,#31751,#31752,
#31753,#31754,#31755,#31756,#31757,#31758,#31759,#31760,#31761,#31762,#31763,
#31764,#31765,#31766,#31767,#31768,#31769,#31770,#31771,#31772,#31773,#31774,
#31775,#31776,#31777,#31778,#31779,#31780,#31781,#31782,#31783,#31784,#31785,
#31786,#31787,#31788,#31789,#31790,#31791,#31792,#31793,#31794,#31795,#31796,
#31797,#31798,#31799,#31800,#31801,#31802,#31803,#31804,#31805,#31806,#31807,
#31808,#31809,#31810,#31811,#31812,#31813,#31814,#31815,#31816,#31817,#31818,
#31819,#31820,#31821,#31822,#31823,#31824,#31825,#31826,#31827,#31828,#31829,
#31830,#31831,#31832,#31833,#31834,#31835,#31836,#31837,#31838,#31839,#31840,
#31841,#31842,#31843,#31844,#31845,#31846,#31847,#31848,#31849,#31850,#31851,
#31852,#31853,#31854,#31855,#31856,#31857,#31858,#31859,#31860,#31861,#31862,
#31863,#31864,#31865,#31866,#31867,#31868,#31869,#31870,#31871,#31872,#31873,
#31874,#31875,#31876,#31877,#31878,#31879,#31880,#31881,#31882,#31883,#31884,
#31885,#31886,#31887,#31888,#31889,#31890,#31891,#31892,#31893,#31894,#31895,
#31896,#31897,#31898,#31899,#31900,#31901,#31902,#31903,#31904,#31905,#31906,
#31907,#31908,#31909,#31910,#31911,#31912,#31913,#31914,#31915,#31916,#31917,
#31918,#31919,#31920,#31921,#31922,#31923,#31924,#31925,#31926,#31927,#31928,
#31929,#31930,#31931,#31932,#31933,#31934,#31935,#31936,#31937,#31938,#31939,
#31940,#31941,#31942,#31943,#31944,#31945,#31946,#31947,#31948,#31949,#31950,
#31951,#31952,#31953,#31954,#31955,#31956,#31957,#31958,#31959,#31960,#31961,
#31962,#31963,#31964,#31965,#31966,#31967,#31968,#31969,#31970,#31971,#31972,
#31973,#31974,#31975,#31976,#31977,#31978,#31979,#31980,#31981,#31982,#31983,
#31984,#31985,#31986,#31987,#31988,#31989,#31990,#31991,#31992,#31993,#31994,
#31995,#31996,#31997,#31998,#31999,#32000,#32001,#32002,#32003,#32004,#32005,
#32006,#32007,#32008,#32009,#32010,#32011,#32012,#32013,#32014,#32015,#32016,
#32017,#32018,#32019,#32020,#32021,#32022,#32023,#32024,#32025,#32026,#32027,
#32028,#32029,#32030,#32031,#32032,#32033,#32034,#32035,#32036,#32037,#32038,
#32039,#32040,#32041,#32042,#32043,#32044,#32045,#32046,#32047,#32048,#32049,
#32050,#32051),.UNSPECIFIED.,.F.,.F.,(4,2,2,2,2,2,2,2,2,2,2,2,2,2,2,2,2,
2,2,2,2,2,2,2,2,2,2,2,2,2,2,2,2,2,2,2,2,2,2,2,2,2,2,2,2,2,2,2,2,2,2,2,2,
2,2,2,2,2,2,2,2,2,2,2,2,2,2,2,2,2,2,2,2,2,2,2,2,2,2,2,2,2,2,2,2,2,2,2,2,
2,2,2,2,2,2,2,2,2,2,2,2,2,2,2,2,2,2,2,2,2,2,2,2,2,2,2,2,2,2,2,2,2,2,2,2,
2,2,2,2,2,2,2,2,2,2,2,2,2,2,2,2,2,2,2,2,2,2,2,2,2,2,2,2,2,2,2,2,2,2,2,2,
2,2,2,2,2,2,2,2,2,2,2,2,2,2,2,2,2,2,2,2,2,2,2,4),(12.2072718274533,12.3977497167711,
12.4542601641789,12.492340157742,12.5318281998818,12.5942206404381,12.6354797337976,
12.8330913798462,12.9304389954081,12.9601760835259,12.9801458178146,13.0038060585305,
13.0537550543852,13.0935674945261,13.2681298160631,13.3865875607127,13.4343428119366,
13.4717005257048,13.5142804954632,13.5942438157573,13.8561141395262,13.906722921667,
13.9307678299505,13.9506034283396,13.9749116314301,14.0288133857135,14.1132843107081,
14.345980084663,14.3930210529472,14.4310628889466,14.4706052945446,14.5333012545417,
14.5748511353524,14.7051500962768,14.7469377194739,14.768758474474,14.8689820838145,
14.8986805456691,14.9186451485686,14.9423254319356,14.9923932900624,15.0323482812315,
15.2082579481845,15.2554131694779,15.3399116421206,15.3832324915028,15.4204957737368,
15.467922240178,15.5828877701329,15.815116838862,15.8573604795725,15.8796388035456,
15.9001484229358,15.9332670072165,16.0831770575733,16.2749317396433,16.3313129842835,
16.369371793282,16.4088898500396,16.4714498617669,16.549106901566,16.7789207200217,
16.8245616193987,16.8474685011202,16.8676799806685,16.8990561683132,16.9195755448626,
16.9793178593975,17.1984043708695,17.2800333779453,17.3228892807793,17.3564722659033,
17.4025394623861,17.5060744367043,17.6892054292528,17.7780476655874,17.807109446059,
17.8269953075165,17.8510269814867,17.9032107517015,17.9834956909541,18.2269717953508,
18.2724926696637,18.3101991603103,18.3503025013178,18.4161155464988,18.4996820679835,
18.6125184861236,18.6843704966532,18.7523022276742,18.7765449539403,18.7964094801789,
18.8205513045987,18.8734142187059,18.9553366890172,19.1958506793755,19.2414905949628,
19.279222241373,19.3192767259005,19.3848195962123,19.4291419028953,19.5747160340016,
19.6135170462254,19.707978132078,19.7411832809283,19.7596914432612,19.7811542150584,
19.8191975518346,19.8697330190019,20.0137621064173,20.1632170884288,20.2095196347705,
20.247395277952,20.2871945323048,20.3513208955801,20.3942535155513,20.531953412779,
20.6724696534244,20.7081667428062,20.7271043221114,20.7479863724557,20.7830944133269,
20.9599919924138,21.0376929821642,21.1425816252534,21.1900246095976,21.2272889499342,
21.2705980495207,21.3550237204654,21.4782143097203,21.6443564483648,21.6785979390088,
21.6972809236204,21.7184752379256,21.7551726872479,21.8032377402809,21.9329033386672,
21.9602240229548,22.1031732687599,22.1488840141077,22.1866308273941,22.2266568842223,
22.2920419213765,22.3362083313097,22.4808751952126,22.5437265258313,22.625444393919,
22.6510891019342,22.6710135673878,22.6940667156398,22.7405233697114,22.7762714348927,
22.9172470237126,22.9361918323935,23.0744560047225,23.1238018227702,23.1613365295802,
23.1999601848588,23.2691837177158,23.3602921810928,23.4629378081837,23.5046776914714,
23.5932273095291,23.6222480465391,23.642128924908,23.6590527974992,23.660973926847,
23.6630216957833,23.6652412710208,23.6676848669956,23.6682091844828,23.6688922373065,
23.6697911582846,23.6709889349966,23.6726089671795,23.6748389801266,23.7445416256931,
23.8828363914229,23.946311966082,24.0502159880961,24.0976017790855,24.1348620029846,
24.1699782283782,24.2130079824613,24.4145864482893),.UNSPECIFIED.) ;
#246=B_SPLINE_CURVE_WITH_KNOTS('',3,(#32056,#32057,#32058,#32059,#32060,
#32061,#32062,#32063,#32064,#32065,#32066,#32067,#32068,#32069,#32070,#32071,
#32072,#32073,#32074,#32075,#32076,#32077,#32078,#32079,#32080,#32081,#32082,
#32083,#32084,#32085,#32086,#32087,#32088,#32089,#32090,#32091,#32092,#32093,
#32094,#32095,#32096,#32097,#32098,#32099,#32100,#32101,#32102,#32103,#32104,
#32105,#32106,#32107,#32108,#32109,#32110,#32111,#32112,#32113,#32114,#32115,
#32116,#32117,#32118,#32119,#32120,#32121,#32122,#32123,#32124,#32125,#32126,
#32127,#32128,#32129,#32130,#32131,#32132,#32133,#32134,#32135,#32136,#32137,
#32138,#32139,#32140,#32141,#32142,#32143,#32144,#32145,#32146,#32147,#32148,
#32149,#32150,#32151,#32152,#32153,#32154,#32155,#32156,#32157,#32158,#32159,
#32160,#32161,#32162,#32163,#32164,#32165,#32166,#32167,#32168,#32169,#32170,
#32171,#32172,#32173,#32174,#32175,#32176,#32177,#32178,#32179,#32180,#32181,
#32182,#32183,#32184,#32185,#32186,#32187,#32188,#32189,#32190,#32191,#32192,
#32193,#32194,#32195,#32196,#32197,#32198,#32199,#32200,#32201,#32202,#32203,
#32204,#32205,#32206,#32207,#32208,#32209,#32210,#32211,#32212,#32213,#32214,
#32215,#32216,#32217,#32218,#32219,#32220,#32221,#32222,#32223,#32224,#32225,
#32226,#32227,#32228,#32229,#32230,#32231,#32232,#32233,#32234,#32235,#32236,
#32237,#32238,#32239,#32240,#32241,#32242,#32243,#32244,#32245,#32246,#32247,
#32248,#32249,#32250,#32251,#32252,#32253,#32254,#32255,#32256,#32257,#32258,
#32259,#32260,#32261,#32262,#32263,#32264,#32265,#32266,#32267,#32268,#32269,
#32270,#32271,#32272,#32273,#32274,#32275,#32276,#32277,#32278,#32279,#32280,
#32281,#32282,#32283,#32284,#32285,#32286,#32287,#32288,#32289,#32290,#32291,
#32292,#32293,#32294,#32295,#32296,#32297,#32298,#32299,#32300,#32301,#32302,
#32303,#32304,#32305,#32306,#32307,#32308,#32309,#32310,#32311,#32312,#32313,
#32314,#32315,#32316,#32317,#32318,#32319,#32320,#32321,#32322,#32323,#32324,
#32325,#32326,#32327,#32328,#32329,#32330,#32331,#32332,#32333,#32334,#32335,
#32336,#32337,#32338,#32339,#32340,#32341,#32342,#32343,#32344,#32345,#32346,
#32347,#32348,#32349,#32350,#32351,#32352,#32353,#32354,#32355,#32356,#32357,
#32358,#32359),.UNSPECIFIED.,.F.,.F.,(4,3,3,3,3,3,3,3,3,3,3,3,3,3,3,3,3,
3,3,3,3,3,3,3,3,3,3,3,3,3,3,3,3,3,3,3,3,3,3,3,3,3,3,3,3,3,3,3,3,3,3,3,3,
3,3,3,3,3,3,3,3,3,3,3,3,3,3,3,3,3,3,3,3,3,3,3,3,3,3,3,3,3,3,3,3,3,3,3,3,
3,3,3,3,3,3,3,3,3,3,3,3,4),(-79.4912145612532,-79.4268580816011,-79.3624817745964,
-79.3186767145631,-79.2563192643158,-79.194009049235,-79.1317055211391,
-79.0694057795137,-79.0070086127814,-78.9447024805901,-78.8822597965874,
-78.8198171125847,-78.7574596623374,-78.6951494239939,-78.6328458722586,
-78.5705461066667,-78.5081489576516,-78.445842800927,-78.3834001557667,
-78.3209575106063,-78.258600060359,-78.1962898663862,-78.1339863594574,
-78.0716866390136,-78.0092894564172,-77.9469833452384,-77.8845406269331,
-77.8220979086279,-77.7597404583806,-77.6974302322208,-77.6351266928235,
-77.5728269396977,-77.5104297814357,-77.44812363737,-77.3856809720097,-77.3232383066495,
-77.2608808564022,-77.1985706471886,-77.1362671248746,-77.0739673889335,
-77.0115702178679,-76.9492640910678,-76.8868213978695,-76.8243787046712,
-76.7620212544239,-76.6997110383436,-76.6374075091123,-76.5751077662177,
-76.5127106003365,-76.4504044665619,-76.3879617846274,-76.3255191026928,
-76.2631616524455,-76.2008514382385,-76.1385479108915,-76.0762481698883,
-76.0138510025948,-75.9515448707106,-75.8891021857125,-75.8266595007144,
-75.7643020504671,-75.7019918362715,-75.6396883089383,-75.5773885679514,
-75.5149914006475,-75.4526852687853,-75.3902425837607,-75.327799898736,
-75.2654424484887,-75.2031322338472,-75.1408287060635,-75.0785289646224,
-75.0161317976562,-74.9538256653351,-74.8913829810463,-74.8289402967576,
-74.7665828465103,-74.704272632244,-74.641969104839,-74.5796693637792,-74.5172721965292,
-74.454966064592,-74.3925233796856,-74.3300806947792,-74.2677232445319,
-74.2054130300514,-74.1431095024306,-74.0808097611533,-74.0184125940652,
-73.9561064619095,-73.8936637773551,-73.8312210928008,-73.7688636425535,
-73.7065534281674,-73.6442499006414,-73.5819501594596,-73.5195529923003,
-73.4572468602403,-73.3948041755314,-73.3323614908225,-73.2668472050594,
-73.2080292600168),.UNSPECIFIED.) ;
#247=B_SPLINE_CURVE_WITH_KNOTS('',3,(#32360,#32361,#32362,#32363,#32364,
#32365,#32366,#32367,#32368,#32369,#32370,#32371,#32372,#32373,#32374,#32375,
#32376,#32377,#32378,#32379,#32380,#32381,#32382,#32383,#32384,#32385,#32386,
#32387,#32388,#32389,#32390,#32391,#32392,#32393,#32394,#32395,#32396,#32397,
#32398,#32399,#32400,#32401,#32402,#32403,#32404,#32405,#32406,#32407,#32408,
#32409,#32410,#32411,#32412,#32413,#32414,#32415,#32416,#32417,#32418,#32419,
#32420,#32421,#32422,#32423,#32424,#32425,#32426,#32427,#32428,#32429,#32430,
#32431,#32432,#32433,#32434,#32435,#32436,#32437,#32438,#32439,#32440,#32441,
#32442,#32443,#32444,#32445,#32446,#32447,#32448,#32449,#32450,#32451,#32452,
#32453,#32454,#32455,#32456,#32457,#32458,#32459,#32460,#32461,#32462,#32463,
#32464,#32465,#32466,#32467,#32468,#32469,#32470,#32471,#32472,#32473,#32474,
#32475,#32476,#32477,#32478,#32479,#32480,#32481,#32482,#32483,#32484,#32485,
#32486,#32487,#32488,#32489,#32490,#32491,#32492,#32493,#32494,#32495,#32496,
#32497,#32498,#32499,#32500,#32501,#32502,#32503,#32504,#32505,#32506,#32507,
#32508,#32509,#32510,#32511,#32512,#32513,#32514,#32515,#32516,#32517,#32518,
#32519,#32520,#32521,#32522,#32523,#32524,#32525,#32526,#32527,#32528,#32529,
#32530,#32531,#32532,#32533,#32534,#32535,#32536,#32537,#32538,#32539,#32540,
#32541,#32542,#32543,#32544,#32545,#32546,#32547,#32548,#32549,#32550,#32551,
#32552,#32553,#32554,#32555,#32556,#32557,#32558,#32559,#32560,#32561,#32562,
#32563,#32564,#32565,#32566,#32567,#32568,#32569,#32570,#32571,#32572,#32573,
#32574,#32575,#32576,#32577,#32578,#32579,#32580,#32581,#32582,#32583,#32584,
#32585,#32586,#32587,#32588,#32589,#32590,#32591,#32592,#32593,#32594,#32595,
#32596,#32597,#32598,#32599,#32600,#32601,#32602,#32603,#32604,#32605,#32606,
#32607,#32608,#32609,#32610,#32611,#32612,#32613,#32614,#32615,#32616,#32617,
#32618,#32619,#32620,#32621,#32622,#32623,#32624,#32625,#32626,#32627,#32628,
#32629,#32630,#32631,#32632,#32633,#32634,#32635,#32636,#32637,#32638,#32639,
#32640,#32641,#32642,#32643,#32644,#32645,#32646,#32647,#32648,#32649,#32650,
#32651,#32652,#32653,#32654,#32655,#32656,#32657,#32658,#32659,#32660,#32661,
#32662,#32663,#32664,#32665,#32666,#32667,#32668,#32669,#32670,#32671,#32672,
#32673,#32674,#32675,#32676,#32677,#32678,#32679,#32680,#32681,#32682,#32683,
#32684,#32685,#32686,#32687,#32688,#32689,#32690,#32691,#32692,#32693,#32694,
#32695,#32696,#32697,#32698,#32699,#32700,#32701,#32702,#32703,#32704,#32705,
#32706,#32707,#32708,#32709,#32710,#32711,#32712,#32713,#32714,#32715,#32716,
#32717,#32718,#32719,#32720,#32721,#32722,#32723,#32724,#32725,#32726,#32727,
#32728,#32729,#32730,#32731,#32732,#32733,#32734,#32735,#32736,#32737,#32738,
#32739,#32740,#32741,#32742,#32743),.UNSPECIFIED.,.F.,.F.,(4,2,2,2,2,2,
2,2,2,2,2,2,2,2,2,2,2,2,2,2,2,2,2,2,2,2,2,2,2,2,2,2,2,2,2,2,2,2,2,2,2,2,
2,2,2,2,2,2,2,2,2,2,2,2,2,2,2,2,2,2,2,2,2,2,2,2,2,2,2,2,2,2,2,2,2,2,2,2,
2,2,2,2,2,2,2,2,2,2,2,2,2,2,2,2,2,2,2,2,2,2,2,2,2,2,2,2,2,2,2,2,2,2,2,2,
2,2,2,2,2,2,2,2,2,2,2,2,2,2,2,2,2,2,2,2,2,2,2,2,2,2,2,2,2,2,2,2,2,2,2,2,
2,2,2,2,2,2,2,2,2,2,2,2,2,2,2,2,2,2,2,2,2,2,2,2,2,2,2,2,2,2,2,2,2,2,2,2,
2,2,2,2,2,4),(5.2387363187429E-5,0.1405308078795,0.165124190737373,0.183885119107637,
0.203738040115377,0.232506750144318,0.319290774131082,0.371642125817686,
0.519414229923385,0.60985617636824,0.636520703677487,0.671400516008268,
0.709276099436823,0.75557745570598,0.902321740580871,0.949174461745862,
1.06096782730526,1.12291765042536,1.14829962710164,1.14917706987226,1.14954701645056,
1.15025320562604,1.15158559594079,1.15271509751055,1.16637849569789,1.19067113203141,
1.2444751441704,1.42807348775699,1.52295990086329,1.57504189836203,1.57808789692835,
1.58078667485465,1.58320080112759,1.58538064790428,1.58736709006859,1.5891936032842,
1.59088789389522,1.59247317004041,1.59396914073202,1.5953928107427,1.59675912418272,
1.5980814985439,1.59937228309313,1.60064317046535,1.60190558840903,1.63800769101212,
1.67595402831942,1.72921571476367,1.95102839234152,2.07280111762692,2.10860996914406,
2.12962862765459,2.14844680189936,2.18346689838626,2.29114286070091,2.45192942298535,
2.4987081052802,2.56670309223246,2.60719912377983,2.64514246625316,2.69838384251997,
2.92031401043612,3.04202877521207,3.07783113743871,3.09884853868992,3.11766779297178,
3.15269396899841,3.26045260830269,3.4211734331033,3.46794215432795,3.53592735543642,
3.57642166201242,3.61436584012224,3.66761258984043,3.88951236659545,4.01124248192391,
4.04704659527464,4.0680643562044,4.08688335485402,4.12190798922611,4.22964512057845,
4.39038340247107,4.43715480200092,4.50514266638918,4.54563748378574,4.58358149785494,
4.63682691619637,4.8587349765706,4.98046124868621,5.01626495545068,5.03728265270326,
5.05610174569895,5.0911268348381,5.19886975695654,5.35960369772108,5.40637446330416,
5.47436172849374,5.51485647088167,5.5528005831335,5.60604642787711,5.86649630065179,
5.93270562666728,5.97864667804191,6.00160770838509,6.0215651460436,6.05258644346674,
6.16219854515578,6.2888140889046,6.37603201315851,6.44379098055487,6.48424491503088,
6.52220786735582,6.57557823168696,6.69375388075133,6.85842528766969,6.89714530466782,
6.9461753718782,6.96967923000966,6.98969095468523,7.01973698793249,7.13275354873733,
7.25938679694259,7.34589523015528,7.41328000525393,7.45366675955542,7.49166104476944,
7.53676175779244,7.6753807065217,7.70864742204927,7.83836787042646,7.88644321797574,
7.92314659309218,7.9443423614454,7.96302496087448,7.99726278780776,8.16345188463413,
8.28662582603297,8.3710454478524,8.41435417208961,8.45161934510122,8.49906496438502,
8.60403012089681,8.68165096613729,8.85855072499019,8.89365876266852,8.91454108634465,
8.93347914361499,8.96917759230719,9.10970932898925,9.2474057180307,9.29033812857189,
9.35446460887873,9.39426442675673,9.43214090035472,9.47844483613853,9.64443274742685,
9.80554922683034,9.85403831555512,9.87744897776189,9.89748754233686,9.92772462730858,
10.0376180736525,10.1732045969089,10.232623032307,10.3122293422575,10.3547501960325,
10.3921181337826,10.4399718695478,10.5584051231605,10.732774186249,10.7725662042014,
10.8224984500119,10.8461561121503,10.8661269329768,10.8958702435779,10.994578182696,
11.0460476076368,11.1850829479737,11.2282576846174,11.2926328486577,11.3324776536624,
11.3703277908964,11.4165113183186,11.5825345314837,11.7408001323303,11.7913812512808,
11.8151482008142,11.835092272962,11.8598176811538,11.9309094264544,12.1305249554991,
12.2072423730149),.UNSPECIFIED.) ;
#248=B_SPLINE_CURVE_WITH_KNOTS('',3,(#32749,#32750,#32751,#32752,#32753,
#32754,#32755,#32756,#32757,#32758,#32759,#32760,#32761,#32762,#32763,#32764,
#32765,#32766,#32767,#32768,#32769,#32770,#32771,#32772,#32773,#32774,#32775,
#32776,#32777,#32778,#32779,#32780,#32781,#32782,#32783,#32784,#32785,#32786,
#32787,#32788,#32789,#32790,#32791,#32792,#32793,#32794,#32795,#32796,#32797,
#32798),.UNSPECIFIED.,.F.,.F.,(4,2,2,2,2,2,2,2,2,2,2,2,2,2,2,2,2,2,2,2,
2,2,2,2,4),(41.7287185600906,41.8375642754602,41.9723397523482,42.0760090490107,
42.223976254466,42.4899520935777,42.6571500039819,42.8888759482191,43.0565538258593,
43.1530925035041,43.4139782595738,43.6194950036453,43.7994553691564,44.0331432752365,
44.1674373114751,44.271451812564,44.4207260572351,44.6841181869952,44.8508350319949,
45.0843043610434,45.2522594766109,45.3495974165661,45.7530389442282,45.906737536888,
46.2267394719888),.UNSPECIFIED.) ;
#249=B_SPLINE_CURVE_WITH_KNOTS('',3,(#32801,#32802,#32803,#32804,#32805,
#32806,#32807,#32808,#32809,#32810,#32811,#32812,#32813,#32814,#32815,#32816,
#32817,#32818,#32819,#32820,#32821,#32822,#32823,#32824,#32825,#32826,#32827,
#32828,#32829,#32830,#32831,#32832),.UNSPECIFIED.,.F.,.F.,(4,2,2,2,2,2,
2,2,2,2,2,2,2,2,2,4),(0.000341622627806292,0.0673400657444466,0.227847209082467,
0.411559779210653,0.57815132892849,0.812417356253106,1.04496426355356,1.13432835898471,
1.33790194751096,1.52715641261998,1.69498193634874,1.96835421119834,2.11155443311271,
2.21386703158126,2.42160026776052,2.45788151536469),.UNSPECIFIED.) ;
#250=B_SPLINE_CURVE_WITH_KNOTS('',3,(#32837,#32838,#32839,#32840,#32841,
#32842,#32843,#32844,#32845,#32846,#32847,#32848,#32849,#32850,#32851,#32852,
#32853,#32854,#32855,#32856,#32857,#32858,#32859,#32860,#32861,#32862,#32863,
#32864,#32865,#32866,#32867,#32868,#32869,#32870,#32871,#32872,#32873,#32874,
#32875,#32876,#32877,#32878,#32879,#32880,#32881,#32882,#32883,#32884,#32885,
#32886,#32887,#32888,#32889,#32890,#32891,#32892,#32893,#32894,#32895,#32896,
#32897,#32898,#32899,#32900,#32901,#32902,#32903,#32904,#32905,#32906,#32907,
#32908,#32909,#32910,#32911,#32912,#32913,#32914,#32915,#32916,#32917,#32918,
#32919,#32920,#32921,#32922,#32923,#32924,#32925,#32926,#32927,#32928,#32929,
#32930,#32931,#32932,#32933,#32934,#32935,#32936,#32937,#32938,#32939,#32940,
#32941,#32942,#32943,#32944,#32945,#32946,#32947,#32948,#32949,#32950,#32951,
#32952,#32953,#32954,#32955,#32956,#32957,#32958,#32959,#32960,#32961,#32962,
#32963,#32964,#32965,#32966,#32967,#32968,#32969,#32970,#32971,#32972,#32973,
#32974,#32975,#32976,#32977,#32978,#32979,#32980,#32981,#32982,#32983,#32984,
#32985,#32986,#32987,#32988,#32989,#32990),.UNSPECIFIED.,.F.,.F.,(4,2,2,
2,2,2,2,2,2,2,2,2,2,2,2,2,2,2,2,2,2,2,2,2,2,2,2,2,2,2,2,2,2,2,2,2,2,2,2,
2,2,2,2,2,2,2,2,2,2,2,2,2,2,2,2,2,2,2,2,2,2,2,2,2,2,2,2,2,2,2,2,2,2,2,2,
2,4),(27.8190516686995,28.0540235284573,28.2596408606393,28.4393565434381,
28.6723158521103,28.8069846106989,28.9108641731384,29.0595232512103,29.3239631514734,
29.4910804091608,29.7230468328308,29.8906690727476,29.9870524844356,30.2446291280341,
30.4523398010245,30.6312239858078,30.8610367252987,31.0025169158246,31.1075312692734,
31.2598656914219,31.5169605627561,31.6838216517124,31.9173531199209,32.0850718077781,
32.1815366645503,32.4423589581098,32.6479885134352,32.8277093378174,33.0606711957569,
33.1953481304821,33.299225384594,33.4478701785114,33.7123598734217,33.8794843925669,
34.1114512397397,34.2790790990271,34.375465620232,34.633051245024,34.840771283573,
35.0196619820374,35.2494823254115,35.3909693236478,35.4959885973176,35.6483316549986,
35.9054290247319,36.0722964432488,36.3058352920589,36.4735590354038,36.570023962846,
36.8308511488704,37.0364974251052,37.2162166432378,37.4491597061846,37.5838559375489,
37.687721235687,37.8363163400969,38.1009267038591,38.2680694397395,38.4999965555923,
38.6676240359239,38.7639977290439,39.0215672768671,39.2293360539831,39.4081912845709,
39.637886369621,39.7795604418841,39.8845711602258,40.0368694462086,40.294084744372,
40.4609885606339,40.69445452348,40.8621804866196,40.958636438836,41.2194417914166,
41.4251129111561,41.6047817746195,41.7287185600906),.UNSPECIFIED.) ;
#251=B_SPLINE_CURVE_WITH_KNOTS('',3,(#32991,#32992,#32993,#32994,#32995,
#32996,#32997,#32998,#32999,#33000,#33001,#33002,#33003,#33004,#33005,#33006,
#33007,#33008,#33009,#33010,#33011,#33012,#33013,#33014,#33015,#33016,#33017,
#33018,#33019,#33020,#33021,#33022,#33023,#33024,#33025,#33026,#33027,#33028,
#33029,#33030,#33031,#33032,#33033,#33034,#33035,#33036,#33037,#33038,#33039,
#33040,#33041,#33042,#33043,#33044,#33045,#33046,#33047,#33048,#33049,#33050,
#33051,#33052,#33053,#33054,#33055,#33056,#33057,#33058,#33059,#33060,#33061,
#33062,#33063,#33064,#33065,#33066,#33067,#33068,#33069,#33070,#33071,#33072,
#33073,#33074,#33075,#33076,#33077,#33078,#33079,#33080,#33081,#33082,#33083,
#33084,#33085,#33086,#33087,#33088,#33089,#33090,#33091,#33092,#33093,#33094,
#33095,#33096,#33097,#33098,#33099,#33100,#33101,#33102,#33103,#33104,#33105,
#33106,#33107,#33108,#33109,#33110,#33111,#33112,#33113,#33114,#33115,#33116,
#33117,#33118,#33119,#33120,#33121,#33122,#33123,#33124,#33125,#33126,#33127,
#33128,#33129,#33130,#33131,#33132,#33133,#33134,#33135,#33136,#33137,#33138,
#33139,#33140,#33141,#33142),.UNSPECIFIED.,.F.,.F.,(4,2,2,2,2,2,2,2,2,2,
2,2,2,2,2,2,2,2,2,2,2,2,2,2,2,2,2,2,2,2,2,2,2,2,2,2,2,2,2,2,2,2,2,2,2,2,
2,2,2,2,2,2,2,2,2,2,2,2,2,2,2,2,2,2,2,2,2,2,2,2,2,2,2,2,2,4),(2.45788151536469,
2.61572539621936,2.78598388195183,3.08078171023571,3.21465083221518,3.31432199203162,
3.46437731498878,3.68336366443902,3.85866608787174,4.06937792176419,4.32664895588177,
4.42141259903627,4.58806490653788,4.81302279923895,4.98186528234662,5.2643125384097,
5.40439542228602,5.5058086928236,5.63875899112841,5.86989141345836,6.04899095963599,
6.25466890087166,6.51329933433767,6.61027514846681,6.79807166592806,6.99695763716408,
7.16745943789951,7.47298648500569,7.60501576704184,7.70392271308596,7.92851927930397,
8.18428585977036,8.35194201046475,8.58095157831059,8.74838260263357,8.84457212200991,
9.10183145747964,9.31016312720026,9.48877639729143,9.71759798271826,9.8605031233545,
9.96525293206253,10.1167206115351,10.3755787449451,10.5425322324869,10.7756652500631,
10.9433779405392,11.0398442315285,11.3006610830669,11.506319792173,11.6860162797535,
11.9188817453385,12.0536204870947,12.157383004324,12.3056508006402,12.5709461774572,
12.7381165289833,12.9699010332766,13.1375293398637,13.2339189450469,13.4915109933954,
13.6992538133391,13.8781451816648,14.1079472058251,14.249486161008,14.3544968433405,
14.5068036390699,14.76400349011,14.9308824549095,15.1644181044631,15.332151221201,
15.428624657939,15.6894701986197,15.8951196283019,16.0475649733886,16.3682710977173),
 .UNSPECIFIED.) ;
#252=B_SPLINE_CURVE_WITH_KNOTS('',3,(#33147,#33148,#33149,#33150,#33151,
#33152,#33153,#33154,#33155,#33156,#33157,#33158,#33159,#33160,#33161,#33162,
#33163,#33164,#33165,#33166,#33167,#33168,#33169,#33170,#33171,#33172,#33173,
#33174,#33175,#33176,#33177,#33178,#33179,#33180,#33181,#33182,#33183,#33184,
#33185,#33186,#33187,#33188,#33189,#33190,#33191,#33192,#33193,#33194,#33195,
#33196,#33197,#33198,#33199,#33200,#33201,#33202,#33203,#33204,#33205,#33206,
#33207,#33208,#33209,#33210,#33211,#33212,#33213,#33214,#33215,#33216,#33217,
#33218,#33219,#33220,#33221,#33222,#33223,#33224,#33225,#33226,#33227,#33228,
#33229,#33230,#33231,#33232,#33233,#33234,#33235,#33236,#33237,#33238,#33239,
#33240,#33241,#33242,#33243,#33244,#33245,#33246,#33247,#33248,#33249,#33250,
#33251,#33252,#33253,#33254,#33255,#33256,#33257,#33258,#33259,#33260,#33261,
#33262,#33263,#33264,#33265,#33266,#33267,#33268,#33269,#33270,#33271,#33272,
#33273,#33274,#33275,#33276,#33277,#33278,#33279,#33280,#33281,#33282,#33283,
#33284,#33285,#33286,#33287,#33288,#33289,#33290,#33291,#33292,#33293,#33294,
#33295,#33296,#33297,#33298,#33299,#33300,#33301,#33302),.UNSPECIFIED.,
 .F.,.F.,(4,2,2,2,2,2,2,2,2,2,2,2,2,2,2,2,2,2,2,2,2,2,2,2,2,2,2,2,2,2,2,
2,2,2,2,2,2,2,2,2,2,2,2,2,2,2,2,2,2,2,2,2,2,2,2,2,2,2,2,2,2,2,2,2,2,2,2,
2,2,2,2,2,2,2,2,2,2,4),(13.9103642396951,14.059290140731,14.3237983625056,
14.4724210040941,14.5762901521091,14.7109677686707,14.943922753552,15.123638578108,
15.329262085377,15.5900705656506,15.6865317966044,15.8542477597018,16.0877656548719,
16.2546245954422,16.511761847043,16.6640612199289,16.7690634207516,16.9105862528965,
17.1403657262307,17.3192378820909,17.5269617415358,17.7845148316813,17.8808886684624,
18.048500856383,18.2803347085067,18.4474698768279,18.7124781184351,18.8608450506072,
18.9646331944916,19.0993477918314,19.3322130954862,19.511900790291,19.7175675247081,
19.978338496364,20.0747801450231,20.242471329193,20.4756670603556,20.6425710537004,
20.9012441620136,21.0527546018228,21.1575112070697,21.3003433500153,21.5291973969586,
21.7078186505762,21.9161865574636,22.1733999212904,22.2695732864486,22.4369325533377,
22.6649689996637,22.8327644295761,23.1136426005817,23.3162890235833,23.4164490753815,
23.5528962226204,23.8237852586347,23.9883724044378,24.0776389286475,24.4097814047875,
24.5080062088504,24.6377712884637,24.9354426049739,25.1024882127116,25.3348355091553,
25.5024751812084,25.598874840555,25.8564748147422,26.0641135164308,26.2430155267256,
26.4729116887741,26.6142560450411,26.7192918204235,26.871702545449,27.1286270367516,
27.2954768834071,27.529031415055,27.6967457248573,27.7932084143236,27.8190516686995),
 .UNSPECIFIED.) ;
#253=B_SPLINE_CURVE_WITH_KNOTS('',3,(#33303,#33304,#33305,#33306,#33307,
#33308,#33309,#33310,#33311,#33312,#33313,#33314,#33315,#33316,#33317,#33318,
#33319,#33320,#33321,#33322,#33323,#33324,#33325,#33326,#33327,#33328,#33329,
#33330,#33331,#33332,#33333,#33334,#33335,#33336,#33337,#33338,#33339,#33340,
#33341,#33342,#33343,#33344,#33345,#33346,#33347,#33348,#33349,#33350,#33351,
#33352,#33353,#33354,#33355,#33356,#33357,#33358,#33359,#33360,#33361,#33362,
#33363,#33364,#33365,#33366,#33367,#33368,#33369,#33370,#33371,#33372,#33373,
#33374,#33375,#33376,#33377,#33378,#33379,#33380,#33381,#33382,#33383,#33384,
#33385,#33386,#33387,#33388,#33389,#33390,#33391,#33392,#33393,#33394,#33395,
#33396,#33397,#33398,#33399,#33400,#33401,#33402,#33403,#33404,#33405,#33406,
#33407,#33408,#33409,#33410,#33411,#33412,#33413,#33414,#33415,#33416,#33417,
#33418,#33419,#33420,#33421,#33422,#33423,#33424,#33425,#33426,#33427,#33428,
#33429,#33430,#33431,#33432,#33433,#33434,#33435,#33436,#33437,#33438,#33439,
#33440,#33441,#33442,#33443,#33444,#33445,#33446,#33447,#33448,#33449,#33450,
#33451,#33452,#33453,#33454,#33455,#33456,#33457,#33458),.UNSPECIFIED.,
 .F.,.F.,(4,2,2,2,2,2,2,2,2,2,2,2,2,2,2,2,2,2,2,2,2,2,2,2,2,2,2,2,2,2,2,
2,2,2,2,2,2,2,2,2,2,2,2,2,2,2,2,2,2,2,2,2,2,2,2,2,2,2,2,2,2,2,2,2,2,2,2,
2,2,2,2,2,2,2,2,2,2,4),(8.88234718024114E-5,0.0601731981236326,0.110544207433153,
0.280019453746977,0.526557105931961,0.686420100604339,0.94582691662437,
1.0970123777365,1.2016778533486,1.34515029285172,1.573614889418,1.75215096620334,
1.96086205048697,2.21796096889079,2.31405837721316,2.48132234554296,2.71655350383365,
2.88303392076658,3.12529198286448,3.28553078281349,3.39298102298311,3.53575118406741,
3.76636756107163,3.94547424543211,4.15265776878262,4.41052553945569,4.50708440246902,
4.6749158123924,4.91021311217619,5.07680440524432,5.32415911551499,5.48160075826832,
5.58819192173581,5.73025418571335,5.96076037630328,6.13983557684914,6.34708723007708,
6.60491304823191,6.70144736191669,6.86925036137248,7.10409881782883,7.27075703608349,
7.52082435426871,7.67681151042562,7.78295420614849,7.92462507781732,8.15507438766519,
8.33413226772008,8.54141594843493,8.79921842941794,8.89573962148368,9.06352678642508,
9.29814912360071,9.46483942112775,9.71618375185056,9.87149161696981,9.97742405377179,
10.1189058542712,10.3493268332367,10.5283749724368,10.7356711879939,10.9934603611286,
11.0899745710014,11.257752759487,11.4922692505847,11.6589725815367,11.910884678648,
12.0658891807724,12.1717270734666,12.3052477517957,12.5402382400976,12.7204909057877,
12.9248764487335,13.1863693694132,13.2832324775336,13.4935240406713,13.7449391001076,
13.9098688392401),.UNSPECIFIED.) ;
#254=B_SPLINE_CURVE_WITH_KNOTS('',3,(#33463,#33464,#33465,#33466,#33467,
#33468,#33469,#33470,#33471,#33472,#33473,#33474,#33475,#33476,#33477,#33478,
#33479,#33480,#33481,#33482,#33483,#33484,#33485,#33486,#33487,#33488,#33489,
#33490,#33491,#33492,#33493,#33494,#33495,#33496,#33497,#33498,#33499,#33500,
#33501,#33502,#33503,#33504,#33505,#33506,#33507,#33508,#33509,#33510,#33511,
#33512,#33513,#33514,#33515,#33516,#33517,#33518,#33519,#33520,#33521,#33522,
#33523,#33524,#33525,#33526,#33527,#33528,#33529,#33530,#33531,#33532,#33533,
#33534,#33535,#33536,#33537,#33538,#33539,#33540,#33541,#33542,#33543,#33544,
#33545,#33546,#33547,#33548,#33549,#33550,#33551,#33552,#33553,#33554,#33555,
#33556,#33557,#33558,#33559,#33560,#33561,#33562,#33563,#33564,#33565,#33566,
#33567,#33568,#33569,#33570,#33571,#33572,#33573,#33574,#33575,#33576,#33577,
#33578,#33579,#33580,#33581,#33582,#33583,#33584,#33585,#33586,#33587,#33588,
#33589,#33590,#33591,#33592,#33593,#33594,#33595,#33596,#33597,#33598,#33599,
#33600,#33601,#33602,#33603,#33604,#33605,#33606,#33607,#33608,#33609,#33610,
#33611,#33612,#33613,#33614,#33615,#33616,#33617,#33618),.UNSPECIFIED.,
 .F.,.F.,(4,2,2,2,2,2,2,2,2,2,2,2,2,2,2,2,2,2,2,2,2,2,2,2,2,2,2,2,2,2,2,
2,2,2,2,2,2,2,2,2,2,2,2,2,2,2,2,2,2,2,2,2,2,2,2,2,2,2,2,2,2,2,2,2,2,2,2,
2,2,2,2,2,2,2,2,2,2,4),(0.000358256576057275,0.228881878662184,0.285883905039836,
0.392988116828161,0.733898218813132,0.893503238773272,1.15802559996168,
1.3066728138271,1.41055610600951,1.54524765423352,1.77823150756874,1.95796833075757,
2.16361352921898,2.42445237999845,2.52092502082217,2.68866053278439,2.92221456396537,
3.08909080129259,3.34620855128427,3.49854988914389,3.60357160178668,3.7450705602412,
3.97490407266984,4.15380392840545,4.36153168449772,4.61912391930075,4.71551468909243,
4.88315305759357,5.11513116765748,5.28226528591404,5.54677768360417,5.69541928404525,
5.79929865587834,5.93398512494897,6.16696018842095,6.34669023172362,6.55232767503622,
6.81315668675464,6.90962568839495,7.07735487321628,7.31090008676587,7.47777003123677,
7.73487812554999,7.88721369588314,7.99223144067999,8.13372509674368,8.36354991594576,
8.54244301745753,8.75016295551668,9.00774546577109,9.1041325946582,9.27176463391636,
9.5037338916022,9.67086172323557,9.93536460275411,10.084000371521,10.1878757558121,
10.3225571827991,10.5555233861152,10.735246631149,10.9408763640544,11.2016955129446,
11.2981608616184,11.4658837034878,11.6994198261313,11.8662835226502,12.1233833316115,
12.2757124374329,12.3807259994421,12.5222154765817,12.7520308131936,12.9309169506701,
13.1386296230641,13.396202127569,13.4925854459245,13.6602109532714,13.8921680337048,
13.9103642396951),.UNSPECIFIED.) ;
#255=B_SPLINE_CURVE_WITH_KNOTS('',3,(#33619,#33620,#33621,#33622,#33623,
#33624,#33625,#33626,#33627,#33628,#33629,#33630,#33631,#33632,#33633,#33634,
#33635,#33636,#33637,#33638,#33639,#33640,#33641,#33642,#33643,#33644,#33645,
#33646,#33647,#33648,#33649,#33650,#33651,#33652,#33653,#33654,#33655,#33656,
#33657,#33658,#33659,#33660,#33661,#33662,#33663,#33664,#33665,#33666,#33667,
#33668,#33669,#33670,#33671,#33672,#33673,#33674,#33675,#33676,#33677,#33678,
#33679,#33680,#33681,#33682,#33683,#33684,#33685,#33686,#33687,#33688,#33689,
#33690,#33691,#33692,#33693,#33694,#33695,#33696,#33697,#33698,#33699,#33700,
#33701,#33702,#33703,#33704,#33705,#33706,#33707,#33708,#33709,#33710,#33711,
#33712,#33713,#33714,#33715,#33716,#33717,#33718,#33719,#33720,#33721,#33722,
#33723,#33724,#33725,#33726,#33727,#33728,#33729,#33730,#33731,#33732,#33733,
#33734,#33735,#33736,#33737,#33738,#33739,#33740,#33741,#33742,#33743,#33744,
#33745,#33746,#33747,#33748,#33749,#33750,#33751,#33752,#33753,#33754,#33755,
#33756,#33757,#33758,#33759,#33760,#33761,#33762,#33763,#33764,#33765,#33766,
#33767,#33768,#33769,#33770,#33771,#33772),.UNSPECIFIED.,.F.,.F.,(4,2,2,
2,2,2,2,2,2,2,2,2,2,2,2,2,2,2,2,2,2,2,2,2,2,2,2,2,2,2,2,2,2,2,2,2,2,2,2,
2,2,2,2,2,2,2,2,2,2,2,2,2,2,2,2,2,2,2,2,2,2,2,2,2,2,2,2,2,2,2,2,2,2,2,2,
2,4),(13.9098688392401,14.1556640945556,14.3228458792463,14.4188879587625,
14.6758880360635,14.8847408681272,15.0632003858644,15.2914213689572,15.4351943825689,
15.5397975605937,15.6907999063745,15.9505284316708,16.1174774019243,16.3504696402124,
16.5181559164659,16.6145926296687,16.8753658706323,17.0810835460594,17.2607658518236,
17.4935838069903,17.6283345220276,17.7320751647221,17.8802772177466,18.1456688450993,
18.3128274245213,18.5445902888266,18.7122051875404,18.8085807795861,19.0661478292541,
19.2739013729509,19.4527775282826,19.6825454438916,19.8241052324821,19.9291087000797,
20.0814014988205,20.3385969942852,20.5054666418987,20.7389878885708,20.9067110744443,
21.0031778248,21.264006667204,21.4696471635165,21.6493715566429,21.882332452245,
22.0170184957055,22.1208909453636,22.269513722124,22.5340676516857,22.7012001115818,
22.933162201478,23.100794947581,23.1971838319584,23.4547765389269,23.6625060379139,
23.8414008388903,24.0712225297513,24.2127230657623,24.3177427228717,24.4700810655704,
24.7272075613882,24.8940807985462,25.1276263420014,25.2953566309189,25.3918277354045,
25.6526675765619,25.858313103886,26.0380451905918,26.2710187231217,26.4057076175683,
26.5095877573895,26.6582285391607,26.9227667038272,27.082368010658,27.4239759561574,
27.5307307926211,27.585780009175,27.8196846114232),.UNSPECIFIED.) ;
#256=B_SPLINE_CURVE_WITH_KNOTS('',3,(#33777,#33778,#33779,#33780,#33781,
#33782,#33783,#33784,#33785,#33786,#33787,#33788,#33789,#33790,#33791,#33792,
#33793,#33794,#33795,#33796,#33797,#33798,#33799,#33800,#33801,#33802,#33803,
#33804,#33805,#33806,#33807,#33808,#33809,#33810,#33811,#33812,#33813,#33814,
#33815,#33816,#33817,#33818,#33819,#33820,#33821,#33822,#33823,#33824,#33825,
#33826,#33827,#33828,#33829,#33830,#33831,#33832,#33833,#33834,#33835,#33836,
#33837,#33838,#33839,#33840,#33841,#33842,#33843,#33844,#33845,#33846,#33847,
#33848,#33849,#33850,#33851,#33852,#33853,#33854,#33855,#33856,#33857,#33858,
#33859,#33860,#33861,#33862,#33863,#33864,#33865,#33866,#33867,#33868,#33869,
#33870,#33871,#33872,#33873,#33874,#33875,#33876,#33877,#33878,#33879,#33880,
#33881,#33882,#33883,#33884,#33885,#33886,#33887,#33888,#33889,#33890,#33891,
#33892,#33893,#33894,#33895,#33896,#33897,#33898,#33899,#33900,#33901,#33902,
#33903,#33904,#33905,#33906,#33907,#33908,#33909,#33910,#33911,#33912,#33913,
#33914,#33915,#33916,#33917,#33918,#33919,#33920,#33921,#33922,#33923,#33924,
#33925,#33926,#33927,#33928,#33929,#33930,#33931,#33932,#33933,#33934,#33935,
#33936,#33937,#33938,#33939,#33940,#33941,#33942,#33943,#33944,#33945,#33946,
#33947,#33948,#33949,#33950,#33951,#33952,#33953,#33954,#33955,#33956,#33957,
#33958,#33959,#33960,#33961,#33962,#33963,#33964,#33965,#33966,#33967,#33968,
#33969,#33970,#33971,#33972,#33973,#33974,#33975,#33976,#33977,#33978,#33979,
#33980,#33981,#33982,#33983,#33984,#33985,#33986,#33987,#33988,#33989,#33990,
#33991,#33992,#33993,#33994,#33995,#33996,#33997,#33998,#33999,#34000,#34001,
#34002,#34003,#34004,#34005,#34006,#34007,#34008,#34009,#34010,#34011,#34012,
#34013,#34014,#34015,#34016,#34017,#34018,#34019,#34020,#34021,#34022,#34023,
#34024,#34025,#34026,#34027,#34028,#34029,#34030,#34031,#34032,#34033,#34034,
#34035,#34036,#34037,#34038,#34039,#34040,#34041,#34042,#34043,#34044,#34045,
#34046,#34047,#34048,#34049,#34050,#34051,#34052,#34053,#34054,#34055,#34056,
#34057,#34058,#34059,#34060,#34061,#34062,#34063,#34064,#34065,#34066,#34067,
#34068,#34069,#34070,#34071,#34072,#34073,#34074,#34075,#34076,#34077,#34078,
#34079,#34080,#34081,#34082,#34083,#34084,#34085,#34086,#34087,#34088,#34089,
#34090,#34091,#34092,#34093,#34094,#34095,#34096,#34097,#34098,#34099,#34100,
#34101,#34102,#34103,#34104,#34105,#34106,#34107,#34108,#34109,#34110,#34111,
#34112,#34113,#34114,#34115,#34116),.UNSPECIFIED.,.F.,.F.,(4,3,3,3,3,3,
3,3,3,3,3,3,3,3,3,3,3,3,3,3,3,3,3,3,3,3,3,3,3,3,3,3,3,3,3,3,3,3,3,3,3,3,
3,3,3,3,3,3,3,3,3,3,3,3,3,3,3,3,3,3,3,3,3,3,3,3,3,3,3,3,3,3,3,3,3,3,3,3,
3,3,3,3,3,3,3,3,3,3,3,3,3,3,3,3,3,3,3,3,3,3,3,3,3,3,3,3,3,3,3,3,3,3,3,4),
(-29.2146074456426,-29.1543978565729,-29.0941972193378,-29.034002687827,
-28.9738114178698,-28.9136143857649,-28.8534164946886,-28.7932062199675,
-28.7441363464316,-28.6821877767195,-28.6218625733065,-28.5615435728776,
-28.501228171081,-28.4380580754944,-28.3777368279562,-28.317412879575,-28.2570789068001,
-28.2485477887345,-28.1865992190224,-28.126274015621,-28.065955015204,-28.0056396134189,
-27.9424695178235,-27.8821482702971,-27.8218243219273,-27.7614903491642,
-27.7529592310374,-27.6910106613253,-27.630685457917,-27.5703664574931,
-27.5100510557013,-27.4468809601111,-27.3865597125778,-27.3262357642009,
-27.2659017914312,-27.2573706733403,-27.1954221036282,-27.1350969002231,
-27.0747778998024,-27.0144624980132,-26.9512924024207,-26.8909711548904,
-26.8306472065173,-26.7703132337501,-26.7617821156432,-26.6998335459311,
-26.639508342525,-26.5791893421032,-26.5188739403131,-26.4557038447214,
-26.3953825971904,-26.3350586488164,-26.2747246760482,-26.2661935579461,
-26.204244988234,-26.1439197848279,-26.0836007844062,-26.0232853826161,
-25.9601152870243,-25.8997940394931,-25.83947009112,-25.7791361183522,-25.770605000249,
-25.7086564305369,-25.6483312271311,-25.5880122267092,-25.5276968249196,
-25.4645267293277,-25.4042054817964,-25.3438815334227,-25.2835475606549,
-25.2750164425519,-25.2130678728398,-25.1527426694337,-25.0924236690117,
-25.0321082672212,-24.9689381716296,-24.9086169240982,-24.8482929757248,
-24.7879590029576,-24.7794278848548,-24.7174793151427,-24.6571541117367,
-24.5968351113151,-24.536519709526,-24.4733496139339,-24.4130283664028,
-24.3527044180278,-24.292370445261,-24.2838393271577,-24.2218907574456,
-24.1615655540396,-24.101246553618,-24.0409311518278,-23.977761056236,-23.9174398087045,
-23.8571158603309,-23.7967818875636,-23.7882507694606,-23.7263021997485,
-23.6659769963423,-23.6056579959201,-23.5453425941303,-23.4821724985386,
-23.4218512510077,-23.361527302633,-23.3011933298654,-23.2926622117635,
-23.2324753090154,-23.1722980607319,-23.1120790869358,-23.0519100205918,
-22.9916660930697,-22.9314221655476),.UNSPECIFIED.) ;
#257=B_SPLINE_CURVE_WITH_KNOTS('',3,(#34117,#34118,#34119,#34120,#34121,
#34122,#34123,#34124,#34125,#34126,#34127,#34128,#34129,#34130,#34131,#34132,
#34133,#34134,#34135,#34136,#34137,#34138,#34139,#34140,#34141,#34142,#34143,
#34144,#34145,#34146,#34147,#34148,#34149,#34150,#34151,#34152,#34153,#34154,
#34155,#34156,#34157,#34158,#34159,#34160,#34161,#34162,#34163,#34164,#34165,
#34166,#34167,#34168,#34169,#34170,#34171,#34172,#34173,#34174,#34175,#34176,
#34177,#34178,#34179,#34180,#34181,#34182,#34183,#34184,#34185,#34186,#34187,
#34188,#34189,#34190,#34191,#34192,#34193,#34194,#34195,#34196,#34197,#34198,
#34199,#34200,#34201,#34202,#34203,#34204,#34205,#34206,#34207,#34208,#34209,
#34210,#34211,#34212,#34213,#34214,#34215,#34216,#34217,#34218,#34219,#34220,
#34221,#34222,#34223,#34224,#34225,#34226,#34227,#34228,#34229,#34230,#34231,
#34232,#34233,#34234,#34235,#34236,#34237,#34238,#34239,#34240,#34241,#34242,
#34243,#34244,#34245,#34246,#34247,#34248,#34249,#34250,#34251,#34252,#34253,
#34254,#34255,#34256,#34257,#34258,#34259,#34260,#34261,#34262,#34263,#34264,
#34265,#34266,#34267,#34268,#34269,#34270,#34271,#34272,#34273,#34274,#34275,
#34276,#34277,#34278,#34279,#34280,#34281,#34282,#34283,#34284,#34285,#34286,
#34287,#34288,#34289,#34290,#34291,#34292,#34293,#34294,#34295,#34296,#34297,
#34298,#34299,#34300,#34301,#34302,#34303,#34304,#34305,#34306,#34307,#34308,
#34309,#34310,#34311,#34312,#34313,#34314,#34315,#34316,#34317,#34318,#34319,
#34320,#34321,#34322,#34323,#34324,#34325,#34326,#34327,#34328,#34329,#34330,
#34331,#34332,#34333,#34334,#34335,#34336,#34337,#34338,#34339,#34340,#34341,
#34342,#34343,#34344,#34345,#34346,#34347,#34348,#34349,#34350,#34351,#34352,
#34353,#34354,#34355,#34356,#34357,#34358,#34359,#34360,#34361,#34362,#34363,
#34364,#34365,#34366,#34367,#34368,#34369,#34370,#34371,#34372,#34373,#34374,
#34375,#34376,#34377,#34378,#34379,#34380,#34381,#34382,#34383,#34384,#34385,
#34386,#34387,#34388,#34389,#34390,#34391,#34392,#34393,#34394,#34395,#34396,
#34397,#34398,#34399,#34400,#34401,#34402,#34403,#34404,#34405,#34406,#34407,
#34408,#34409,#34410,#34411,#34412,#34413,#34414,#34415,#34416,#34417,#34418,
#34419,#34420,#34421,#34422,#34423,#34424,#34425,#34426,#34427,#34428,#34429,
#34430,#34431,#34432,#34433,#34434,#34435,#34436,#34437,#34438,#34439,#34440,
#34441,#34442,#34443,#34444,#34445,#34446,#34447,#34448,#34449,#34450,#34451,
#34452,#34453,#34454,#34455,#34456),.UNSPECIFIED.,.F.,.F.,(4,3,3,3,3,3,
3,3,3,3,3,3,3,3,3,3,3,3,3,3,3,3,3,3,3,3,3,3,3,3,3,3,3,3,3,3,3,3,3,3,3,3,
3,3,3,3,3,3,3,3,3,3,3,3,3,3,3,3,3,3,3,3,3,3,3,3,3,3,3,3,3,3,3,3,3,3,3,3,
3,3,3,3,3,3,3,3,3,3,3,3,3,3,3,3,3,3,3,3,3,3,3,3,3,3,3,3,3,3,3,3,3,3,3,4),
(19.9596011324501,20.0197790710957,20.079953312403,20.1401332122979,20.2003136007354,
20.2605071303629,20.3191308655809,20.381079435293,20.4414046386991,20.5017236391209,
20.5620390409103,20.6252091365022,20.6855303840333,20.7458543324078,20.8061883051758,
20.814719423278,20.8766679929901,20.9369931963961,20.9973121968177,21.0576275986076,
21.1207976941995,21.1811189417305,21.2414428901052,21.301776862873,21.3103079809751,
21.3722565506872,21.4325817540933,21.492900754515,21.5532161563048,21.6163862518967,
21.6767074994277,21.7370314478021,21.7973654205698,21.8058965386722,21.8678451083843,
21.9281703117903,21.988489312212,22.0488047140018,22.1119748095937,22.1722960571249,
22.2326200054995,22.292953978267,22.3014850963693,22.3634336660814,22.4237588694873,
22.4840778699091,22.5443932716994,22.6075633672911,22.6678846148225,22.7282085631966,
22.7885425359647,22.7970736540664,22.8590222237785,22.9193474271845,22.9796664276061,
23.0399818293961,23.103151924988,23.1634731725189,23.2237971208939,23.2841310936618,
23.2926622117635,23.3546107814756,23.4149359848817,23.4752549853033,23.5355703870933,
23.5987404826852,23.6590617302163,23.7193856785906,23.7797196513582,23.7882507694606,
23.8501993391727,23.9105245425788,23.9708435430002,24.0311589447903,24.0943290403821,
24.1546502879132,24.2149742362876,24.2753082090551,24.2838393271577,24.3457878968698,
24.4061131002758,24.4664321006976,24.5267475024869,24.5899175980789,24.6502388456092,
24.7105627939837,24.7708967667503,24.7794278848548,24.8413764545669,24.9017016579728,
24.9620206583941,25.0223360601837,25.0855061557758,25.145827403307,25.2061513516832,
25.2664853244505,25.2750164425519,25.336965012264,25.3972902156699,25.4576092160917,
25.517924617882,25.5810947134737,25.6414159610052,25.7017399093814,25.7620738821499,
25.770605000249,25.8308224790742,25.8910307598749,25.9512326757154,26.0114310576459,
26.0716348337217,26.1318391994483,26.1920557052503,26.2427864138602),
 .UNSPECIFIED.) ;
#258=B_SPLINE_CURVE_WITH_KNOTS('',3,(#34461,#34462,#34463,#34464,#34465,
#34466,#34467,#34468,#34469,#34470,#34471,#34472,#34473,#34474,#34475,#34476,
#34477,#34478,#34479,#34480,#34481,#34482,#34483,#34484,#34485,#34486,#34487,
#34488,#34489,#34490,#34491,#34492,#34493,#34494,#34495,#34496,#34497,#34498,
#34499,#34500,#34501,#34502,#34503,#34504,#34505,#34506,#34507,#34508,#34509,
#34510,#34511,#34512,#34513,#34514,#34515,#34516,#34517,#34518,#34519,#34520,
#34521,#34522,#34523,#34524,#34525,#34526,#34527,#34528,#34529,#34530,#34531,
#34532,#34533,#34534,#34535,#34536,#34537,#34538,#34539,#34540,#34541,#34542,
#34543,#34544,#34545,#34546,#34547,#34548,#34549,#34550,#34551,#34552,#34553,
#34554,#34555,#34556,#34557,#34558,#34559,#34560,#34561,#34562,#34563,#34564,
#34565,#34566,#34567,#34568,#34569,#34570,#34571,#34572,#34573,#34574,#34575,
#34576,#34577,#34578,#34579,#34580,#34581,#34582,#34583,#34584,#34585,#34586,
#34587,#34588,#34589,#34590,#34591,#34592,#34593,#34594,#34595,#34596,#34597,
#34598,#34599,#34600,#34601,#34602,#34603,#34604,#34605,#34606,#34607,#34608,
#34609,#34610,#34611,#34612,#34613,#34614,#34615,#34616,#34617,#34618,#34619,
#34620,#34621,#34622,#34623,#34624,#34625,#34626,#34627,#34628,#34629,#34630,
#34631,#34632,#34633,#34634,#34635,#34636,#34637,#34638,#34639,#34640,#34641,
#34642,#34643,#34644,#34645,#34646,#34647,#34648,#34649,#34650,#34651,#34652,
#34653,#34654,#34655,#34656,#34657,#34658,#34659,#34660,#34661,#34662,#34663,
#34664,#34665,#34666,#34667,#34668,#34669,#34670,#34671,#34672,#34673,#34674,
#34675,#34676,#34677,#34678,#34679,#34680,#34681,#34682,#34683,#34684,#34685,
#34686,#34687,#34688,#34689,#34690,#34691,#34692,#34693,#34694,#34695,#34696,
#34697,#34698,#34699,#34700,#34701,#34702,#34703,#34704,#34705,#34706,#34707,
#34708,#34709,#34710,#34711,#34712,#34713,#34714,#34715,#34716,#34717,#34718,
#34719,#34720,#34721,#34722,#34723,#34724,#34725,#34726,#34727,#34728,#34729,
#34730,#34731,#34732,#34733,#34734,#34735,#34736,#34737,#34738,#34739,#34740,
#34741,#34742,#34743,#34744,#34745,#34746,#34747,#34748,#34749,#34750,#34751,
#34752,#34753,#34754,#34755,#34756,#34757,#34758,#34759,#34760,#34761,#34762,
#34763,#34764,#34765,#34766,#34767,#34768,#34769,#34770,#34771,#34772,#34773,
#34774,#34775,#34776,#34777,#34778,#34779,#34780,#34781,#34782,#34783,#34784,
#34785,#34786,#34787,#34788,#34789,#34790,#34791,#34792,#34793,#34794,#34795,
#34796,#34797,#34798,#34799,#34800,#34801,#34802,#34803,#34804,#34805,#34806),
 .UNSPECIFIED.,.F.,.F.,(4,3,3,3,3,3,3,3,3,3,3,3,3,3,3,3,3,3,3,3,3,3,3,3,
3,3,3,3,3,3,3,3,3,3,3,3,3,3,3,3,3,3,3,3,3,3,3,3,3,3,3,3,3,3,3,3,3,3,3,3,
3,3,3,3,3,3,3,3,3,3,3,3,3,3,3,3,3,3,3,3,3,3,3,3,3,3,3,3,3,3,3,3,3,3,3,3,
3,3,3,3,3,3,3,3,3,3,3,3,3,3,3,3,3,3,3,4),(-35.4977927799067,-35.4373549022818,
-35.3747130758348,-35.314266582531,-35.2538167087216,-35.1933564437769,
-35.1867875964938,-35.1248390267817,-35.0645138625596,-35.0041949016703,
-34.9438795396833,-34.8807094144617,-34.8203882070317,-34.7600642987708,
-34.699730365999,-34.6911990387967,-34.6292504690846,-34.5689252380228,
-34.5086062097224,-34.4482907798863,-34.3851207051896,-34.3247994294596,
-34.2644754528975,-34.2041414520523,-34.1956104810996,-34.1336619113875,
-34.0733367226025,-34.0130177369113,-33.9527023499317,-33.8895322432994,
-33.8292110106377,-33.7688870771199,-33.7085531191401,-33.7000219234025,
-33.6380733536904,-33.577748144358,-33.5174291379697,-33.4571137301851,
-33.3939436390652,-33.3336223855255,-33.2732984311522,-33.2129644524189,
-33.2044333657054,-33.1424847959933,-33.0821595941034,-33.0218405952054,
-32.9615251949437,-32.8983550982098,-32.8380338522037,-32.7777099053508,
-32.7173759340923,-32.7088448080083,-32.6468962382962,-32.5865710350704,
-32.5262520348324,-32.4659366332302,-32.4027665375005,-32.3424452901631,
-32.2821213419845,-32.2217873694142,-32.2132562503113,-32.1513076805991,
-32.0909824766373,-32.0306634756543,-31.9703480732994,-31.9071779781281,
-31.8468567300272,-31.7865327810836,-31.7261988077471,-31.7176676926141,
-31.655719122902,-31.5953939199476,-31.5350749199809,-31.4747595186488,
-31.4115894227158,-31.3512681756456,-31.2909442277319,-31.2306102554234,
-31.2220791349171,-31.160130565205,-31.0998053615387,-31.0394863608549,
-30.9791709588018,-30.9160008634064,-30.8556796156103,-30.7953556669706,
-30.7350216939395,-30.72649057722,-30.6645420075079,-30.604216804218,-30.5438978039128,
-30.4835824022401,-30.4204123065608,-30.3600910591481,-30.2997671108904,
-30.2394331382394,-30.2309020195229,-30.1689534498108,-30.108628246368,
-30.0483092459097,-29.9879938440825,-29.9248237485183,-29.8645025009507,
-29.8041785525403,-29.7438445797366,-29.7353134618258,-29.6733648921137,
-29.6130396887101,-29.5527206882902,-29.4924052865024,-29.429235190909,
-29.36891394338,-29.3085899950081,-29.2482560222431,-29.2397249041287,-29.2146074727272),
 .UNSPECIFIED.) ;
#259=B_SPLINE_CURVE_WITH_KNOTS('',3,(#34807,#34808,#34809,#34810,#34811,
#34812,#34813,#34814,#34815,#34816,#34817,#34818,#34819,#34820,#34821,#34822,
#34823,#34824,#34825,#34826,#34827,#34828,#34829,#34830,#34831,#34832,#34833,
#34834,#34835,#34836,#34837,#34838,#34839,#34840,#34841,#34842,#34843,#34844,
#34845,#34846,#34847,#34848,#34849,#34850,#34851,#34852,#34853,#34854,#34855,
#34856,#34857,#34858,#34859,#34860,#34861,#34862,#34863,#34864,#34865,#34866,
#34867,#34868,#34869,#34870,#34871,#34872,#34873,#34874,#34875,#34876,#34877,
#34878,#34879,#34880,#34881,#34882,#34883,#34884,#34885,#34886,#34887,#34888,
#34889,#34890,#34891,#34892,#34893,#34894,#34895,#34896,#34897,#34898,#34899,
#34900,#34901,#34902,#34903,#34904,#34905,#34906,#34907,#34908,#34909,#34910,
#34911,#34912,#34913,#34914,#34915,#34916,#34917,#34918,#34919,#34920,#34921,
#34922,#34923,#34924,#34925,#34926,#34927,#34928,#34929,#34930,#34931,#34932,
#34933,#34934,#34935,#34936,#34937,#34938,#34939,#34940,#34941,#34942,#34943,
#34944,#34945,#34946,#34947,#34948,#34949,#34950,#34951,#34952,#34953,#34954,
#34955,#34956,#34957,#34958,#34959,#34960,#34961,#34962,#34963,#34964,#34965,
#34966,#34967,#34968,#34969,#34970,#34971,#34972,#34973,#34974,#34975,#34976,
#34977,#34978,#34979,#34980,#34981,#34982,#34983,#34984,#34985,#34986,#34987,
#34988,#34989,#34990,#34991,#34992,#34993,#34994,#34995,#34996,#34997,#34998,
#34999,#35000,#35001,#35002,#35003,#35004,#35005,#35006,#35007,#35008,#35009,
#35010,#35011,#35012,#35013,#35014,#35015,#35016,#35017,#35018,#35019,#35020,
#35021,#35022,#35023,#35024,#35025,#35026,#35027,#35028,#35029,#35030,#35031,
#35032,#35033,#35034,#35035,#35036,#35037,#35038,#35039,#35040,#35041,#35042,
#35043,#35044,#35045,#35046,#35047,#35048,#35049,#35050,#35051,#35052,#35053,
#35054,#35055,#35056,#35057,#35058,#35059,#35060,#35061,#35062,#35063,#35064,
#35065,#35066,#35067,#35068,#35069,#35070,#35071,#35072,#35073,#35074,#35075,
#35076,#35077,#35078,#35079,#35080,#35081,#35082,#35083,#35084,#35085,#35086,
#35087,#35088,#35089,#35090,#35091,#35092,#35093,#35094,#35095,#35096,#35097,
#35098,#35099,#35100,#35101,#35102,#35103,#35104,#35105,#35106,#35107,#35108,
#35109,#35110,#35111,#35112,#35113,#35114,#35115,#35116,#35117,#35118,#35119,
#35120,#35121,#35122,#35123,#35124,#35125,#35126,#35127,#35128,#35129,#35130,
#35131,#35132,#35133,#35134,#35135,#35136,#35137,#35138,#35139,#35140,#35141,
#35142,#35143,#35144,#35145,#35146,#35147,#35148,#35149,#35150,#35151,#35152),
 .UNSPECIFIED.,.F.,.F.,(4,3,3,3,3,3,3,3,3,3,3,3,3,3,3,3,3,3,3,3,3,3,3,3,
3,3,3,3,3,3,3,3,3,3,3,3,3,3,3,3,3,3,3,3,3,3,3,3,3,3,3,3,3,3,3,3,3,3,3,3,
3,3,3,3,3,3,3,3,3,3,3,3,3,3,3,3,3,3,3,3,3,3,3,3,3,3,3,3,3,3,3,3,3,3,3,3,
3,3,3,3,3,3,3,3,3,3,3,3,3,3,3,3,3,3,3,4),(26.2427864396297,26.2661935579461,
26.3281421276582,26.388467331065,26.4487863314875,26.509101733278,26.5722718288693,
26.6325930764013,26.6929170247759,26.7532509975444,26.7617821156432,26.8237306853553,
26.8840558887602,26.9443748891806,27.0046902909692,27.067860386562,27.128181634092,
27.1885055824644,27.2488395552309,27.2573706733403,27.3193192430524,27.3796444464606,
27.4399634468845,27.5002788486765,27.5634489442667,27.6237701918,27.6840941401761,
27.744428112946,27.7529592310374,27.8149078007495,27.875233004151,27.9355520045683,
27.9958674063536,28.0590375019488,28.1193587494755,28.1796826978451,28.2400166706085,
28.2485477887345,28.3104963584466,28.3708215618596,28.4311405622883,28.4914559640852,
28.5546260596718,28.6149473072098,28.6752712555904,28.735605228365,28.7441363464316,
28.8060849161437,28.8664101195424,28.9267291199569,28.9870445217396,29.0502146173369,
29.1105358648609,29.1708598132279,29.2311937859887,29.2397249041287,29.3016734738408,
29.3619986772444,29.4223176776636,29.482633079451,29.5458031750447,29.6061244225732,
29.6664483709447,29.7267823437097,29.7353134618258,29.7972620315379,29.8575872349799,
29.9179062354377,29.9782216372637,30.0413917328285,30.1017129803954,30.1620369288052,
30.2223709016083,30.2309020195229,30.292850589235,30.3531757925255,30.4134947928316,
30.4738101945057,30.5369802901843,30.597301537601,30.6576254858612,30.7179594585165,
30.72649057722,30.7884391469321,30.848764350598,30.9090833512799,30.9693987533295,
31.0325688487264,31.0928900965141,31.1532140451428,31.2135480181622,31.2220791349171,
31.2840277046292,31.3443529075824,31.4046719075513,31.4649873088892,31.5281574048204,
31.5884786519057,31.6488025998371,31.709136572168,31.7176676926141,31.7796162623263,
31.839941466294,31.9002604672771,31.9605758696268,32.0237459647979,32.0840672128796,
32.1443911617988,32.2047251351045,32.2132562503113,32.2737037987142,32.336770785738,
32.397202128338,32.457628314494,32.5180533031214,32.5259717468093),
 .UNSPECIFIED.) ;
#260=B_SPLINE_CURVE_WITH_KNOTS('',3,(#35159,#35160,#35161,#35162,#35163,
#35164,#35165,#35166,#35167,#35168,#35169,#35170,#35171,#35172,#35173,#35174,
#35175,#35176,#35177,#35178,#35179,#35180,#35181,#35182,#35183,#35184,#35185,
#35186,#35187,#35188,#35189,#35190,#35191,#35192,#35193,#35194,#35195,#35196,
#35197,#35198,#35199,#35200,#35201,#35202,#35203,#35204,#35205,#35206,#35207,
#35208,#35209,#35210,#35211,#35212,#35213,#35214,#35215,#35216,#35217,#35218,
#35219,#35220,#35221,#35222,#35223,#35224,#35225,#35226,#35227,#35228,#35229,
#35230,#35231,#35232,#35233,#35234,#35235,#35236,#35237,#35238,#35239,#35240,
#35241,#35242,#35243,#35244,#35245,#35246,#35247,#35248,#35249,#35250,#35251,
#35252,#35253,#35254,#35255,#35256,#35257,#35258,#35259,#35260,#35261,#35262,
#35263,#35264,#35265,#35266,#35267,#35268,#35269,#35270,#35271,#35272,#35273,
#35274,#35275,#35276,#35277,#35278,#35279,#35280,#35281,#35282,#35283,#35284,
#35285,#35286,#35287,#35288,#35289,#35290,#35291,#35292,#35293,#35294,#35295,
#35296,#35297,#35298,#35299,#35300,#35301,#35302,#35303,#35304,#35305,#35306,
#35307,#35308,#35309,#35310,#35311,#35312,#35313,#35314,#35315,#35316,#35317,
#35318,#35319,#35320,#35321,#35322,#35323,#35324,#35325,#35326,#35327,#35328,
#35329,#35330,#35331,#35332,#35333,#35334,#35335,#35336,#35337,#35338,#35339,
#35340,#35341,#35342,#35343,#35344,#35345,#35346,#35347,#35348,#35349,#35350,
#35351,#35352,#35353,#35354,#35355,#35356,#35357,#35358,#35359,#35360,#35361,
#35362,#35363,#35364,#35365,#35366,#35367,#35368,#35369,#35370,#35371,#35372,
#35373,#35374,#35375,#35376,#35377,#35378,#35379,#35380,#35381,#35382,#35383,
#35384,#35385,#35386,#35387,#35388,#35389,#35390,#35391,#35392,#35393,#35394,
#35395,#35396,#35397,#35398,#35399,#35400,#35401,#35402,#35403,#35404,#35405,
#35406,#35407,#35408,#35409,#35410,#35411,#35412,#35413,#35414,#35415,#35416,
#35417,#35418,#35419,#35420,#35421,#35422,#35423,#35424,#35425,#35426,#35427,
#35428,#35429,#35430,#35431,#35432,#35433,#35434,#35435,#35436,#35437,#35438,
#35439,#35440,#35441,#35442,#35443,#35444,#35445,#35446,#35447,#35448,#35449,
#35450,#35451,#35452,#35453,#35454,#35455,#35456,#35457,#35458,#35459,#35460,
#35461,#35462,#35463,#35464,#35465,#35466,#35467,#35468,#35469,#35470,#35471,
#35472,#35473,#35474,#35475,#35476,#35477,#35478,#35479,#35480,#35481,#35482,
#35483,#35484,#35485,#35486,#35487,#35488,#35489,#35490,#35491,#35492),
 .UNSPECIFIED.,.F.,.F.,(4,3,3,3,3,3,3,3,3,3,3,3,3,3,3,3,3,3,3,3,3,3,3,3,
3,3,3,3,3,3,3,3,3,3,3,3,3,3,3,3,3,3,3,3,3,3,3,3,3,3,3,3,3,3,3,3,3,3,3,3,
3,3,3,3,3,3,3,3,3,3,3,3,3,3,3,3,3,3,3,3,3,3,3,3,3,3,3,3,3,3,3,3,3,3,3,3,
3,3,3,3,3,3,3,3,3,3,3,3,3,3,3,4),(-41.6294388465561,-41.567490276844,-41.5068129036286,
-41.4461373909485,-41.3854619060442,-41.3225590017479,-41.2618724615581,
-41.2011823182609,-41.1404821935598,-41.133850288859,-41.0719017191469,
-41.0117574354034,-40.9516209847975,-40.8914894119347,-40.8313597630322,
-40.7712239022798,-40.7110856043998,-40.650936698952,-40.6382617311619,
-40.5763131614498,-40.5158900890388,-40.4554724366547,-40.3950577994203,
-40.3319616429314,-40.2715406611331,-40.2111170377586,-40.1506838110237,
-40.1426731734648,-40.0807246037527,-40.0204417302746,-39.9601653570302,
-39.8998927959327,-39.8366907508915,-39.7764124738498,-39.7161314439029,
-39.6558401732367,-39.6470846157677,-39.5851360460556,-39.5247976669795,
-39.4644654135086,-39.4041367076079,-39.3409765452236,-39.2806419927029,
-39.2203047694599,-39.1599576085501,-39.1514960580706,-39.0895474883585,
-39.0292231358422,-38.968904978419,-38.9085904100647,-38.8454196826419,
-38.7850992366082,-38.7247760768171,-38.6644428719227,-38.6559075003735,
-38.5939589306614,-38.5336363799959,-38.4733200593599,-38.4130073590988,
-38.3498352549932,-38.2895167377735,-38.2291955234812,-38.1688642808967,
-38.1603189426764,-38.0983703729643,-38.038042569437,-37.9777209466698,
-37.9174029055051,-37.8542347753736,-37.7939108709406,-37.7335842656406,
-37.6732476448322,-37.6647303849793,-37.6027818152672,-37.5424582539623,
-37.4821409085262,-37.4218271713306,-37.3586558353185,-37.2983362606098,
-37.2380139841017,-37.1776816762533,-37.1691418272822,-37.1071932575701,
-37.0468672569077,-36.9865474534408,-36.9262312444077,-36.863061750702,
-36.8027396930987,-36.7424149355172,-36.6820801574679,-36.6735532695851,
-36.611604699873,-36.551279784747,-36.4909610744466,-36.4306459640453,-36.367475651006,
-36.3071546952618,-36.2468310381478,-36.1864973549261,-36.177964711888,
-36.1160161421759,-36.0556908873698,-35.9953718354003,-35.9350563820169,
-35.8718863250604,-35.811565026313,-35.7512410269701,-35.6909070037518,
-35.6823761541909,-35.6203299863175,-35.5582978922954,-35.4977928149021),
 .UNSPECIFIED.) ;
#261=B_SPLINE_CURVE_WITH_KNOTS('',3,(#35493,#35494,#35495,#35496,#35497,
#35498,#35499,#35500,#35501,#35502,#35503,#35504,#35505,#35506,#35507,#35508,
#35509,#35510,#35511,#35512,#35513,#35514,#35515,#35516,#35517,#35518,#35519,
#35520,#35521,#35522,#35523,#35524,#35525,#35526,#35527,#35528,#35529,#35530,
#35531,#35532,#35533,#35534,#35535,#35536,#35537,#35538,#35539,#35540,#35541,
#35542,#35543,#35544,#35545,#35546,#35547,#35548,#35549,#35550,#35551,#35552,
#35553,#35554,#35555,#35556,#35557,#35558,#35559,#35560,#35561,#35562,#35563,
#35564,#35565,#35566,#35567,#35568,#35569,#35570,#35571,#35572,#35573,#35574,
#35575,#35576,#35577,#35578,#35579,#35580,#35581,#35582,#35583,#35584,#35585,
#35586,#35587,#35588,#35589,#35590,#35591,#35592,#35593,#35594,#35595,#35596,
#35597,#35598,#35599,#35600,#35601,#35602,#35603,#35604,#35605,#35606,#35607,
#35608,#35609,#35610,#35611,#35612,#35613,#35614,#35615,#35616,#35617,#35618,
#35619,#35620,#35621,#35622,#35623,#35624,#35625,#35626,#35627,#35628,#35629,
#35630,#35631,#35632,#35633,#35634,#35635,#35636,#35637,#35638,#35639,#35640,
#35641,#35642,#35643,#35644,#35645,#35646,#35647,#35648,#35649,#35650,#35651,
#35652,#35653,#35654,#35655,#35656,#35657,#35658,#35659,#35660,#35661,#35662,
#35663,#35664,#35665,#35666,#35667,#35668,#35669,#35670,#35671,#35672,#35673,
#35674,#35675,#35676,#35677,#35678,#35679,#35680,#35681,#35682,#35683,#35684,
#35685,#35686,#35687,#35688,#35689,#35690,#35691,#35692,#35693,#35694,#35695,
#35696,#35697,#35698,#35699,#35700,#35701,#35702,#35703,#35704,#35705,#35706,
#35707,#35708,#35709,#35710,#35711,#35712,#35713,#35714,#35715,#35716,#35717,
#35718,#35719,#35720,#35721,#35722,#35723,#35724,#35725,#35726,#35727,#35728,
#35729,#35730,#35731,#35732,#35733,#35734,#35735,#35736,#35737,#35738,#35739,
#35740,#35741,#35742,#35743,#35744,#35745,#35746,#35747,#35748,#35749,#35750,
#35751,#35752,#35753,#35754,#35755,#35756,#35757,#35758,#35759,#35760,#35761,
#35762,#35763,#35764,#35765,#35766,#35767,#35768,#35769,#35770,#35771,#35772,
#35773,#35774,#35775,#35776,#35777,#35778,#35779,#35780,#35781,#35782,#35783,
#35784,#35785,#35786,#35787,#35788,#35789,#35790,#35791,#35792,#35793,#35794,
#35795,#35796,#35797,#35798,#35799,#35800,#35801,#35802,#35803,#35804,#35805,
#35806,#35807,#35808,#35809,#35810,#35811,#35812,#35813,#35814,#35815,#35816,
#35817,#35818,#35819,#35820,#35821,#35822,#35823,#35824,#35825,#35826,#35827,
#35828,#35829,#35830,#35831,#35832,#35833,#35834,#35835),.UNSPECIFIED.,
 .F.,.F.,(4,3,3,3,3,3,3,3,3,3,3,3,3,3,3,3,3,3,3,3,3,3,3,3,3,3,3,3,3,3,3,
3,3,3,3,3,3,3,3,3,3,3,3,3,3,3,3,3,3,3,3,3,3,3,3,3,3,3,3,3,3,3,3,3,3,3,3,
3,3,3,3,3,3,3,3,3,3,3,3,3,3,3,3,3,3,3,3,3,3,3,3,3,3,3,3,3,3,3,3,3,3,3,3,
3,3,3,3,3,3,3,3,3,3,3,4),(32.5259717819584,32.588029893979,32.6501070318688,
32.7088448080084,32.7707933777205,32.8311185796354,32.8914375785607,32.951752978852,
33.0149230755653,33.0752443216065,33.1355682684968,33.1959022397947,33.2044333657054,
33.2663819354175,33.3267071447261,33.3870261510605,33.4473415587615,33.5105116499217,
33.5708329033046,33.6311568574965,33.6914908360153,33.7000219234025,33.7619704931146,
33.8222956818779,33.8826146676421,33.9429300547883,34.0061001613661,34.066421394426,
34.1267453284214,34.1870792869874,34.1956104810996,34.2575590508117,34.3178842820452,
34.3782033103068,34.4385187398944,34.50168881462,34.5620100895816,34.6223340651971,
34.6826680648513,34.6911990387967,34.7531476085088,34.8134727722351,34.8737917329921,
34.9341070952092,34.9972772205304,35.0575984290914,35.1179223387918,35.1782562734283,
35.1867875964938,35.2487361662059,35.3090613994056,35.369380429522,35.4296958608503,
35.4928659341855,35.5531872105891,35.6135111875406,35.6738451883794,35.6823761541909,
35.744324723903,35.8046499773561,35.8649690281093,35.9252844804149,35.9884545382831,
36.0487758363077,36.1090998350517,36.1694338578468,36.177964711888,36.2399132816001,
36.300238197271,36.3605569093567,36.4208720227762,36.4840423344784,36.5443632962832,
36.6046869604949,36.6650206522349,36.6735532695851,36.7355018392972,36.7958278437611,
36.8561476462205,36.9164638494562,36.9796333439127,37.0399553838398,37.1002801196819,
37.1606148704077,37.1691418272822,37.2310903969943,37.291413942665,37.3517312842844,
37.4120450294478,37.4752163683307,37.5355359802912,37.5958583040811,37.6561906730196,
37.6647303849793,37.7266789546914,37.7870067972581,37.8473284367508,37.9076464723714,
37.9708145899476,38.031138433411,38.0914649587342,38.1518014733698,38.1603189426764,
38.2222675123885,38.2825899914703,38.3429062719906,38.4032189635737,38.4663910977737,
38.5267096847223,38.5870309956665,38.6473623720695,38.6559075003735,38.7185947802169,
38.7812660984336,38.8091570245189),.UNSPECIFIED.) ;
#262=B_SPLINE_CURVE_WITH_KNOTS('',3,(#35841,#35842,#35843,#35844,#35845,
#35846,#35847,#35848,#35849,#35850,#35851,#35852,#35853,#35854,#35855,#35856,
#35857,#35858,#35859,#35860,#35861,#35862,#35863,#35864,#35865,#35866,#35867,
#35868,#35869,#35870,#35871,#35872,#35873,#35874,#35875,#35876,#35877,#35878,
#35879,#35880,#35881,#35882,#35883,#35884,#35885,#35886,#35887,#35888,#35889,
#35890,#35891,#35892,#35893,#35894,#35895,#35896,#35897,#35898,#35899,#35900,
#35901,#35902,#35903,#35904,#35905,#35906,#35907,#35908,#35909,#35910,#35911,
#35912,#35913,#35914,#35915,#35916,#35917,#35918,#35919,#35920,#35921,#35922,
#35923,#35924,#35925,#35926,#35927,#35928,#35929,#35930,#35931,#35932,#35933,
#35934,#35935,#35936,#35937,#35938),.UNSPECIFIED.,.F.,.F.,(4,2,2,2,2,2,
2,2,2,2,2,2,2,2,2,2,2,2,2,2,2,2,2,2,2,2,2,2,2,2,2,2,2,2,2,2,2,2,2,2,2,2,
2,2,2,2,2,2,4),(-8.6283049271654,-8.44563511642056,-8.26252267487022,-8.09546352263789,
-7.93482896054982,-7.81992734806337,-7.62625451933204,-7.42468926409441,
-7.23019569314527,-6.99118982362461,-6.89161836480484,-6.7080558318219,
-6.44464309997694,-6.27048108699121,-6.05333123482325,-5.92170915794646,
-5.81119227905867,-5.63452184767797,-5.42175995687018,-5.23923964233179,
-5.11200558695375,-4.92271658910161,-4.82048727563227,-4.67440773777088,
-4.43080365520216,-4.25778980550549,-4.04526002899663,-3.90739432205506,
-3.79929099426129,-3.63162373705064,-3.42044304635338,-3.24652543009668,
-3.03042830592731,-2.89736788090823,-2.78721938360196,-2.61200305571173,
-2.39899408459298,-2.21760220863657,-1.97106907021256,-1.8636225674043,
-1.67308020303453,-1.4019990020959,-1.22784167090017,-1.01012824950624,
-0.871498618028422,-0.746912125939072,-0.403443808576563,-0.30289397028493,
-1.00000000635703E-6),.UNSPECIFIED.) ;
#263=B_SPLINE_CURVE_WITH_KNOTS('',3,(#35941,#35942,#35943,#35944,#35945,
#35946,#35947,#35948,#35949,#35950,#35951,#35952,#35953,#35954,#35955,#35956,
#35957,#35958,#35959,#35960,#35961,#35962,#35963,#35964,#35965,#35966,#35967,
#35968,#35969,#35970,#35971,#35972,#35973,#35974,#35975,#35976,#35977,#35978,
#35979,#35980,#35981,#35982,#35983,#35984,#35985,#35986,#35987,#35988,#35989,
#35990,#35991,#35992,#35993,#35994,#35995,#35996,#35997,#35998,#35999,#36000,
#36001,#36002,#36003,#36004,#36005,#36006,#36007,#36008,#36009,#36010,#36011,
#36012),.UNSPECIFIED.,.F.,.F.,(4,2,2,2,2,2,2,2,2,2,2,2,2,2,2,2,2,2,2,2,
2,2,2,2,2,2,2,2,2,2,2,2,2,2,2,4),(-80.5246266814036,-80.1666400655345,-80.0053224599515,
-79.7602571484243,-79.6065532257719,-79.5034892892416,-79.3649560014289,
-79.149023933939,-78.9752478356705,-78.7288342161045,-78.5853061673665,
-78.4835684711015,-78.3013460459308,-78.1711839038137,-77.986351085049,
-77.7720026203175,-77.5968503405372,-77.4864799335814,-77.3241970195642,
-77.124749503217,-76.9556934438728,-76.6796488708706,-76.5012330945668,
-76.3898224188898,-76.1560480763953,-75.9710887556106,-75.7582801102011,
-75.5807809927086,-75.4699172140184,-75.3359737020451,-75.1206153925808,
-74.9470295109835,-74.7403046328623,-74.569427574836,-74.4605084889714,
-74.4589523653195),.UNSPECIFIED.) ;
#264=B_SPLINE_CURVE_WITH_KNOTS('',3,(#36017,#36018,#36019,#36020,#36021,
#36022,#36023,#36024,#36025,#36026,#36027,#36028,#36029,#36030,#36031,#36032,
#36033,#36034,#36035,#36036,#36037,#36038,#36039,#36040,#36041,#36042,#36043,
#36044,#36045,#36046,#36047,#36048,#36049,#36050,#36051,#36052,#36053,#36054,
#36055,#36056,#36057,#36058,#36059,#36060,#36061,#36062,#36063,#36064,#36065,
#36066,#36067,#36068,#36069,#36070,#36071,#36072,#36073,#36074,#36075,#36076,
#36077,#36078,#36079,#36080,#36081,#36082,#36083,#36084,#36085,#36086,#36087,
#36088,#36089,#36090,#36091,#36092,#36093,#36094,#36095,#36096,#36097,#36098,
#36099,#36100,#36101,#36102,#36103,#36104,#36105,#36106,#36107,#36108,#36109,
#36110,#36111,#36112,#36113,#36114,#36115,#36116,#36117,#36118,#36119,#36120,
#36121,#36122,#36123,#36124,#36125,#36126,#36127,#36128,#36129,#36130,#36131,
#36132,#36133,#36134,#36135,#36136,#36137,#36138,#36139,#36140,#36141,#36142,
#36143,#36144,#36145,#36146,#36147,#36148,#36149,#36150,#36151,#36152,#36153,
#36154,#36155,#36156,#36157,#36158,#36159,#36160),.UNSPECIFIED.,.F.,.F.,
(4,2,2,2,2,2,2,2,2,2,2,2,2,2,2,2,2,2,2,2,2,2,2,2,2,2,2,2,2,2,2,2,2,2,2,
2,2,2,2,2,2,2,2,2,2,2,2,2,2,2,2,2,2,2,2,2,2,2,2,2,2,2,2,2,2,2,2,2,2,2,2,
4),(-21.4112482236887,-21.395018839335,-21.1786168465405,-21.0460115238846,
-20.9359359568184,-20.7609107582667,-20.5479128146165,-20.3669372388779,
-20.1219005459217,-20.01212254847,-19.8210807003159,-19.5511547240092,-19.3765640904682,
-19.1576946106882,-19.0206800954041,-18.8974475163927,-18.5178607380296,
-18.3260088901507,-18.0897196278096,-17.9872267539132,-17.7957545253425,
-17.5358887773981,-17.3619377606238,-17.1456460818616,-17.0129023635293,
-16.9028860341006,-16.7280790286043,-16.5150805001345,-16.3343156219491,
-16.0901169990782,-15.9796193960046,-15.7901984333427,-15.517685168774,
-15.3429409300139,-15.1234403336084,-14.9873344434116,-14.8636672269134,
-14.4862875752506,-14.2959466369376,-14.0612755975542,-13.9567916457698,
-13.7788983270654,-13.5003576759277,-13.3252913165706,-13.10447614829,-12.9775670876658,
-12.8648511184702,-12.6797428835252,-12.4739818922446,-12.2873174175172,
-11.9780281867481,-11.8741210996828,-11.7218506369985,-11.489466218588,
-11.3168413061589,-11.105915354737,-10.9663548850042,-10.8594637224488,
-10.6962625606892,-10.4804969704791,-10.3075555629212,-10.0953574493798,
-9.95702541736544,-9.84903262735902,-9.68177387436709,-9.47012502269245,
-9.29625963443787,-9.08033275022843,-8.94708756555045,-8.83727055637995,
-8.66321978929217,-8.6283049271654),.UNSPECIFIED.) ;
#265=B_SPLINE_CURVE_WITH_KNOTS('',3,(#36161,#36162,#36163,#36164,#36165,
#36166,#36167,#36168,#36169,#36170,#36171,#36172,#36173,#36174,#36175,#36176,
#36177,#36178,#36179,#36180,#36181,#36182,#36183,#36184,#36185,#36186,#36187,
#36188,#36189,#36190,#36191,#36192,#36193,#36194,#36195,#36196,#36197,#36198,
#36199,#36200,#36201,#36202,#36203,#36204,#36205,#36206,#36207,#36208,#36209,
#36210,#36211,#36212,#36213,#36214,#36215,#36216,#36217,#36218,#36219,#36220,
#36221,#36222,#36223,#36224,#36225,#36226,#36227,#36228,#36229,#36230,#36231,
#36232,#36233,#36234,#36235,#36236,#36237,#36238,#36239,#36240,#36241,#36242,
#36243,#36244,#36245,#36246,#36247,#36248,#36249,#36250,#36251,#36252,#36253,
#36254,#36255,#36256,#36257,#36258,#36259,#36260,#36261,#36262,#36263,#36264,
#36265,#36266,#36267,#36268,#36269,#36270,#36271,#36272,#36273,#36274,#36275,
#36276,#36277,#36278,#36279,#36280,#36281,#36282,#36283,#36284,#36285,#36286,
#36287,#36288,#36289,#36290,#36291,#36292,#36293,#36294,#36295,#36296,#36297,
#36298,#36299,#36300,#36301,#36302,#36303,#36304,#36305,#36306,#36307,#36308,
#36309,#36310,#36311,#36312),.UNSPECIFIED.,.F.,.F.,(4,2,2,2,2,2,2,2,2,2,
2,2,2,2,2,2,2,2,2,2,2,2,2,2,2,2,2,2,2,2,2,2,2,2,2,2,2,2,2,2,2,2,2,2,2,2,
2,2,2,2,2,2,2,2,2,2,2,2,2,2,2,2,2,2,2,2,2,2,2,2,2,2,2,2,2,4),(-74.4589523653195,
-74.3265007778098,-74.1110963267903,-73.9373025312386,-73.7347057927969,
-73.561860568035,-73.4523376858543,-73.3176312089985,-73.1027395663676,
-72.9291097723617,-72.726632241673,-72.5536717587562,-72.4441399440812,
-72.3004543074962,-72.0903185907499,-71.9178862184339,-71.6982031634796,
-71.5382433967428,-71.4322305051113,-71.292424008278,-71.0820984090018,
-70.9095934273694,-70.6889884263145,-70.5295921806519,-70.4237274826831,
-70.2838865719299,-70.0737103989504,-69.9012631469297,-69.6810805418431,
-69.5214303218753,-69.41550305007,-69.2756816129106,-69.0654273530361,-68.8929521476015,
-68.6726317279836,-68.5130705959056,-68.4071647676874,-68.2673383955658,
-68.0571217499896,-67.884661524328,-67.6645673682827,-67.5048663734266,
-67.3989249106178,-67.2591098422661,-67.0488598611346,-66.8763918770729,
-66.658651669558,-66.4974507682909,-66.3911002858384,-66.2513826672066,
-66.0408439496718,-65.8683060418149,-65.6401772541515,-65.4309829879885,
-65.3350553589436,-65.0929076908778,-64.8950377985158,-64.6972644760291,
-64.4491847467691,-64.4060739836119,-64.2986816063683,-64.0508943899226,
-63.8691274930506,-63.6561956981757,-63.4803176045911,-63.3700110952462,
-63.2379366317503,-63.0211171077155,-62.8470246104173,-62.6395444686835,
-62.4692160690279,-62.3603925705269,-62.2244718845535,-62.0105182173817,
-61.8371361301002,-61.6753285154585),.UNSPECIFIED.) ;
#266=B_SPLINE_CURVE_WITH_KNOTS('',3,(#36317,#36318,#36319,#36320,#36321,
#36322,#36323,#36324,#36325,#36326,#36327,#36328,#36329,#36330,#36331,#36332,
#36333,#36334,#36335,#36336,#36337,#36338,#36339,#36340,#36341,#36342,#36343,
#36344,#36345,#36346,#36347,#36348,#36349,#36350,#36351,#36352,#36353,#36354,
#36355,#36356,#36357,#36358,#36359,#36360,#36361,#36362,#36363,#36364,#36365,
#36366,#36367,#36368,#36369,#36370,#36371,#36372,#36373,#36374,#36375,#36376,
#36377,#36378,#36379,#36380,#36381,#36382,#36383,#36384,#36385,#36386,#36387,
#36388,#36389,#36390,#36391,#36392,#36393,#36394,#36395,#36396,#36397,#36398,
#36399,#36400,#36401,#36402,#36403,#36404,#36405,#36406,#36407,#36408,#36409,
#36410,#36411,#36412,#36413,#36414,#36415,#36416,#36417,#36418,#36419,#36420,
#36421,#36422,#36423,#36424,#36425,#36426,#36427,#36428,#36429,#36430,#36431,
#36432,#36433,#36434,#36435,#36436,#36437,#36438,#36439,#36440,#36441,#36442,
#36443,#36444,#36445,#36446,#36447,#36448,#36449,#36450,#36451,#36452,#36453,
#36454,#36455,#36456,#36457,#36458,#36459,#36460,#36461,#36462,#36463,#36464),
 .UNSPECIFIED.,.F.,.F.,(4,2,2,2,2,2,2,2,2,2,2,2,2,2,2,2,2,2,2,2,2,2,2,2,
2,2,2,2,2,2,2,2,2,2,2,2,2,2,2,2,2,2,2,2,2,2,2,2,2,2,2,2,2,2,2,2,2,2,2,2,
2,2,2,2,2,2,2,2,2,2,2,2,2,4),(-34.1936391063407,-34.1526970834958,-34.0424813560459,
-33.8669170704365,-33.6539735846087,-33.4724917747383,-33.2253958642913,
-33.1173551327557,-32.9264081971104,-32.6582814268131,-32.483810603873,
-32.265402438362,-32.1277449105955,-32.0048155318769,-31.62374016017,-31.4308157047062,
-31.1934125312668,-31.0922100941797,-31.046804554797,-30.9172170606046,
-30.640647352708,-30.4656834280484,-30.2452703249294,-30.1184391905269,
-30.0066984351524,-29.825338795797,-29.6181078581474,-29.4345881974818,
-29.1783538943782,-29.0766484422157,-29.0314901472356,-28.903181133213,
-28.6240155892456,-28.4489244570544,-28.2279958106869,-28.101300372818,
-27.9885874062051,-27.8034838329686,-27.5977287160442,-27.4110695718176,
-27.1017882629211,-26.9978834700024,-26.8456153892239,-26.6132401534391,
-26.4406194907526,-26.2296982363399,-26.090141922616,-25.9832525168262,
-25.8200514725944,-25.6042957006854,-25.4313581532595,-25.2191616273762,
-25.0808395456631,-24.9728489461978,-24.8055916252599,-24.5939515075186,
-24.4200907745686,-24.2041691860031,-24.0709281545374,-23.9611090447325,
-23.7870453902097,-23.569558169572,-23.3864923558574,-23.2164704392175,
-23.0586180687099,-22.9436096408969,-22.7495001276715,-22.5483067922997,
-22.353543415325,-22.1142890470351,-22.0149792499618,-21.8292879644468,
-21.568999457946,-21.4112482236887),.UNSPECIFIED.) ;
#267=B_SPLINE_CURVE_WITH_KNOTS('',3,(#36465,#36466,#36467,#36468,#36469,
#36470,#36471,#36472,#36473,#36474,#36475,#36476,#36477,#36478,#36479,#36480,
#36481,#36482,#36483,#36484,#36485,#36486,#36487,#36488,#36489,#36490,#36491,
#36492,#36493,#36494,#36495,#36496,#36497,#36498,#36499,#36500,#36501,#36502,
#36503,#36504,#36505,#36506,#36507,#36508,#36509,#36510,#36511,#36512,#36513,
#36514,#36515,#36516,#36517,#36518,#36519,#36520,#36521,#36522,#36523,#36524,
#36525,#36526,#36527,#36528,#36529,#36530,#36531,#36532,#36533,#36534,#36535,
#36536,#36537,#36538,#36539,#36540,#36541,#36542,#36543,#36544,#36545,#36546,
#36547,#36548,#36549,#36550,#36551,#36552,#36553,#36554,#36555,#36556,#36557,
#36558,#36559,#36560,#36561,#36562,#36563,#36564,#36565,#36566,#36567,#36568,
#36569,#36570,#36571,#36572,#36573,#36574,#36575,#36576,#36577,#36578,#36579,
#36580,#36581,#36582,#36583,#36584,#36585,#36586,#36587,#36588,#36589,#36590,
#36591,#36592,#36593,#36594,#36595,#36596,#36597,#36598,#36599,#36600,#36601,
#36602,#36603,#36604,#36605,#36606,#36607,#36608,#36609,#36610,#36611,#36612),
 .UNSPECIFIED.,.F.,.F.,(4,2,2,2,2,2,2,2,2,2,2,2,2,2,2,2,2,2,2,2,2,2,2,2,
2,2,2,2,2,2,2,2,2,2,2,2,2,2,2,2,2,2,2,2,2,2,2,2,2,2,2,2,2,2,2,2,2,2,2,2,
2,2,2,2,2,2,2,2,2,2,2,2,2,4),(-61.6753285154585,-61.6228359350141,-61.4580058246525,
-61.3506687888318,-61.2112613683406,-60.9999976335177,-60.82728245136,-60.6109254773445,
-60.4484481206533,-60.3417516253654,-60.202128704269,-59.9913443765748,
-59.8187492239848,-59.6021458502637,-59.4400166941392,-59.333415823976,
-59.1937688820631,-58.9830552850426,-58.8104791396269,-58.5801878127834,
-58.4266935186611,-58.3224509856121,-58.0123777319399,-57.8258717399889,
-57.6200037585776,-57.4350862756363,-57.3224177640415,-57.1958753725372,
-56.9748722836351,-56.7997560142291,-56.5202163191938,-56.3431495648183,
-56.2386178812058,-56.0039804817052,-55.8136681421047,-55.4363229335071,
-55.3126407866901,-55.1765513551912,-54.9570357797179,-54.7822842467627,
-54.5097109125687,-54.3222211715738,-54.2137989371203,-53.9671522627128,
-53.7857752745581,-53.5728020054108,-53.3973461293979,-53.2871555118113,
-53.1548254634903,-52.9382182238007,-52.7641853742159,-52.5549825616221,
-52.3858738418835,-52.2773823413023,-52.1405410142872,-51.9272766375091,
-51.7540723281387,-51.5071681601972,-51.3121195888342,-51.2138263409947,
-50.973471975645,-50.7775697538017,-50.5777247821068,-50.3307160871589,
-50.2881713296445,-50.1786052451498,-49.9333229491322,-49.7522852299641,
-49.5392844508873,-49.3641886634143,-49.2540937423335,-49.1215300736148,
-48.9050993610572,-48.8923243137223),.UNSPECIFIED.) ;
#268=B_SPLINE_CURVE_WITH_KNOTS('',3,(#36617,#36618,#36619,#36620,#36621,
#36622,#36623,#36624,#36625,#36626,#36627,#36628,#36629,#36630,#36631,#36632,
#36633,#36634,#36635,#36636,#36637,#36638,#36639,#36640,#36641,#36642,#36643,
#36644,#36645,#36646,#36647,#36648,#36649,#36650,#36651,#36652,#36653,#36654,
#36655,#36656,#36657,#36658,#36659,#36660,#36661,#36662,#36663,#36664,#36665,
#36666,#36667,#36668,#36669,#36670,#36671,#36672,#36673,#36674,#36675,#36676,
#36677,#36678,#36679,#36680,#36681,#36682,#36683,#36684,#36685,#36686,#36687,
#36688,#36689,#36690,#36691,#36692,#36693,#36694,#36695,#36696,#36697,#36698,
#36699,#36700,#36701,#36702,#36703,#36704,#36705,#36706,#36707,#36708,#36709,
#36710,#36711,#36712,#36713,#36714,#36715,#36716,#36717,#36718,#36719,#36720,
#36721,#36722,#36723,#36724,#36725,#36726,#36727,#36728,#36729,#36730,#36731,
#36732,#36733,#36734,#36735,#36736,#36737,#36738,#36739,#36740,#36741,#36742,
#36743,#36744,#36745,#36746,#36747,#36748,#36749,#36750,#36751,#36752,#36753,
#36754,#36755,#36756),.UNSPECIFIED.,.F.,.F.,(4,2,2,2,2,2,2,2,2,2,2,2,2,
2,2,2,2,2,2,2,2,2,2,2,2,2,2,2,2,2,2,2,2,2,2,2,2,2,2,2,2,2,2,2,2,2,2,2,2,
2,2,2,2,2,2,2,2,2,2,2,2,2,2,2,2,2,2,2,2,4),(-46.9761112544596,-46.887959319714,
-46.7131715474143,-46.4396544303016,-46.2630271782697,-46.1624606952762,
-45.924487784234,-45.7310006255373,-45.3491627751212,-45.2263888687142,
-45.0883949216917,-44.8702369915205,-44.6958328063143,-44.4286423908784,
-44.2476883150171,-44.1477658417111,-43.9091656490518,-43.7150557229674,
-43.3323905629399,-43.2097750395941,-43.0714067915801,-42.8534998994136,
-42.6791555505541,-42.41295365977,-42.2267415181231,-42.1241220332522,-41.8879612904891,
-41.6962270516749,-41.3168066906816,-41.1935489113774,-41.0566066379994,
-40.8377084040195,-40.6631167026597,-40.3930248956316,-40.2602686457487,
-40.1614948136577,-39.9712357283276,-39.717589879487,-39.5440241228471,
-39.3292689229644,-39.1944821485798,-39.0852649836751,-38.9134417067484,
-38.7085802334176,-38.5346327441269,-38.3183406707748,-38.1856101147548,
-38.0755933914421,-37.9007777221915,-37.6877856691828,-37.507012703818,
-37.2627670479032,-37.1523202854762,-37.1099843269924,-36.8628889891071,
-36.6625531933715,-36.4670986898819,-36.2271740881804,-36.128511827087,
-35.9372096831459,-35.6850548715227,-35.5115749896293,-35.2971675371291,
-35.1619082853902,-35.0528651788837,-34.8816915200588,-34.6756393220112,
-34.5016007066658,-34.2849409728589,-34.1936391063407),.UNSPECIFIED.) ;
#269=B_SPLINE_CURVE_WITH_KNOTS('',3,(#36757,#36758,#36759,#36760,#36761,
#36762,#36763,#36764,#36765,#36766,#36767,#36768,#36769,#36770,#36771,#36772,
#36773,#36774,#36775,#36776,#36777,#36778,#36779,#36780,#36781,#36782,#36783,
#36784,#36785,#36786,#36787,#36788,#36789,#36790,#36791,#36792,#36793,#36794,
#36795,#36796,#36797,#36798,#36799,#36800,#36801,#36802,#36803,#36804,#36805,
#36806,#36807,#36808,#36809,#36810,#36811,#36812,#36813,#36814,#36815,#36816,
#36817,#36818,#36819,#36820,#36821,#36822,#36823,#36824,#36825,#36826,#36827,
#36828,#36829,#36830,#36831,#36832,#36833,#36834,#36835,#36836,#36837,#36838,
#36839,#36840,#36841,#36842,#36843,#36844,#36845,#36846,#36847,#36848,#36849,
#36850,#36851,#36852,#36853,#36854,#36855,#36856,#36857,#36858,#36859,#36860,
#36861,#36862,#36863,#36864,#36865,#36866,#36867,#36868,#36869,#36870,#36871,
#36872,#36873,#36874,#36875,#36876,#36877,#36878,#36879,#36880,#36881,#36882,
#36883,#36884,#36885,#36886,#36887,#36888,#36889,#36890,#36891,#36892,#36893,
#36894,#36895,#36896,#36897,#36898,#36899,#36900,#36901,#36902),
 .UNSPECIFIED.,.F.,.F.,(4,2,2,2,2,2,2,2,2,2,2,2,2,2,2,2,2,2,2,2,2,2,2,2,
2,2,2,2,2,2,2,2,2,2,2,2,2,2,2,2,2,2,2,2,2,2,2,2,2,2,2,2,2,2,2,2,2,2,2,2,
2,2,2,2,2,2,2,2,2,2,2,2,4),(-48.8923243137223,-48.7311102437702,-48.4706971753778,
-48.2850805924847,-48.1857596435972,-47.9465181468345,-47.7517652195359,
-47.5505532007241,-47.3564530917116,-47.2414462242878,-47.0837073368052,
-46.9138544860948,-46.7306722642033,-46.518172647404,-46.3406619295693,
-46.2299276804503,-46.0988870050805,-45.881301830456,-45.7070281233357,
-45.4421203801134,-45.2492795993685,-45.1421281434426,-44.8938617393175,
-44.7121152693629,-44.4991963054057,-44.3233385544006,-44.2130416958794,
-44.0809711977412,-43.8641696370465,-43.6900895105923,-43.4824272948797,
-43.3122402199191,-43.2034588723095,-43.0674485332026,-42.8535811826038,
-42.680228459931,-42.3945193861139,-42.271790433139,-42.2277299954773,-42.1233538359875,
-41.8885949478744,-41.6981709741039,-41.3206583063989,-41.197009222143,
-41.060852538196,-40.8413838659923,-40.6666437124145,-40.3942671157565,
-40.2626060616138,-40.1640932887395,-39.9712757348543,-39.7212425122708,
-39.5478712057474,-39.3339324865582,-39.1980079905828,-39.0891951193058,
-38.918893231552,-38.711410109376,-38.5373264214066,-38.3205144570587,-38.1884461808277,
-38.0781473211432,-37.9022844381012,-37.6893683189646,-37.5076112921277,
-37.2597770807576,-37.1524168668946,-36.9755748468808,-36.6921066358992,
-36.5167312594253,-36.294688310285,-36.1710739584292,-36.1093811124386),
 .UNSPECIFIED.) ;
#270=B_SPLINE_CURVE_WITH_KNOTS('',3,(#36907,#36908,#36909,#36910,#36911,
#36912,#36913,#36914,#36915,#36916,#36917,#36918,#36919,#36920,#36921,#36922,
#36923,#36924,#36925,#36926,#36927,#36928,#36929,#36930,#36931,#36932,#36933,
#36934,#36935,#36936,#36937,#36938,#36939,#36940,#36941,#36942,#36943,#36944,
#36945,#36946,#36947,#36948,#36949,#36950,#36951,#36952,#36953,#36954,#36955,
#36956,#36957,#36958,#36959,#36960,#36961,#36962,#36963,#36964,#36965,#36966,
#36967,#36968,#36969,#36970,#36971,#36972,#36973,#36974,#36975,#36976,#36977,
#36978,#36979,#36980,#36981,#36982,#36983,#36984,#36985,#36986,#36987,#36988,
#36989,#36990,#36991,#36992,#36993,#36994,#36995,#36996,#36997,#36998,#36999,
#37000,#37001,#37002,#37003,#37004,#37005,#37006,#37007,#37008,#37009,#37010,
#37011,#37012,#37013,#37014,#37015,#37016,#37017,#37018,#37019,#37020,#37021,
#37022,#37023,#37024,#37025,#37026,#37027,#37028,#37029,#37030,#37031,#37032,
#37033,#37034,#37035,#37036,#37037,#37038,#37039,#37040,#37041,#37042,#37043,
#37044,#37045,#37046,#37047,#37048,#37049,#37050,#37051,#37052,#37053,#37054,
#37055,#37056),.UNSPECIFIED.,.F.,.F.,(4,2,2,2,2,2,2,2,2,2,2,2,2,2,2,2,2,
2,2,2,2,2,2,2,2,2,2,2,2,2,2,2,2,2,2,2,2,2,2,2,2,2,2,2,2,2,2,2,2,2,2,2,2,
2,2,2,2,2,2,2,2,2,2,2,2,2,2,2,2,2,2,2,2,2,4),(-59.7576642542407,-59.5933744459689,
-59.4338184624438,-59.3279219508154,-59.188111664293,-58.9779089966092,
-58.8054641205551,-58.5851882669472,-58.4256344828241,-58.3197393690206,
-58.1799308625549,-57.9697309211142,-57.7972882660943,-57.577015372777,
-57.4174635456083,-57.3115697652949,-57.1717630540937,-56.9615657795836,
-56.7891253229855,-56.5688551907947,-56.4093054418243,-56.3034130257952,
-56.1636081016588,-55.9534135298879,-55.7809752851254,-55.5607079879421,
-55.4011602717046,-55.2952692091105,-55.1554660753708,-54.9452741896308,
-54.7728381505053,-54.5525736959291,-54.3930280076242,-54.2871382963303,
-54.1473369529504,-53.9371477560825,-53.7647139239242,-53.5444513981186,
-53.3849083145396,-53.279020112319,-53.1392205235918,-52.9290341279034,
-52.7566025303904,-52.5363804760838,-52.3768156488363,-52.2709223086606,
-52.1311259868732,-51.9209375912665,-51.7485070421084,-51.5295534196106,
-51.3691865786828,-51.2630751521756,-51.1233310020683,-50.9129874194926,
-50.7405200698919,-50.5147898879696,-50.3072521043426,-50.2112007438594,
-49.9432253358134,-49.7565323181416,-49.5508157270068,-49.3656601613506,
-49.2529377922316,-49.1261477278738,-48.9052897136255,-48.7302234356747,
-48.4513591565083,-48.2728065805656,-48.1675160513685,-47.9334953291543,
-47.7437434841282,-47.3672580888974,-47.2434274595821,-47.1076791434906,
-46.9761112544596),.UNSPECIFIED.) ;
#271=B_SPLINE_CURVE_WITH_KNOTS('',3,(#37057,#37058,#37059,#37060,#37061,
#37062,#37063,#37064,#37065,#37066,#37067,#37068,#37069,#37070,#37071,#37072,
#37073,#37074,#37075,#37076,#37077,#37078,#37079,#37080,#37081,#37082,#37083,
#37084,#37085,#37086,#37087,#37088,#37089,#37090,#37091,#37092,#37093,#37094,
#37095,#37096,#37097,#37098,#37099,#37100,#37101,#37102,#37103,#37104,#37105,
#37106,#37107,#37108,#37109,#37110,#37111,#37112,#37113,#37114,#37115,#37116,
#37117,#37118,#37119,#37120,#37121,#37122,#37123,#37124,#37125,#37126,#37127,
#37128,#37129,#37130,#37131,#37132,#37133,#37134,#37135,#37136,#37137,#37138,
#37139,#37140,#37141,#37142,#37143,#37144,#37145,#37146,#37147,#37148,#37149,
#37150,#37151,#37152,#37153,#37154,#37155,#37156,#37157,#37158,#37159,#37160,
#37161,#37162,#37163,#37164,#37165,#37166,#37167,#37168,#37169,#37170,#37171,
#37172,#37173,#37174,#37175,#37176,#37177,#37178,#37179,#37180,#37181,#37182,
#37183,#37184,#37185,#37186,#37187,#37188,#37189,#37190,#37191,#37192,#37193,
#37194,#37195,#37196,#37197,#37198,#37199,#37200,#37201,#37202),
 .UNSPECIFIED.,.F.,.F.,(4,2,2,2,2,2,2,2,2,2,2,2,2,2,2,2,2,2,2,2,2,2,2,2,
2,2,2,2,2,2,2,2,2,2,2,2,2,2,2,2,2,2,2,2,2,2,2,2,2,2,2,2,2,2,2,2,2,2,2,2,
2,2,2,2,2,2,2,2,2,2,2,2,4),(-36.1093811124386,-36.059797019336,-35.8802277972535,
-35.6828168746143,-35.5069094314293,-35.2827111342303,-35.151117375553,
-35.0190731635707,-34.6470151800124,-34.4493600629226,-34.2073681631372,
-34.1113225917796,-33.9041369981001,-33.6734984391581,-33.5009153618648,
-33.2901659340044,-33.1505319122536,-33.0438858079697,-32.8815878157741,
-32.6651157479579,-32.492461697318,-32.2814314033653,-32.1419106931438,
-32.0348828588114,-31.8711850728226,-31.6558375621578,-31.4827493038765,
-31.2699695197905,-31.1324358815375,-31.0241753827991,-30.8559313620608,
-30.645560686355,-30.4715926842249,-30.2552634409984,-30.1225430663045,
-30.0125066105907,-29.8376391204446,-29.6246274794085,-29.4438028008348,
-29.1993945104597,-29.0890593822841,-28.8990471431737,-28.6273506283001,
-28.4526447571417,-28.2333306667098,-28.0969315775383,-27.9733961740721,
-27.5952916723206,-27.4044669019083,-27.1692706080269,-27.0654291954941,
-26.8759947765048,-26.6115868538986,-26.4373403468686,-26.2198756063967,
-26.088660565147,-25.9779984966219,-25.8007665613539,-25.5881753882271,
-25.4052207109607,-25.277012342567,-25.0908300755658,-24.9892704444479,
-24.845701269077,-24.5972924815534,-24.4240009379411,-24.2104076248183,
-24.0739894173798,-23.9653435726816,-23.7956737648866,-23.5872421169101,
-23.4131668872054,-23.3261135788128),.UNSPECIFIED.) ;
#272=B_SPLINE_CURVE_WITH_KNOTS('',3,(#37207,#37208,#37209,#37210,#37211,
#37212,#37213,#37214,#37215,#37216,#37217,#37218,#37219,#37220,#37221,#37222,
#37223,#37224,#37225,#37226,#37227,#37228,#37229,#37230,#37231,#37232,#37233,
#37234,#37235,#37236,#37237,#37238,#37239,#37240,#37241,#37242,#37243,#37244,
#37245,#37246,#37247,#37248,#37249,#37250,#37251,#37252,#37253,#37254,#37255,
#37256,#37257,#37258,#37259,#37260,#37261,#37262,#37263,#37264,#37265,#37266,
#37267,#37268,#37269,#37270,#37271,#37272,#37273,#37274,#37275,#37276,#37277,
#37278,#37279,#37280,#37281,#37282,#37283,#37284,#37285,#37286,#37287,#37288,
#37289,#37290,#37291,#37292,#37293,#37294,#37295,#37296,#37297,#37298,#37299,
#37300,#37301,#37302,#37303,#37304,#37305,#37306,#37307,#37308,#37309,#37310,
#37311,#37312,#37313,#37314,#37315,#37316,#37317,#37318,#37319,#37320,#37321,
#37322,#37323,#37324,#37325,#37326,#37327,#37328,#37329,#37330,#37331,#37332,
#37333,#37334,#37335,#37336,#37337,#37338,#37339,#37340,#37341,#37342,#37343,
#37344,#37345,#37346,#37347,#37348,#37349,#37350,#37351,#37352,#37353,#37354,
#37355,#37356,#37357,#37358,#37359,#37360,#37361,#37362),.UNSPECIFIED.,
 .F.,.F.,(4,2,2,2,2,2,2,2,2,2,2,2,2,2,2,2,2,2,2,2,2,2,2,2,2,2,2,2,2,2,2,
2,2,2,2,2,2,2,2,2,2,2,2,2,2,2,2,2,2,2,2,2,2,2,2,2,2,2,2,2,2,2,2,2,2,2,2,
2,2,2,2,2,2,2,2,2,2,4),(-72.5408068653678,-72.4391534491535,-72.2954642163267,
-72.0853270421682,-71.9128932356433,-71.6931951744418,-71.5332421280119,
-71.4272305392111,-71.2874223100186,-71.077096347533,-70.9045903798868,
-70.6839783638239,-70.5245839584325,-70.4187192648185,-70.2788769277484,
-70.0686992119904,-69.8962505191355,-69.676056586719,-69.5164108517257,
-69.4104842553953,-69.2706612128027,-69.0604062046357,-68.8879298574234,
-68.6676033055693,-68.5080433944154,-68.4021373891409,-68.262309628792,
-68.05209139734,-67.8796297739851,-67.659319606616,-67.4997525201673,-67.393847081321,
-67.25402236401,-67.0437970512951,-66.8713341719612,-66.6510498184925,-66.4914713007699,
-66.3855629356491,-66.2457405650643,-66.0355178602222,-65.8630570459642,
-65.6427513883988,-65.4831893790932,-65.3772864117109,-65.2374650056748,
-65.0272476019066,-64.8547900216135,-64.6345028319881,-64.474933400994,
-64.3690292788099,-64.2292102574205,-64.0189932278641,-63.8465369725667,
-63.6262448370045,-63.4666821782468,-63.3607806131091,-63.2209630624664,
-63.0107501229198,-62.8382965998372,-62.6180101833715,-62.4584477843913,
-62.3525471496183,-62.2127315202632,-62.0025206188915,-61.8300690621381,
-61.6097848819375,-61.4502248961111,-61.3443256863569,-61.2045118116099,
-60.994303823011,-60.8218545537725,-60.6015729642054,-60.4420151511489,
-60.3361173450703,-60.1963052573786,-59.9860999300074,-59.8136528590843,
-59.7576642542407),.UNSPECIFIED.) ;
#273=B_SPLINE_CURVE_WITH_KNOTS('',3,(#37363,#37364,#37365,#37366,#37367,
#37368,#37369,#37370,#37371,#37372,#37373,#37374,#37375,#37376,#37377,#37378,
#37379,#37380,#37381,#37382,#37383,#37384,#37385,#37386,#37387,#37388,#37389,
#37390,#37391,#37392,#37393,#37394,#37395,#37396,#37397,#37398,#37399,#37400,
#37401,#37402,#37403,#37404,#37405,#37406,#37407,#37408,#37409,#37410,#37411,
#37412,#37413,#37414,#37415,#37416,#37417,#37418,#37419,#37420,#37421,#37422,
#37423,#37424,#37425,#37426,#37427,#37428,#37429,#37430,#37431,#37432,#37433,
#37434,#37435,#37436,#37437,#37438,#37439,#37440,#37441,#37442,#37443,#37444,
#37445,#37446,#37447,#37448,#37449,#37450,#37451,#37452,#37453,#37454,#37455,
#37456,#37457,#37458,#37459,#37460,#37461,#37462,#37463,#37464,#37465,#37466,
#37467,#37468,#37469,#37470,#37471,#37472,#37473,#37474,#37475,#37476,#37477,
#37478,#37479,#37480,#37481,#37482,#37483,#37484,#37485,#37486,#37487,#37488,
#37489,#37490,#37491,#37492,#37493,#37494,#37495,#37496,#37497,#37498,#37499,
#37500,#37501,#37502,#37503,#37504,#37505,#37506,#37507,#37508),
 .UNSPECIFIED.,.F.,.F.,(4,2,2,2,2,2,2,2,2,2,2,2,2,2,2,2,2,2,2,2,2,2,2,2,
2,2,2,2,2,2,2,2,2,2,2,2,2,2,2,2,2,2,2,2,2,2,2,2,2,2,2,2,2,2,2,2,2,2,2,2,
2,2,2,2,2,2,2,2,2,2,2,2,4),(-23.3261135788128,-23.1964122101452,-23.0642484493351,
-22.9539813882199,-22.778249740813,-22.5653025552382,-22.3836641930565,
-22.1282235208404,-22.0242491936684,-21.8369835871211,-21.5698412106102,
-21.3954151573718,-21.1772412301014,-21.0391945576416,-20.9164167373402,
-20.5344605856882,-20.3408935159719,-20.1028309733555,-20.0023019437154,
-19.8253186808675,-19.5522518367965,-19.3774650802196,-19.1578223420381,
-19.0218904733213,-18.8981241350163,-18.5211803167825,-18.3311315652274,
-18.0967783795858,-17.9918572842245,-17.8015295407976,-17.5365947175085,
-17.3623149656535,-17.1447146028426,-17.0136779253518,-16.9029390390793,
-16.7254157304334,-16.5129199959725,-16.3297211405915,-16.1459749552859,
-16.0078912622961,-15.8998137655918,-15.7322476667436,-15.5209855844207,
-15.3470836956579,-15.1310224393778,-14.9979448674968,-14.8880515511446,
-14.7137223485656,-14.4976288883751,-14.3152746440806,-14.1883830381326,
-13.9980150996916,-13.8955256353688,-13.7484955119404,-13.5066310847622,
-13.3336531396858,-13.1213377043073,-12.9831420011226,-12.8750953885095,
-12.7076522530855,-12.4962138280885,-12.3223183804109,-12.1063015828812,
-11.9731491078745,-11.8632801018285,-11.6890507397833,-11.4723357756697,
-11.2896572000988,-11.1620685942577,-10.9738931175874,-10.8718966904332,
-10.7267076612704,-10.5425049368748),.UNSPECIFIED.) ;
#274=B_SPLINE_CURVE_WITH_KNOTS('',3,(#37514,#37515,#37516,#37517,#37518,
#37519,#37520,#37521,#37522,#37523,#37524,#37525,#37526,#37527,#37528,#37529,
#37530,#37531,#37532,#37533,#37534,#37535,#37536,#37537,#37538,#37539,#37540,
#37541,#37542,#37543,#37544,#37545,#37546,#37547,#37548,#37549,#37550,#37551,
#37552,#37553,#37554,#37555,#37556,#37557,#37558,#37559,#37560,#37561,#37562,
#37563,#37564,#37565,#37566,#37567,#37568,#37569,#37570,#37571,#37572,#37573,
#37574,#37575,#37576,#37577,#37578,#37579,#37580,#37581,#37582,#37583,#37584,
#37585,#37586,#37587,#37588,#37589,#37590,#37591,#37592,#37593,#37594,#37595,
#37596,#37597,#37598,#37599,#37600,#37601,#37602,#37603,#37604,#37605,#37606,
#37607,#37608,#37609,#37610,#37611,#37612,#37613,#37614,#37615,#37616,#37617,
#37618,#37619,#37620,#37621,#37622,#37623,#37624,#37625,#37626,#37627,#37628,
#37629,#37630,#37631,#37632,#37633,#37634,#37635,#37636,#37637,#37638,#37639,
#37640,#37641,#37642,#37643,#37644,#37645,#37646,#37647,#37648,#37649,#37650,
#37651,#37652,#37653,#37654,#37655,#37656,#37657,#37658,#37659,#37660,#37661,
#37662,#37663,#37664,#37665,#37666,#37667,#37668,#37669,#37670,#37671,#37672,
#37673,#37674,#37675,#37676,#37677,#37678,#37679,#37680,#37681,#37682,#37683,
#37684,#37685,#37686,#37687,#37688,#37689,#37690,#37691,#37692,#37693,#37694,
#37695,#37696,#37697,#37698,#37699,#37700,#37701,#37702,#37703,#37704,#37705,
#37706,#37707,#37708,#37709,#37710,#37711,#37712,#37713,#37714,#37715,#37716,
#37717,#37718,#37719,#37720,#37721,#37722,#37723,#37724,#37725,#37726,#37727,
#37728,#37729,#37730,#37731,#37732,#37733,#37734,#37735,#37736,#37737,#37738,
#37739,#37740,#37741,#37742,#37743,#37744,#37745,#37746,#37747,#37748,#37749,
#37750,#37751,#37752,#37753),.UNSPECIFIED.,.F.,.F.,(4,2,2,2,2,2,2,2,2,2,
2,2,2,2,2,2,2,2,2,2,2,2,2,2,2,2,2,2,2,2,2,2,2,2,2,2,2,2,2,2,2,2,2,2,2,2,
2,2,2,2,2,2,2,2,2,2,2,2,2,2,2,2,2,2,2,2,2,2,2,2,2,2,2,2,2,2,2,2,2,2,2,2,
2,2,2,2,2,2,2,2,2,2,2,2,2,2,2,2,2,2,2,2,2,2,2,2,2,2,2,2,2,2,2,2,2,2,2,2,
2,4),(-7.07001074019559,-6.97214799296548,-6.86257413286767,-6.815076472517,
-6.77781127057839,-6.73435011765435,-6.64787909076555,-6.51661040762408,
-6.38274658248721,-6.34808760339101,-6.32936344415715,-6.30808846045213,
-6.27074207319299,-6.2211598558415,-6.07834832333788,-5.94288381481757,
-5.89779633375777,-5.85982903394297,-5.81931476283132,-5.75073449114823,
-5.70297785800585,-5.52925430061811,-5.44364308355816,-5.41803276265346,
-5.39792813650759,-5.37448251943844,-5.32533346674813,-5.17375247153273,
-5.01651467495703,-4.97144238528326,-4.9334755870355,-4.89294824119181,
-4.82430744727727,-4.77648907560603,-4.60228634462766,-4.51736172903062,
-4.49173201521265,-4.47162424844343,-4.44819645774043,-4.39913656527529,
-4.247686484259,-4.10327612770059,-4.04763579703826,-4.00973399465062,-3.96992400695954,
-3.9053390477792,-3.8233409502829,-3.71812616332203,-3.68973805571307,-3.59319124604815,
-3.56382019913162,-3.5439000307015,-3.51973495493247,-3.46614699626435,
-3.38120386675306,-3.16800726161808,-3.12137332113153,-3.08345076694654,
-3.04365603404235,-2.97918496125071,-2.89740332700571,-2.79191626716292,
-2.77546374061009,-2.67591475821705,-2.64203033053413,-2.62343344176577,
-2.60194884328964,-2.56356273770187,-2.51202638466183,-2.35598119717274,
-2.26681982957397,-2.20328757294974,-2.16365752688015,-2.12518099839849,
-2.06837297332616,-2.00026103662752,-1.83338532789489,-1.73975551249685,
-1.71080075654854,-1.69093948456169,-1.66657999711708,-1.61159897970373,
-1.52303217123091,-1.31734880043544,-1.26458886979624,-1.22676414386914,
-1.1914426910813,-1.13499811808568,-1.06156327628703,-0.855608151594484,
-0.801459131626637,-0.777206119362864,-0.758416903670133,-0.7559933625668,
-0.754383203189016,-0.753152784062996,-0.752131919506535,-0.751234637396342,
-0.750409970413967,-0.749623510843456,-0.748848986992787,-0.748063705107264,
-0.747245569367162,-0.746370635723716,-0.74541057345217,-0.744329492112801,
-0.743079473345434,-0.741593827743262,-0.739776504427147,-0.737485107454084,
-0.734503627617138,-0.730500059700828,-0.696818098040978,-0.627882540733976,
-0.390114315027872,-0.343393722788442,-0.305390732344919,-0.270426232424303,
-0.230894996292773,-1.96849127237957E-5),.UNSPECIFIED.) ;
#275=B_SPLINE_CURVE_WITH_KNOTS('',3,(#37756,#37757,#37758,#37759,#37760,
#37761,#37762,#37763,#37764,#37765,#37766,#37767,#37768,#37769,#37770,#37771,
#37772,#37773,#37774,#37775,#37776,#37777,#37778,#37779,#37780,#37781,#37782,
#37783,#37784,#37785,#37786,#37787,#37788,#37789,#37790,#37791,#37792,#37793,
#37794,#37795,#37796,#37797,#37798,#37799,#37800,#37801,#37802,#37803,#37804,
#37805,#37806,#37807,#37808,#37809,#37810,#37811,#37812,#37813,#37814,#37815,
#37816,#37817,#37818,#37819,#37820,#37821,#37822,#37823,#37824,#37825,#37826,
#37827,#37828,#37829,#37830,#37831,#37832,#37833,#37834,#37835,#37836,#37837,
#37838,#37839,#37840,#37841,#37842,#37843,#37844,#37845,#37846,#37847,#37848,
#37849,#37850,#37851,#37852,#37853,#37854,#37855,#37856,#37857,#37858,#37859,
#37860,#37861,#37862,#37863,#37864,#37865,#37866,#37867,#37868,#37869,#37870,
#37871,#37872,#37873,#37874,#37875,#37876,#37877,#37878,#37879,#37880,#37881,
#37882,#37883,#37884,#37885,#37886,#37887,#37888,#37889,#37890,#37891,#37892,
#37893,#37894,#37895,#37896,#37897,#37898,#37899,#37900,#37901,#37902,#37903),
 .UNSPECIFIED.,.F.,.F.,(4,2,2,2,2,2,2,2,2,2,2,2,2,2,2,2,2,2,2,2,2,2,2,2,
2,2,2,2,2,2,2,2,2,2,2,2,2,2,2,2,2,2,2,2,2,2,2,2,2,2,2,2,2,2,2,2,2,2,2,2,
2,2,2,2,2,2,2,2,2,2,2,2,2,4),(-30.9360917508779,-30.9172686061639,-30.8923525799296,
-30.7520148786595,-30.5902087215969,-30.5487737722513,-30.5131684200696,
-30.4746533000097,-30.4207200076829,-30.1401595208009,-30.0752894875511,
-30.0431710704356,-30.034244148993,-30.030559360134,-30.0270253893342,-30.0247930648611,
-30.0234480796277,-30.0056381873835,-29.9849208811472,-29.9509450339346,
-29.8001616461514,-29.6825535715349,-29.6247809295708,-29.5852819125843,
-29.5503343290935,-29.5123662271205,-29.4565029910238,-29.2798001519611,
-29.127372093649,-29.0970176100024,-29.0770243913552,-29.0533768770667,
-29.0035447573524,-28.8098233148861,-28.7273054275376,-28.6623184632453,
-28.6221834204209,-28.5838750031023,-28.5273482769931,-28.4143021457096,
-28.2673071730302,-28.2170454955267,-28.1792760863907,-28.1577694941432,
-28.1390211672174,-28.1042164905962,-27.983621445643,-27.8440240607279,
-27.8013736683322,-27.7379011213654,-27.6984264085651,-27.6606470540911,
-27.6140179451516,-27.399599766512,-27.3142149514903,-27.2604789252421,
-27.2363937886926,-27.2165494279139,-27.1874346688687,-27.0921926598196,
-26.9605183436304,-26.8764532442066,-26.8107295661752,-26.7706516210622,
-26.7327487215632,-26.6864909734428,-26.4362394890791,-26.3900300566055,
-26.3353779971005,-26.3109960011018,-26.2910617730222,-26.2618384231154,
-26.1649960376261,-26.1634755787047),.UNSPECIFIED.) ;
#276=B_SPLINE_CURVE_WITH_KNOTS('',3,(#37906,#37907,#37908,#37909,#37910,
#37911,#37912,#37913,#37914,#37915,#37916,#37917,#37918,#37919,#37920,#37921,
#37922,#37923,#37924,#37925,#37926,#37927,#37928,#37929,#37930,#37931,#37932,
#37933,#37934,#37935,#37936,#37937,#37938,#37939,#37940,#37941,#37942,#37943,
#37944,#37945,#37946,#37947,#37948,#37949,#37950,#37951,#37952,#37953,#37954,
#37955,#37956,#37957,#37958,#37959,#37960,#37961,#37962,#37963,#37964,#37965,
#37966,#37967,#37968,#37969,#37970,#37971,#37972,#37973,#37974,#37975,#37976,
#37977,#37978,#37979,#37980,#37981,#37982,#37983,#37984,#37985,#37986,#37987,
#37988,#37989,#37990,#37991,#37992,#37993,#37994,#37995,#37996,#37997,#37998,
#37999,#38000,#38001,#38002,#38003,#38004,#38005,#38006,#38007,#38008,#38009,
#38010,#38011,#38012,#38013,#38014,#38015,#38016,#38017,#38018,#38019,#38020,
#38021,#38022,#38023,#38024,#38025,#38026,#38027,#38028,#38029,#38030,#38031,
#38032,#38033,#38034,#38035,#38036,#38037,#38038,#38039,#38040,#38041,#38042,
#38043,#38044,#38045,#38046,#38047,#38048,#38049,#38050,#38051,#38052,#38053,
#38054,#38055,#38056,#38057,#38058,#38059,#38060,#38061,#38062,#38063,#38064,
#38065,#38066,#38067,#38068,#38069,#38070,#38071,#38072,#38073,#38074,#38075,
#38076,#38077,#38078,#38079,#38080,#38081,#38082,#38083,#38084,#38085,#38086,
#38087,#38088,#38089,#38090,#38091,#38092,#38093,#38094,#38095,#38096,#38097,
#38098,#38099,#38100,#38101,#38102,#38103,#38104,#38105,#38106,#38107,#38108,
#38109,#38110,#38111,#38112,#38113,#38114,#38115,#38116,#38117,#38118,#38119,
#38120,#38121,#38122,#38123,#38124,#38125,#38126,#38127,#38128,#38129,#38130,
#38131,#38132,#38133,#38134,#38135,#38136,#38137,#38138,#38139,#38140,#38141,
#38142,#38143,#38144,#38145,#38146,#38147,#38148,#38149,#38150,#38151,#38152,
#38153,#38154,#38155,#38156,#38157,#38158,#38159,#38160,#38161,#38162,#38163,
#38164,#38165,#38166,#38167,#38168,#38169,#38170,#38171,#38172,#38173,#38174,
#38175,#38176,#38177,#38178,#38179,#38180,#38181,#38182,#38183,#38184,#38185,
#38186,#38187,#38188,#38189,#38190,#38191,#38192,#38193,#38194,#38195,#38196,
#38197,#38198,#38199,#38200,#38201,#38202,#38203,#38204,#38205,#38206,#38207,
#38208,#38209,#38210,#38211,#38212,#38213,#38214,#38215,#38216,#38217,#38218,
#38219,#38220,#38221,#38222,#38223,#38224,#38225,#38226,#38227,#38228,#38229,
#38230,#38231,#38232,#38233,#38234,#38235,#38236,#38237,#38238,#38239,#38240,
#38241,#38242,#38243,#38244,#38245,#38246,#38247,#38248,#38249,#38250,#38251,
#38252,#38253),.UNSPECIFIED.,.F.,.F.,(4,2,2,2,2,2,2,2,2,2,2,2,2,2,2,2,2,
2,2,2,2,2,2,2,2,2,2,2,2,2,2,2,2,2,2,2,2,2,2,2,2,2,2,2,2,2,2,2,2,2,2,2,2,
2,2,2,2,2,2,2,2,2,2,2,2,2,2,2,2,2,2,2,2,2,2,2,2,2,2,2,2,2,2,2,2,2,2,2,2,
2,2,2,2,2,2,2,2,2,2,2,2,2,2,2,2,2,2,2,2,2,2,2,2,2,2,2,2,2,2,2,2,2,2,2,2,
2,2,2,2,2,2,2,2,2,2,2,2,2,2,2,2,2,2,2,2,2,2,2,2,2,2,2,2,2,2,2,2,2,2,2,2,
2,2,2,2,2,2,2,2,2,2,2,2,4),(-18.7375580075198,-18.4579862149391,-18.4189665915328,
-18.3950896458485,-18.3765503519507,-18.3564393637291,-18.3307942748687,
-18.2435404331931,-18.0711070497076,-18.002110175455,-17.9473726343971,
-17.9121469745524,-17.8746723335695,-17.8194209847092,-17.6491524721797,
-17.5408669391277,-17.4975238639656,-17.466216439978,-17.4657178120353,
-17.4652033870502,-17.4646735204379,-17.4644742782827,-17.4642379308623,
-17.4514439563287,-17.4315024961516,-17.4019551080055,-17.2981709672734,
-17.0915058608801,-17.026191244316,-16.9862503614574,-16.9484199348765,
-16.9021972840528,-16.6842688407334,-16.6016590989677,-16.5489939740601,
-16.5249748299567,-16.5050232052533,-16.4753921015072,-16.3941272611813,
-16.2192353158017,-16.1713310421565,-16.1026095418212,-16.0620700389661,
-16.0241128501855,-15.9790775254471,-15.8391124156287,-15.6996396583568,
-15.6505860584727,-15.6135237322754,-15.5923039017763,-15.5708356149652,
-15.5325076210353,-15.4716811480552,-15.2938771520068,-15.2456114567767,
-15.1765461579765,-15.1359465892385,-15.0980158784726,-15.0446834466261,
-14.7992645355587,-14.7361154894136,-14.6919246450575,-14.6693481043091,
-14.6491422861336,-14.6164600620795,-14.4200521381964,-14.2779941690264,
-14.2287347246425,-14.1913198099039,-14.1489593791614,-14.0718962488988,
-14.0157724419108,-13.8533561274452,-13.8155744269607,-13.7676372195694,
-13.7443988307045,-13.7244580450334,-13.6934549235393,-13.6155297746863,
-13.4402812588759,-13.3923320717822,-13.3235676473882,-13.2830204898403,
-13.245066420483,-13.200047091984,-13.0602747993704,-12.9206195344528,-12.8715365279665,
-12.8344583063442,-12.8132352961779,-12.7944728373515,-12.7595883915594,
-12.6220963203171,-12.4934358876886,-12.4079185211845,-12.364602993916,
-12.3273239633255,-12.279618745961,-12.1674567067921,-12.0015541338996,
-11.9633925239032,-11.9151355134899,-11.891842360134,-11.8719193134874,
-11.846229077102,-11.7583416989424,-11.5864570876021,-11.5389362017157,
-11.4705808491239,-11.4301052145122,-11.3921186562034,-11.3469414307865,
-11.2104010046782,-11.0686129972136,-11.0191911391835,-10.9819306659204,
-10.960671940907,-10.9419353528719,-10.9072032009569,-10.8388377710356,
-10.7140137820564,-10.6045049784185,-10.5405651203629,-10.5008659476202,
-10.4628881492575,-10.415995008236,-10.2045122278261,-10.1189250065178,
-10.0650866756129,-10.0408829515528,-10.0209694345372,-9.99166274633418,
-9.8932218354319,-9.85210782893539,-9.71760557152259,-9.67579407772946,
-9.61309082906137,-9.57360868241256,-9.53548183038103,-9.4784518693945,
-9.36876339638761,-9.24465830736443,-9.15053143643168,-9.12150471572193,
-9.10162210812889,-9.07725134688667,-9.02232972364714,-8.93392214376293,
-8.72837701308831,-8.67568573773897,-8.63784685011571,-8.59702284837532,
-8.52667079192331,-8.43341338631384,-8.23354100927888,-8.19988798492783,
-8.18133139913975,-8.15979651614854,-8.12112799589184,-8.06905216477359,
-7.90911878531789,-7.84122831140762,-7.76847067488092,-7.72723151293331,
-7.6895395441119,-7.63792504560375,-7.46602620876009,-7.3064207474548,-7.27316757229043,
-7.2546757637246,-7.23302751088149,-7.19377779746802,-7.1405877102439,-7.07001074019559),
 .UNSPECIFIED.) ;
#277=B_SPLINE_CURVE_WITH_KNOTS('',3,(#38255,#38256,#38257,#38258,#38259,
#38260,#38261,#38262,#38263,#38264,#38265,#38266,#38267,#38268,#38269,#38270,
#38271,#38272,#38273,#38274,#38275,#38276,#38277,#38278,#38279,#38280,#38281,
#38282,#38283,#38284,#38285,#38286,#38287,#38288,#38289,#38290,#38291,#38292,
#38293,#38294,#38295,#38296,#38297,#38298,#38299,#38300,#38301,#38302,#38303,
#38304,#38305,#38306,#38307,#38308,#38309,#38310,#38311,#38312,#38313,#38314,
#38315,#38316,#38317,#38318,#38319,#38320,#38321,#38322,#38323,#38324,#38325,
#38326,#38327,#38328,#38329,#38330,#38331,#38332,#38333,#38334,#38335,#38336,
#38337,#38338,#38339,#38340,#38341,#38342,#38343,#38344,#38345,#38346,#38347,
#38348,#38349,#38350,#38351,#38352,#38353,#38354,#38355,#38356,#38357,#38358,
#38359,#38360,#38361,#38362,#38363,#38364,#38365,#38366,#38367,#38368,#38369,
#38370,#38371,#38372,#38373,#38374,#38375,#38376,#38377,#38378,#38379,#38380,
#38381,#38382,#38383,#38384,#38385,#38386,#38387,#38388,#38389,#38390,#38391,
#38392,#38393,#38394,#38395,#38396,#38397,#38398,#38399,#38400,#38401,#38402,
#38403,#38404,#38405,#38406,#38407,#38408,#38409,#38410,#38411,#38412,#38413,
#38414,#38415,#38416,#38417,#38418,#38419,#38420,#38421,#38422,#38423,#38424,
#38425,#38426,#38427,#38428,#38429,#38430,#38431,#38432,#38433,#38434,#38435,
#38436,#38437,#38438,#38439,#38440,#38441,#38442,#38443,#38444,#38445,#38446,
#38447,#38448,#38449,#38450,#38451,#38452,#38453,#38454,#38455,#38456,#38457,
#38458,#38459,#38460,#38461,#38462,#38463,#38464,#38465,#38466,#38467,#38468,
#38469,#38470,#38471,#38472,#38473,#38474,#38475,#38476,#38477,#38478,#38479,
#38480,#38481,#38482,#38483,#38484,#38485,#38486,#38487,#38488,#38489,#38490,
#38491,#38492,#38493,#38494,#38495,#38496,#38497,#38498,#38499,#38500,#38501,
#38502,#38503,#38504,#38505,#38506,#38507,#38508,#38509,#38510,#38511,#38512,
#38513,#38514,#38515,#38516,#38517,#38518,#38519,#38520,#38521,#38522,#38523,
#38524,#38525,#38526,#38527,#38528,#38529,#38530,#38531,#38532,#38533,#38534,
#38535,#38536,#38537,#38538,#38539,#38540,#38541,#38542,#38543,#38544,#38545,
#38546,#38547,#38548,#38549,#38550,#38551,#38552,#38553,#38554,#38555,#38556,
#38557,#38558,#38559,#38560,#38561,#38562,#38563,#38564,#38565,#38566,#38567,
#38568,#38569,#38570,#38571,#38572,#38573,#38574,#38575,#38576,#38577,#38578,
#38579,#38580,#38581,#38582,#38583,#38584,#38585,#38586,#38587,#38588,#38589,
#38590,#38591,#38592,#38593,#38594),.UNSPECIFIED.,.F.,.F.,(4,2,2,2,2,2,
2,2,2,2,2,2,2,2,2,2,2,2,2,2,2,2,2,2,2,2,2,2,2,2,2,2,2,2,2,2,2,2,2,2,2,2,
2,2,2,2,2,2,2,2,2,2,2,2,2,2,2,2,2,2,2,2,2,2,2,2,2,2,2,2,2,2,2,2,2,2,2,2,
2,2,2,2,2,2,2,2,2,2,2,2,2,2,2,2,2,2,2,2,2,2,2,2,2,2,2,2,2,2,2,2,2,2,2,2,
2,2,2,2,2,2,2,2,2,2,2,2,2,2,2,2,2,2,2,2,2,2,2,2,2,2,2,2,2,2,2,2,2,2,2,2,
2,2,2,2,2,2,2,2,2,2,2,2,2,2,2,2,2,2,2,4),(-26.1634755787047,-26.0334578101818,
-25.9504826045188,-25.8853926173577,-25.845512348684,-25.8076959446399,
-25.7524802596143,-25.5601565951091,-25.4664566749428,-25.4095722102639,
-25.3849267470747,-25.3651098408812,-25.3366010798324,-25.2524470344086,
-25.0778485204486,-25.0299764394409,-24.9612816156411,-24.9207429868624,
-24.8827774449592,-24.8377196036669,-24.680749271585,-24.5291081290318,
-24.47990017027,-24.4564407657557,-24.4363330047353,-24.4107237026037,-24.3247986950126,
-24.1513140492844,-24.1035878508508,-24.0350350372646,-23.994522228116,
-23.9565470107593,-23.9029335603355,-23.7800342326202,-23.7631464770853,
-23.6915944362003,-23.6082744927197,-23.5553254744775,-23.5312605194321,
-23.5113191418352,-23.4817705923174,-23.3784408919763,-23.2545749027527,
-23.1712797749366,-23.1060055837674,-23.0660737334587,-23.0282427254408,
-22.9820082805796,-22.7642624404873,-22.6815391212178,-22.6288287860635,
-22.6048036276971,-22.5848537202244,-22.5552366934647,-22.4549707926327,
-22.244644209188,-22.1794742414709,-22.139556268115,-22.1017069034204,-22.0554084880218,
-21.8389686594796,-21.7555482547361,-21.7025598368536,-21.6784878355756,
-21.6585458632077,-21.629002846757,-21.5254158127055,-21.4015473708483,
-21.3183763153513,-21.2531668134287,-21.2132443344753,-21.1754032963411,
-21.1291319650173,-20.9120770749062,-20.8289772122803,-20.7761163517607,
-20.7520663224401,-20.7321212779141,-20.7025461935975,-20.5982709956715,
-20.5751683037172,-20.4329515751015,-20.3427035642946,-20.2986821008092,
-20.2614593501161,-20.2147099154791,-20.1078032032136,-19.9354950561963,
-19.8818222480587,-19.84232239296,-19.82062539022,-19.8021596011287,-19.7690707945252,
-19.5746299471708,-19.4778269621961,-19.4437671476783,-19.3893374251967,
-19.3512414944441,-19.3109881599704,-19.2439038410166,-19.1628658358809,
-19.1298207123143,-19.0598117780832,-18.976431156369,-18.9234587075389,
-18.8993904387056,-18.8794487274373,-18.849903798898,-18.7464455849048,
-18.6225743880683,-18.5393385104102,-18.4740940557718,-18.4341644156287,
-18.3963251901799,-18.3500668533918,-18.1327488461618,-18.0498014893005,
-17.9970010415534,-17.972959813284,-17.9530120082177,-17.9234177827661,
-17.8188701633905,-17.6950080951325,-17.6123680686955,-17.5474392610172,
-17.5075650230533,-17.4696931585916,-17.4142691816239,-17.2224434605133,
-17.1290756929418,-17.0723115543148,-17.0476632564873,-17.0278239029684,
-16.9992329475797,-16.911219304383,-16.7396509046822,-16.6921700598255,
-16.6238522577736,-16.5833822121358,-16.5453911231349,-16.5001967572111,
-16.3595290896939,-16.2209117567024,-16.1719947945481,-16.1350056779493,
-16.1137995674763,-16.0950232893443,-16.0600606581171,-15.9220580798422,
-15.7938067505655,-15.7084393456323,-15.6651456164388,-15.6278626728261,
-15.5801212498485,-15.4682741747646,-15.3431173637202,-15.2403231128215,
-15.2062431753446,-15.1876157061126,-15.1661936280959,-15.128104445325,
-15.0771291151771,-14.9250567613349,-14.8138260063995,-14.7585515137222,
-14.7207029072916,-14.6807888986875,-14.6156342640823,-14.5325682072647,
-14.4958190039446),.UNSPECIFIED.) ;
#278=B_SPLINE_CURVE_WITH_KNOTS('',3,(#38600,#38601,#38602,#38603,#38604,
#38605,#38606,#38607,#38608,#38609,#38610,#38611,#38612,#38613,#38614,#38615,
#38616,#38617,#38618,#38619,#38620,#38621,#38622,#38623,#38624,#38625,#38626,
#38627,#38628,#38629,#38630,#38631,#38632,#38633,#38634,#38635,#38636,#38637,
#38638,#38639,#38640,#38641,#38642,#38643,#38644,#38645,#38646,#38647,#38648,
#38649,#38650,#38651,#38652,#38653,#38654,#38655,#38656,#38657,#38658,#38659,
#38660,#38661,#38662,#38663,#38664,#38665,#38666,#38667,#38668,#38669,#38670,
#38671,#38672,#38673,#38674,#38675,#38676,#38677,#38678,#38679,#38680,#38681,
#38682,#38683,#38684,#38685,#38686,#38687,#38688,#38689,#38690,#38691,#38692,
#38693,#38694,#38695,#38696,#38697,#38698,#38699,#38700,#38701,#38702,#38703,
#38704,#38705,#38706,#38707,#38708,#38709,#38710,#38711,#38712,#38713,#38714,
#38715,#38716,#38717,#38718,#38719,#38720,#38721,#38722,#38723,#38724,#38725,
#38726,#38727,#38728,#38729,#38730,#38731,#38732,#38733,#38734,#38735,#38736,
#38737,#38738,#38739,#38740,#38741,#38742,#38743,#38744,#38745,#38746,#38747,
#38748,#38749,#38750,#38751,#38752,#38753,#38754,#38755,#38756,#38757,#38758,
#38759,#38760,#38761,#38762,#38763,#38764,#38765,#38766,#38767,#38768,#38769,
#38770,#38771,#38772,#38773,#38774,#38775,#38776,#38777,#38778,#38779,#38780,
#38781,#38782,#38783,#38784,#38785,#38786,#38787,#38788,#38789,#38790,#38791,
#38792,#38793,#38794,#38795,#38796,#38797,#38798,#38799,#38800,#38801,#38802,
#38803,#38804,#38805,#38806,#38807,#38808,#38809,#38810,#38811,#38812,#38813,
#38814,#38815,#38816,#38817,#38818,#38819,#38820,#38821,#38822,#38823,#38824,
#38825,#38826,#38827,#38828,#38829,#38830,#38831,#38832,#38833,#38834,#38835,
#38836,#38837,#38838,#38839,#38840,#38841,#38842,#38843,#38844,#38845,#38846,
#38847,#38848,#38849,#38850,#38851,#38852,#38853,#38854,#38855,#38856,#38857,
#38858,#38859,#38860,#38861,#38862,#38863,#38864,#38865,#38866,#38867,#38868,
#38869,#38870,#38871,#38872,#38873,#38874,#38875,#38876,#38877,#38878,#38879,
#38880,#38881,#38882,#38883,#38884,#38885,#38886,#38887,#38888,#38889,#38890,
#38891,#38892,#38893,#38894,#38895,#38896,#38897,#38898,#38899,#38900,#38901,
#38902,#38903,#38904,#38905,#38906,#38907,#38908,#38909,#38910,#38911,#38912,
#38913,#38914,#38915,#38916,#38917,#38918,#38919,#38920,#38921,#38922,#38923,
#38924,#38925,#38926,#38927,#38928,#38929,#38930,#38931,#38932,#38933,#38934,
#38935,#38936,#38937,#38938,#38939,#38940,#38941,#38942,#38943,#38944,#38945,
#38946,#38947,#38948,#38949,#38950,#38951,#38952,#38953,#38954,#38955,#38956,
#38957,#38958,#38959,#38960,#38961,#38962,#38963,#38964,#38965,#38966,#38967,
#38968,#38969,#38970,#38971,#38972,#38973,#38974,#38975,#38976,#38977,#38978,
#38979,#38980,#38981,#38982,#38983,#38984,#38985,#38986,#38987,#38988,#38989,
#38990,#38991,#38992,#38993,#38994,#38995,#38996,#38997,#38998,#38999,#39000,
#39001,#39002,#39003,#39004,#39005,#39006,#39007,#39008,#39009,#39010,#39011,
#39012,#39013,#39014,#39015,#39016,#39017,#39018,#39019,#39020,#39021,#39022,
#39023,#39024,#39025,#39026,#39027,#39028,#39029,#39030,#39031,#39032,#39033,
#39034,#39035,#39036,#39037,#39038,#39039,#39040,#39041,#39042,#39043,#39044,
#39045,#39046,#39047),.UNSPECIFIED.,.F.,.F.,(4,2,2,2,2,2,2,2,2,2,2,2,2,
2,2,2,2,2,2,2,2,2,2,2,2,2,2,2,2,2,2,2,2,2,2,2,2,2,2,2,2,2,2,2,2,2,2,2,2,
2,2,2,2,2,2,2,2,2,2,2,2,2,2,2,2,2,2,2,2,2,2,2,2,2,2,2,2,2,2,2,2,2,2,2,2,
2,2,2,2,2,2,2,2,2,2,2,2,2,2,2,2,2,2,2,2,2,2,2,2,2,2,2,2,2,2,2,2,2,2,2,2,
2,2,2,2,2,2,2,2,2,2,2,2,2,2,2,2,2,2,2,2,2,2,2,2,2,2,2,2,2,2,2,2,2,2,2,2,
2,2,2,2,2,2,2,2,2,2,2,2,2,2,2,2,2,2,2,2,2,2,2,2,2,2,2,2,2,2,2,2,2,2,2,2,
2,2,2,2,2,2,2,2,2,2,2,2,2,2,2,2,2,2,2,2,2,2,2,2,2,2,2,2,2,2,4),(-11.6673889993071,
-11.6414158400702,-11.574563813691,-11.4494678783821,-11.2996368794634,
-11.2457355278412,-11.2077198576758,-11.1673044897343,-11.09929592368,-11.0521367785433,
-10.883020098933,-10.791878724752,-10.7632000319207,-10.7433526304018,-10.7187624297976,
-10.6623875084877,-10.5700847614003,-10.3719797181445,-10.3186429934542,
-10.2807109571705,-10.2401114659179,-10.1710504826137,-10.122789864657,
-9.9450344115547,-9.88371728784024,-9.84562761555956,-9.8242057096389,-9.80294122763359,
-9.76565255217539,-9.71617859054154,-9.57406061285339,-9.43787150157558,
-9.39272212907696,-9.35474086781874,-9.31425176949696,-9.24582213852396,
-9.19822399215516,-9.02574538146354,-8.93853351698104,-8.91289018339228,
-8.89277914104077,-8.86935672527111,-8.82033933013097,-8.66896001451323,
-8.52441849268399,-8.46878038716984,-8.43087566782274,-8.39105849649317,
-8.32645040204664,-8.24441196995473,-8.1392464068676,-8.11095470271037,
-8.01427096839576,-7.98492889911764,-7.96501121266049,-7.94082773342848,
-7.88712014908426,-7.80186914220275,-7.58948821901505,-7.54273746537615,
-7.50479103653867,-7.46504181575087,-7.40081894061912,-7.35750887844528,
-7.21427302371124,-7.15529565952184,-7.08298489450034,-7.05847113541836,
-7.03856328301299,-7.01432999532432,-6.96030171930695,-6.87422518718765,
-6.66409589106449,-6.6118194202079,-6.57403825712675,-6.53306024102123,
-6.46182006489084,-6.26674497875347,-6.16208775740732,-6.13248527924259,
-6.11253694301691,-6.08850145365457,-6.03573443577002,-5.95286975655572,
-5.73593068717517,-5.6894879676015,-5.6516094364336,-5.61174994372923,-5.54689951350203,
-5.46440551573931,-5.34054763232634,-5.23575780896039,-5.20614345195109,
-5.18619375261828,-5.16216504835746,-5.10944035135405,-5.02668165853167,
-4.80903328253382,-4.76279440965888,-4.72496028014888,-4.68502512561532,
-4.61974424975641,-4.53643800115724,-4.41256755889412,-4.30927179621196,
-4.27972045625702,-4.25977844870596,-4.23571483789555,-4.18276914930895,
-4.09945442821063,-4.02775996688346,-4.01153331695854,-3.88734656622141,
-3.83408553643121,-3.79616515728329,-3.75554128637079,-3.68633732835755,
-3.63792546766863,-3.45892387997426,-3.40815982734118,-3.36473450414089,
-3.34229783286455,-3.32177272874948,-3.28841027202112,-3.24601785790036,
-3.14222177441733,-2.9664581223,-2.91075932621465,-2.87284554315337,-2.8330448517961,
-2.76852779212229,-2.68665930884086,-2.58127511655769,-2.51565062616614,
-2.4495181143703,-2.42337079637734,-2.4036443268204,-2.37743220141496,-2.30894087780662,
-2.17776609758675,-2.1262685594329,-2.01854812418162,-1.97167615226222,
-1.93444879885877,-1.89052670097352,-1.80095296929998,-1.6607640988575,
-1.61024194317157,-1.53271424601636,-1.50202682426316,-1.48193460790729,
-1.46682602892255,-1.46649107583697,-1.46615059335386,-1.46580418068822,
-1.46545142230802,-1.46509188656417,-1.46472512422194,-1.46435066697454,
-1.46396802583975,-1.4635766895023,-1.46317612256954,-1.46276576371511,
-1.46234502373877,-1.46191328348857,-1.46146989169033,-1.46101416264418,
-1.46054537374701,-1.46006276290185,-1.45956552574377,-1.45905281271588,
-1.45852372593188,-1.4579773158531,-1.45741257775742,-1.4568284479894,-1.45622379995191,
-1.45559743985673,-1.4549481021682,-1.45427444480741,-1.45357504398354,
-1.45335387401897,-1.45311011695992,-1.45284129123703,-1.45254461133786,
-1.45221694541013,-1.45185476635826,-1.45145409541343,-1.45101043684475,
-1.45051870253417,-1.44997312487016,-1.44936715631,-1.44869335374756,-1.44794324588435,
-1.44710718164647,-1.44617415778365,-1.44513162420742,-1.44396526597181,
-1.44265876160541,-1.44119351879905,-1.4395483901838,-1.43769937447867,
-1.43561931224237,-1.39307777380501,-1.28858811270789,-1.11266457863325,
-1.05749935428708,-1.02810363060601,-0.998871842682495,-0.951127935374367,
-0.896784254548924,-0.792829289920703,-0.614202334992856,-0.579506851910618,
-0.560776545599971,-0.542649433513584,-0.520930955994243,-0.438846879756886,
-0.435132429627941,-0.293457525354243,-0.170016495734836,-0.122152514992153,
-0.0863789722169139,-0.0514477278305473,-2.04088515964041E-6),
 .UNSPECIFIED.) ;
#279=B_SPLINE_CURVE_WITH_KNOTS('',3,(#39048,#39049,#39050,#39051,#39052,
#39053,#39054,#39055,#39056,#39057,#39058,#39059,#39060,#39061,#39062,#39063,
#39064,#39065,#39066,#39067,#39068,#39069,#39070,#39071,#39072,#39073,#39074,
#39075,#39076,#39077,#39078,#39079,#39080,#39081,#39082,#39083,#39084,#39085,
#39086,#39087,#39088,#39089,#39090,#39091,#39092,#39093,#39094,#39095,#39096,
#39097,#39098,#39099,#39100,#39101,#39102,#39103,#39104,#39105,#39106,#39107,
#39108,#39109,#39110,#39111,#39112,#39113,#39114,#39115,#39116,#39117,#39118,
#39119,#39120,#39121,#39122,#39123,#39124,#39125,#39126,#39127,#39128,#39129,
#39130,#39131,#39132,#39133,#39134,#39135,#39136,#39137,#39138,#39139,#39140,
#39141,#39142,#39143,#39144,#39145,#39146,#39147,#39148,#39149,#39150,#39151,
#39152,#39153,#39154,#39155,#39156,#39157,#39158,#39159,#39160,#39161,#39162,
#39163,#39164,#39165,#39166,#39167,#39168,#39169,#39170,#39171,#39172,#39173,
#39174,#39175,#39176,#39177,#39178,#39179,#39180,#39181,#39182,#39183,#39184,
#39185,#39186,#39187,#39188,#39189,#39190,#39191,#39192,#39193,#39194,#39195,
#39196,#39197,#39198,#39199,#39200,#39201,#39202,#39203,#39204,#39205,#39206,
#39207,#39208,#39209,#39210,#39211,#39212,#39213,#39214,#39215,#39216,#39217,
#39218,#39219,#39220,#39221,#39222,#39223,#39224,#39225,#39226,#39227,#39228,
#39229,#39230,#39231,#39232,#39233,#39234,#39235,#39236,#39237,#39238,#39239,
#39240,#39241,#39242,#39243,#39244,#39245,#39246,#39247,#39248,#39249,#39250,
#39251,#39252,#39253,#39254,#39255,#39256,#39257,#39258,#39259,#39260,#39261,
#39262,#39263,#39264,#39265,#39266,#39267,#39268,#39269,#39270,#39271,#39272,
#39273,#39274,#39275,#39276,#39277,#39278,#39279,#39280,#39281,#39282,#39283,
#39284,#39285,#39286,#39287,#39288,#39289,#39290,#39291,#39292,#39293,#39294,
#39295,#39296,#39297,#39298,#39299,#39300,#39301,#39302,#39303,#39304,#39305,
#39306,#39307,#39308,#39309,#39310,#39311,#39312,#39313,#39314,#39315,#39316,
#39317,#39318,#39319,#39320,#39321,#39322,#39323,#39324,#39325,#39326,#39327,
#39328,#39329,#39330,#39331,#39332,#39333,#39334,#39335,#39336,#39337,#39338,
#39339,#39340,#39341,#39342,#39343,#39344,#39345,#39346,#39347,#39348,#39349,
#39350,#39351,#39352,#39353,#39354,#39355,#39356,#39357,#39358,#39359,#39360,
#39361,#39362,#39363,#39364,#39365,#39366,#39367,#39368,#39369,#39370,#39371,
#39372,#39373,#39374,#39375,#39376,#39377,#39378,#39379,#39380,#39381,#39382,
#39383),.UNSPECIFIED.,.F.,.F.,(4,2,2,2,2,2,2,2,2,2,2,2,2,2,2,2,2,2,2,2,
2,2,2,2,2,2,2,2,2,2,2,2,2,2,2,2,2,2,2,2,2,2,2,2,2,2,2,2,2,2,2,2,2,2,2,2,
2,2,2,2,2,2,2,2,2,2,2,2,2,2,2,2,2,2,2,2,2,2,2,2,2,2,2,2,2,2,2,2,2,2,2,2,
2,2,2,2,2,2,2,2,2,2,2,2,2,2,2,2,2,2,2,2,2,2,2,2,2,2,2,2,2,2,2,2,2,2,2,2,
2,2,2,2,2,2,2,2,2,2,2,2,2,2,2,2,2,2,2,2,2,2,2,2,2,2,2,2,2,2,2,2,2,2,2,2,
2,2,2,4),(-14.4958190039446,-14.3373580112747,-14.2892645766673,-14.2659988076896,
-14.2458353919106,-14.2146688434469,-14.0720874915304,-13.8858491284987,
-13.8312840022495,-13.7935440679781,-13.7534322144962,-13.6871543830497,
-13.6417767672902,-13.4853593191387,-13.3797252932852,-13.3495916421851,
-13.329575243453,-13.3058213253949,-13.2548079991878,-13.1762655815467,
-12.947765396533,-12.8986464350487,-12.8611514255218,-12.8191761917304,
-12.7420623141319,-12.4866696467823,-12.4371289540817,-12.4136182847426,
-12.3935337433925,-12.3629051488733,-12.3251885068873,-12.2413098127795,
-12.0256913649303,-11.9793452928128,-11.9414867355403,-11.9015893161373,
-11.836529715951,-11.7536432399417,-11.6297751182179,-11.5256561631738,
-11.4960899097444,-11.4761453995416,-11.4520883724604,-11.3991886383168,
-11.3159918858435,-11.0991258788283,-11.0528460253069,-11.015001960363,
-10.9750800429482,-10.9098805554953,-10.7432958967631,-10.6093683514663,
-10.5747075359722,-10.5559825690707,-10.5347057711346,-10.497355721679,
-10.4477677459395,-10.3049250258376,-10.1694961801413,-10.1244102830015,
-10.0864415013633,-10.0459224602998,-9.97732500005632,-9.92955173854313,
-9.75570691724357,-9.6702532905009,-9.64463908730002,-9.62453360736005,
-9.6010917422683,-9.55196070433939,-9.40040044806362,-9.24306493930806,
-9.19799743020723,-9.16003250290041,-9.11950526695179,-9.05086049031395,
-9.00303758733737,-8.82880065026865,-8.74391729420133,-8.7182856712044,
-8.69817673488079,-8.67474615810394,-8.62568187671633,-8.47422725134347,
-8.32983414661231,-8.27419096187223,-8.23628495157328,-8.19646817427363,
-8.13186505488578,-8.04983661421166,-7.9446543047438,-7.91632465043103,
-7.81973292762577,-7.79036065623526,-7.77043920706713,-7.74627248813241,
-7.69267397627321,-7.60770319538625,-7.39459142778028,-7.34794861107074,
-7.31002554400733,-7.27023713204597,-7.20579432265316,-7.12406588933853,
-7.01849447414561,-6.99301117600529,-6.89336047762903,-6.86398960192666,
-6.84406839667928,-6.81990107813924,-6.76629822444857,-6.68131607690297,
-6.46823527272909,-6.42158835331446,-6.38366452062368,-6.34387785454935,
-6.27944415674602,-6.1977325731074,-6.09214050287717,-6.06326256988111,
-5.96680599970245,-5.93752327798759,-5.91761225440428,-5.89339393817029,
-5.83946327651986,-5.75363919801492,-5.54280490221809,-5.49065808921857,
-5.4528943433869,-5.41186601331318,-5.34033653135174,-5.24465911125954,
-5.11984237775976,-5.05028395605779,-5.01609857056104,-4.99745380556073,
-4.97605956254654,-4.93811073441908,-4.88739977756039,-4.73713714189295,
-4.62715388854455,-4.57023292808584,-4.53212351801521,-4.49261641560508,
-4.42977225479692,-4.38782299203269,-4.25254437429793,-4.12492568549646,
-4.09021634206403,-4.07148342536188,-4.05021883608906,-4.01292952283937,
-3.96345434829835,-3.82132844087882,-3.68514808807925,-3.6399994745683,
-3.60201840653155,-3.56152904505586,-3.49309770319846,-3.44549773920924,
-3.27300476488007,-3.1858102547822,-3.1601679109962,-3.14005708743202,-3.11663409172876,
-3.06761314366686,-2.9162282990954,-2.82796833318193),.UNSPECIFIED.) ;
#280=B_SPLINE_CURVE_WITH_KNOTS('',3,(#39388,#39389,#39390,#39391,#39392,
#39393,#39394,#39395,#39396,#39397,#39398,#39399,#39400,#39401,#39402,#39403,
#39404,#39405,#39406,#39407,#39408,#39409,#39410,#39411,#39412,#39413,#39414,
#39415,#39416,#39417,#39418,#39419,#39420,#39421,#39422,#39423,#39424,#39425,
#39426,#39427,#39428,#39429,#39430,#39431,#39432,#39433,#39434,#39435,#39436,
#39437,#39438,#39439,#39440,#39441,#39442,#39443,#39444,#39445,#39446,#39447,
#39448,#39449,#39450,#39451,#39452,#39453,#39454,#39455,#39456,#39457,#39458,
#39459,#39460,#39461,#39462,#39463,#39464,#39465,#39466,#39467,#39468,#39469,
#39470,#39471,#39472,#39473,#39474,#39475,#39476,#39477,#39478,#39479,#39480,
#39481,#39482,#39483,#39484,#39485,#39486,#39487,#39488,#39489,#39490,#39491,
#39492,#39493,#39494,#39495,#39496,#39497,#39498,#39499,#39500,#39501,#39502,
#39503,#39504,#39505,#39506,#39507,#39508,#39509,#39510,#39511,#39512,#39513,
#39514,#39515,#39516,#39517,#39518,#39519,#39520,#39521,#39522,#39523,#39524,
#39525,#39526,#39527,#39528,#39529,#39530,#39531,#39532,#39533,#39534,#39535,
#39536,#39537,#39538,#39539,#39540,#39541,#39542,#39543,#39544,#39545,#39546,
#39547,#39548,#39549,#39550,#39551,#39552,#39553,#39554,#39555,#39556,#39557,
#39558,#39559,#39560,#39561,#39562,#39563,#39564,#39565,#39566,#39567,#39568,
#39569,#39570,#39571,#39572,#39573,#39574,#39575,#39576,#39577,#39578,#39579,
#39580,#39581,#39582,#39583,#39584,#39585,#39586,#39587,#39588,#39589,#39590,
#39591,#39592,#39593,#39594,#39595,#39596,#39597,#39598,#39599,#39600,#39601,
#39602,#39603,#39604,#39605,#39606,#39607,#39608,#39609,#39610,#39611,#39612,
#39613,#39614,#39615,#39616,#39617,#39618,#39619,#39620,#39621,#39622,#39623,
#39624,#39625,#39626,#39627,#39628,#39629,#39630,#39631,#39632,#39633,#39634,
#39635,#39636,#39637,#39638,#39639,#39640,#39641,#39642,#39643,#39644,#39645,
#39646,#39647,#39648,#39649,#39650,#39651,#39652,#39653,#39654,#39655,#39656,
#39657,#39658,#39659,#39660,#39661,#39662,#39663,#39664,#39665,#39666,#39667,
#39668,#39669,#39670,#39671,#39672,#39673,#39674,#39675,#39676,#39677,#39678,
#39679,#39680,#39681,#39682,#39683,#39684,#39685,#39686,#39687,#39688,#39689,
#39690,#39691,#39692,#39693,#39694,#39695,#39696,#39697,#39698,#39699,#39700,
#39701,#39702,#39703,#39704,#39705,#39706,#39707,#39708,#39709,#39710,#39711,
#39712,#39713,#39714,#39715,#39716,#39717,#39718,#39719,#39720,#39721,#39722,
#39723,#39724,#39725,#39726,#39727,#39728,#39729,#39730,#39731,#39732,#39733,
#39734,#39735,#39736,#39737,#39738,#39739,#39740,#39741,#39742,#39743,#39744,
#39745,#39746,#39747,#39748,#39749,#39750,#39751,#39752,#39753,#39754,#39755,
#39756,#39757,#39758,#39759,#39760,#39761,#39762,#39763,#39764,#39765,#39766,
#39767,#39768,#39769,#39770,#39771,#39772,#39773,#39774,#39775,#39776,#39777,
#39778,#39779),.UNSPECIFIED.,.F.,.F.,(4,2,2,2,2,2,2,2,2,2,2,2,2,2,2,2,2,
2,2,2,2,2,2,2,2,2,2,2,2,2,2,2,2,2,2,2,2,2,2,2,2,2,2,2,2,2,2,2,2,2,2,2,2,
2,2,2,2,2,2,2,2,2,2,2,2,2,2,2,2,2,2,2,2,2,2,2,2,2,2,2,2,2,2,2,2,2,2,2,2,
2,2,2,2,2,2,2,2,2,2,2,2,2,2,2,2,2,2,2,2,2,2,2,2,2,2,2,2,2,2,2,2,2,2,2,2,
2,2,2,2,2,2,2,2,2,2,2,2,2,2,2,2,2,2,2,2,2,2,2,2,2,2,2,2,2,2,2,2,2,2,2,2,
2,2,2,2,2,2,2,2,2,2,2,2,2,2,2,2,2,2,2,2,2,2,2,2,2,2,2,2,2,2,2,2,2,2,4),
(-23.3348397112233,-23.2993172367671,-23.2669907699709,-23.2311740902177,
-23.1832226642003,-23.0578285182112,-22.9159484900769,-22.9124521050827,
-22.832303470825,-22.8106450701826,-22.7924825678868,-22.7737003328901,
-22.7387000238908,-22.5603221831332,-22.4565494278997,-22.4022565325379,
-22.3545258305532,-22.3249389228639,-22.2939916884548,-22.239021017315,
-22.0760469565898,-21.9637527372471,-21.9195901089961,-21.9178419690096,
-21.916568182451,-21.9156417127412,-21.9149686193334,-21.9130725270963,
-21.9113831215892,-21.9098767733616,-21.9085325006564,-21.907331728677,
-21.9062580508492,-21.9052969994771,-21.9044358303664,-21.9036633241023,
-21.9029696051567,-21.9023459790588,-21.901784787155,-21.9012792779261,
-21.9008234936442,-21.9004121709575,-21.9000406540205,-21.8997048187409,
-21.8802652480536,-21.8662520969433,-21.84749733324,-21.8126580356763,-21.6920591698447,
-21.5522998020584,-21.4628701923475,-21.418969195433,-21.3817404211713,
-21.3348411377723,-21.2317368614652,-21.027681516855,-20.9716590136785,
-20.9471217365161,-20.9272666823625,-20.898506883662,-20.8066224826225,
-20.7793855072209,-20.6303414366049,-20.5379163061973,-20.4935845081535,
-20.4563794804764,-20.4100153315694,-20.3116036153469,-20.2930191907013,
-20.247453441294,-20.1176861630082,-20.0702541324799,-20.0340718473344,
-20.0130228466001,-19.991360001033,-19.9520332253064,-19.833261044638,-19.6975645945741,
-19.6095239728515,-19.5658277971769,-19.5285838033317,-19.4814131870597,
-19.3728146795223,-19.2028458265398,-19.1494632485972,-19.1101139362712,
-19.0884467229887,-19.0699659367477,-19.0367806247737,-18.8736215107497,
-18.7334569860586,-18.6682795218591,-18.6283624779642,-18.5905177106118,
-18.5442301628618,-18.2966978568228,-18.2320920446824,-18.1872146957074,
-18.1645139264421,-18.1443653337862,-18.1120286163427,-18.0383448332831,
-17.8619196996226,-17.8138235638719,-17.7449190549555,-17.7043471740428,
-17.6664035806144,-17.6214367948851,-17.4824571593927,-17.3420832662042,
-17.2928852187869,-17.2557449801477,-17.2345097225891,-17.2157559516563,
-17.1809231758297,-17.0664081209725,-16.9604194089774,-16.8790235539479,
-16.8147590459264,-16.7750025587324,-16.7370608076141,-16.6903309771244,
-16.4778103087671,-16.3926109482357,-16.3389235630559,-16.3147432581902,
-16.2948249833002,-16.2654775656503,-16.1688107937782,-16.1405146486189,
-16.0353487870993,-15.9533129918301,-15.888706252311,-15.8488893784422,
-15.8109845857131,-15.7553457168384,-15.610746559667,-15.4593949970142,
-15.4103959631573,-15.3869766688053,-15.3668646835359,-15.3412165793642,
-15.2539205290033,-15.0815165746579,-15.0339283242457,-14.9655081608823,
-14.92502077795,-14.8870388222489,-14.8418858525222,-14.7056531737461,-14.5635732085539,
-14.5141050458567,-14.4768195612773,-14.4555557338694,-14.4368222866574,
-14.4021098083766,-14.2746835941915,-14.1392855571267,-14.097315329346,
-14.0344497216388,-13.9949388714451,-13.9568321545062,-13.8999278188513,
-13.7932230015052,-13.7663699859351,-13.6959834222626,-13.6125862230555,
-13.5596074619825,-13.5355383153788,-13.5155969994046,-13.4860541266841,
-13.3824732918141,-13.1755593667015,-13.1102575285974,-13.0703182074741,
-13.0324854227903,-12.9862549739649,-12.7684338779628,-12.6857621677955,
-12.6330718402318,-12.6090483168674,-12.5890970462745,-12.5594720934808,
-12.4594863109513,-12.2982877355796,-12.2311402042666,-12.1749026291894,
-12.1365217343892,-12.1015045217743,-12.0421914371924,-11.941913865857,
-11.7879382633651,-11.7139919945353,-11.6871599737912,-11.6674293422724,
-11.6673889993071),.UNSPECIFIED.) ;
#281=B_SPLINE_CURVE_WITH_KNOTS('',3,(#39781,#39782,#39783,#39784,#39785,
#39786,#39787,#39788,#39789,#39790,#39791,#39792,#39793,#39794,#39795,#39796,
#39797,#39798,#39799,#39800,#39801,#39802,#39803,#39804,#39805,#39806,#39807,
#39808,#39809,#39810,#39811,#39812,#39813,#39814,#39815,#39816,#39817,#39818,
#39819,#39820,#39821,#39822,#39823,#39824,#39825,#39826,#39827,#39828,#39829,
#39830,#39831,#39832,#39833,#39834,#39835,#39836,#39837,#39838,#39839,#39840,
#39841,#39842,#39843,#39844,#39845,#39846,#39847,#39848,#39849,#39850,#39851,
#39852,#39853,#39854,#39855,#39856,#39857,#39858,#39859,#39860,#39861,#39862,
#39863,#39864,#39865,#39866,#39867,#39868,#39869,#39870,#39871,#39872,#39873,
#39874,#39875,#39876,#39877,#39878,#39879,#39880,#39881,#39882,#39883,#39884,
#39885,#39886,#39887,#39888,#39889,#39890,#39891,#39892,#39893,#39894,#39895,
#39896,#39897,#39898,#39899,#39900),.UNSPECIFIED.,.F.,.F.,(4,2,2,2,2,2,
2,2,2,2,2,2,2,2,2,2,2,2,2,2,2,2,2,2,2,2,2,2,2,2,2,2,2,2,2,2,2,2,2,2,2,2,
2,2,2,2,2,2,2,2,2,2,2,2,2,2,2,2,2,4),(-2.82796833318193,-2.77169818879921,
-2.71606011920696,-2.67815545324654,-2.63833836198687,-2.57373045869571,
-2.49169232342441,-2.38652668618395,-2.35823445383571,-2.26155274844925,
-2.23221005884666,-2.21229232822597,-2.18810927709837,-2.13440427339247,
-2.04915980214108,-1.83676235265293,-1.79001426271762,-1.75206846843233,
-1.71231840360563,-1.6480904686316,-1.60477534110728,-1.46150870661961,
-1.39838276334144,-1.32958338414609,-1.30533091289941,-1.28546182358305,
-1.27967754629077,-1.27910834204922,-1.27816310482052,-1.2773134432467,
-1.27655559111289,-1.27588483640795,-1.27529565715373,-1.27478190628782,
-1.27433702662791,-1.27395427410561,-1.27362692883975,-1.27334847788875,
-1.27311275978566,-1.27291406723207,-1.27238427551862,-1.2718699315524,
-1.27137139093596,-1.24006028294253,-1.19671105207008,-1.08839688598522,
-0.9181710735731,-0.862918002163598,-0.82544265927117,-0.790217316412342,
-0.735418657931634,-0.666372985295183,-0.49363333447154,-0.406738998577033,
-0.381111444865455,-0.3610037663698,-0.342461169469871,-0.318572664411245,
-0.279521614387501,-1.00000000635703E-6),.UNSPECIFIED.) ;
#282=B_SPLINE_CURVE_WITH_KNOTS('',3,(#39901,#39902,#39903,#39904,#39905,
#39906,#39907,#39908,#39909,#39910,#39911,#39912,#39913,#39914,#39915,#39916,
#39917,#39918,#39919,#39920,#39921,#39922,#39923,#39924,#39925,#39926,#39927,
#39928,#39929,#39930,#39931,#39932,#39933,#39934,#39935,#39936,#39937,#39938,
#39939,#39940,#39941,#39942,#39943,#39944,#39945,#39946,#39947,#39948,#39949,
#39950,#39951,#39952,#39953,#39954,#39955,#39956,#39957,#39958,#39959,#39960,
#39961,#39962,#39963,#39964,#39965,#39966,#39967,#39968,#39969,#39970,#39971,
#39972,#39973,#39974,#39975,#39976,#39977,#39978,#39979,#39980,#39981,#39982,
#39983,#39984,#39985,#39986,#39987,#39988,#39989,#39990,#39991,#39992,#39993,
#39994,#39995,#39996,#39997,#39998,#39999,#40000,#40001,#40002,#40003,#40004,
#40005,#40006,#40007,#40008,#40009,#40010,#40011,#40012,#40013,#40014,#40015,
#40016,#40017,#40018,#40019,#40020,#40021,#40022,#40023,#40024,#40025,#40026,
#40027,#40028,#40029,#40030,#40031,#40032,#40033,#40034,#40035,#40036,#40037,
#40038,#40039,#40040,#40041,#40042,#40043,#40044,#40045,#40046,#40047,#40048,
#40049,#40050,#40051,#40052,#40053,#40054,#40055,#40056,#40057,#40058,#40059,
#40060,#40061,#40062,#40063,#40064,#40065,#40066,#40067,#40068,#40069,#40070,
#40071,#40072,#40073,#40074,#40075,#40076,#40077,#40078,#40079,#40080,#40081,
#40082,#40083,#40084,#40085,#40086,#40087,#40088,#40089,#40090,#40091,#40092,
#40093,#40094,#40095,#40096,#40097,#40098,#40099,#40100,#40101,#40102,#40103,
#40104,#40105,#40106,#40107,#40108,#40109,#40110,#40111,#40112,#40113,#40114,
#40115,#40116,#40117,#40118,#40119,#40120,#40121,#40122,#40123,#40124,#40125,
#40126,#40127,#40128,#40129,#40130,#40131,#40132,#40133,#40134,#40135,#40136,
#40137,#40138,#40139,#40140,#40141,#40142,#40143,#40144,#40145,#40146,#40147,
#40148,#40149,#40150,#40151,#40152,#40153,#40154,#40155,#40156,#40157,#40158,
#40159,#40160,#40161,#40162,#40163,#40164,#40165,#40166,#40167,#40168,#40169,
#40170,#40171,#40172,#40173,#40174,#40175,#40176,#40177,#40178),
 .UNSPECIFIED.,.F.,.F.,(4,2,2,2,2,2,2,2,2,2,2,2,2,2,2,2,2,2,2,2,2,2,2,2,
2,2,2,2,2,2,2,2,2,2,2,2,2,2,2,2,2,2,2,2,2,2,2,2,2,2,2,2,2,2,2,2,2,2,2,2,
2,2,2,2,2,2,2,2,2,2,2,2,2,2,2,2,2,2,2,2,2,2,2,2,2,2,2,2,2,2,2,2,2,2,2,2,
2,2,2,2,2,2,2,2,2,2,2,2,2,2,2,2,2,2,2,2,2,2,2,2,2,2,2,2,2,2,2,2,2,2,2,2,
2,2,2,2,2,2,4),(-32.1749139758755,-32.1234445413344,-32.0885145288793,-32.0527255510178,
-32.0048303950346,-31.8809426218388,-31.73887653435,-31.6556357235931,-31.6334812934669,
-31.6153322341368,-31.5968705120142,-31.5638047818036,-31.3835735070858,
-31.2787683039668,-31.224188226212,-31.1762912027275,-31.1470066806158,
-31.1176462889212,-31.0626692938337,-30.8843551462058,-30.7812177052451,
-30.7389675472676,-30.7383270818889,-30.7363538389313,-30.7345990938568,
-30.7330371366753,-30.7316452795556,-30.7304035535523,-30.7057319756753,
-30.685212448733,-30.6627650321193,-30.6192818218547,-30.5191256613385,
-30.3755827046354,-30.332222088579,-30.2679484579597,-30.2281904562499,
-30.1902498561424,-30.1435248321897,-29.9309741851585,-29.8457868201532,
-29.7921041792333,-29.7679246649735,-29.748006312417,-29.7186577589798,
-29.6194386270037,-29.4572657456978,-29.4110567724104,-29.3439672486347,
-29.3037135243254,-29.2660470162103,-29.2119652825699,-29.0973255522735,
-29.0661791079758,-28.9384104652755,-28.8708271839429,-28.8447243360711,
-28.8269503209363,-28.8015313391385,-28.7435801251643,-28.6577803337735,
-28.5200387815974,-28.4776591623938,-28.4143767406085,-28.3747929357461,
-28.3367378210081,-28.2801519650378,-28.1725772837586,-28.1419630000505,
-27.9883740115552,-27.9379552638988,-27.9142993004938,-27.8942574170918,
-27.8689675188123,-27.7847630684693,-27.6600735992862,-27.5654110630461,
-27.4943726339059,-27.4534293484341,-27.4156351513558,-27.363265706846,
-27.1536299428732,-27.0673719562485,-27.0132733568616,-26.9890290587264,
-26.9691231505486,-26.9398850335921,-26.837587846541,-26.8116286256321,
-26.6695201160768,-26.579308637423,-26.5352931941648,-26.5018233147707,
-26.4569760599015,-26.3608175362302,-26.3054806974993,-26.1639327835766,
-26.1145483933945,-26.0773078940499,-26.0560528918878,-26.0373131455154,
-26.0025634956857,-25.9342338034163,-25.7572472695213,-25.7090814967771,
-25.6401106156737,-25.5995269377324,-25.5615881301547,-25.5166458687692,
-25.2936575456301,-25.2120228240571,-25.1597480368229,-25.1357906865815,
-25.1158245435788,-25.086078834622,-24.9837408349233,-24.8598634940935,
-24.7762838607387,-24.7108580824416,-24.6708967913419,-24.6330761684987,
-24.5779795501058,-24.3858072049656,-24.2921967120047,-24.2353448226708,
-24.210683816046,-24.1908466327638,-24.1622760018495,-24.0727358870121,
-23.9022662937596,-23.8335777406837,-23.7764342289586,-23.7379050371185,
-23.7030382873186,-23.6447052194208,-23.5384870893744,-23.3875898346536,
-23.3511393588933,-23.3353514234518),.UNSPECIFIED.) ;
#283=B_SPLINE_CURVE_WITH_KNOTS('',3,(#40183,#40184,#40185,#40186,#40187,
#40188,#40189,#40190,#40191,#40192,#40193,#40194,#40195,#40196,#40197,#40198,
#40199,#40200,#40201,#40202,#40203,#40204,#40205,#40206,#40207,#40208,#40209,
#40210,#40211,#40212,#40213,#40214,#40215,#40216,#40217,#40218,#40219,#40220,
#40221,#40222,#40223,#40224,#40225,#40226,#40227,#40228,#40229,#40230,#40231,
#40232,#40233,#40234,#40235,#40236,#40237,#40238,#40239,#40240,#40241,#40242,
#40243,#40244,#40245,#40246,#40247,#40248,#40249,#40250,#40251,#40252,#40253,
#40254,#40255,#40256,#40257,#40258,#40259,#40260,#40261,#40262,#40263,#40264,
#40265,#40266,#40267,#40268,#40269,#40270,#40271,#40272,#40273,#40274,#40275,
#40276,#40277,#40278,#40279,#40280,#40281,#40282,#40283,#40284,#40285,#40286,
#40287,#40288,#40289,#40290,#40291,#40292,#40293,#40294,#40295,#40296,#40297,
#40298,#40299,#40300,#40301,#40302,#40303,#40304,#40305,#40306,#40307,#40308,
#40309,#40310,#40311,#40312,#40313,#40314,#40315,#40316,#40317,#40318,#40319,
#40320,#40321,#40322,#40323,#40324,#40325,#40326,#40327,#40328,#40329,#40330,
#40331,#40332,#40333,#40334,#40335,#40336,#40337,#40338,#40339,#40340,#40341,
#40342,#40343,#40344,#40345,#40346,#40347,#40348,#40349,#40350,#40351,#40352,
#40353,#40354,#40355,#40356,#40357,#40358,#40359,#40360,#40361,#40362,#40363,
#40364,#40365,#40366,#40367,#40368,#40369,#40370,#40371,#40372,#40373,#40374,
#40375,#40376,#40377,#40378,#40379,#40380,#40381,#40382,#40383,#40384,#40385,
#40386,#40387,#40388,#40389,#40390,#40391,#40392,#40393,#40394,#40395,#40396,
#40397,#40398,#40399,#40400,#40401,#40402,#40403,#40404,#40405,#40406,#40407,
#40408,#40409,#40410,#40411,#40412,#40413,#40414,#40415,#40416,#40417,#40418,
#40419,#40420,#40421,#40422,#40423,#40424,#40425,#40426,#40427,#40428,#40429,
#40430,#40431,#40432,#40433,#40434,#40435,#40436,#40437,#40438,#40439,#40440,
#40441,#40442,#40443,#40444,#40445,#40446,#40447,#40448,#40449,#40450,#40451,
#40452,#40453,#40454,#40455,#40456,#40457,#40458,#40459,#40460,#40461,#40462,
#40463,#40464,#40465,#40466,#40467,#40468,#40469,#40470,#40471,#40472,#40473,
#40474,#40475,#40476,#40477,#40478,#40479,#40480,#40481,#40482,#40483,#40484,
#40485,#40486,#40487,#40488,#40489,#40490,#40491,#40492,#40493,#40494,#40495,
#40496,#40497,#40498,#40499,#40500,#40501,#40502,#40503,#40504,#40505,#40506,
#40507,#40508,#40509,#40510,#40511,#40512,#40513,#40514,#40515,#40516,#40517,
#40518,#40519,#40520,#40521,#40522,#40523,#40524,#40525,#40526,#40527,#40528),
 .UNSPECIFIED.,.F.,.F.,(4,2,2,2,2,2,2,2,2,2,2,2,2,2,2,2,2,2,2,2,2,2,2,2,
2,2,2,2,2,2,2,2,2,2,2,2,2,2,2,2,2,2,2,2,2,2,2,2,2,2,2,2,2,2,2,2,2,2,2,2,
2,2,2,2,2,2,2,2,2,2,2,2,2,2,2,2,2,2,2,2,2,2,2,2,2,2,2,2,2,2,2,2,2,2,2,2,
2,2,2,2,2,2,2,2,2,2,2,2,2,2,2,2,2,2,2,2,2,2,2,2,2,2,2,2,2,2,2,2,2,2,2,2,
2,2,2,2,2,2,2,2,2,2,2,2,2,2,2,2,2,2,2,2,2,2,2,2,2,2,2,2,2,2,2,2,2,2,2,2,
2,2,2,2,4),(-11.6678427707497,-11.6678175290612,-11.6336314550966,-11.5424990175251,
-11.51382078103,-11.4939730324175,-11.4693815468937,-11.4130004897398,-11.3206824183468,
-11.1225442412055,-11.0692274479373,-11.0312976302417,-10.990690078636,
-10.9215866936304,-10.8732819623636,-10.6951708379899,-10.6369369784023,
-10.5973211250985,-10.5756018451578,-10.5545975409668,-10.5186505341154,
-10.4716487990387,-10.3443355835049,-10.3295003766852,-10.1888194348089,
-10.1435413749685,-10.1055327949303,-10.065099664423,-9.99699344885882,
-9.94973323856204,-9.77985593358532,-9.68957805151048,-9.66097249826407,
-9.64113169951097,-9.61649282180796,-9.55979264937159,-9.46660102146701,
-9.2750055228268,-9.21935575517764,-9.181448484148,-9.14163298116555,-9.07703836113052,
-8.99502615575051,-8.88982093324299,-8.86143034680384,-8.76488264372093,
-8.73551216482047,-8.71559079382582,-8.69142271883687,-8.63781631608035,
-8.55282575248703,-8.33976089712768,-8.29311067467974,-8.25518576034033,
-8.21539954934082,-8.15097050509996,-8.06926811964727,-7.9636615432727,
-7.93259790083748,-7.83790849534589,-7.80881444329642,-7.78892414707992,
-7.76459316046365,-7.7099341459535,-7.66369143202974,-7.41212526762461,
-7.36593635765425,-7.32811219161243,-7.28815639564545,-7.22276304848743,
-7.13924501324903,-7.01536646221562,-6.9127043236503,-6.88305025245966,
-6.86309530871848,-6.8390875574717,-6.78649723896041,-6.70407638583837,
-6.48578017493408,-6.43957954906868,-6.40175299482887,-6.36180193944418,
-6.29643471577007,-6.21296597641834,-6.08908911960547,-5.98623839752679,
-5.95662722232766,-5.93667758970236,-5.91264633032177,-5.85990745317786,
-5.77711414845469,-5.55952252414827,-5.51327941410975,-5.47544382428296,
-5.4355091477315,-5.37023414558013,-5.32587148003723,-5.17610582780607,
-5.15702154995673,-5.05870275363856,-5.02963007660712,-5.00974236743992,
-4.9853991386362,-4.93065858616744,-4.88430622739851,-4.63289530046974,
-4.58673579424507,-4.54891841598725,-4.50895234253447,-4.44349799382778,
-4.35986365060906,-4.23598441835955,-4.13404710424258,-4.10416402675081,
-4.08418071905752,-4.06029746899842,-4.00848367057867,-3.92798804788365,
-3.70299751181169,-3.653736982684,-3.61622618653403,-3.5743260164386,-3.49765864507666,
-3.44097870517749,-3.33363210772645,-3.31887184001726,-3.21604777308864,
-3.18196655315214,-3.1633392903041,-3.14191851702691,-3.10383372051061,
-3.05286600650788,-2.90083989264133,-2.78937452912237,-2.73418605816945,
-2.69635170776026,-2.65641625503964,-2.59113472775737,-2.50782750601567,
-2.38395625577425,-2.28066084122462,-2.2511092441252,-2.23116709993902,
-2.20710337112163,-2.1541575766174,-2.07084291212987,-1.85420212691175,
-1.80791403531042,-1.77006921177343,-1.73015249992359,-1.66497661967465,
-1.46380943584966,-1.36307276819266,-1.32913323091078,-1.31052951300075,
-1.29228857727534,-1.27033953391371,-1.23657942584488,-1.16728479137407,
-0.927790949628409,-0.87737059778315,-0.840365950065773,-0.803100134060258,
-0.761758184915453,-0.621177597732689,-0.445029393994813,-0.406453413416984,
-0.384936587192776,-0.366763387244894,-0.345122971337476,-0.312200863253871,
-0.245779091502141,-1.00000000458067E-6),.UNSPECIFIED.) ;
#284=B_SPLINE_CURVE_WITH_KNOTS('',3,(#40529,#40530,#40531,#40532,#40533,
#40534,#40535,#40536,#40537,#40538,#40539,#40540,#40541,#40542,#40543,#40544,
#40545,#40546,#40547,#40548,#40549,#40550,#40551,#40552,#40553,#40554,#40555,
#40556,#40557,#40558,#40559,#40560,#40561,#40562,#40563,#40564,#40565,#40566,
#40567,#40568,#40569,#40570,#40571,#40572,#40573,#40574,#40575,#40576,#40577,
#40578,#40579,#40580,#40581,#40582,#40583,#40584,#40585,#40586,#40587,#40588,
#40589,#40590,#40591,#40592,#40593,#40594,#40595,#40596,#40597,#40598,#40599,
#40600,#40601,#40602,#40603,#40604,#40605,#40606,#40607,#40608,#40609,#40610,
#40611,#40612,#40613,#40614,#40615,#40616,#40617,#40618,#40619,#40620,#40621,
#40622,#40623,#40624,#40625,#40626,#40627,#40628,#40629,#40630,#40631,#40632,
#40633,#40634,#40635,#40636,#40637,#40638,#40639,#40640,#40641,#40642,#40643,
#40644,#40645,#40646,#40647,#40648,#40649,#40650,#40651,#40652,#40653,#40654,
#40655,#40656,#40657,#40658,#40659,#40660,#40661,#40662,#40663,#40664,#40665,
#40666,#40667,#40668,#40669,#40670,#40671,#40672,#40673,#40674,#40675,#40676,
#40677,#40678,#40679,#40680,#40681,#40682,#40683,#40684,#40685,#40686,#40687,
#40688,#40689,#40690,#40691,#40692,#40693,#40694,#40695,#40696,#40697,#40698,
#40699,#40700,#40701,#40702,#40703,#40704,#40705,#40706,#40707,#40708,#40709,
#40710,#40711,#40712,#40713,#40714,#40715,#40716,#40717,#40718,#40719,#40720,
#40721,#40722,#40723,#40724,#40725,#40726,#40727,#40728,#40729,#40730,#40731,
#40732,#40733,#40734,#40735,#40736,#40737,#40738,#40739,#40740,#40741,#40742,
#40743,#40744,#40745,#40746,#40747,#40748,#40749,#40750,#40751,#40752,#40753,
#40754,#40755,#40756,#40757,#40758,#40759,#40760,#40761,#40762,#40763,#40764,
#40765,#40766,#40767,#40768,#40769,#40770,#40771,#40772,#40773,#40774,#40775,
#40776,#40777,#40778,#40779,#40780,#40781,#40782,#40783,#40784,#40785,#40786,
#40787,#40788,#40789,#40790,#40791,#40792,#40793,#40794,#40795,#40796,#40797,
#40798,#40799,#40800,#40801,#40802,#40803,#40804,#40805,#40806,#40807,#40808,
#40809,#40810,#40811,#40812,#40813,#40814,#40815,#40816,#40817,#40818,#40819,
#40820,#40821,#40822,#40823,#40824,#40825,#40826,#40827,#40828,#40829,#40830,
#40831,#40832,#40833,#40834,#40835,#40836,#40837,#40838,#40839,#40840,#40841,
#40842,#40843,#40844,#40845,#40846,#40847,#40848,#40849,#40850,#40851,#40852,
#40853,#40854,#40855,#40856,#40857,#40858,#40859,#40860,#40861,#40862,#40863,
#40864,#40865,#40866,#40867,#40868),.UNSPECIFIED.,.F.,.F.,(4,2,2,2,2,2,
2,2,2,2,2,2,2,2,2,2,2,2,2,2,2,2,2,2,2,2,2,2,2,2,2,2,2,2,2,2,2,2,2,2,2,2,
2,2,2,2,2,2,2,2,2,2,2,2,2,2,2,2,2,2,2,2,2,2,2,2,2,2,2,2,2,2,2,2,2,2,2,2,
2,2,2,2,2,2,2,2,2,2,2,2,2,2,2,2,2,2,2,2,2,2,2,2,2,2,2,2,2,2,2,2,2,2,2,2,
2,2,2,2,2,2,2,2,2,2,2,2,2,2,2,2,2,2,2,2,2,2,2,2,2,2,2,2,2,2,2,2,2,2,2,2,
2,2,2,2,2,2,2,2,2,2,2,2,2,2,2,2,2,2,2,4),(-23.3353514234518,-23.304336453575,
-23.281294079642,-23.2612840850882,-23.229821444945,-23.1541190155707,-22.977897528171,
-22.9298262389341,-22.8609449829051,-22.8203766943299,-22.7824305977091,
-22.7374538524634,-22.5983246910093,-22.4580803357955,-22.4089024897131,
-22.3717729443308,-22.3505395482959,-22.3317838523465,-22.2969410096231,
-22.1765810732244,-22.0366597186924,-21.9471746377961,-21.9032647347992,
-21.8660355302898,-21.8191451233293,-21.7164608524388,-21.5120261802275,
-21.4559473848375,-21.4314012607999,-21.4115469685829,-21.3827992814526,
-21.2992958957657,-21.0816728163509,-21.0101544844516,-20.9691278405556,
-20.9313630355502,-20.8792104609235,-20.6683991293658,-20.5825633677076,
-20.5286280051641,-20.5044088132735,-20.4844977395687,-20.4599653856239,
-20.3875328247002,-20.1441231857728,-20.0788220747043,-20.0388825825197,
-20.0010492585766,-19.9548176682012,-19.7370054663383,-19.6543268760753,
-19.6016335952436,-19.5776094383401,-19.5576580422244,-19.528033468963,
-19.4280228110715,-19.2668385347409,-19.2207690814492,-19.1538148733074,
-19.1135843371879,-19.0759052612154,-19.0304024690919,-18.9016097494586,
-18.7545389997685,-18.70430236801,-18.6666057156846,-18.6452608895655,-18.6239206275512,
-18.5862471877911,-18.5240761343268,-18.3464164134873,-18.2981674523852,
-18.2291172121456,-18.1885192579184,-18.1505858694052,-18.1056723658765,
-17.9675279960662,-17.8263953691815,-17.7553917397604,-17.7288856825717,
-17.709159565226,-17.6832971146946,-17.6343960574231,-17.5505491160553,
-17.4446689283901,-17.3631835310849,-17.2988705962436,-17.2591049536508,
-17.2211675349858,-17.1744600877133,-16.9617799636402,-16.8766381582123,
-16.8229727789355,-16.7987955566402,-16.7788761186885,-16.7495217937295,
-16.6502024839808,-16.4881035471758,-16.4419044104947,-16.3748238887758,
-16.3345710224327,-16.2969026386361,-16.2514521025166,-16.1203438919195,
-16.0873458892449,-15.9146317727454,-15.8826212314254,-15.8625251603367,
-15.8397009874527,-15.7941362623971,-15.7591093759334,-15.6194755139688,
-15.4796741021172,-15.4346514637233,-15.396695768019,-15.3561481123711,
-15.287386297156,-15.2394406118933,-15.0642288413577,-14.9858793657378,
-14.9550511939247,-14.9349380919672,-14.9115208804347,-14.8625356897023,
-14.7112061105873,-14.5665648564298,-14.5109240705266,-14.4730184917753,
-14.4332011979365,-14.3685948388047,-14.2865602505239,-14.181386408875,
-14.1530778828282,-14.0564409906452,-14.0270820511801,-14.0071621733911,
-13.9829878372708,-13.9293403680683,-13.8442441936181,-13.6314536771025,
-13.5847637994324,-13.5468304089743,-13.5070588478134,-13.4427114666762,
-13.3992777944032,-13.2552948477284,-13.228538501451,-13.1299692058251,
-13.1006549069615,-13.0807402262999,-13.0565401821588,-13.0027273818341,
-12.917206832101,-12.7055402023887,-12.6586759385115,-12.6207040346553,
-12.5809938094974,-12.5169942859756,-12.4071733459207,-12.2102847793757,
-12.1776937999183,-12.1575029135442,-12.1348934026794,-12.0905227261423,
-12.0269946598089,-11.8389652654348,-11.7544461169129,-11.711283458406,
-11.6743418796539,-11.6675240120961),.UNSPECIFIED.) ;
#285=B_SPLINE_CURVE_WITH_KNOTS('',3,(#40873,#40874,#40875,#40876,#40877,
#40878,#40879,#40880,#40881,#40882,#40883,#40884,#40885,#40886,#40887,#40888,
#40889,#40890,#40891,#40892,#40893,#40894,#40895,#40896,#40897,#40898,#40899,
#40900,#40901,#40902,#40903,#40904,#40905,#40906,#40907,#40908,#40909,#40910,
#40911,#40912,#40913,#40914,#40915,#40916,#40917,#40918,#40919,#40920,#40921,
#40922,#40923,#40924,#40925,#40926,#40927,#40928,#40929,#40930,#40931,#40932,
#40933,#40934,#40935,#40936,#40937,#40938,#40939,#40940,#40941,#40942,#40943,
#40944,#40945,#40946,#40947,#40948,#40949,#40950,#40951,#40952,#40953,#40954,
#40955,#40956,#40957,#40958,#40959,#40960,#40961,#40962,#40963,#40964,#40965,
#40966,#40967,#40968,#40969,#40970,#40971,#40972,#40973,#40974,#40975,#40976,
#40977,#40978,#40979,#40980,#40981,#40982,#40983,#40984,#40985,#40986,#40987,
#40988,#40989,#40990,#40991,#40992,#40993,#40994,#40995,#40996,#40997,#40998,
#40999,#41000,#41001,#41002,#41003,#41004,#41005,#41006,#41007,#41008,#41009,
#41010,#41011,#41012,#41013,#41014,#41015,#41016,#41017,#41018,#41019,#41020,
#41021,#41022,#41023,#41024,#41025,#41026,#41027,#41028,#41029,#41030,#41031,
#41032,#41033,#41034,#41035,#41036,#41037,#41038,#41039,#41040,#41041,#41042,
#41043,#41044,#41045,#41046,#41047,#41048,#41049,#41050,#41051,#41052,#41053,
#41054,#41055,#41056,#41057,#41058,#41059,#41060,#41061,#41062,#41063,#41064,
#41065,#41066,#41067,#41068,#41069,#41070,#41071,#41072,#41073,#41074,#41075,
#41076,#41077,#41078,#41079,#41080,#41081,#41082,#41083,#41084,#41085,#41086,
#41087,#41088,#41089,#41090,#41091,#41092,#41093,#41094,#41095,#41096,#41097,
#41098,#41099,#41100,#41101,#41102,#41103,#41104,#41105,#41106,#41107,#41108,
#41109,#41110,#41111,#41112,#41113,#41114,#41115,#41116,#41117,#41118,#41119,
#41120,#41121,#41122,#41123,#41124,#41125,#41126,#41127,#41128,#41129,#41130,
#41131,#41132,#41133,#41134,#41135,#41136,#41137,#41138,#41139,#41140,#41141,
#41142,#41143,#41144,#41145,#41146,#41147,#41148,#41149,#41150,#41151,#41152,
#41153,#41154,#41155,#41156,#41157,#41158,#41159,#41160,#41161,#41162,#41163,
#41164,#41165,#41166,#41167,#41168,#41169,#41170,#41171,#41172,#41173,#41174,
#41175,#41176,#41177,#41178,#41179,#41180,#41181,#41182,#41183,#41184,#41185,
#41186,#41187,#41188,#41189,#41190,#41191,#41192,#41193,#41194,#41195,#41196,
#41197,#41198,#41199,#41200,#41201,#41202,#41203,#41204,#41205,#41206,#41207,
#41208,#41209,#41210,#41211,#41212,#41213,#41214,#41215,#41216,#41217,#41218,
#41219,#41220,#41221,#41222,#41223,#41224,#41225,#41226,#41227,#41228,#41229,
#41230,#41231,#41232,#41233,#41234,#41235,#41236,#41237,#41238,#41239,#41240),
 .UNSPECIFIED.,.F.,.F.,(4,2,2,2,2,2,2,2,2,2,2,2,2,2,2,2,2,2,2,2,2,2,2,2,
2,2,2,2,2,2,2,2,2,2,2,2,2,2,2,2,2,2,2,2,2,2,2,2,2,2,2,2,2,2,2,2,2,2,2,2,
2,2,2,2,2,2,2,2,2,2,2,2,2,2,2,2,2,2,2,2,2,2,2,2,2,2,2,2,2,2,2,2,2,2,2,2,
2,2,2,2,2,2,2,2,2,2,2,2,2,2,2,2,2,2,2,2,2,2,2,2,2,2,2,2,2,2,2,2,2,2,2,2,
2,2,2,2,2,2,2,2,2,2,2,2,2,2,2,2,2,2,2,2,2,2,2,2,2,2,2,2,2,2,2,2,2,2,2,2,
2,2,2,2,2,2,2,2,2,2,2,2,2,2,2,4),(-23.3356224284091,-23.1752910327308,-23.1316004967274,
-23.0963736709529,-23.0591486217279,-23.0123353436188,-22.9106695363059,
-22.8968366236876,-22.829460335953,-22.7154050385202,-22.6527838974531,
-22.6502910072541,-22.6483669204974,-22.6468396735258,-22.6455953700816,
-22.6445568376552,-22.6436704743946,-22.642898083557,-22.6422117177883,
-22.6415903506155,-22.641017669718,-22.6404805653369,-22.639968048979,-22.6233708392609,
-22.6034050406333,-22.5736620172565,-22.4681488137098,-22.3110706125266,
-22.2446510118568,-22.1924312768605,-22.1591672125633,-22.1214468788745,
-22.0757448693712,-21.852652184604,-21.7723994397085,-21.7206842785241,
-21.6968167216298,-21.676829288011,-21.6469156172914,-21.5411988871072,
-21.3371071938026,-21.2718599740503,-21.231930083881,-21.1940915042348,
-21.1478350896097,-20.9304875416017,-20.8475579134906,-20.7947646885645,
-20.7707247477425,-20.7507769061461,-20.7211810756207,-20.6166100158651,
-20.4927492977278,-20.4101241445086,-20.3452034357598,-20.305330903538,
-20.2674586402655,-20.2210476816895,-20.0061876026044,-19.9219374250095,
-19.8841264053389,-19.8534416545061,-19.8333493391444,-19.8098657015225,
-19.7604851009467,-19.5663838114834,-19.4837408746199,-19.4188107775557,
-19.3789366685353,-19.3410655011596,-19.2946592305909,-19.0797556479186,
-18.9955260509616,-18.9422183284378,-18.9180972046655,-18.8981665403129,
-18.8687148877574,-18.760886463944,-18.605002188652,-18.5597042151212,-18.4935048224512,
-18.4534071115013,-18.4156604272277,-18.3610485514088,-18.2479329730214,
-18.0961873250121,-18.0452593272866,-18.0071953634659,-17.9857783572679,
-17.9671479237223,-17.9330494845069,-17.8299930382376,-17.8155501407971,
-17.6727746622876,-17.6295407314629,-17.5653940078109,-17.5256576707772,
-17.4877019370155,-17.4409114754964,-17.3165702342082,-17.1449489384995,
-17.0901507259142,-17.0657984303569,-17.0459119808705,-17.0168532591001,
-16.9194146268465,-16.8913393696762,-16.7863228085223,-16.7041704285616,
-16.6395011227664,-16.5996726790366,-16.5617736885086,-16.5061754583293,
-16.3145305336669,-16.2212961331576,-16.1645805521732,-16.1399394985055,
-16.1200991742111,-16.0914974017609,-16.0012744793912,-15.9611054693506,
-15.8194922398149,-15.7764522341081,-15.7125007195857,-15.6727985114528,
-15.6348204659372,-15.58793050243,-15.3764110668331,-15.2510581494459,-15.2209530159252,
-15.2009404123223,-15.1771719402775,-15.1260692815802,-15.0897247834949,
-14.9087052186348,-14.8600504736467,-14.8272824585023,-14.7742974318444,
-14.7364157470234,-14.6956943939728,-14.6259378508564,-14.5511590725254,
-14.3925642374133,-14.3552103295018,-14.3076347380174,-14.2844580112734,
-14.2644954456196,-14.2333484987246,-14.1557598209334,-13.9804683780983,
-13.9325128277285,-13.8637414695466,-13.8231920245191,-13.7852368628706,
-13.7317466302716,-13.6121153731153,-13.4634711540442,-13.4272952331865,
-13.3807289011451,-13.3577277014064,-13.3377018792542,-13.306137865739,
-13.1288631944879,-13.0206247346011,-12.9433266888803,-12.9013208071003,
-12.8638324018811,-12.8147714037803,-12.6793344274383,-12.6665414627295,
-12.5937503995926,-12.5104432089797,-12.457499674592,-12.4334357262163,
-12.4134927114653,-12.3839388680023,-12.2800487751444,-12.1561803460734,
-12.0731681060141,-12.008041786093,-11.9681326365893,-11.9302809200484,
-11.8839663264008,-11.6678427707497),.UNSPECIFIED.) ;
#286=B_SPLINE_CURVE_WITH_KNOTS('',3,(#41241,#41242,#41243,#41244,#41245,
#41246,#41247,#41248,#41249,#41250,#41251,#41252,#41253,#41254,#41255,#41256,
#41257,#41258,#41259,#41260,#41261,#41262,#41263,#41264,#41265,#41266,#41267,
#41268,#41269,#41270,#41271,#41272,#41273,#41274,#41275,#41276,#41277,#41278,
#41279,#41280,#41281,#41282,#41283,#41284,#41285,#41286,#41287,#41288,#41289,
#41290,#41291,#41292,#41293,#41294,#41295,#41296,#41297,#41298,#41299,#41300,
#41301,#41302,#41303,#41304,#41305,#41306,#41307,#41308,#41309,#41310,#41311,
#41312,#41313,#41314,#41315,#41316,#41317,#41318,#41319,#41320,#41321,#41322,
#41323,#41324,#41325,#41326,#41327,#41328,#41329,#41330,#41331,#41332,#41333,
#41334,#41335,#41336,#41337,#41338,#41339,#41340,#41341,#41342,#41343,#41344,
#41345,#41346,#41347,#41348,#41349,#41350,#41351,#41352,#41353,#41354,#41355,
#41356,#41357,#41358,#41359,#41360,#41361,#41362,#41363,#41364,#41365,#41366,
#41367,#41368,#41369,#41370,#41371,#41372,#41373,#41374,#41375,#41376,#41377,
#41378,#41379,#41380,#41381,#41382,#41383,#41384,#41385,#41386,#41387,#41388,
#41389,#41390,#41391,#41392,#41393,#41394,#41395,#41396,#41397,#41398,#41399,
#41400,#41401,#41402,#41403,#41404,#41405,#41406,#41407,#41408,#41409,#41410,
#41411,#41412,#41413,#41414,#41415,#41416,#41417,#41418,#41419,#41420,#41421,
#41422,#41423,#41424,#41425,#41426,#41427,#41428,#41429,#41430,#41431,#41432,
#41433,#41434,#41435,#41436,#41437,#41438,#41439,#41440,#41441,#41442,#41443,
#41444,#41445,#41446,#41447,#41448,#41449,#41450,#41451,#41452,#41453,#41454,
#41455,#41456,#41457,#41458,#41459,#41460,#41461,#41462,#41463,#41464,#41465,
#41466,#41467,#41468,#41469,#41470,#41471,#41472,#41473,#41474,#41475,#41476,
#41477,#41478,#41479,#41480,#41481,#41482,#41483,#41484,#41485,#41486,#41487,
#41488,#41489,#41490,#41491,#41492,#41493,#41494,#41495,#41496,#41497,#41498,
#41499,#41500,#41501,#41502,#41503,#41504,#41505,#41506,#41507,#41508,#41509,
#41510,#41511,#41512,#41513,#41514,#41515,#41516,#41517,#41518,#41519,#41520,
#41521,#41522,#41523,#41524,#41525,#41526,#41527,#41528,#41529,#41530,#41531,
#41532,#41533,#41534,#41535,#41536,#41537,#41538,#41539,#41540,#41541,#41542,
#41543,#41544,#41545,#41546,#41547,#41548,#41549,#41550,#41551,#41552,#41553,
#41554,#41555,#41556,#41557,#41558,#41559,#41560,#41561,#41562,#41563,#41564,
#41565,#41566,#41567,#41568,#41569,#41570,#41571,#41572,#41573,#41574,#41575,
#41576,#41577,#41578,#41579,#41580,#41581,#41582,#41583,#41584,#41585,#41586,
#41587,#41588,#41589,#41590,#41591,#41592,#41593,#41594,#41595,#41596,#41597,
#41598,#41599,#41600,#41601,#41602,#41603,#41604,#41605,#41606,#41607,#41608,
#41609,#41610,#41611,#41612,#41613,#41614,#41615,#41616),.UNSPECIFIED.,
 .F.,.F.,(4,2,2,2,2,2,2,2,2,2,2,2,2,2,2,2,2,2,2,2,2,2,2,2,2,2,2,2,2,2,2,
2,2,2,2,2,2,2,2,2,2,2,2,2,2,2,2,2,2,2,2,2,2,2,2,2,2,2,2,2,2,2,2,2,2,2,2,
2,2,2,2,2,2,2,2,2,2,2,2,2,2,2,2,2,2,2,2,2,2,2,2,2,2,2,2,2,2,2,2,2,2,2,2,
2,2,2,2,2,2,2,2,2,2,2,2,2,2,2,2,2,2,2,2,2,2,2,2,2,2,2,2,2,2,2,2,2,2,2,2,
2,2,2,2,2,2,2,2,2,2,2,2,2,2,2,2,2,2,2,2,2,2,2,2,2,2,2,2,2,2,2,2,2,2,2,2,
2,2,2,2,2,2,2,2,2,2,2,2,4),(-11.6675240120961,-11.626614261062,-11.5049066428377,
-11.3810336064293,-11.2777209614977,-11.2481698993271,-11.2282275661209,
-11.2041629116592,-11.1512127953789,-11.0678880142526,-10.9967659838497,
-10.977751297978,-10.8499086117722,-10.8041375398596,-10.7664026992862,
-10.7262834839868,-10.6599603784825,-10.6145361677103,-10.4578007729936,
-10.3520937954821,-10.3222118954192,-10.3022286112759,-10.2783444258485,
-10.2265255765459,-10.1460179022355,-9.92104580533755,-9.87178409363482,
-9.83427290890201,-9.79237281908231,-9.71570730203895,-9.65902977923404,
-9.55167974144845,-9.53689295720504,-9.43408751358441,-9.40000741883825,
-9.38138024151623,-9.35995893963465,-9.32187200628127,-9.27090042167162,
-9.11884914963252,-9.00752064757142,-8.95228302574212,-8.91444083486559,
-8.87451822236405,-8.80931087495381,-8.72614425572813,-8.60227479504981,
-8.49867645786069,-8.46913362584126,-8.44919240456902,-8.4251234477171,
-8.37214533693766,-8.28874956921323,-8.21836199001807,-8.19154616899052,
-8.08468912089318,-8.0278417951736,-7.98974446150653,-7.95022092751081,
-7.88728221260635,-7.84524019312781,-7.70943455738341,-7.64748291069781,
-7.60182199900407,-7.55571338915206,-7.53279313130586,-7.51249899088974,
-7.48049690347562,-7.45932726468103,-7.39645619054944,-7.14385659417263,
-7.09832078990359,-7.06063546462461,-7.02042004895647,-6.95354844654136,
-6.90756323880015,-6.7469677099623,-6.64607943621641,-6.61648311801943,
-6.59653550494772,-6.57249653672232,-6.51970770671173,-6.43678831565594,
-6.21987280606089,-6.17345337947077,-6.13557988886499,-6.09571174864011,
-6.03081244115732,-5.94822653317546,-5.8243673140553,-5.71973179984141,
-5.69013120920131,-5.67018315733077,-5.6461467582124,-5.59337366596395,
-5.51049356779011,-5.29429626749042,-5.24758346204922,-5.20964571598462,
-5.16988371332307,-5.10558650251306,-5.02412910350441,-4.91821717895962,
-4.82759925792647,-4.77828363620081,-4.75481130912595,-4.7347162726686,
-4.70400959377336,-4.66616154134513,-4.58176361132367,-4.36725077541677,
-4.32080295046152,-4.28292339972129,-4.24306597573255,-4.17822674347864,
-4.09575367539922,-3.97189645241117,-3.86707273230806,-3.83745510444977,
-3.81750506333563,-3.79347831068277,-3.74076558260037,-3.65803674921595,
-3.44033417820391,-3.39409851502524,-3.35626517413593,-3.3163290030225,
-3.25104180351796,-2.99795430518477,-2.93294312668903,-2.90697357423404,
-2.88724827418492,-2.86085582917944,-2.79083463512742,-2.65369318337073,
-2.51180083625297,-2.46635287345153,-2.42868599869819,-2.38843410048223,
-2.32135355339895,-2.27515356203339,-2.11304433646482,-2.01374467084728,
-1.98439211488226,-1.96447345391899,-1.94029662431368,-1.88663023856808,
-1.80148409268042,-1.58883537611954,-1.54212652776392,-1.50418975191282,
-1.46897020179996,-1.4667986765337,-1.46461856627264,-1.46239741478584,
-1.46010269786793,-1.45770010998939,-1.45515187655848,-1.45241493705354,
-1.44943886143034,-1.44616336709126,-1.44251530824729,-1.43840502985344,
-1.43372204246142,-1.42833013370374,-1.36985256116618,-1.25016199999906,
-1.09631907853567,-1.06253542577883,-1.04395749049124,-1.02997228115826,
-1.00120584322775,-0.965459138600484,-0.889063567284749,-0.669843809898982,
-0.614806598336588,-0.576995909451253,-0.542128550249746,-0.520825383229167,
-0.499904143437578,-0.449780354056626,-0.30945191890729,-0.171121419916737,
-0.136721806125387,-0.118041454839647,-0.0999484447591764,-0.0781695906212831,
-1.00000000660683E-6),.UNSPECIFIED.) ;
#287=B_SPLINE_CURVE_WITH_KNOTS('',3,(#41621,#41622,#41623,#41624,#41625,
#41626,#41627,#41628,#41629,#41630,#41631,#41632,#41633,#41634,#41635,#41636,
#41637,#41638,#41639,#41640,#41641,#41642,#41643,#41644,#41645,#41646,#41647,
#41648,#41649,#41650,#41651,#41652,#41653,#41654,#41655,#41656,#41657,#41658,
#41659,#41660,#41661,#41662,#41663,#41664,#41665,#41666,#41667,#41668,#41669,
#41670,#41671,#41672,#41673,#41674,#41675,#41676,#41677,#41678,#41679,#41680,
#41681,#41682,#41683,#41684,#41685,#41686,#41687,#41688,#41689,#41690,#41691,
#41692,#41693,#41694,#41695,#41696,#41697,#41698,#41699,#41700,#41701,#41702,
#41703,#41704,#41705,#41706,#41707,#41708,#41709,#41710,#41711,#41712,#41713,
#41714,#41715,#41716,#41717,#41718,#41719,#41720,#41721,#41722,#41723,#41724,
#41725,#41726,#41727,#41728,#41729,#41730,#41731,#41732,#41733,#41734,#41735,
#41736,#41737,#41738,#41739,#41740,#41741,#41742,#41743,#41744,#41745,#41746,
#41747,#41748,#41749,#41750,#41751,#41752,#41753,#41754,#41755,#41756,#41757,
#41758,#41759,#41760,#41761,#41762,#41763,#41764,#41765,#41766,#41767,#41768,
#41769,#41770,#41771,#41772,#41773,#41774,#41775,#41776,#41777,#41778,#41779,
#41780,#41781,#41782,#41783,#41784,#41785,#41786,#41787,#41788,#41789,#41790,
#41791,#41792,#41793,#41794,#41795,#41796,#41797,#41798,#41799,#41800,#41801,
#41802,#41803,#41804,#41805,#41806,#41807,#41808,#41809,#41810,#41811,#41812,
#41813,#41814,#41815,#41816,#41817,#41818,#41819,#41820,#41821,#41822,#41823,
#41824,#41825,#41826,#41827,#41828,#41829,#41830,#41831,#41832,#41833,#41834,
#41835,#41836,#41837,#41838,#41839,#41840,#41841,#41842,#41843,#41844,#41845,
#41846,#41847,#41848,#41849,#41850,#41851,#41852,#41853,#41854,#41855,#41856,
#41857,#41858,#41859,#41860,#41861,#41862,#41863,#41864,#41865,#41866,#41867,
#41868,#41869,#41870,#41871,#41872,#41873,#41874,#41875,#41876,#41877,#41878,
#41879,#41880,#41881,#41882,#41883,#41884,#41885,#41886,#41887,#41888,#41889,
#41890,#41891,#41892,#41893,#41894,#41895,#41896,#41897,#41898,#41899,#41900,
#41901,#41902,#41903,#41904,#41905,#41906,#41907,#41908,#41909,#41910,#41911,
#41912,#41913,#41914,#41915,#41916,#41917,#41918,#41919,#41920,#41921,#41922,
#41923,#41924,#41925,#41926,#41927,#41928,#41929,#41930,#41931,#41932,#41933,
#41934,#41935,#41936,#41937,#41938,#41939,#41940,#41941,#41942,#41943,#41944,
#41945,#41946,#41947,#41948,#41949,#41950,#41951,#41952,#41953,#41954,#41955,
#41956,#41957,#41958,#41959,#41960,#41961,#41962,#41963,#41964,#41965,#41966,
#41967,#41968,#41969,#41970,#41971,#41972,#41973,#41974,#41975,#41976,#41977,
#41978,#41979,#41980,#41981,#41982),.UNSPECIFIED.,.F.,.F.,(4,2,2,2,2,2,
2,2,2,2,2,2,2,2,2,2,2,2,2,2,2,2,2,2,2,2,2,2,2,2,2,2,2,2,2,2,2,2,2,2,2,2,
2,2,2,2,2,2,2,2,2,2,2,2,2,2,2,2,2,2,2,2,2,2,2,2,2,2,2,2,2,2,2,2,2,2,2,2,
2,2,2,2,2,2,2,2,2,2,2,2,2,2,2,2,2,2,2,2,2,2,2,2,2,2,2,2,2,2,2,2,2,2,2,2,
2,2,2,2,2,2,2,2,2,2,2,2,2,2,2,2,2,2,2,2,2,2,2,2,2,2,2,2,2,2,2,2,2,2,2,2,
2,2,2,2,2,2,2,2,2,2,2,2,2,2,2,2,2,2,2,2,2,2,2,2,2,2,2,2,2,2,4),(-11.6674812185143,
-11.6250639341939,-11.452758614136,-11.3653419798497,-11.3396861835031,
-11.3195725537615,-11.2961578970493,-11.2471869236146,-11.095880570994,
-10.9512030144633,-10.8955607672905,-10.8576552586143,-10.8178388970075,
-10.7532361748559,-10.6712080015292,-10.5660279602421,-10.537701199713,
-10.4411061122323,-10.4117353694135,-10.3918142977727,-10.3676471955674,
-10.3140450010698,-10.2290641620888,-10.0159831768752,-9.96933684787503,
-9.93141334317261,-9.89162686979631,-9.82719310907355,-9.74548112754296,
-9.639891111604,-9.61122440863084,-9.51459368712576,-9.48529475573627,-9.46538200855945,
-9.44117345798131,-9.38730488311043,-9.30164030901264,-9.09037053895614,
-9.04344259947757,-9.00545681747296,-8.96576913842449,-8.90189602246303,
-8.8212285645194,-8.7144919510522,-8.63680863312446,-8.5790685732414,-8.55368028483248,
-8.53590456504855,-8.50976772224468,-8.44190412092377,-8.31309460352719,
-8.24729796672785,-8.14809719214093,-8.10212655204483,-8.06493335961516,
-8.02026032297791,-7.92538306037018,-7.76812338690922,-7.66276767904412,
-7.63307051890696,-7.61311055057693,-7.58912712131054,-7.53668797455304,
-7.45464381966607,-7.2356073071504,-7.18946333331688,-7.15164944554759,
-7.11167773561874,-7.04619051473791,-6.96249359454973,-6.83861351932384,
-6.73740638782467,-6.70723702141564,-6.68721641940793,-6.66348203429672,
-6.61258501742843,-6.5343218996708,-6.30532873394259,-6.25623282981488,
-6.21874160611061,-6.1767566613799,-6.09957817794074,-5.85038241694493,
-5.79732852069243,-5.77292106510181,-5.75323374648202,-5.72442534241997,
-5.62743568691826,-5.44413721835684,-5.35988754664747,-5.31676700650914,
-5.27982100499634,-5.23203175716964,-5.1096397012042,-4.98575863720367,
-4.88561384303071,-4.85496873549817,-4.83488243151526,-4.81138097380995,
-4.76189196102184,-4.6097691271684,-4.60131147568333,-4.58685289213873,
-4.45118108351957,-4.4026239527585,-4.36519316845768,-4.32291588513274,
-4.24396160179546,-4.13187072449056,-3.9664113497804,-3.93213211999609,
-3.91347183275484,-3.89210188443545,-3.85427577016492,-3.80379554769993,
-3.65509167807215,-3.53585953630813,-3.48223661083977,-3.44426288449034,
-3.40375899392297,-3.33524257144796,-3.28755332486283,-3.11436112041818,
-3.02803584316149,-3.00242473939964,-2.98232038937175,-2.9588778863584,
-2.90973999638714,-2.75817144637901,-2.60087707652758,-2.55580768467391,
-2.51784334726336,-2.47731904322722,-2.40868548786738,-2.36087352344309,
-2.18671604919849,-2.10172654422203,-2.07610002701691,-2.05599262562791,
-2.0325601309602,-1.98348140961611,-1.83200650639649,-1.68767487707398,
-1.63203041603379,-1.594125196244,-1.55431058712312,-1.55222433781072,-1.55008167205715,
-1.54785282433669,-1.54550542370535,-1.54300298035776,-1.54030315603164,
-1.53735569514967,-1.53409988425154,-1.48470822882833,-1.39749447046565,
-1.29950401058437,-1.24933120713727,-1.20159772880599,-1.159153294331,-1.13689806285749,
-1.1237037002735,-1.12331886021745,-1.12242255779361,-1.12160855836381,
-1.09513478026533,-1.01999273177026,-0.853056510683363,-0.742518967345985,
-0.694690698631797,-0.65740269551631,-0.618224087802075,-0.605760054832675,
-0.511200275098992,-0.345374345319041,-0.250657363238717,-0.221560729498369,
-0.201670745750975,-0.182879237196195,-0.158118805160595,-1.00000000458067E-6),
 .UNSPECIFIED.) ;
#288=B_SPLINE_CURVE_WITH_KNOTS('',3,(#41983,#41984,#41985,#41986,#41987,
#41988,#41989,#41990,#41991,#41992,#41993,#41994,#41995,#41996,#41997,#41998,
#41999,#42000,#42001,#42002,#42003,#42004,#42005,#42006,#42007,#42008,#42009,
#42010,#42011,#42012,#42013,#42014,#42015,#42016,#42017,#42018,#42019,#42020,
#42021,#42022,#42023,#42024,#42025,#42026,#42027,#42028,#42029,#42030,#42031,
#42032,#42033,#42034,#42035,#42036,#42037,#42038,#42039,#42040,#42041,#42042,
#42043,#42044,#42045,#42046,#42047,#42048,#42049,#42050,#42051,#42052,#42053,
#42054,#42055,#42056,#42057,#42058,#42059,#42060,#42061,#42062,#42063,#42064,
#42065,#42066,#42067,#42068,#42069,#42070,#42071,#42072,#42073,#42074,#42075,
#42076,#42077,#42078,#42079,#42080,#42081,#42082,#42083,#42084,#42085,#42086,
#42087,#42088,#42089,#42090,#42091,#42092,#42093,#42094,#42095,#42096,#42097,
#42098,#42099,#42100,#42101,#42102,#42103,#42104,#42105,#42106,#42107,#42108,
#42109,#42110,#42111,#42112,#42113,#42114,#42115,#42116,#42117,#42118,#42119,
#42120,#42121,#42122,#42123,#42124,#42125,#42126,#42127,#42128,#42129,#42130,
#42131,#42132,#42133,#42134,#42135,#42136,#42137,#42138,#42139,#42140,#42141,
#42142,#42143,#42144,#42145,#42146,#42147,#42148,#42149,#42150,#42151,#42152,
#42153,#42154,#42155,#42156,#42157,#42158,#42159,#42160,#42161,#42162,#42163,
#42164,#42165,#42166,#42167,#42168,#42169,#42170,#42171,#42172,#42173,#42174,
#42175,#42176,#42177,#42178,#42179,#42180,#42181,#42182,#42183,#42184,#42185,
#42186,#42187,#42188,#42189,#42190,#42191,#42192,#42193,#42194,#42195,#42196,
#42197,#42198,#42199,#42200,#42201,#42202,#42203,#42204,#42205,#42206,#42207,
#42208,#42209,#42210,#42211,#42212,#42213,#42214,#42215,#42216,#42217,#42218,
#42219,#42220,#42221,#42222,#42223,#42224,#42225,#42226,#42227,#42228,#42229,
#42230,#42231,#42232,#42233,#42234,#42235,#42236,#42237,#42238,#42239,#42240,
#42241,#42242,#42243,#42244,#42245,#42246,#42247,#42248,#42249,#42250,#42251,
#42252,#42253,#42254,#42255,#42256,#42257,#42258,#42259,#42260,#42261,#42262,
#42263,#42264,#42265,#42266,#42267,#42268,#42269,#42270,#42271,#42272,#42273,
#42274,#42275,#42276,#42277,#42278,#42279,#42280,#42281,#42282,#42283,#42284,
#42285,#42286,#42287,#42288,#42289,#42290,#42291,#42292,#42293,#42294,#42295,
#42296,#42297,#42298,#42299,#42300,#42301,#42302,#42303,#42304,#42305,#42306,
#42307,#42308,#42309,#42310,#42311,#42312,#42313,#42314,#42315,#42316,#42317,
#42318,#42319,#42320,#42321,#42322,#42323,#42324,#42325,#42326,#42327,#42328,
#42329,#42330,#42331,#42332),.UNSPECIFIED.,.F.,.F.,(4,2,2,2,2,2,2,2,2,2,
2,2,2,2,2,2,2,2,2,2,2,2,2,2,2,2,2,2,2,2,2,2,2,2,2,2,2,2,2,2,2,2,2,2,2,2,
2,2,2,2,2,2,2,2,2,2,2,2,2,2,2,2,2,2,2,2,2,2,2,2,2,2,2,2,2,2,2,2,2,2,2,2,
2,2,2,2,2,2,2,2,2,2,2,2,2,2,2,2,2,2,2,2,2,2,2,2,2,2,2,2,2,2,2,2,2,2,2,2,
2,2,2,2,2,2,2,2,2,2,2,2,2,2,2,2,2,2,2,2,2,2,2,2,2,2,2,2,2,2,2,2,2,2,2,2,
2,2,2,2,2,2,2,2,2,2,2,2,2,2,2,2,2,2,2,2,4),(-26.1634555927762,-25.9005456295573,
-25.8600838083982,-25.8252427581716,-25.7873788085081,-25.734512258233,
-25.6130482706574,-25.4647201032695,-25.4142954645128,-25.3864213717277,
-25.3844024290128,-25.382774964513,-25.3814232611875,-25.3802679922519,
-25.3792529907394,-25.3783368821727,-25.3774876173322,-25.3766786756518,
-25.375886125169,-25.3750858987278,-25.354804803248,-25.3360605959684,-25.3012841550326,
-25.1873106731379,-25.0430099848548,-24.9790256235431,-24.9278006216719,
-24.8952378510719,-24.8572941145254,-24.8105553531357,-24.5980929156349,
-24.512871195488,-24.459175077678,-24.4349934041492,-24.4150753922217,-24.3857303139356,
-24.2865798222306,-24.1243511429391,-24.0781342201265,-24.0110368873529,
-23.9707816888126,-23.9331156938107,-23.8876737258095,-23.7461806934493,
-23.668699420783,-23.5854307848718,-23.5325030712123,-23.5084420375879,
-23.4884990609389,-23.4589419283742,-23.3549762451747,-23.1965191409114,
-23.1298531155164,-23.0739005284528,-23.0355657586829,-22.9957331307228,
-22.9310370363089,-22.8442856845235,-22.6879151558265,-22.6134544937361,
-22.5865674439942,-22.5668355786942,-22.5413199412167,-22.4834442323932,
-22.2836432920101,-22.2329477168704,-22.1616080174331,-22.1206126392663,
-22.0828374267399,-22.0306056096125,-21.8202292630448,-21.7342388213413,
-21.6802437786536,-21.6560155463226,-21.636106571774,-21.6068411676604,
-21.5040598381009,-21.306447110696,-21.2351700303235,-21.1941854110295,
-21.1564062027908,-21.1041457964309,-20.8939220934962,-20.8078762863678,
-20.7538597494541,-20.7296281461066,-20.709719764947,-20.6804599451628,
-20.5842388264993,-20.5474181173527,-20.4085456092294,-20.3194142234463,
-20.2755563358497,-20.2383237952918,-20.1913663274925,-20.08337294593,-19.9124234870151,
-19.8589183604534,-19.8195054100113,-19.7978256430033,-19.7793512276182,
-19.746207064751,-19.5520249341974,-19.4410474997005,-19.376799582891,-19.3370457439736,
-19.2991017312293,-19.25236286487,-19.0398963674548,-18.9546746733153,-18.9009783782314,
-18.8767965322115,-18.8568783280013,-18.8275328959924,-18.7283798655883,
-18.6993466763047,-18.5573457725992,-18.4671694667898,-18.4231589409445,
-18.3859362788938,-18.3391750213158,-18.2318737943291,-18.0295479009915,
-17.9749827787363,-17.9506663174477,-17.9307735668863,-17.9016559045358,
-17.8034618068912,-17.7844372269668,-17.6346122604599,-17.5902402468478,
-17.5249557153422,-17.4850191029655,-17.4471840492026,-17.4009446318418,
-17.1832689341992,-17.1005167582596,-17.0477941075134,-17.0237652693973,
-17.0038148665442,-16.9741986450779,-16.8739082490558,-16.8555838522135,
-16.7074615332913,-16.6153215954891,-16.5710292439237,-16.5338213263505,
-16.4874071327477,-16.3886563685478,-16.3255127177209,-16.1953454964747,
-16.1271189396966,-16.1009379292865,-16.0831595837025,-16.0578098398817,
-16.0010039944814,-15.7581977319401,-15.6809418056191,-15.6389432856571,
-15.601453866195,-15.5523805409929,-15.4168210638147,-15.404303705419,-15.2702466876122,
-15.2010056304652,-15.1747039748708,-15.1569190219069,-15.1316758310669,
-15.0770469074865,-14.8110317928371,-14.745738297446,-14.7058003368894,
-14.6679665446841,-14.6217319227932,-14.4955868793316),.UNSPECIFIED.) ;
#289=B_SPLINE_CURVE_WITH_KNOTS('',3,(#42337,#42338,#42339,#42340,#42341,
#42342,#42343,#42344,#42345,#42346,#42347,#42348,#42349,#42350,#42351,#42352,
#42353,#42354,#42355,#42356,#42357,#42358,#42359,#42360,#42361,#42362,#42363,
#42364,#42365,#42366,#42367,#42368,#42369,#42370,#42371,#42372,#42373,#42374,
#42375,#42376,#42377,#42378,#42379,#42380,#42381,#42382,#42383,#42384,#42385,
#42386,#42387,#42388,#42389,#42390,#42391,#42392,#42393,#42394,#42395,#42396,
#42397,#42398,#42399,#42400,#42401,#42402,#42403,#42404,#42405,#42406,#42407,
#42408,#42409,#42410,#42411,#42412,#42413,#42414,#42415,#42416,#42417,#42418,
#42419,#42420,#42421,#42422,#42423,#42424,#42425,#42426,#42427,#42428,#42429,
#42430,#42431,#42432,#42433,#42434,#42435,#42436,#42437,#42438,#42439,#42440,
#42441,#42442,#42443,#42444,#42445,#42446,#42447,#42448,#42449,#42450,#42451,
#42452,#42453,#42454,#42455,#42456,#42457,#42458,#42459,#42460,#42461,#42462,
#42463,#42464,#42465,#42466,#42467,#42468,#42469,#42470,#42471,#42472,#42473,
#42474,#42475,#42476,#42477,#42478,#42479,#42480,#42481,#42482,#42483,#42484,
#42485,#42486,#42487,#42488,#42489,#42490,#42491,#42492,#42493,#42494,#42495,
#42496,#42497,#42498,#42499,#42500,#42501,#42502,#42503,#42504,#42505,#42506,
#42507,#42508,#42509,#42510,#42511,#42512,#42513,#42514,#42515,#42516,#42517,
#42518,#42519,#42520,#42521,#42522,#42523,#42524,#42525,#42526,#42527,#42528,
#42529,#42530,#42531,#42532,#42533,#42534,#42535,#42536,#42537,#42538,#42539,
#42540,#42541,#42542,#42543,#42544,#42545,#42546,#42547,#42548,#42549,#42550,
#42551,#42552,#42553,#42554,#42555,#42556,#42557,#42558,#42559,#42560,#42561,
#42562,#42563,#42564,#42565,#42566,#42567,#42568,#42569,#42570,#42571,#42572,
#42573,#42574,#42575,#42576,#42577,#42578,#42579,#42580,#42581,#42582,#42583,
#42584,#42585,#42586,#42587,#42588,#42589,#42590,#42591,#42592,#42593,#42594,
#42595,#42596,#42597,#42598,#42599,#42600,#42601,#42602,#42603,#42604,#42605,
#42606,#42607,#42608,#42609,#42610,#42611,#42612,#42613,#42614,#42615,#42616,
#42617,#42618,#42619,#42620,#42621,#42622,#42623,#42624,#42625,#42626,#42627,
#42628,#42629,#42630,#42631,#42632,#42633,#42634,#42635,#42636,#42637,#42638,
#42639,#42640,#42641,#42642,#42643,#42644,#42645,#42646,#42647,#42648,#42649,
#42650,#42651,#42652,#42653,#42654,#42655,#42656,#42657,#42658,#42659,#42660,
#42661,#42662,#42663,#42664,#42665,#42666,#42667,#42668,#42669,#42670,#42671,
#42672,#42673,#42674,#42675,#42676,#42677,#42678,#42679,#42680,#42681,#42682),
 .UNSPECIFIED.,.F.,.F.,(4,2,2,2,2,2,2,2,2,2,2,2,2,2,2,2,2,2,2,2,2,2,2,2,
2,2,2,2,2,2,2,2,2,2,2,2,2,2,2,2,2,2,2,2,2,2,2,2,2,2,2,2,2,2,2,2,2,2,2,2,
2,2,2,2,2,2,2,2,2,2,2,2,2,2,2,2,2,2,2,2,2,2,2,2,2,2,2,2,2,2,2,2,2,2,2,2,
2,2,2,2,2,2,2,2,2,2,2,2,2,2,2,2,2,2,2,2,2,2,2,2,2,2,2,2,2,2,2,2,2,2,2,2,
2,2,2,2,2,2,2,2,2,2,2,2,2,2,2,2,2,2,2,2,2,2,2,2,2,2,2,2,2,2,2,2,2,2,2,2,
2,2,2,2,4),(-23.3349707992079,-23.3239989922033,-23.2274410553899,-23.1990240476791,
-23.0938151116522,-23.0118143646992,-22.9472266039377,-22.9074134561651,
-22.8695072376447,-22.8138567655311,-22.6695990338205,-22.5180893204448,
-22.468989507289,-22.4455534313055,-22.4254471005389,-22.3998260719168,
-22.314678798683,-22.1406314632797,-22.0928336449136,-22.0242135104071,
-21.9836915128912,-21.945726031682,-21.900651319766,-21.7434025499433,-21.5918145040618,
-21.5426652260224,-21.5192207757426,-21.4991169770238,-21.4735087958048,
-21.3876212384794,-21.2141006998859,-21.1663697481116,-21.097813392588,
-21.0573024673435,-21.0193318152379,-20.9742323342496,-20.8337931661458,
-20.7542881292985,-20.6710366417479,-20.6181158670165,-20.5940560346243,
-20.5741129661683,-20.5445541653208,-20.440554184855,-20.3166909204677,
-20.2337443427625,-20.1686535080152,-20.1287515477145,-20.0908976740466,
-20.0355839580884,-19.8425220773191,-19.7498203057522,-19.6932995032669,
-19.668687742462,-19.6488437458234,-19.6201988448173,-19.5294090246976,
-19.49350484282,-19.3879702952107,-19.3062179237801,-19.241762545288,-19.2019723597133,
-19.1640513280577,-19.1174158592369,-18.9042572573285,-18.8193055305962,
-18.765714794811,-18.7415495247288,-18.7216281558883,-18.6922544503117,
-18.5957102482914,-18.5673310201109,-18.4621333355221,-18.3801212151583,
-18.3155270288677,-18.2757122615612,-18.2378059618934,-18.1821581645104,
-18.0378488734775,-17.886357665714,-17.8372703761585,-17.8138361492038,
-17.7937287675624,-17.7681037877475,-17.683060504112,-17.50893803918,-17.4611302574943,
-17.3925002185211,-17.3519759984953,-17.3140105524144,-17.268938417913,
-17.1116537719647,-16.9600753526623,-16.9109329760767,-16.8874894267804,
-16.8673848764319,-16.8417742281581,-16.7555044665352,-16.5822678654633,
-16.5345726919139,-16.4660501272825,-16.4255446265172,-16.3875705491433,
-16.3424567945677,-16.2019590351409,-16.1225479323325,-16.0392939849133,
-15.986371892441,-15.9623115821687,-15.9423681850436,-15.9128089919985,
-15.809603313635,-15.6857304891592,-15.6023847873357,-15.5370824006422,
-15.4971426973787,-15.4593095220977,-15.413078559313,-15.1952561319728,
-15.1125831345607,-15.0598920956018,-15.0358683020998,-15.0159168375672,
-14.9862916396495,-14.8863030501742,-14.7251040700319,-14.6790325390657,
-14.6120763189037,-14.5718454426768,-14.5341665611389,-14.4800057606724,
-14.362322645614,-14.3349578000564,-14.2067675568506,-14.1390697175955,
-14.1129525875296,-14.0951775335738,-14.0697704865219,-14.0119037940393,
-13.7703337862915,-13.6930624711711,-13.6510614580554,-13.6135726811405,
-13.5645043561546,-13.428992268934,-13.2853742085968,-13.2137761940229,
-13.1872028594267,-13.1674763559152,-13.1416772799711,-13.0814214710313,
-12.9726925023648,-12.9299558829238,-12.7905693845878,-12.7455763520613,
-12.7076269340837,-12.6670661609092,-12.5982279800385,-12.5502019133739,
-12.3743456840732,-12.295004629071,-12.2650674026273,-12.2450769181647,
-12.2212217132812,-12.1695832220456,-12.0140833218758,-11.9835391163372,
-11.8922817073756,-11.8294225786088,-11.7899126742753,-11.7513554355678,
-11.6940425261241,-11.6674812185143),.UNSPECIFIED.) ;
#290=B_SPLINE_CURVE_WITH_KNOTS('',3,(#42683,#42684,#42685,#42686,#42687,
#42688,#42689,#42690,#42691,#42692,#42693,#42694,#42695,#42696,#42697,#42698,
#42699,#42700,#42701,#42702,#42703,#42704,#42705,#42706,#42707,#42708,#42709,
#42710,#42711,#42712,#42713,#42714,#42715,#42716,#42717,#42718,#42719,#42720,
#42721,#42722,#42723,#42724,#42725,#42726,#42727,#42728,#42729,#42730,#42731,
#42732,#42733,#42734,#42735,#42736,#42737,#42738,#42739,#42740,#42741,#42742,
#42743,#42744,#42745,#42746,#42747,#42748,#42749,#42750,#42751,#42752,#42753,
#42754,#42755,#42756,#42757,#42758,#42759,#42760,#42761,#42762,#42763,#42764,
#42765,#42766,#42767,#42768,#42769,#42770,#42771,#42772,#42773,#42774,#42775,
#42776,#42777,#42778,#42779,#42780,#42781,#42782,#42783,#42784,#42785,#42786,
#42787,#42788,#42789,#42790,#42791,#42792,#42793,#42794,#42795,#42796,#42797,
#42798,#42799,#42800,#42801,#42802,#42803,#42804,#42805,#42806,#42807,#42808,
#42809,#42810,#42811,#42812,#42813,#42814,#42815,#42816,#42817,#42818,#42819,
#42820,#42821,#42822,#42823,#42824,#42825,#42826,#42827,#42828,#42829,#42830,
#42831,#42832,#42833,#42834,#42835,#42836,#42837,#42838,#42839,#42840,#42841,
#42842,#42843,#42844,#42845,#42846,#42847,#42848,#42849,#42850,#42851,#42852,
#42853,#42854,#42855,#42856,#42857,#42858,#42859,#42860,#42861,#42862,#42863,
#42864,#42865,#42866,#42867,#42868,#42869,#42870,#42871,#42872,#42873,#42874,
#42875,#42876,#42877,#42878,#42879,#42880,#42881,#42882,#42883,#42884,#42885,
#42886,#42887,#42888,#42889,#42890,#42891,#42892,#42893,#42894,#42895,#42896,
#42897,#42898,#42899,#42900,#42901,#42902,#42903,#42904,#42905,#42906,#42907,
#42908,#42909,#42910,#42911,#42912,#42913,#42914,#42915,#42916,#42917,#42918,
#42919,#42920,#42921,#42922,#42923,#42924,#42925,#42926,#42927,#42928,#42929,
#42930,#42931,#42932,#42933,#42934,#42935,#42936,#42937,#42938,#42939,#42940,
#42941,#42942,#42943,#42944,#42945,#42946,#42947,#42948,#42949,#42950,#42951,
#42952,#42953,#42954,#42955,#42956,#42957,#42958,#42959,#42960,#42961,#42962,
#42963,#42964,#42965,#42966,#42967,#42968,#42969,#42970,#42971,#42972,#42973,
#42974,#42975,#42976,#42977,#42978,#42979,#42980,#42981,#42982,#42983,#42984,
#42985,#42986,#42987,#42988,#42989,#42990,#42991,#42992,#42993,#42994,#42995,
#42996,#42997,#42998,#42999,#43000,#43001,#43002,#43003,#43004,#43005,#43006,
#43007,#43008,#43009,#43010,#43011,#43012,#43013,#43014,#43015,#43016,#43017,
#43018,#43019,#43020,#43021,#43022,#43023,#43024),.UNSPECIFIED.,.F.,.F.,
(4,2,2,2,2,2,2,2,2,2,2,2,2,2,2,2,2,2,2,2,2,2,2,2,2,2,2,2,2,2,2,2,2,2,2,
2,2,2,2,2,2,2,2,2,2,2,2,2,2,2,2,2,2,2,2,2,2,2,2,2,2,2,2,2,2,2,2,2,2,2,2,
2,2,2,2,2,2,2,2,2,2,2,2,2,2,2,2,2,2,2,2,2,2,2,2,2,2,2,2,2,2,2,2,2,2,2,2,
2,2,2,2,2,2,2,2,2,2,2,2,2,2,2,2,2,2,2,2,2,2,2,2,2,2,2,2,2,2,2,2,2,2,2,2,
2,2,2,2,2,2,2,2,2,2,2,2,2,2,2,2,2,2,2,2,2,2,2,2,2,2,2,4),(-14.4955868793316,
-14.4039793170469,-14.3212701233793,-14.2685647675828,-14.2445387984084,
-14.2245879677227,-14.1949671515612,-14.0901164688323,-13.9662581554151,
-13.8837995239049,-13.818967367714,-13.7791105038954,-13.7412291128518,
-13.6857417290152,-13.4454965581512,-13.3821441933305,-13.3378565835037,
-13.3152620374607,-13.29506387067,-13.2624299488094,-13.0815402128621,-13.0552579637053,
-12.9287762164095,-12.8826137696698,-12.8447955346388,-12.8048301231133,
-12.7393808313133,-12.6557564066087,-12.5318764198995,-12.4298476854656,
-12.3999971117681,-12.3800178084561,-12.3561169356853,-12.3041943909403,
-12.2234313772468,-12.0125505313966,-11.9569134908243,-11.9190089599369,
-11.8791915540792,-11.8145820097614,-11.732540833122,-11.6273789954797,
-11.599096028804,-11.502381473842,-11.4730505829374,-11.453134192005,-11.4289442618914,
-11.3751952309114,-11.2898378643987,-11.0777384421734,-11.0309439647207,
-10.9929878708533,-10.9532540167676,-10.8891183497146,-10.8458949680382,
-10.7031814765845,-10.6882010948926,-10.5855391011472,-10.5514693862968,
-10.5328439803766,-10.5114200871932,-10.4733196929336,-10.4223226058006,
-10.2700942582674,-10.1597890125376,-10.104188150797,-10.066289455147,-10.0264629941703,
-9.96180111446944,-9.87966156226488,-9.77463037878878,-9.74654599323164,
-9.65616965373775,-9.62368751845823,-9.60351496148271,-9.58086708463561,
-9.53628310367461,-9.5023622158865,-9.37083921768833,-9.32767411642239,
-9.30812174256324,-9.21036054192749,-9.16409192863681,-9.12689018779048,
-9.08247743215429,-8.98947772570046,-8.83856297365265,-8.82205571155216,
-8.7233601673296,-8.69403940962128,-8.67412430492512,-8.64992880103779,
-8.59614322763526,-8.51069163470255,-8.2988475014797,-8.25201322898575,
-8.2140485133544,-8.17432895057607,-8.11027328158569,-8.06712919649685,
-7.92489080825616,-7.90248048993045,-7.79764620296472,-7.76802746102402,
-7.7480772430249,-7.72405100507957,-7.67134177166229,-7.5886218284831,-7.37090178651196,
-7.32466695889884,-7.28683372805554,-7.24689709566393,-7.18160768543455,
-6.92363123316017,-6.86309710298538,-6.83729101113456,-6.81756499659706,
-6.79100033675199,-6.71947556664963,-6.5761623686038,-6.44034623790568,
-6.39124741547667,-6.3537557613976,-6.3117721511883,-6.2346022165538,-5.98462798559819,
-5.93147205349662,-5.90737507205986,-5.8894540419988,-5.86162268850463,
-5.77741720675405,-5.56334169413312,-5.48980431784596,-5.44806685953881,
-5.41051656611965,-5.36003403345945,-5.18444949296384,-5.02599200081779,
-4.99261966705988,-4.97410867131996,-4.95249508261339,-4.91342284446691,
-4.86057417999203,-4.69480579808704,-4.58240258557219,-4.53472468081932,
-4.49744729924692,-4.45411235710466,-4.36846993305474,-4.23947159206005,
-4.10239999887364,-4.06756899516444,-4.04881551835389,-4.02757981635413,
-3.990437399122,-3.94123543379691,-3.80083578355941,-3.66188827416622,-3.61692358349515,
-3.5789803919992,-3.53840749432713,-3.46949737322776,-3.42139531978016,
-3.24492466024322,-3.17165719730139,-3.13913700231706,-3.11895810454882,
-3.09632383325239,-3.05181526940531,-2.98799466372576,-2.82792612848063),
 .UNSPECIFIED.) ;
#291=B_SPLINE_CURVE_WITH_KNOTS('',3,(#43030,#43031,#43032,#43033,#43034,
#43035,#43036,#43037,#43038,#43039,#43040,#43041,#43042,#43043,#43044,#43045,
#43046,#43047,#43048,#43049,#43050,#43051,#43052,#43053,#43054,#43055,#43056,
#43057,#43058,#43059,#43060,#43061,#43062,#43063,#43064,#43065,#43066,#43067,
#43068,#43069,#43070,#43071,#43072,#43073,#43074,#43075,#43076,#43077,#43078,
#43079,#43080,#43081,#43082,#43083,#43084,#43085,#43086,#43087,#43088,#43089,
#43090,#43091,#43092,#43093,#43094,#43095,#43096,#43097,#43098,#43099,#43100,
#43101,#43102,#43103,#43104,#43105,#43106,#43107,#43108,#43109,#43110,#43111,
#43112,#43113,#43114,#43115,#43116,#43117,#43118,#43119,#43120,#43121,#43122,
#43123,#43124,#43125,#43126,#43127,#43128,#43129,#43130,#43131,#43132,#43133,
#43134,#43135,#43136,#43137,#43138,#43139,#43140,#43141,#43142,#43143,#43144,
#43145,#43146,#43147,#43148,#43149,#43150,#43151,#43152,#43153,#43154,#43155,
#43156,#43157,#43158,#43159,#43160,#43161,#43162,#43163,#43164,#43165,#43166,
#43167,#43168,#43169,#43170,#43171,#43172,#43173,#43174,#43175,#43176,#43177,
#43178,#43179,#43180,#43181,#43182,#43183,#43184,#43185,#43186,#43187,#43188,
#43189,#43190,#43191,#43192,#43193,#43194,#43195,#43196,#43197,#43198,#43199,
#43200,#43201,#43202,#43203,#43204,#43205,#43206,#43207,#43208,#43209,#43210,
#43211,#43212,#43213,#43214,#43215,#43216,#43217,#43218,#43219,#43220,#43221,
#43222,#43223,#43224,#43225,#43226,#43227,#43228,#43229,#43230,#43231,#43232,
#43233,#43234,#43235,#43236,#43237,#43238,#43239,#43240,#43241,#43242,#43243,
#43244,#43245,#43246,#43247,#43248,#43249,#43250,#43251,#43252,#43253,#43254,
#43255,#43256,#43257,#43258,#43259,#43260,#43261,#43262,#43263,#43264,#43265,
#43266,#43267,#43268,#43269,#43270,#43271,#43272,#43273,#43274,#43275,#43276,
#43277,#43278,#43279,#43280,#43281,#43282,#43283,#43284,#43285,#43286,#43287,
#43288,#43289,#43290,#43291,#43292,#43293,#43294,#43295,#43296,#43297),
 .UNSPECIFIED.,.F.,.F.,(4,2,2,2,2,2,2,2,2,2,2,2,2,2,2,2,2,2,2,2,2,2,2,2,
2,2,2,2,2,2,2,2,2,2,2,2,2,2,2,2,2,2,2,2,2,2,2,2,2,2,2,2,2,2,2,2,2,2,2,2,
2,2,2,2,2,2,2,2,2,2,2,2,2,2,2,2,2,2,2,2,2,2,2,2,2,2,2,2,2,2,2,2,2,2,2,2,
2,2,2,2,2,2,2,2,2,2,2,2,2,2,2,2,2,2,2,2,2,2,2,2,2,2,2,2,2,2,2,2,2,2,2,2,
2,4),(-8.83945532408071,-8.81772296497787,-8.77981688992475,-8.74000136067843,
-8.67540352300486,-8.59338454410489,-8.48819223953054,-8.45983298970468,
-8.36327884080695,-8.3339011300318,-8.313979235886,-8.28981610975072,-8.23623945405055,
-8.15132397785674,-7.93807746110587,-7.89145490121599,-7.8535366028422,
-7.81374158039737,-7.74925940985965,-7.66745688941652,-7.5619835882094,
-7.53134212096736,-7.43637551815251,-7.40724975211934,-7.38735631909881,
-7.36304522409823,-7.30851372638641,-7.22113035751957,-7.01406654748622,
-6.96134665866414,-6.92350346431488,-6.88268928374934,-6.81239518505327,
-6.71925619475584,-6.5947381301372,-6.50834087970517,-6.48272835949858,
-6.46262363412635,-6.43918179811748,-6.39004842026468,-6.23848654365196,
-6.08117096506745,-6.03610325029695,-5.99813908142674,-5.95761364055599,
-5.88897458095356,-5.84115699579456,-5.66695637310105,-5.58202864716916,
-5.55639960356666,-5.53629160286888,-5.51286048360273,-5.46379047419234,
-5.3123288773162,-5.16796451107701,-5.11232159130715,-5.07441643550708,
-5.03460109859423,-4.97000165847179,-4.88797902381774,-4.78279506124984,
-4.75445410765858,-4.65788350880418,-4.62850800295046,-4.60858663971583,
-4.58442292871877,-4.53084084653061,-4.44591062717666,-4.23270834965547,
-4.18608074271722,-4.14816179496332,-4.10836952055798,-4.04390026569526,
-3.96212126842258,-3.8566210513172,-3.73523163742586,-3.7040891185304,-3.68412781972634,
-3.66095061508918,-3.61336883076644,-3.57600692301453,-3.41733343367493,
-3.34301308077549,-3.27306337647489,-3.23230953181443,-3.19444318982108,
-3.14155708152949,-3.07998366293311,-2.94707990393144,-2.89773104151819,
-2.80428847398365,-2.77534451285491,-2.75547084430239,-2.73104971675999,
-2.67579621070942,-2.5865098677734,-2.38291387507709,-2.32996762224583,
-2.29209281180773,-2.25136043184919,-2.18153343131242,-2.13246145383143,
-1.94786327624138,-1.93470102807542,-1.87124632747421,-1.84545302553626,
-1.82572708541858,-1.7991492386095,-1.72750584998882,-1.58369019303517,
-1.44839253437952,-1.39934788487226,-1.36186284374058,-1.32694073848364,
-1.28519128592769,-1.1525946536019,-0.961623155505617,-0.928367322517469,
-0.907931625399414,-0.889741860057858,-0.875874959638054,-0.814163079981681,
-0.706304858487514,-0.667332989671791,-0.524217272788026,-0.478765902264634,
-0.441098484134846,-0.406249494706772,-0.366330681831491,-0.307347671505237,
-0.167385808365722,-0.0429957109239202,-0.0182555783699187,-1.00000000173572E-6),
 .UNSPECIFIED.) ;
#292=B_SPLINE_CURVE_WITH_KNOTS('',3,(#43298,#43299,#43300,#43301,#43302,
#43303,#43304,#43305,#43306,#43307,#43308,#43309,#43310,#43311,#43312,#43313,
#43314,#43315,#43316,#43317,#43318,#43319,#43320,#43321,#43322,#43323,#43324,
#43325,#43326,#43327,#43328,#43329,#43330,#43331,#43332,#43333,#43334,#43335,
#43336,#43337,#43338,#43339,#43340,#43341,#43342,#43343,#43344,#43345,#43346,
#43347,#43348,#43349,#43350,#43351,#43352,#43353,#43354,#43355,#43356,#43357,
#43358,#43359,#43360,#43361,#43362,#43363,#43364,#43365,#43366,#43367,#43368,
#43369,#43370,#43371,#43372,#43373,#43374,#43375,#43376,#43377,#43378,#43379,
#43380,#43381,#43382,#43383,#43384,#43385,#43386,#43387,#43388,#43389,#43390,
#43391,#43392,#43393,#43394,#43395,#43396,#43397,#43398,#43399,#43400,#43401,
#43402,#43403,#43404,#43405,#43406,#43407,#43408,#43409),.UNSPECIFIED.,
 .F.,.F.,(4,2,2,2,2,2,2,2,2,2,2,2,2,2,2,2,2,2,2,2,2,2,2,2,2,2,2,2,2,2,2,
2,2,2,2,2,2,2,2,2,2,2,2,2,2,2,2,2,2,2,2,2,2,2,2,4),(-26.1629118607084,-26.1454935044846,
-26.1261207928679,-26.0917122142876,-25.9628614800202,-25.8273404683811,
-25.7414593988453,-25.7054475674227,-25.6681895085004,-25.6246522692977,
-25.537676959584,-25.3506240911098,-25.2886646959746,-25.2450408134631,
-25.2262511845348,-25.2115733057507,-25.187046031042,-25.1337856122842,
-24.9286494438691,-24.8552799980706,-24.8509574230423,-24.8387277361866,
-24.83388082635,-24.8255983766822,-24.8199213669822,-24.8160452575958,-24.813395492473,
-24.8115785832224,-24.8103287015693,-24.8064810097528,-24.803093528574,
-24.8000903033327,-24.7974062205088,-24.7949856496721,-24.7601013428692,
-24.7221954241647,-24.6665495485182,-24.489860052902,-24.3389903115827,
-24.3083751113904,-24.2882932115933,-24.2647779655738,-24.2152056292869,
-24.1249752275425,-24.0190672851008,-23.9376097197101,-23.8733124310856,
-23.8335505595953,-23.7956130296214,-23.748900607415,-23.5362722260045,
-23.4511164813559,-23.397446393384,-23.3732690015012,-23.3533504815712,
-23.3349707992079),.UNSPECIFIED.) ;
#293=B_SPLINE_CURVE_WITH_KNOTS('',3,(#43411,#43412,#43413,#43414,#43415,
#43416,#43417,#43418,#43419,#43420,#43421,#43422,#43423,#43424,#43425,#43426,
#43427,#43428,#43429,#43430,#43431,#43432,#43433,#43434,#43435,#43436,#43437,
#43438,#43439,#43440,#43441,#43442,#43443,#43444,#43445,#43446,#43447,#43448,
#43449,#43450,#43451,#43452,#43453,#43454,#43455,#43456,#43457,#43458,#43459,
#43460,#43461,#43462,#43463,#43464,#43465,#43466,#43467,#43468,#43469,#43470,
#43471,#43472,#43473,#43474,#43475,#43476,#43477,#43478,#43479,#43480,#43481,
#43482,#43483,#43484,#43485,#43486,#43487,#43488,#43489,#43490,#43491,#43492,
#43493,#43494,#43495,#43496,#43497,#43498,#43499,#43500,#43501,#43502,#43503,
#43504,#43505,#43506,#43507,#43508,#43509,#43510,#43511,#43512,#43513,#43514,
#43515,#43516,#43517,#43518),.UNSPECIFIED.,.F.,.F.,(4,2,2,2,2,2,2,2,2,2,
2,2,2,2,2,2,2,2,2,2,2,2,2,2,2,2,2,2,2,2,2,2,2,2,2,2,2,2,2,2,2,2,2,2,2,2,
2,2,2,2,2,2,2,4),(-2.82792612848063,-2.8041603327855,-2.71722452840601,
-2.67369354603614,-2.63643530107694,-2.58903728134093,-2.4708245315289,
-2.36446470976795,-2.24363929252875,-2.21196612827096,-2.19192388812018,
-2.16896819323943,-2.12265796130199,-2.08677713582502,-1.94050254230746,
-1.80722666065535,-1.75862839639159,-1.72119316882715,-1.67893897308388,
-1.6001259222878,-1.48836799577483,-1.32226757322654,-1.28803156524166,
-1.26937851219505,-1.25378343596525,-1.25321556649319,-1.25271179604491,
-1.25226639635086,-1.25187384333195,-1.25152887399879,-1.25122653042299,
-1.25096219051075,-1.25073158616506,-1.25053081021818,-1.2500027044565,
-1.2494860725939,-1.24898097171239,-1.21745789151553,-1.17423099090844,
-1.06650389790476,-0.89558294968666,-0.840263873650828,-0.802778320537367,
-0.766902826466558,-0.716509180206056,-0.650490717393987,-0.495617729964171,
-0.395330090035875,-0.361413339863902,-0.342813367365246,-0.324703471960157,
-0.302795572703682,-0.269147194228328,-9.99999989481637E-7),
 .UNSPECIFIED.) ;
#294=B_SPLINE_CURVE_WITH_KNOTS('',3,(#43519,#43520,#43521,#43522,#43523,
#43524,#43525,#43526,#43527,#43528,#43529,#43530,#43531,#43532,#43533,#43534,
#43535,#43536,#43537,#43538,#43539,#43540,#43541,#43542,#43543,#43544,#43545,
#43546,#43547,#43548,#43549,#43550,#43551,#43552,#43553,#43554,#43555,#43556,
#43557,#43558,#43559,#43560,#43561,#43562,#43563,#43564,#43565,#43566,#43567,
#43568,#43569,#43570,#43571,#43572,#43573,#43574,#43575,#43576,#43577,#43578,
#43579,#43580,#43581,#43582,#43583,#43584,#43585,#43586,#43587,#43588,#43589,
#43590,#43591,#43592,#43593,#43594,#43595,#43596,#43597,#43598,#43599,#43600,
#43601,#43602,#43603,#43604,#43605,#43606,#43607,#43608,#43609,#43610,#43611,
#43612,#43613,#43614,#43615,#43616,#43617,#43618,#43619,#43620,#43621,#43622,
#43623,#43624,#43625,#43626,#43627,#43628,#43629,#43630,#43631,#43632,#43633,
#43634,#43635,#43636,#43637,#43638,#43639,#43640,#43641,#43642,#43643,#43644,
#43645,#43646,#43647,#43648,#43649,#43650,#43651,#43652,#43653,#43654,#43655,
#43656,#43657,#43658,#43659,#43660,#43661,#43662,#43663,#43664,#43665,#43666,
#43667,#43668,#43669,#43670,#43671,#43672,#43673,#43674,#43675,#43676,#43677,
#43678,#43679,#43680,#43681,#43682,#43683,#43684,#43685,#43686,#43687,#43688,
#43689,#43690,#43691,#43692,#43693,#43694,#43695,#43696,#43697,#43698,#43699,
#43700,#43701,#43702,#43703,#43704,#43705,#43706,#43707,#43708,#43709,#43710,
#43711,#43712,#43713,#43714,#43715,#43716,#43717,#43718,#43719,#43720,#43721,
#43722,#43723,#43724,#43725,#43726,#43727,#43728,#43729,#43730,#43731,#43732,
#43733,#43734,#43735,#43736,#43737,#43738,#43739,#43740,#43741,#43742,#43743,
#43744,#43745,#43746,#43747,#43748,#43749,#43750,#43751,#43752,#43753,#43754,
#43755,#43756,#43757,#43758,#43759,#43760,#43761,#43762,#43763,#43764,#43765,
#43766,#43767,#43768,#43769,#43770,#43771,#43772,#43773,#43774,#43775,#43776,
#43777,#43778,#43779,#43780,#43781,#43782,#43783,#43784,#43785,#43786,#43787,
#43788,#43789,#43790,#43791,#43792,#43793,#43794,#43795,#43796,#43797,#43798,
#43799,#43800,#43801,#43802,#43803,#43804,#43805,#43806,#43807,#43808,#43809,
#43810,#43811,#43812,#43813,#43814,#43815,#43816,#43817,#43818,#43819,#43820,
#43821,#43822,#43823,#43824,#43825,#43826,#43827,#43828,#43829,#43830,#43831,
#43832,#43833,#43834,#43835,#43836,#43837,#43838,#43839,#43840,#43841,#43842,
#43843,#43844,#43845,#43846,#43847,#43848,#43849,#43850,#43851,#43852,#43853,
#43854,#43855,#43856,#43857,#43858,#43859,#43860,#43861,#43862,#43863,#43864,
#43865,#43866,#43867,#43868,#43869,#43870,#43871,#43872,#43873,#43874,#43875,
#43876,#43877,#43878,#43879,#43880,#43881,#43882,#43883,#43884),
 .UNSPECIFIED.,.F.,.F.,(4,2,2,2,2,2,2,2,2,2,2,2,2,2,2,2,2,2,2,2,2,2,2,2,
2,2,2,2,2,2,2,2,2,2,2,2,2,2,2,2,2,2,2,2,2,2,2,2,2,2,2,2,2,2,2,2,2,2,2,2,
2,2,2,2,2,2,2,2,2,2,2,2,2,2,2,2,2,2,2,2,2,2,2,2,2,2,2,2,2,2,2,2,2,2,2,2,
2,2,2,2,2,2,2,2,2,2,2,2,2,2,2,2,2,2,2,2,2,2,2,2,2,2,2,2,2,2,2,2,2,2,2,2,
2,2,2,2,2,2,2,2,2,2,2,2,2,2,2,2,2,2,2,2,2,2,2,2,2,2,2,2,2,2,2,2,2,2,2,2,
2,2,2,2,2,2,2,2,2,2,2,2,2,2,4),(-23.3351463080753,-23.294167951005,-23.2607234492997,
-23.2258029543077,-23.1899174225933,-23.1418265154115,-23.0158784775917,
-22.8703830766604,-22.8097257526394,-22.7771067645078,-22.7583306858827,
-22.7384307415802,-22.7092439655656,-22.6137266913003,-22.5914715742371,
-22.4421401846129,-22.3771646348096,-22.3258402204451,-22.292806562641,
-22.2554008546556,-22.2005981424254,-22.0148262787654,-21.9165041602218,
-21.8753201060059,-21.8735469715915,-21.8719714444937,-21.8705696836065,
-21.8693208279231,-21.868206647997,-21.8672112252402,-21.8663206615595,
-21.8655228197381,-21.8648070935743,-21.8641642059376,-21.8635860324511,
-21.8630654482073,-21.8625961950523,-21.8621727669429,-21.8617903110256,
-21.8614445424995,-21.8611316712138,-21.860848338432,-21.8605915624252,
-21.8603586914862,-21.8601473633363,-21.8594299393724,-21.8587391921259,
-21.8580736184432,-21.857431804381,-21.8568124193287,-21.8562142105715,
-21.8556359981386,-21.8550766700135,-21.8545351776685,-21.8540105318744,
-21.8535017987687,-21.853008096188,-21.8525285902435,-21.852062492069,-21.8516090548073,
-21.8511675708174,-21.850737368974,-21.8503178121519,-21.8499082949377,
-21.8495082413861,-21.8491171029318,-21.848734356484,-21.8483595025164,
-21.8479920633295,-21.8476315814089,-21.8472776178631,-21.8469297508675,
-21.8465875743004,-21.8462506963629,-21.8459187382141,-21.8455913327549,
-21.8452681233537,-21.8449487627008,-21.8303501039131,-21.8102318170827,
-21.7845517460689,-21.6967912768393,-21.5247930905553,-21.4772574380689,
-21.4088878749417,-21.3684096724222,-21.3304241416761,-21.2852522741711,
-21.1487804911606,-21.0069275054717,-20.9574953331976,-20.9202292887279,
-20.8989694292156,-20.8802335287785,-20.8455057344452,-20.7096122929139,
-20.5797387920721,-20.4937753602065,-20.4503916108007,-20.4131193577101,
-20.3655125350636,-20.2554343035864,-20.0433495689906,-19.9987394987869,
-19.9760868720848,-19.9559164124966,-19.9234472134472,-19.7259266535772,
-19.6301546078995,-19.5585797029641,-19.5175438020412,-19.4797831953867,
-19.4276574179106,-19.1811606293551,-19.117013450659,-19.0955400340761,
-19.063208342075,-19.0428600036321,-19.0200649975175,-18.9746619643204,
-18.7771066036361,-18.6931403601937,-18.6275112187552,-18.587514481014,
-18.5497144507524,-18.4947491724804,-18.3120770146737,-18.2118982483161,
-18.1702979781377,-18.137390627667,-18.1169448064465,-18.0943557802202,
-18.0500968134275,-18.0009297486148,-17.8217266458526,-17.7517048340439,
-17.693785196244,-17.6551273509583,-17.6203792254955,-17.5628254584511,
-17.4578846589815,-17.3047234125667,-17.2535919136577,-17.2154205256659,
-17.1939827757626,-17.1753663220772,-17.1413502110518,-17.0394372067765,
-17.011667863475,-16.8769013833938,-16.7891854527113,-16.7455375226847,
-16.7082894285267,-16.6610528831851,-16.5522755775284,-16.3825985754233,
-16.3292523611245,-16.2899218375541,-16.2682582040096,-16.2497753201483,
-16.2165772725303,-16.0237724688728,-15.9111734778208,-15.8471138037135,
-15.8073934530403,-15.7694290347796,-15.7225965045835,-15.5107357727681,
-15.4252878551299,-15.3715036616736,-15.3473083162426,-15.3273930978448,
-15.2980718425089,-15.2014729188486,-15.1730243944334,-15.0678042440994,
-14.9858103705424,-14.9212260620675,-14.8814132303399,-14.8435061826619,
-14.787852332879,-14.6436272489799,-14.4955154817265),.UNSPECIFIED.) ;
#295=B_SPLINE_CURVE_WITH_KNOTS('',3,(#43889,#43890,#43891,#43892,#43893,
#43894,#43895,#43896,#43897,#43898,#43899,#43900,#43901,#43902,#43903,#43904,
#43905,#43906,#43907,#43908,#43909,#43910,#43911,#43912,#43913,#43914,#43915,
#43916,#43917,#43918,#43919,#43920,#43921,#43922,#43923,#43924,#43925,#43926,
#43927,#43928,#43929,#43930,#43931,#43932,#43933,#43934,#43935,#43936,#43937,
#43938,#43939,#43940,#43941,#43942,#43943,#43944,#43945,#43946,#43947,#43948,
#43949,#43950,#43951,#43952,#43953,#43954,#43955,#43956,#43957,#43958,#43959,
#43960,#43961,#43962,#43963,#43964,#43965,#43966,#43967,#43968,#43969,#43970,
#43971,#43972,#43973,#43974,#43975,#43976,#43977,#43978,#43979,#43980,#43981,
#43982,#43983,#43984,#43985,#43986,#43987,#43988,#43989,#43990,#43991,#43992,
#43993,#43994,#43995,#43996,#43997,#43998,#43999,#44000,#44001,#44002,#44003,
#44004,#44005,#44006,#44007,#44008,#44009,#44010,#44011,#44012,#44013,#44014,
#44015,#44016,#44017,#44018,#44019,#44020,#44021,#44022,#44023,#44024,#44025,
#44026,#44027,#44028,#44029,#44030,#44031,#44032,#44033,#44034,#44035,#44036,
#44037,#44038,#44039,#44040,#44041,#44042,#44043,#44044,#44045,#44046,#44047,
#44048,#44049,#44050,#44051,#44052,#44053,#44054,#44055,#44056,#44057,#44058,
#44059,#44060,#44061,#44062,#44063,#44064,#44065,#44066,#44067,#44068,#44069,
#44070,#44071,#44072,#44073,#44074,#44075,#44076,#44077,#44078,#44079,#44080,
#44081,#44082,#44083,#44084,#44085,#44086,#44087,#44088,#44089,#44090,#44091,
#44092,#44093,#44094,#44095,#44096,#44097,#44098,#44099,#44100,#44101,#44102,
#44103,#44104,#44105,#44106,#44107,#44108,#44109,#44110,#44111,#44112,#44113,
#44114,#44115,#44116,#44117,#44118,#44119,#44120,#44121,#44122,#44123,#44124,
#44125,#44126,#44127,#44128,#44129,#44130,#44131,#44132,#44133,#44134,#44135,
#44136,#44137,#44138,#44139,#44140,#44141,#44142,#44143,#44144,#44145,#44146,
#44147,#44148,#44149,#44150,#44151,#44152,#44153,#44154,#44155,#44156,#44157,
#44158,#44159,#44160,#44161,#44162,#44163,#44164,#44165,#44166,#44167,#44168,
#44169,#44170,#44171,#44172,#44173,#44174,#44175,#44176,#44177,#44178,#44179,
#44180,#44181,#44182,#44183,#44184,#44185,#44186,#44187,#44188,#44189,#44190,
#44191,#44192,#44193,#44194,#44195,#44196,#44197,#44198,#44199,#44200,#44201,
#44202,#44203,#44204,#44205,#44206,#44207,#44208,#44209,#44210,#44211,#44212,
#44213,#44214,#44215,#44216,#44217,#44218,#44219,#44220,#44221,#44222,#44223,
#44224,#44225,#44226,#44227,#44228,#44229,#44230),.UNSPECIFIED.,.F.,.F.,
(4,2,2,2,2,2,2,2,2,2,2,2,2,2,2,2,2,2,2,2,2,2,2,2,2,2,2,2,2,2,2,2,2,2,2,
2,2,2,2,2,2,2,2,2,2,2,2,2,2,2,2,2,2,2,2,2,2,2,2,2,2,2,2,2,2,2,2,2,2,2,2,
2,2,2,2,2,2,2,2,2,2,2,2,2,2,2,2,2,2,2,2,2,2,2,2,2,2,2,2,2,2,2,2,2,2,2,2,
2,2,2,2,2,2,2,2,2,2,2,2,2,2,2,2,2,2,2,2,2,2,2,2,2,2,2,2,2,2,2,2,2,2,2,2,
2,2,2,2,2,2,2,2,2,2,2,2,2,2,2,2,2,2,2,2,2,2,2,2,2,2,2,4),(-20.507299559048,
-20.4750081423604,-20.423427616719,-20.3850189726539,-20.3635343236376,
-20.3423278927266,-20.3053371938717,-20.2417535837765,-20.0642492426348,
-20.0160191618219,-19.9469866841915,-19.9063916276704,-19.8684565790793,
-19.8235359106753,-19.5998889145673,-19.480904253598,-19.4509981832004,
-19.4310114714177,-19.4071392645321,-19.3553967726712,-19.1033233011638,
-19.026174929525,-18.9841940818035,-18.9467004710437,-18.897592665659,-18.7616985398062,
-18.7499181832599,-18.5964517061827,-18.5413589484032,-18.5169616415103,
-18.4970829854371,-18.4680977629777,-18.3863969883353,-18.2107771347324,
-18.1412880234492,-18.0836772949979,-18.0450702467323,-18.0102751325587,
-17.9524152039754,-17.8482896755343,-17.6949818457012,-17.6438285025493,
-17.6056452472752,-17.5842047694776,-17.5655891152944,-17.5315800762635,
-17.4616337607536,-17.2848149921297,-17.2366694582687,-17.167717391648,
-17.1271364794953,-17.089195442148,-17.0358005384335,-16.912419010596,-16.7665123516105,
-16.6943773689444,-16.6677436538751,-16.6480163172177,-16.6222726702742,
-16.5628157894647,-16.5459300492343,-16.5166574195152,-16.3535473228537,
-16.2860706759758,-16.2296386412465,-16.1912257849105,-16.1515111531045,
-16.0874885728065,-15.9778210838673,-15.7807494027894,-15.7481927004737,
-15.7280073419323,-15.705385210704,-15.6609458650914,-15.5972727980809,
-15.4113448369261,-15.3256133611883,-15.2822641229311,-15.2449872097988,
-15.1973274194708,-15.0763627005395,-14.8817611245948,-14.8329607746095,
-14.8095747422674,-14.7894515705858,-14.7585549201691,-14.7203883996381,
-14.634731627884,-14.4234290614924,-14.3765044069543,-14.3385186501703,
-14.2988284107755,-14.2349448942323,-14.123153347139,-13.9286985245183,
-13.8957537749415,-13.8773108952936,-13.8555713510835,-13.8158501977611,
-13.7617482839575,-13.5858872438347,-13.4836610011631,-13.436795019513,
-13.3995666614531,-13.3556368965417,-13.2660186282788,-13.1257014179184,
-13.0792665967161,-12.9928456922186,-12.967232109516,-12.9471267977523,
-12.9236846494042,-12.8745516636906,-12.7229885612288,-12.5656622906149,
-12.5205940942157,-12.4826291101795,-12.4421023657926,-12.3734599204552,
-12.3256393886276,-12.1514205649339,-12.0665113087927,-12.0408808137782,
-12.0207721481933,-11.9973409647251,-11.9482728184068,-11.7968123188526,
-11.6524335746977,-11.5967898492279,-11.5588838394353,-11.5190673594432,
-11.4544654554578,-11.3724391764939,-11.2672546875182,-11.2389185811808,
-11.1423377633651,-11.11296308292,-11.0930414032415,-11.0688761918549,-11.0152870292955,
-10.9303400032328,-10.7171694674061,-10.6705353715052,-10.6326143056607,
-10.5928229432139,-10.5283628987424,-10.4466021050839,-10.3410730945386,
-10.3372134355085,-10.2264782260157,-10.191829022171,-10.1731062028581,
-10.1518270378394,-10.1144639207663,-10.0648512839366,-9.92184798585374,
-9.78659161028094,-9.74152124345755,-9.70355605191445,-9.66303080138468,
-9.59439554852061,-9.5465823544125,-9.37241980257034,-9.28743000167747,
-9.26180284009967,-9.24169496852961,-9.21826197903713,-9.16918237066026,
-9.01770438184618,-8.87336864188202,-8.83945532408071),.UNSPECIFIED.) ;
#296=B_SPLINE_CURVE_WITH_KNOTS('',3,(#44231,#44232,#44233,#44234,#44235,
#44236,#44237,#44238,#44239,#44240,#44241,#44242,#44243,#44244,#44245,#44246,
#44247,#44248,#44249,#44250,#44251,#44252,#44253,#44254,#44255,#44256,#44257,
#44258,#44259,#44260,#44261,#44262,#44263,#44264,#44265,#44266,#44267,#44268,
#44269,#44270,#44271,#44272,#44273,#44274,#44275,#44276,#44277,#44278,#44279,
#44280,#44281,#44282,#44283,#44284,#44285,#44286,#44287,#44288,#44289,#44290,
#44291,#44292,#44293,#44294,#44295,#44296,#44297,#44298,#44299,#44300,#44301,
#44302,#44303,#44304,#44305,#44306,#44307,#44308,#44309,#44310,#44311,#44312,
#44313,#44314,#44315,#44316,#44317,#44318,#44319,#44320,#44321,#44322,#44323,
#44324,#44325,#44326,#44327,#44328,#44329,#44330,#44331,#44332,#44333,#44334,
#44335,#44336,#44337,#44338,#44339,#44340,#44341,#44342,#44343,#44344,#44345,
#44346,#44347,#44348,#44349,#44350,#44351,#44352,#44353,#44354,#44355,#44356,
#44357,#44358,#44359,#44360,#44361,#44362,#44363,#44364,#44365,#44366,#44367,
#44368,#44369,#44370,#44371,#44372,#44373,#44374,#44375,#44376,#44377,#44378,
#44379,#44380,#44381,#44382,#44383,#44384,#44385,#44386,#44387,#44388,#44389,
#44390,#44391,#44392,#44393,#44394,#44395,#44396,#44397,#44398,#44399,#44400,
#44401,#44402,#44403,#44404,#44405,#44406,#44407,#44408,#44409,#44410,#44411,
#44412,#44413,#44414,#44415,#44416,#44417,#44418,#44419,#44420,#44421,#44422,
#44423,#44424,#44425,#44426,#44427,#44428,#44429,#44430,#44431,#44432,#44433,
#44434,#44435,#44436,#44437,#44438,#44439,#44440,#44441,#44442,#44443,#44444,
#44445,#44446,#44447,#44448,#44449,#44450,#44451,#44452,#44453,#44454,#44455,
#44456,#44457,#44458,#44459,#44460,#44461,#44462,#44463,#44464,#44465,#44466,
#44467,#44468,#44469,#44470,#44471,#44472,#44473,#44474,#44475,#44476,#44477,
#44478,#44479,#44480,#44481,#44482,#44483,#44484,#44485,#44486,#44487,#44488,
#44489,#44490,#44491,#44492,#44493,#44494,#44495,#44496,#44497,#44498,#44499,
#44500,#44501,#44502,#44503,#44504,#44505,#44506,#44507,#44508,#44509,#44510,
#44511,#44512,#44513,#44514,#44515,#44516,#44517,#44518,#44519,#44520,#44521,
#44522,#44523,#44524,#44525,#44526,#44527,#44528,#44529,#44530,#44531,#44532,
#44533,#44534,#44535,#44536,#44537,#44538,#44539,#44540,#44541,#44542,#44543,
#44544,#44545,#44546,#44547,#44548,#44549,#44550,#44551,#44552,#44553,#44554,
#44555,#44556,#44557,#44558,#44559,#44560,#44561,#44562,#44563,#44564,#44565,
#44566,#44567,#44568),.UNSPECIFIED.,.F.,.F.,(4,2,2,2,2,2,2,2,2,2,2,2,2,
2,2,2,2,2,2,2,2,2,2,2,2,2,2,2,2,2,2,2,2,2,2,2,2,2,2,2,2,2,2,2,2,2,2,2,2,
2,2,2,2,2,2,2,2,2,2,2,2,2,2,2,2,2,2,2,2,2,2,2,2,2,2,2,2,2,2,2,2,2,2,2,2,
2,2,2,2,2,2,2,2,2,2,2,2,2,2,2,2,2,2,2,2,2,2,2,2,2,2,2,2,2,2,2,2,2,2,2,2,
2,2,2,2,2,2,2,2,2,2,2,2,2,2,2,2,2,2,2,2,2,2,2,2,2,2,2,2,2,2,2,2,2,2,2,2,
2,2,2,2,2,2,2,2,2,2,2,4),(-14.4955154817265,-14.4921015805046,-14.4429921461233,
-14.4195542924433,-14.3994482342011,-14.3738293341153,-14.288601347128,
-14.1640202039879,-14.0702953232699,-13.9997138545117,-13.9588497000149,
-13.9210256786476,-13.8684426683958,-13.6625403707464,-13.5428991907983,
-13.5076878109589,-13.4868239037886,-13.4677532750718,-13.431095049103,
-13.3668216546039,-13.1893972668873,-13.1411775992524,-13.0721555325839,
-13.031562936377,-12.9936280679082,-12.9402713709789,-12.7403375790634,
-12.6172144382479,-12.5816262233561,-12.5606908888506,-12.5416892169662,
-12.5054232410481,-12.4403274337214,-12.2629929906486,-12.214784389061,
-12.1457728406979,-12.1051820907638,-12.0672464351001,-12.0138842923567,
-11.8137937063797,-11.72283332356,-11.6669536294428,-11.6424376059487,-11.622578985395,
-11.5937850759278,-11.4970168396412,-11.3138423765389,-11.2293454773349,
-11.1861864978242,-11.1492448225963,-11.1015126039201,-10.9797513977014,
-10.8558786437209,-10.7526483369395,-10.7230915832855,-10.7031486968195,
-10.6790875506406,-10.6261588459311,-10.5428876384062,-10.4659573371001,
-10.3239452887559,-10.2784953828644,-10.2408278191866,-10.2005761398127,
-10.1334984835463,-10.0873016961473,-9.92521685684855,-9.82588359837368,
-9.79652907563537,-9.7766100200221,-9.75243390964364,-9.69877316019389,
-9.6136419842748,-9.40095006549675,-9.35424691911125,-9.31631112205278,
-9.27654532718786,-9.21222764979518,-9.00669827909516,-8.90102697631658,
-8.870950534164,-8.85094220246908,-8.8271601757043,-8.77597140710462,-8.69700263764407,
-8.46928380234722,-8.42013382164952,-8.38263617210211,-8.34067919193864,
-8.26366977592732,-8.15608774708344,-7.97944719429653,-7.94700264990251,
-7.92683636024456,-7.90417502294572,-7.85951623847511,-7.79537636151634,
-7.54889819588217,-7.49676299144869,-7.45900141417797,-7.4179697725824,
-7.34641793604392,-7.25069311358847,-7.12587250001796,-7.05699974038036,
-7.02250120812312,-7.00380417152983,-6.98248919080206,-6.94494191718322,
-6.8949846511611,-6.74974558110172,-6.62506639957466,-6.57186842119787,
-6.53395716584005,-6.49331174479136,-6.42398451921839,-6.37544251481086,
-6.19536113237998,-6.15273948416572,-6.10950881197842,-6.08472608306475,
-6.06490585258803,-6.0365181463832,-5.94548206320116,-5.69430151266495,
-5.64802322418462,-5.61018064190618,-5.57026049271225,-5.50506440693273,
-5.46078067688279,-5.31151435228598,-5.28830411326515,-5.19347775773949,
-5.16436847469594,-5.1444771683531,-5.12015698276449,-5.06556431195823,
-4.97801994561764,-4.77113274387754,-4.71844772505787,-4.68061005017704,
-4.6397844335495,-4.56942128337941,-4.47614069820228,-4.27632410469421,
-4.24266710881524,-4.2241099891639,-4.20257635055,-4.16391381474872,-4.11184919599735,
-3.95199560771034,-3.88371022260167,-3.811129721386,-3.76992120239732,-3.73221979722566,
-3.68053162209566,-3.50682596208475,-3.34957756713854,-3.31613220568713,
-3.29760956654551,-3.27601709180426,-3.23705248412017,-3.18441010424254,
-3.02022349162204,-3.00028739678404,-2.95464433693914,-2.88364754025106,
-2.8427119762498,-2.82789765027506),.UNSPECIFIED.) ;
#297=B_SPLINE_CURVE_WITH_KNOTS('',3,(#44573,#44574,#44575,#44576,#44577,
#44578,#44579,#44580,#44581,#44582,#44583,#44584,#44585,#44586,#44587,#44588,
#44589,#44590,#44591,#44592,#44593,#44594,#44595,#44596,#44597,#44598,#44599,
#44600,#44601,#44602,#44603,#44604,#44605,#44606,#44607,#44608,#44609,#44610,
#44611,#44612,#44613,#44614,#44615,#44616,#44617,#44618,#44619,#44620,#44621,
#44622,#44623,#44624,#44625,#44626,#44627,#44628,#44629,#44630,#44631,#44632,
#44633,#44634,#44635,#44636,#44637,#44638,#44639,#44640,#44641,#44642,#44643,
#44644,#44645,#44646,#44647,#44648,#44649,#44650,#44651,#44652,#44653,#44654,
#44655,#44656,#44657,#44658,#44659,#44660,#44661,#44662,#44663,#44664,#44665,
#44666,#44667,#44668,#44669,#44670,#44671,#44672,#44673,#44674,#44675,#44676,
#44677,#44678,#44679,#44680,#44681,#44682,#44683,#44684,#44685,#44686,#44687,
#44688,#44689,#44690,#44691,#44692,#44693,#44694,#44695,#44696,#44697,#44698,
#44699,#44700,#44701,#44702,#44703,#44704,#44705,#44706,#44707,#44708,#44709,
#44710,#44711,#44712,#44713,#44714,#44715,#44716,#44717,#44718,#44719,#44720,
#44721,#44722,#44723,#44724,#44725,#44726,#44727,#44728,#44729,#44730,#44731,
#44732,#44733,#44734,#44735,#44736,#44737,#44738,#44739,#44740,#44741,#44742,
#44743,#44744,#44745,#44746,#44747,#44748,#44749,#44750,#44751,#44752,#44753,
#44754,#44755,#44756,#44757,#44758,#44759,#44760,#44761,#44762,#44763,#44764,
#44765,#44766,#44767,#44768,#44769,#44770,#44771,#44772,#44773,#44774,#44775,
#44776,#44777,#44778,#44779,#44780,#44781,#44782,#44783,#44784,#44785,#44786,
#44787,#44788,#44789,#44790,#44791,#44792,#44793,#44794,#44795,#44796,#44797,
#44798,#44799,#44800,#44801,#44802,#44803,#44804,#44805,#44806,#44807,#44808,
#44809,#44810,#44811,#44812,#44813,#44814,#44815,#44816,#44817,#44818,#44819,
#44820,#44821,#44822,#44823,#44824,#44825,#44826,#44827,#44828,#44829,#44830,
#44831,#44832,#44833,#44834,#44835,#44836,#44837,#44838,#44839,#44840,#44841,
#44842,#44843,#44844,#44845,#44846,#44847,#44848,#44849,#44850,#44851,#44852,
#44853,#44854,#44855,#44856,#44857,#44858,#44859,#44860,#44861,#44862,#44863,
#44864,#44865,#44866,#44867,#44868,#44869,#44870,#44871,#44872,#44873,#44874,
#44875,#44876,#44877,#44878,#44879,#44880,#44881,#44882,#44883,#44884,#44885,
#44886,#44887,#44888,#44889,#44890,#44891,#44892,#44893,#44894,#44895,#44896,
#44897,#44898,#44899,#44900,#44901,#44902,#44903,#44904,#44905,#44906,#44907,
#44908,#44909,#44910,#44911,#44912,#44913,#44914,#44915,#44916,#44917,#44918),
 .UNSPECIFIED.,.F.,.F.,(4,2,2,2,2,2,2,2,2,2,2,2,2,2,2,2,2,2,2,2,2,2,2,2,
2,2,2,2,2,2,2,2,2,2,2,2,2,2,2,2,2,2,2,2,2,2,2,2,2,2,2,2,2,2,2,2,2,2,2,2,
2,2,2,2,2,2,2,2,2,2,2,2,2,2,2,2,2,2,2,2,2,2,2,2,2,2,2,2,2,2,2,2,2,2,2,2,
2,2,2,2,2,2,2,2,2,2,2,2,2,2,2,2,2,2,2,2,2,2,2,2,2,2,2,2,2,2,2,2,2,2,2,2,
2,2,2,2,2,2,2,2,2,2,2,2,2,2,2,2,2,2,2,2,2,2,2,2,2,2,2,2,2,2,2,2,2,2,2,2,
2,2,2,2,4),(-32.1750764478982,-32.0207553169334,-31.9813013241376,-31.9464178057449,
-31.908516085165,-31.8528969676883,-31.7086263720659,-31.528646642724,-31.50065638766,
-31.4844759542813,-31.4643647427817,-31.4387206369914,-31.3514941384981,
-31.311554194876,-31.1674620938463,-31.1035194047997,-31.0526466261229,
-31.0202426277755,-30.982368352764,-30.9359472703877,-30.7210857662802,
-30.6368557993027,-30.583548018481,-30.5594269537457,-30.5394963850721,
-30.5100449398096,-30.4022393723395,-30.1991173198759,-30.1339423933532,
-30.0940252284562,-30.0561793152143,-30.0098890417771,-29.7932611781259,
-29.7099323537193,-29.6569805222344,-29.6329154869372,-29.6129730635167,
-29.5834221965595,-29.4801056572308,-29.3562335811888,-29.2345293742903,
-29.1868019031081,-29.1495203415574,-29.1062179339575,-29.0207918920525,
-28.8343326620093,-28.7706960958894,-28.7262741198875,-28.7036552199766,
-28.6834685260311,-28.6509033227743,-28.5777361234241,-28.401253769229,
-28.353149973984,-28.2842376816045,-28.2436638265746,-28.2057199008725,
-28.1607545267688,-28.0218099534825,-27.8813989465371,-27.8321944101105,
-27.7950504506345,-27.7738141644002,-27.7550604070396,-27.7202293332302,
-27.6058088560617,-27.4618746577715,-27.4184490615059,-27.3541096608302,
-27.3143393972536,-27.2764049412821,-27.2205804084513,-27.0290266593841,
-26.93605909713,-26.8794407852576,-26.854814205345,-26.8349718752996,-26.8063482614371,
-26.7158171125605,-26.5461617183768,-26.4776028718446,-26.4205351055321,
-26.3820181525979,-26.342452768001,-26.2792789873513,-26.1887963941779,
-26.0330924962666,-25.9815993865763,-25.943236842607,-25.9217612811732,
-25.9031676436787,-25.8692915243263,-25.7699242773961,-25.7507713551287,
-25.741627264221,-25.7347998279155,-25.6029889384459,-25.541658071247,-25.4889197060988,
-25.4510732424879,-25.4102644316514,-25.3400047891248,-25.2663898578329,
-25.10757207869,-25.0556471834723,-25.0170575511103,-24.9955375930234,-24.9769710303939,
-24.9432595549775,-24.872657806435,-24.6959079620363,-24.6477709588806,
-24.578827011004,-24.5382475283352,-24.500305885695,-24.4553522124513,-24.2326711685105,
-24.1128746462818,-24.0829405635136,-24.0629503166061,-24.0390930462161,
-23.9874427598014,-23.7352330484433,-23.6580864573933,-23.6161060135417,
-23.5786124867964,-23.5295043894913,-23.3936060694109,-23.3818356569591,
-23.2308869698538,-23.1740059759665,-23.1493405565464,-23.1295038312328,
-23.1009394119394,-23.0118351682198,-22.9703946806594,-22.96247501611,-22.8261832729238,
-22.7840556958983,-22.7210293050245,-22.6814898249792,-22.6434024408258,
-22.5866202859186,-22.4795778109928,-22.4528044631825,-22.3823183919003,
-22.2989789741983,-22.2460228294659,-22.2219570243986,-22.2020146247,-22.1724647241394,
-22.0691279808191,-21.9452553811855,-21.8619640131505,-21.7966901863892,
-21.7567553066748,-21.7189189361172,-21.6726741164618,-21.4550916503824,
-21.3722880192855,-21.3195447577275,-21.2955125674727,-21.275562763714,
-21.2459521953679,-21.1430964664194,-20.9839239494493,-20.9171302953464,
-20.8611017335229,-20.8227540765982,-20.7829394768408,-20.7183494474712,
-20.6313350432498,-20.507299559048),.UNSPECIFIED.) ;
#298=B_SPLINE_CURVE_WITH_KNOTS('',3,(#44920,#44921,#44922,#44923,#44924,
#44925,#44926,#44927,#44928,#44929,#44930,#44931,#44932,#44933,#44934,#44935,
#44936,#44937,#44938,#44939,#44940,#44941,#44942,#44943,#44944,#44945,#44946,
#44947,#44948,#44949,#44950,#44951,#44952,#44953,#44954,#44955,#44956,#44957,
#44958,#44959,#44960,#44961,#44962,#44963,#44964,#44965,#44966,#44967,#44968,
#44969,#44970,#44971,#44972,#44973,#44974,#44975,#44976,#44977,#44978,#44979,
#44980,#44981,#44982,#44983,#44984,#44985,#44986,#44987,#44988,#44989,#44990,
#44991,#44992,#44993,#44994,#44995,#44996,#44997,#44998,#44999,#45000,#45001,
#45002,#45003,#45004,#45005,#45006,#45007,#45008,#45009,#45010,#45011,#45012,
#45013,#45014,#45015,#45016,#45017,#45018,#45019,#45020,#45021,#45022,#45023,
#45024,#45025,#45026,#45027,#45028,#45029,#45030,#45031,#45032,#45033,#45034,
#45035,#45036,#45037,#45038,#45039,#45040,#45041,#45042,#45043,#45044,#45045),
 .UNSPECIFIED.,.F.,.F.,(4,2,2,2,2,2,2,2,2,2,2,2,2,2,2,2,2,2,2,2,2,2,2,2,
2,2,2,2,2,2,2,2,2,2,2,2,2,2,2,2,2,2,2,2,2,2,2,2,2,2,2,2,2,2,2,2,2,2,2,2,
2,2,4),(-2.82789765027506,-2.80491587923842,-2.75252875979998,-2.69176955209418,
-2.56248106626684,-2.4257920012106,-2.39100182663586,-2.37225547168151,
-2.3510106267097,-2.31382050770316,-2.26452956679996,-2.12356759474721,
-1.98524905487421,-1.94032515680157,-1.9023906560633,-1.86179967690516,
-1.79278379025566,-1.7445701196702,-1.56719242407696,-1.50250281169606,
-1.46604416157332,-1.44700891037799,-1.43290375683057,-1.41340814401782,
-1.41297209775783,-1.41248755497472,-1.4119487288995,-1.41134908705566,
-1.41068125200755,-1.4099368906042,-1.40910659127049,-1.408179729461,-1.40714432181633,
-1.40598687042924,-1.40469219953839,-1.40324328826263,-1.40162110455089,
-1.399804447703,-1.39898693511867,-1.39786866932377,-1.39634240263808,-1.39426620597236,
-1.39145600046461,-1.38768037979173,-1.33858895621796,-1.19887936310669,
-1.05917041085551,-1.01013404551959,-0.978758906063135,-0.939967697712623,
-0.899290885858743,-0.731746744846582,-0.569941484339615,-0.536828717737774,
-0.518359610198079,-0.500213170638933,-0.478073369992099,-0.395171047276128,
-0.210481860352328,-0.118823237187442,-0.0747521515350052,-0.040571949127146,
-1.0000000096877E-6),.UNSPECIFIED.) ;
#299=B_SPLINE_CURVE_WITH_KNOTS('',3,(#45046,#45047,#45048,#45049,#45050,
#45051,#45052,#45053,#45054,#45055,#45056,#45057,#45058,#45059,#45060,#45061,
#45062,#45063,#45064,#45065,#45066,#45067,#45068,#45069,#45070,#45071,#45072,
#45073,#45074,#45075,#45076,#45077,#45078,#45079,#45080,#45081,#45082,#45083,
#45084,#45085,#45086,#45087,#45088,#45089,#45090,#45091,#45092,#45093,#45094,
#45095,#45096,#45097,#45098,#45099,#45100,#45101,#45102,#45103,#45104,#45105,
#45106,#45107,#45108,#45109,#45110,#45111,#45112,#45113,#45114,#45115,#45116,
#45117,#45118,#45119,#45120,#45121,#45122,#45123,#45124,#45125,#45126,#45127,
#45128,#45129,#45130,#45131,#45132,#45133,#45134,#45135,#45136,#45137,#45138,
#45139,#45140,#45141,#45142,#45143,#45144,#45145,#45146,#45147,#45148,#45149,
#45150,#45151,#45152,#45153,#45154,#45155,#45156,#45157,#45158,#45159,#45160,
#45161,#45162,#45163,#45164,#45165,#45166,#45167,#45168,#45169,#45170,#45171,
#45172,#45173,#45174,#45175,#45176,#45177,#45178,#45179,#45180,#45181,#45182,
#45183,#45184,#45185,#45186,#45187,#45188,#45189,#45190,#45191,#45192,#45193,
#45194,#45195,#45196,#45197,#45198,#45199,#45200,#45201,#45202,#45203,#45204,
#45205,#45206,#45207,#45208,#45209,#45210,#45211,#45212,#45213,#45214,#45215,
#45216,#45217,#45218,#45219,#45220,#45221,#45222,#45223,#45224,#45225,#45226,
#45227,#45228,#45229,#45230,#45231,#45232,#45233,#45234,#45235,#45236,#45237,
#45238,#45239,#45240,#45241,#45242,#45243,#45244,#45245,#45246,#45247,#45248,
#45249,#45250,#45251,#45252,#45253,#45254,#45255,#45256,#45257,#45258,#45259,
#45260,#45261,#45262,#45263,#45264,#45265,#45266,#45267,#45268,#45269,#45270,
#45271,#45272,#45273,#45274,#45275,#45276,#45277,#45278,#45279,#45280,#45281,
#45282,#45283,#45284,#45285,#45286,#45287,#45288,#45289,#45290,#45291,#45292,
#45293,#45294,#45295,#45296,#45297,#45298,#45299,#45300,#45301,#45302,#45303,
#45304,#45305,#45306,#45307,#45308,#45309,#45310,#45311,#45312,#45313,#45314,
#45315,#45316,#45317),.UNSPECIFIED.,.F.,.F.,(4,2,2,2,2,2,2,2,2,2,2,2,2,
2,2,2,2,2,2,2,2,2,2,2,2,2,2,2,2,2,2,2,2,2,2,2,2,2,2,2,2,2,2,2,2,2,2,2,2,
2,2,2,2,2,2,2,2,2,2,2,2,2,2,2,2,2,2,2,2,2,2,2,2,2,2,2,2,2,2,2,2,2,2,2,2,
2,2,2,2,2,2,2,2,2,2,2,2,2,2,2,2,2,2,2,2,2,2,2,2,2,2,2,2,2,2,2,2,2,2,2,2,
2,2,2,2,2,2,2,2,2,2,2,2,2,2,4),(-32.1748014029942,-32.1217728507451,-31.9110886571694,
-31.8419207857683,-31.8081973307716,-31.7862618783361,-31.768148047931,
-31.7495648135089,-31.7157486512336,-31.5633091967486,-31.38845875213,-31.3476096594065,
-31.3108449372146,-31.2737290336029,-31.2225437870683,-30.988005450012,
-30.9168700971781,-30.8825836466127,-30.8604407612231,-30.8462404556041,
-30.826136254408,-30.800525326171,-30.7149601337697,-30.5412074560776,-30.493447215244,
-30.4248631121917,-30.3843476135401,-30.3463795865153,-30.3012915074843,
-30.1658223922661,-30.0230260151101,-29.9734461993299,-29.9361010365137,
-29.914825787547,-29.8961011411747,-29.8614390598299,-29.7273293862152,
-29.7224373879445,-29.5944797563901,-29.5092229360122,-29.4659474170641,
-29.4286642699448,-29.3809007063307,-29.26930398573,-29.1030759131334,-29.0648794349637,
-29.0165932222484,-28.9932951386548,-28.9733737771776,-28.9476916629009,
-28.8599036583143,-28.6879315104497,-28.6403993924543,-28.5720333676748,
-28.5315559770895,-28.4935704548857,-28.4483976917787,-28.3119117671141,
-28.1700738139059,-28.120644190398,-28.0833795867322,-28.0621201037945,
-28.0433841629174,-28.0086556193548,-27.9402827661942,-27.7633040379646,
-27.7151396875567,-27.6461705627761,-27.6055876893548,-27.5676495011915,
-27.5142667021209,-27.3138048905067,-27.2231239297503,-27.1673484243307,
-27.142848279012,-27.122987437994,-27.0941693815941,-27.001789726951,-26.9644116148836,
-26.8227021794838,-26.7796467122456,-26.7156803233494,-26.6759764936705,
-26.6380017183422,-26.5911221199755,-26.3795562256849,-26.2939997356236,
-26.2401733721356,-26.2159715214406,-26.1960576758965,-26.1667478737976,
-26.0682502219196,-26.0515086166581,-26.0468111029761,-25.8991525652874,
-25.8345017653895,-25.7797511522522,-25.7416064300295,-25.7063078392734,
-25.6451885867517,-25.5495665681602,-25.3947774519404,-25.3434140562006,
-25.3051201934907,-25.2836584378892,-25.2650570506229,-25.2311319733638,
-25.1306762208981,-24.9504184135711,-24.8730075399343,-24.8309839665196,
-24.793501035518,-24.7444780002106,-24.6093877280885,-24.4653617847604,
-24.3936680835194,-24.3670843235507,-24.3473580894345,-24.321569669536,
-24.2581952288189,-24.2460425931659,-24.0605977208903,-23.9896890169054,
-23.9312566816054,-23.8925125734221,-23.8578371470493,-23.8007681670583,
-23.694515025,-23.6675550360273,-23.5971764338513,-23.5137804818024,-23.4608024520918,
-23.4367336088587,-23.4167925289507,-23.3872499858046,-23.3353232287531),
 .UNSPECIFIED.) ;
#300=B_SPLINE_CURVE_WITH_KNOTS('',3,(#45322,#45323,#45324,#45325,#45326,
#45327,#45328,#45329,#45330,#45331,#45332,#45333,#45334,#45335,#45336,#45337,
#45338,#45339,#45340,#45341,#45342,#45343,#45344,#45345,#45346,#45347,#45348,
#45349,#45350,#45351,#45352,#45353,#45354,#45355,#45356,#45357,#45358,#45359,
#45360,#45361,#45362,#45363,#45364,#45365,#45366,#45367,#45368,#45369,#45370,
#45371,#45372,#45373,#45374,#45375,#45376,#45377,#45378,#45379,#45380,#45381,
#45382,#45383,#45384,#45385,#45386,#45387,#45388,#45389,#45390,#45391,#45392,
#45393,#45394,#45395,#45396,#45397,#45398,#45399,#45400,#45401,#45402,#45403,
#45404,#45405,#45406,#45407,#45408,#45409,#45410,#45411,#45412,#45413,#45414,
#45415,#45416,#45417,#45418,#45419,#45420,#45421,#45422,#45423,#45424,#45425,
#45426,#45427,#45428,#45429,#45430,#45431,#45432,#45433,#45434,#45435,#45436,
#45437,#45438,#45439,#45440,#45441,#45442,#45443,#45444,#45445,#45446,#45447,
#45448,#45449,#45450,#45451,#45452,#45453,#45454,#45455,#45456,#45457,#45458,
#45459,#45460,#45461,#45462,#45463,#45464,#45465,#45466,#45467,#45468,#45469,
#45470,#45471,#45472,#45473,#45474,#45475,#45476,#45477,#45478,#45479,#45480,
#45481,#45482,#45483,#45484,#45485,#45486,#45487,#45488,#45489,#45490,#45491,
#45492,#45493,#45494,#45495,#45496,#45497,#45498,#45499,#45500,#45501,#45502,
#45503,#45504,#45505,#45506,#45507,#45508,#45509,#45510,#45511,#45512,#45513,
#45514,#45515,#45516,#45517,#45518,#45519,#45520,#45521,#45522,#45523,#45524,
#45525,#45526,#45527,#45528,#45529,#45530,#45531,#45532,#45533,#45534,#45535,
#45536,#45537,#45538,#45539,#45540,#45541,#45542,#45543,#45544,#45545,#45546,
#45547,#45548,#45549,#45550,#45551,#45552,#45553,#45554,#45555,#45556,#45557,
#45558,#45559,#45560,#45561,#45562,#45563,#45564,#45565,#45566,#45567,#45568,
#45569,#45570,#45571,#45572,#45573,#45574,#45575,#45576,#45577,#45578,#45579,
#45580,#45581,#45582,#45583,#45584,#45585,#45586,#45587,#45588,#45589,#45590,
#45591,#45592,#45593,#45594,#45595,#45596,#45597,#45598,#45599,#45600,#45601,
#45602,#45603,#45604,#45605,#45606,#45607,#45608,#45609,#45610,#45611,#45612,
#45613,#45614,#45615,#45616,#45617,#45618,#45619,#45620,#45621,#45622,#45623,
#45624,#45625,#45626,#45627,#45628,#45629,#45630,#45631,#45632,#45633,#45634,
#45635,#45636,#45637,#45638,#45639,#45640,#45641,#45642,#45643,#45644,#45645,
#45646,#45647,#45648,#45649,#45650,#45651,#45652,#45653,#45654,#45655,#45656,
#45657,#45658,#45659,#45660,#45661,#45662,#45663,#45664,#45665,#45666,#45667,
#45668,#45669,#45670,#45671,#45672,#45673,#45674,#45675,#45676,#45677,#45678,
#45679,#45680,#45681,#45682,#45683,#45684,#45685),.UNSPECIFIED.,.F.,.F.,
(4,2,2,2,2,2,2,2,2,2,2,2,2,2,2,2,2,2,2,2,2,2,2,2,2,2,2,2,2,2,2,2,2,2,2,
2,2,2,2,2,2,2,2,2,2,2,2,2,2,2,2,2,2,2,2,2,2,2,2,2,2,2,2,2,2,2,2,2,2,2,2,
2,2,2,2,2,2,2,2,2,2,2,2,2,2,2,2,2,2,2,2,2,2,2,2,2,2,2,2,2,2,2,2,2,2,2,2,
2,2,2,2,2,2,2,2,2,2,2,2,2,2,2,2,2,2,2,2,2,2,2,2,2,2,2,2,2,2,2,2,2,2,2,2,
2,2,2,2,2,2,2,2,2,2,2,2,2,2,2,2,2,2,2,2,2,2,2,2,2,2,2,2,2,2,2,2,2,2,2,2,
2,2,4),(-11.667685703203,-11.5974316070097,-11.4728113815751,-11.388239375587,
-11.3625934376122,-11.3424815815118,-11.319060060456,-11.2700497058543,
-11.1186800799611,-10.9741112869419,-10.9184720436934,-10.8805665823937,
-10.8407486584663,-10.7761394093138,-10.6940995674359,-10.5889317420429,
-10.560638938262,-10.4639551648775,-10.434611881157,-10.4146937354645,-10.3905101640877,
-10.3368039476596,-10.2515574620737,-10.0391562301076,-9.99240706610917,
-9.95446045546595,-9.91470958945891,-9.85048049035179,-9.80716463512985,
-9.66389607316894,-9.60090983144109,-9.53199958485302,-9.50773402142319,
-9.48786273237982,-9.46342260346886,-9.40804740665859,-9.31843932378605,
-9.11610453475213,-9.06281925821977,-9.02489446901323,-8.98427710712707,
-8.91511519644477,-8.86674841066104,-8.68812478378421,-8.634248218679,-8.59242807224055,
-8.57028917102263,-8.54958726553916,-8.51524638483093,-8.49188971516608,
-8.45358188185071,-8.28631500837497,-8.1761112626246,-8.12830621713902,
-8.09101892603745,-8.04776902200252,-7.96268558383584,-7.83519696495176,
-7.8234755887839,-7.69552189760284,-7.6608178807833,-7.64208571903125,-7.6208195215608,
-7.58352282643212,-7.534034126159,-7.39182402862126,-7.25572991788653,-7.21058800169032,
-7.17260798260029,-7.13211490016285,-7.06366418059457,-7.01604423487268,
-6.84339802489378,-6.75638356189347,-6.73075018124856,-6.71064099122271,
-6.68721180492634,-6.63815517092944,-6.48671312983415,-6.34229597796817,
-6.28665432214012,-6.24874874692571,-6.20893193690682,-6.14432754988181,
-6.06229646880678,-5.95711908004927,-5.92880045397095,-5.83218829117392,
-5.80282200565116,-5.78290135902911,-5.75873146098656,-5.70511192280679,
-5.62008699319999,-5.40711588233199,-5.36045309394554,-5.32252581126531,
-5.28274489541692,-5.218343590184,-5.13669251266178,-5.03102307268413,-4.99997135019261,
-4.90524538946022,-4.8761473308443,-4.85625684222584,-4.83192888097718,
-4.77728807338461,-4.73106933108943,-4.47938065706351,-4.43322146343006,
-4.39540410139643,-4.35543780296601,-4.28998247231869,-4.20634634088272,
-4.08246684328929,-3.98054395488003,-3.95065546503768,-3.93067143708637,
-3.90679098702943,-3.85499474867049,-3.77454239226924,-3.54947440591486,
-3.50021681022972,-3.46270630537767,-3.42080451150579,-3.34412770873095,
-3.28743684411569,-3.18009978881906,-3.16543813015873,-3.0625413429593,
-3.02845485427676,-3.00982669158184,-2.9884072310827,-2.9503292557538,-2.8993744629628,
-2.74743795751088,-2.63545496828495,-2.58044893052033,-2.54264267093298,
-2.50265725830496,-2.43709231660903,-2.23104960744161,-2.12711269220111,
-2.09755713542059,-2.077614443664,-2.05355275275202,-2.0006202909316,-1.91733945460583,
-1.70063633900036,-1.6543508588316,-1.6165064788147,-1.57658853522894,-1.51140636916261,
-1.42828700664986,-1.32457658289954,-1.28695820099813,-1.1986314477956,
-1.17005474682505,-1.15021734082862,-1.14858911206641,-1.14728987946515,
-1.14654805879147,-1.14612909829587,-1.14522873617732,-1.14441150981607,
-1.14366947301655,-1.1429954656423,-1.1156623398666,-1.02845255432607,-0.776871849066619,
-0.724417052628229,-0.686611486371154,-0.649544161006118,-0.63311295881949,
-0.607229325938222,-0.455355961206685,-0.278739403615303,-0.247060802035675,
-0.227017815742242,-0.208598596012939,-0.185182493756475,-0.147428453795999,
-1.00000001260203E-6),.UNSPECIFIED.) ;
#301=B_SPLINE_CURVE_WITH_KNOTS('',3,(#45686,#45687,#45688,#45689,#45690,
#45691,#45692,#45693,#45694,#45695,#45696,#45697,#45698,#45699,#45700,#45701,
#45702,#45703,#45704,#45705,#45706,#45707,#45708,#45709,#45710,#45711,#45712,
#45713,#45714,#45715,#45716,#45717,#45718,#45719,#45720,#45721,#45722,#45723,
#45724,#45725,#45726,#45727,#45728,#45729,#45730,#45731,#45732,#45733,#45734,
#45735,#45736,#45737,#45738,#45739,#45740,#45741,#45742,#45743,#45744,#45745,
#45746,#45747,#45748,#45749,#45750,#45751,#45752,#45753,#45754,#45755,#45756,
#45757,#45758,#45759,#45760,#45761,#45762,#45763,#45764,#45765,#45766,#45767,
#45768,#45769,#45770,#45771,#45772,#45773,#45774,#45775,#45776,#45777,#45778,
#45779,#45780,#45781,#45782,#45783,#45784,#45785,#45786,#45787,#45788,#45789,
#45790,#45791,#45792,#45793,#45794,#45795,#45796,#45797,#45798,#45799,#45800,
#45801,#45802,#45803,#45804,#45805,#45806,#45807,#45808,#45809,#45810,#45811,
#45812,#45813,#45814,#45815,#45816,#45817,#45818,#45819,#45820,#45821,#45822,
#45823,#45824,#45825,#45826,#45827,#45828,#45829,#45830,#45831,#45832,#45833,
#45834,#45835,#45836,#45837,#45838,#45839,#45840,#45841,#45842,#45843,#45844,
#45845,#45846,#45847,#45848,#45849,#45850,#45851,#45852,#45853,#45854,#45855,
#45856,#45857,#45858,#45859,#45860,#45861,#45862,#45863,#45864,#45865,#45866,
#45867,#45868,#45869,#45870,#45871,#45872,#45873,#45874,#45875,#45876,#45877,
#45878,#45879,#45880,#45881,#45882,#45883,#45884,#45885,#45886,#45887,#45888,
#45889,#45890,#45891,#45892,#45893,#45894,#45895,#45896,#45897,#45898,#45899,
#45900,#45901,#45902,#45903,#45904,#45905,#45906,#45907,#45908,#45909,#45910,
#45911,#45912,#45913,#45914,#45915,#45916,#45917,#45918,#45919,#45920,#45921,
#45922,#45923,#45924,#45925,#45926,#45927,#45928,#45929,#45930,#45931,#45932,
#45933,#45934,#45935,#45936,#45937,#45938,#45939,#45940,#45941,#45942,#45943,
#45944,#45945,#45946,#45947,#45948,#45949,#45950,#45951,#45952,#45953,#45954,
#45955,#45956,#45957,#45958,#45959,#45960,#45961,#45962,#45963,#45964,#45965,
#45966,#45967,#45968,#45969,#45970,#45971,#45972,#45973,#45974,#45975,#45976,
#45977,#45978,#45979,#45980,#45981,#45982,#45983,#45984,#45985,#45986,#45987,
#45988,#45989,#45990,#45991,#45992,#45993,#45994,#45995,#45996,#45997,#45998,
#45999,#46000,#46001,#46002,#46003,#46004,#46005,#46006,#46007,#46008,#46009,
#46010,#46011,#46012,#46013,#46014,#46015,#46016,#46017,#46018,#46019,#46020,
#46021),.UNSPECIFIED.,.F.,.F.,(4,2,2,2,2,2,2,2,2,2,2,2,2,2,2,2,2,2,2,2,
2,2,2,2,2,2,2,2,2,2,2,2,2,2,2,2,2,2,2,2,2,2,2,2,2,2,2,2,2,2,2,2,2,2,2,2,
2,2,2,2,2,2,2,2,2,2,2,2,2,2,2,2,2,2,2,2,2,2,2,2,2,2,2,2,2,2,2,2,2,2,2,2,
2,2,2,2,2,2,2,2,2,2,2,2,2,2,2,2,2,2,2,2,2,2,2,2,2,2,2,2,2,2,2,2,2,2,2,2,
2,2,2,2,2,2,2,2,2,2,2,2,2,2,2,2,2,2,2,2,2,2,2,2,2,2,2,2,2,2,2,2,2,2,2,2,
2,2,2,4),(-23.3353232287531,-23.2836336843603,-23.1597669879378,-23.0766117993692,
-23.011410553683,-22.9714892140942,-22.9336466929956,-22.8873700048232,
-22.670465504122,-22.5872940294445,-22.5344049672141,-22.5103501075281,
-22.4904059026293,-22.4608380148715,-22.3566770690333,-22.2328149271518,
-22.1499579392554,-22.0849145359343,-22.0450208533294,-22.0071619949999,
-21.960810602154,-21.7436000868795,-21.6607478120452,-21.6079856022095,
-21.5839507497518,-21.5640020783355,-21.5343979004054,-21.4297222106453,
-21.2718411334518,-21.226248649101,-21.1597606128989,-21.1196124854158,
-21.0818928015084,-21.0274569293033,-20.84005715869,-20.6974413726604,-20.6667214742891,
-20.6466243023904,-20.6231575702143,-20.5738766568391,-20.4832057966711,
-20.3393116945671,-20.2958929918039,-20.231560821376,-20.1917922543951,
-20.1538576769389,-20.1071610683738,-19.8944172125292,-19.8093027510303,
-19.7556483783176,-19.7314731302676,-19.7115536997074,-19.6821971135982,
-19.5828258142415,-19.4207723138667,-19.3745799675933,-19.3075064088695,
-19.26725522758,-19.2295869505261,-19.1841347141394,-19.0419469538013,-18.9050282021086,
-18.8350619139842,-18.8086754926488,-18.7908855514234,-18.7657158095996,
-18.7086357071888,-18.6297396143924,-18.5230143732836,-18.442334207463,
-18.3784539759465,-18.3387648031809,-18.3007794290804,-18.253854408906,
-18.0382158373008,-17.9553268138185,-17.9025498101062,-17.8785124860334,
-17.8585641498629,-17.8289638313947,-17.7260579793596,-17.6021830902463,
-17.5187317541391,-17.4533736063989,-17.4134241267227,-17.3755966089807,
-17.3204559828818,-17.128328726292,-17.034751643352,-16.9779117914376,-16.95325250703,
-16.933414999532,-16.9048415322082,-16.8163979931498,-16.6451222197646,
-16.5976796631281,-16.5293988090945,-16.4889355510299,-16.4509419474887,
-16.3971896204609,-16.1482849279925,-16.0876403506079,-16.0446502676035,
-16.0222933193482,-16.001722798788,-15.9681072300132,-15.9252723255546,
-15.8194108553877,-15.7788843401984,-15.6343652298015,-15.5889389460784,
-15.5512756036654,-15.5110125094001,-15.4438736671729,-15.3976144736802,
-15.2350904277882,-15.1362980871434,-15.1069714197455,-15.0870551794142,
-15.0628619666166,-15.0090939145782,-14.9236887794412,-14.7117078992256,
-14.6648931206517,-14.6269319683612,-14.587204069174,-14.5231055020978,
-14.4799193883562,-14.3374321834459,-14.320088167473,-14.2192161202029,
-14.1852686149023,-14.1666632176757,-14.1452066779954,-14.1069411468773,
-14.055632052595,-13.9012291566851,-13.8033983278317,-13.7431414538368,
-13.7079773708991,-13.6697247418832,-13.6142897791556,-13.4062335559749,
-13.3797718028052,-13.2834220783063,-13.2541494193847,-13.2342393781621,
-13.2100147758301,-13.1560446141659,-13.0701192042578,-12.8595611044772,
-12.8073623837127,-12.7695912504969,-12.7285822922506,-12.6571665694385,
-12.4489214808299,-12.3561288309886,-12.3272611370388,-12.3073947818981,
-12.2829247002842,-12.227351545166,-12.0267256243128,-11.9192684382317,
-11.8724689891664,-11.8352443755935,-11.7912636631108,-11.7012933700652,
-11.6675653273102),.UNSPECIFIED.) ;
#302=B_SPLINE_CURVE_WITH_KNOTS('',3,(#46026,#46027,#46028,#46029,#46030,
#46031,#46032,#46033,#46034,#46035,#46036,#46037,#46038,#46039,#46040,#46041,
#46042,#46043,#46044,#46045,#46046,#46047,#46048,#46049,#46050,#46051,#46052,
#46053,#46054,#46055,#46056,#46057,#46058,#46059,#46060,#46061,#46062,#46063,
#46064,#46065,#46066,#46067,#46068,#46069,#46070,#46071,#46072,#46073,#46074,
#46075,#46076,#46077,#46078,#46079,#46080,#46081,#46082,#46083,#46084,#46085,
#46086,#46087,#46088,#46089,#46090,#46091,#46092,#46093,#46094,#46095,#46096,
#46097,#46098,#46099,#46100,#46101,#46102,#46103,#46104,#46105,#46106,#46107,
#46108,#46109,#46110,#46111,#46112,#46113,#46114,#46115,#46116,#46117,#46118,
#46119,#46120,#46121,#46122,#46123,#46124,#46125,#46126,#46127,#46128,#46129,
#46130,#46131,#46132,#46133,#46134,#46135,#46136,#46137,#46138,#46139,#46140,
#46141,#46142,#46143,#46144,#46145,#46146,#46147,#46148,#46149,#46150,#46151,
#46152,#46153,#46154,#46155,#46156,#46157,#46158,#46159,#46160,#46161,#46162,
#46163,#46164,#46165,#46166,#46167,#46168,#46169,#46170,#46171,#46172,#46173,
#46174,#46175,#46176,#46177,#46178,#46179,#46180,#46181,#46182,#46183,#46184,
#46185,#46186,#46187,#46188,#46189,#46190,#46191,#46192,#46193,#46194,#46195,
#46196,#46197,#46198,#46199,#46200,#46201,#46202,#46203,#46204,#46205,#46206,
#46207,#46208,#46209,#46210,#46211,#46212,#46213,#46214,#46215,#46216,#46217,
#46218,#46219,#46220,#46221,#46222,#46223,#46224,#46225,#46226,#46227,#46228,
#46229,#46230,#46231,#46232,#46233,#46234,#46235,#46236,#46237,#46238,#46239,
#46240,#46241,#46242,#46243,#46244,#46245,#46246,#46247,#46248,#46249,#46250,
#46251,#46252,#46253,#46254,#46255,#46256,#46257,#46258,#46259,#46260,#46261,
#46262,#46263,#46264,#46265,#46266,#46267,#46268,#46269,#46270,#46271,#46272,
#46273,#46274,#46275,#46276,#46277,#46278,#46279,#46280,#46281,#46282,#46283,
#46284,#46285,#46286,#46287,#46288,#46289,#46290,#46291,#46292,#46293,#46294,
#46295,#46296,#46297,#46298,#46299,#46300,#46301,#46302,#46303,#46304,#46305,
#46306,#46307,#46308,#46309,#46310,#46311,#46312,#46313,#46314,#46315,#46316,
#46317,#46318,#46319,#46320,#46321,#46322,#46323,#46324,#46325,#46326,#46327,
#46328,#46329,#46330,#46331,#46332,#46333,#46334,#46335,#46336,#46337,#46338,
#46339,#46340,#46341,#46342,#46343,#46344,#46345,#46346,#46347,#46348,#46349,
#46350,#46351,#46352,#46353,#46354,#46355,#46356,#46357,#46358,#46359,#46360,
#46361),.UNSPECIFIED.,.F.,.F.,(4,2,2,2,2,2,2,2,2,2,2,2,2,2,2,2,2,2,2,2,
2,2,2,2,2,2,2,2,2,2,2,2,2,2,2,2,2,2,2,2,2,2,2,2,2,2,2,2,2,2,2,2,2,2,2,2,
2,2,2,2,2,2,2,2,2,2,2,2,2,2,2,2,2,2,2,2,2,2,2,2,2,2,2,2,2,2,2,2,2,2,2,2,
2,2,2,2,2,2,2,2,2,2,2,2,2,2,2,2,2,2,2,2,2,2,2,2,2,2,2,2,2,2,2,2,2,2,2,2,
2,2,2,2,2,2,2,2,2,2,2,2,2,2,2,2,2,2,2,2,2,2,2,2,2,2,2,2,2,2,2,2,2,2,2,2,
2,2,2,4),(-23.3355609284769,-23.2597287932774,-23.222225214567,-23.1167937467186,
-23.0349671579936,-22.970471448011,-22.9306716603284,-22.8927506184788,
-22.8461267646939,-22.6328417921701,-22.5479273841423,-22.4943501547635,
-22.4701863473356,-22.4502652883526,-22.4208902220894,-22.324326615371,
-22.295965597956,-22.190758663422,-22.1087525408583,-22.0441626782366,-22.0043511077128,
-21.9664486753242,-21.9108091228529,-21.7661909080502,-21.6148359855681,
-21.5658384152302,-21.542420742005,-21.5223090739911,-21.4966619460148,
-21.4093946091982,-21.3656175211198,-21.2241436401028,-21.1341396575724,
-21.0901521948904,-21.0529251825028,-21.0061266185742,-20.900500509744,
-20.6979596889977,-20.6424521270335,-20.6179906439059,-20.5981217166481,
-20.569235622051,-20.4762894630837,-20.3088312370607,-20.2406290264233,
-20.1837707184177,-20.1452890794756,-20.1056772895833,-20.0422349775556,
-19.9524022454156,-19.7965777892175,-19.7450676412924,-19.7066963236677,
-19.6852196704393,-19.666627582009,-19.6327603484839,-19.5625011539637,
-19.3857148475227,-19.3375731352389,-19.268624464095,-19.2280438247443,
-19.1901019842602,-19.1451490323796,-18.9224525442309,-18.8406516377513,
-18.7883096075161,-18.7643409489732,-18.7443765958703,-18.7146490032512,
-18.6091820724899,-18.4028767473322,-18.3384652674937,-18.2986821920745,
-18.2607554267598,-18.2140966586248,-18.0010833329753,-17.9160690783646,
-17.8624534034883,-17.8382839374336,-17.8183629236402,-17.7889951995181,
-17.692386261373,-17.6640648724364,-17.5588847300649,-17.4768551992637,
-17.4122512188597,-17.3724340540874,-17.3345277451068,-17.2788842798252,
-17.1344789791574,-16.9830255971562,-16.9339633145125,-16.9105329295557,
-16.8904236533959,-16.8647911132839,-16.7799269527606,-16.6056779782297,
-16.557853550413,-16.4892070546307,-16.4486792379562,-16.4107139895469,
-16.3656463550079,-16.2304299890274,-16.0873796485533,-16.0377588955467,
-16.0003912625658,-15.9791109182628,-15.9603882297376,-15.9257413546584,
-15.8150473175076,-15.6683381522635,-15.5766415197884,-15.5324117847278,
-15.4952004255303,-15.448709384268,-15.3687398273464,-15.1734945703925,
-15.091969191924,-15.064378514863,-15.0464838897029,-15.0222268448732,-14.9680489709915,
-14.9374316069859,-14.7666760261359,-14.6585565290365,-14.6115564470379,
-14.5743207148758,-14.5304932832417,-14.4415745340718,-14.3033318174456,
-14.2657208310757,-14.1693589954677,-14.1400849184509,-14.1201745068449,
-14.0959502124043,-14.0419832792392,-13.9560668426929,-13.7454784744436,
-13.6932842652118,-13.6555133797642,-13.6145019552021,-13.5430739617164,
-13.3338533275426,-13.2418465028581,-13.2130717535092,-13.1932145700271,
-13.1686851991473,-13.1127194909873,-13.02152844155,-12.821763904206,-12.7684100370052,
-12.7304748610735,-12.6898799021145,-12.6208483030156,-12.5726191450503,
-12.3951246716236,-12.3314273615835,-12.2944906744239,-12.2753705715818,
-12.2545542479143,-12.2195978170628,-12.1022591009582,-11.8934143193826,
-11.8408999442353,-11.8030847950654,-11.7621939182167,-11.6914624396032,
-11.667685703203),.UNSPECIFIED.) ;
#303=B_SPLINE_CURVE_WITH_KNOTS('',3,(#46362,#46363,#46364,#46365,#46366,
#46367,#46368,#46369,#46370,#46371,#46372,#46373,#46374,#46375,#46376,#46377,
#46378,#46379,#46380,#46381,#46382,#46383,#46384,#46385,#46386,#46387,#46388,
#46389,#46390,#46391,#46392,#46393,#46394,#46395,#46396,#46397,#46398,#46399,
#46400,#46401,#46402,#46403,#46404,#46405,#46406,#46407,#46408,#46409,#46410,
#46411,#46412,#46413,#46414,#46415,#46416,#46417,#46418,#46419,#46420,#46421,
#46422,#46423,#46424,#46425,#46426,#46427,#46428,#46429,#46430,#46431,#46432,
#46433,#46434,#46435,#46436,#46437,#46438,#46439,#46440,#46441,#46442,#46443,
#46444,#46445,#46446,#46447,#46448,#46449,#46450,#46451,#46452,#46453,#46454,
#46455,#46456,#46457,#46458,#46459,#46460,#46461,#46462,#46463,#46464,#46465,
#46466,#46467,#46468,#46469,#46470,#46471,#46472,#46473,#46474,#46475,#46476,
#46477,#46478,#46479,#46480,#46481,#46482,#46483,#46484,#46485,#46486,#46487,
#46488,#46489,#46490,#46491,#46492,#46493,#46494,#46495,#46496,#46497,#46498,
#46499,#46500,#46501,#46502,#46503,#46504,#46505,#46506,#46507,#46508,#46509,
#46510,#46511,#46512,#46513,#46514,#46515,#46516,#46517,#46518,#46519,#46520,
#46521,#46522,#46523,#46524,#46525,#46526,#46527,#46528,#46529,#46530,#46531,
#46532,#46533,#46534,#46535,#46536,#46537,#46538,#46539,#46540,#46541,#46542,
#46543,#46544,#46545,#46546,#46547,#46548,#46549,#46550,#46551,#46552,#46553,
#46554,#46555,#46556,#46557,#46558,#46559,#46560,#46561,#46562,#46563,#46564,
#46565,#46566,#46567,#46568,#46569,#46570,#46571,#46572,#46573,#46574,#46575,
#46576,#46577,#46578,#46579,#46580,#46581,#46582,#46583,#46584,#46585,#46586,
#46587,#46588,#46589,#46590,#46591,#46592,#46593,#46594,#46595,#46596,#46597,
#46598,#46599,#46600,#46601,#46602,#46603,#46604,#46605,#46606,#46607,#46608,
#46609,#46610,#46611,#46612,#46613,#46614,#46615,#46616,#46617,#46618,#46619,
#46620,#46621,#46622,#46623,#46624,#46625,#46626,#46627,#46628,#46629,#46630,
#46631,#46632,#46633,#46634,#46635,#46636,#46637,#46638,#46639,#46640,#46641,
#46642,#46643,#46644,#46645,#46646,#46647,#46648,#46649,#46650,#46651,#46652,
#46653,#46654,#46655,#46656,#46657,#46658,#46659,#46660,#46661,#46662,#46663,
#46664,#46665,#46666,#46667,#46668,#46669,#46670,#46671,#46672,#46673,#46674,
#46675,#46676,#46677,#46678,#46679,#46680,#46681,#46682,#46683,#46684,#46685,
#46686,#46687,#46688,#46689,#46690,#46691,#46692,#46693,#46694,#46695,#46696,
#46697,#46698,#46699,#46700,#46701,#46702,#46703,#46704,#46705),
 .UNSPECIFIED.,.F.,.F.,(4,2,2,2,2,2,2,2,2,2,2,2,2,2,2,2,2,2,2,2,2,2,2,2,
2,2,2,2,2,2,2,2,2,2,2,2,2,2,2,2,2,2,2,2,2,2,2,2,2,2,2,2,2,2,2,2,2,2,2,2,
2,2,2,2,2,2,2,2,2,2,2,2,2,2,2,2,2,2,2,2,2,2,2,2,2,2,2,2,2,2,2,2,2,2,2,2,
2,2,2,2,2,2,2,2,2,2,2,2,2,2,2,2,2,2,2,2,2,2,2,2,2,2,2,2,2,2,2,2,2,2,2,2,
2,2,2,2,2,2,2,2,2,2,2,2,2,2,2,2,2,2,2,2,2,2,2,2,2,2,2,2,2,2,2,2,2,2,2,2,
2,2,2,4),(-11.6675653273102,-11.5599168418434,-11.5138978859093,-11.4286591377124,
-11.4030401139979,-11.3829338798932,-11.3594956788994,-11.3103851182522,
-11.158858251161,-11.0146362717321,-10.9589821415689,-10.9210747439862,
-10.88126140232,-10.8166759692942,-10.7346802388235,-10.6294574700789,-10.6010083746183,
-10.5044076668633,-10.4750857885122,-10.4551703247593,-10.4309748975263,
-10.3771912316371,-10.2917452730081,-10.0798798522952,-10.033047849607,
-9.99508325386252,-9.95536212172787,-9.89129978676861,-9.77864771153884,
-9.58591803710041,-9.55270602054035,-9.53422075328706,-9.51256083029925,
-9.47325028766468,-9.41994299387689,-9.25057680579537,-9.14160855047381,
-9.09430226539542,-9.05704949204078,-9.01345156463859,-8.92607244779549,
-8.79226385861574,-8.76997211879241,-8.7398532298263,-8.65004988525598,
-8.62147046078619,-8.60163258060766,-8.57697768547286,-8.52016631170477,
-8.42666703187411,-8.23465175162409,-8.17941132443611,-8.1415686792487,
-8.10164678549299,-8.03644362733608,-7.99361729264837,-7.84751934126576,
-7.8132801927561,-7.72368356416008,-7.69511152101925,-7.67527438556438,
-7.65061475848494,-7.59377101735208,-7.50018232480575,-7.30804148474877,
-7.25291997497611,-7.21509581752658,-7.17514188290794,-7.10975626871894,
-7.02625217938331,-6.90237607585637,-6.79966350634897,-6.77002270784409,
-6.7500696742293,-6.72605531614973,-6.6734216888468,-6.59089159087684,-6.37281143620365,
-6.32659770885665,-6.28876881795864,-6.2488237484525,-6.18348767917299,
-6.10007723808647,-5.9762037781576,-5.87317433023502,-5.84359489475306,
-5.82364939269744,-5.79960120016814,-5.74675369433131,-5.66368658126237,
-5.44660058565869,-5.40033301199408,-5.36249261974491,-5.3225681743427,
-5.25734844163975,-5.05044538559886,-4.94670944706507,-4.91716409227892,
-4.89722272587147,-4.87315557143905,-4.82018792259332,-4.73681806161008,
-4.66686438021753,-4.63281709456112,-4.55575940012506,-4.48698750433858,
-4.44643899776407,-4.40848544550055,-4.35499874965015,-4.29244025956197,
-4.15501239002384,-4.02572471520113,-3.9935906114256,-3.97347515068028,
-3.95069921434655,-3.90540206240404,-3.87067828988611,-3.73331562450593,
-3.59170345279729,-3.54625997369065,-3.5085940574052,-3.46834032614663,
-3.40124916719926,-3.3550382379002,-3.19285128415213,-3.09364913210538,
-3.06430162556963,-3.0443835577571,-3.02020382675209,-2.96651880486555,
-2.88132485994284,-2.66880115808774,-2.62207346237968,-2.58413253698623,
-2.54437601617899,-2.48010929894564,-2.37234582510119,-2.18914481939562,
-2.14803908722876,-2.12603539898619,-2.10524481282176,-2.07042276007788,
-1.94444877599146,-1.74586073057188,-1.69255191172432,-1.65462457524464,
-1.61401689884784,-1.54490566428976,-1.45415188442675,-1.24868373760917,
-1.2155060805417,-1.19702656937367,-1.18210690130692,-1.18162985498578,
-1.1811982453945,-1.1523101414957,-1.11465893813669,-1.03103382139579,-0.816009129807846,
-0.769297196591649,-0.731359689374574,-0.695161004090526,-0.665273959345048,
-0.612753371120607,-0.515190768148353,-0.322330617910769,-0.289141854711983,
-0.270660559861515,-0.252517933370279,-0.23040098625164,-0.196185058895016,
-1.00000001085343E-6),.UNSPECIFIED.) ;
#304=B_SPLINE_CURVE_WITH_KNOTS('',3,(#46708,#46709,#46710,#46711,#46712,
#46713,#46714,#46715,#46716,#46717,#46718,#46719,#46720,#46721,#46722,#46723,
#46724,#46725,#46726,#46727,#46728,#46729,#46730,#46731,#46732,#46733,#46734,
#46735,#46736,#46737,#46738,#46739,#46740,#46741,#46742,#46743,#46744,#46745,
#46746,#46747,#46748,#46749,#46750,#46751,#46752,#46753,#46754,#46755,#46756,
#46757,#46758,#46759,#46760,#46761,#46762,#46763,#46764,#46765,#46766,#46767,
#46768,#46769,#46770,#46771,#46772,#46773,#46774,#46775,#46776,#46777,#46778,
#46779,#46780,#46781,#46782,#46783,#46784,#46785,#46786,#46787,#46788,#46789,
#46790,#46791,#46792,#46793,#46794,#46795,#46796,#46797,#46798,#46799,#46800,
#46801,#46802,#46803,#46804,#46805,#46806,#46807,#46808,#46809,#46810,#46811,
#46812,#46813,#46814,#46815,#46816,#46817,#46818,#46819,#46820,#46821,#46822,
#46823,#46824,#46825,#46826,#46827,#46828,#46829,#46830,#46831,#46832,#46833,
#46834,#46835,#46836,#46837,#46838,#46839,#46840,#46841,#46842,#46843,#46844,
#46845,#46846,#46847,#46848,#46849,#46850,#46851,#46852,#46853,#46854,#46855,
#46856,#46857,#46858,#46859,#46860,#46861,#46862,#46863,#46864,#46865,#46866,
#46867,#46868,#46869,#46870,#46871,#46872,#46873,#46874,#46875,#46876,#46877,
#46878,#46879,#46880,#46881,#46882,#46883,#46884,#46885,#46886,#46887,#46888,
#46889,#46890,#46891,#46892,#46893,#46894,#46895,#46896,#46897,#46898,#46899,
#46900,#46901,#46902,#46903,#46904,#46905,#46906,#46907,#46908,#46909,#46910,
#46911,#46912,#46913,#46914,#46915,#46916,#46917,#46918,#46919,#46920,#46921,
#46922,#46923,#46924,#46925,#46926,#46927,#46928,#46929,#46930,#46931,#46932,
#46933,#46934,#46935,#46936,#46937,#46938,#46939,#46940,#46941,#46942,#46943,
#46944,#46945,#46946,#46947,#46948,#46949,#46950,#46951,#46952,#46953,#46954,
#46955,#46956,#46957,#46958,#46959,#46960,#46961,#46962,#46963,#46964,#46965,
#46966,#46967,#46968,#46969,#46970,#46971,#46972,#46973,#46974,#46975,#46976,
#46977,#46978,#46979,#46980,#46981,#46982,#46983,#46984,#46985,#46986,#46987,
#46988,#46989,#46990,#46991,#46992,#46993,#46994,#46995,#46996,#46997,#46998,
#46999,#47000,#47001,#47002,#47003,#47004,#47005,#47006,#47007,#47008,#47009,
#47010,#47011,#47012,#47013,#47014,#47015,#47016,#47017,#47018,#47019,#47020,
#47021,#47022,#47023,#47024,#47025,#47026,#47027,#47028,#47029,#47030,#47031,
#47032,#47033,#47034,#47035,#47036,#47037,#47038,#47039,#47040,#47041,#47042,
#47043,#47044,#47045,#47046,#47047),.UNSPECIFIED.,.F.,.F.,(4,2,2,2,2,2,
2,2,2,2,2,2,2,2,2,2,2,2,2,2,2,2,2,2,2,2,2,2,2,2,2,2,2,2,2,2,2,2,2,2,2,2,
2,2,2,2,2,2,2,2,2,2,2,2,2,2,2,2,2,2,2,2,2,2,2,2,2,2,2,2,2,2,2,2,2,2,2,2,
2,2,2,2,2,2,2,2,2,2,2,2,2,2,2,2,2,2,2,2,2,2,2,2,2,2,2,2,2,2,2,2,2,2,2,2,
2,2,2,2,2,2,2,2,2,2,2,2,2,2,2,2,2,2,2,2,2,2,2,2,2,2,2,2,2,2,2,2,2,2,2,2,
2,2,2,2,2,2,2,2,2,2,2,2,2,2,2,2,2,2,2,4),(-8.83672325566634,-8.72339974280114,
-8.68386166002427,-8.64898714110386,-8.61113228183851,-8.55580942003574,
-8.41502260358477,-8.24221691069678,-8.2075784098526,-8.18873874032175,
-8.16887711629528,-8.14004990527668,-8.04759292469131,-8.02017856555552,
-7.87175350041695,-7.80695344124842,-7.75554249950216,-7.72279298257082,
-7.68495941869026,-7.63872276554454,-7.39884911134843,-7.32969916943655,
-7.29598074784733,-7.2955179103999,-7.29510143853705,-7.29472630908798,
-7.29438810083793,-7.29408291437532,-7.293807303533,-7.2935582167102,-7.29277562897946,
-7.29202378623707,-7.29130089086543,-7.29060525972034,-7.28993531600412,
-7.28928958179882,-7.2886666710752,-7.28806528324593,-7.28748419720352,
-7.28692226574861,-7.28637841042325,-7.28585161673894,-7.28534092970952,
-7.28484544971679,-7.28436432868456,-7.28389676647281,-7.28344200755974,
-7.28299933792181,-7.28256808213522,-7.28214760070153,-7.28173728752033,
-7.28133656751879,-7.25871267664155,-7.2385286762415,-7.20597878339026,
-7.13277680018572,-6.95631015395828,-6.90820931273134,-6.83930044602996,
-6.7987276617651,-6.76078407611064,-6.7158182518756,-6.57685725872102,-6.56230945149741,
-6.43287466606539,-6.36484382465875,-6.33868687537384,-6.3209106907098,
-6.29554250608781,-6.24019703235213,-6.15517165334181,-6.01508567695931,
-5.92554561400664,-5.88162904051464,-5.84440243176646,-5.79752642833198,
-5.69330620821936,-5.48953004821778,-5.43405628175592,-5.40960168586134,
-5.38973203905418,-5.36083768558537,-5.26782049869653,-5.10044717430939,
-5.03225969114084,-4.9754096148371,-4.93692739785334,-4.90201110844253,
-4.84336205128404,-4.74133357887729,-4.58766642049797,-4.5364620580424,
-4.49825191469023,-4.47680613613605,-4.45556687016721,-4.41839852922431,
-4.27942759244415,-4.10338407788865,-4.0476993631982,-4.00979041154072,
-3.96999151060022,-3.90547052297783,-3.82359252103421,-3.71821960242769,
-3.60344920293334,-3.56894117433974,-3.55024320585233,-3.5289305704546,
-3.49139794606272,-3.44146906294306,-3.29642535072114,-3.18159511238375,
-3.12376680441117,-3.08897503512535,-3.0503597725156,-2.9927092509224,-2.92315179708276,
-2.74707523567595,-2.6700207679134,-2.63913558248495,-2.61920824042201,
-2.59590213134742,-2.54759846309893,-2.5093829502471,-2.34293671861362,
-2.23190743042217,-2.1841018291998,-2.14681130373033,-2.10355330181405,
-2.01843491008466,-1.89086859611604,-1.88015634021239,-1.8415520780261,
-1.74116925266082,-1.71156202771834,-1.6916255070351,-1.66764616256745,
-1.61510573303749,-1.53280351586751,-1.31373289219991,-1.26755185166437,
-1.22975151575445,-1.19703210946525,-1.1456923152463,-1.08096298290102,
-0.932797394368955,-0.815064462429085,-0.785120838675239,-0.765424231108012,
-0.750109886792035,-0.749330846664115,-0.748554575935521,-0.747758918081246,
-0.746921327833159,-0.746016452447542,-0.745013409506678,-0.743872194103966,
-0.742538455551737,-0.740935468372936,-0.738951391871269,-0.736418772801353,
-0.733081877396021,-0.701181541314413,-0.638260302490662,-0.386295812752923,
-0.340986276786363,-0.302905898673403,-0.267984339448119,-0.227731199758877,
-1.96846129342848E-5),.UNSPECIFIED.) ;
#305=B_SPLINE_CURVE_WITH_KNOTS('',3,(#47050,#47051,#47052,#47053,#47054,
#47055,#47056,#47057,#47058,#47059,#47060,#47061,#47062,#47063,#47064,#47065,
#47066,#47067,#47068,#47069,#47070,#47071,#47072,#47073,#47074,#47075,#47076,
#47077,#47078,#47079,#47080,#47081,#47082,#47083,#47084,#47085,#47086,#47087,
#47088,#47089,#47090,#47091,#47092,#47093,#47094,#47095,#47096,#47097,#47098,
#47099,#47100,#47101,#47102,#47103,#47104,#47105,#47106,#47107,#47108,#47109,
#47110,#47111,#47112,#47113,#47114,#47115,#47116,#47117,#47118,#47119,#47120,
#47121,#47122,#47123,#47124,#47125,#47126,#47127,#47128,#47129,#47130,#47131,
#47132,#47133,#47134,#47135,#47136,#47137,#47138,#47139,#47140,#47141,#47142,
#47143,#47144,#47145,#47146,#47147,#47148,#47149,#47150,#47151,#47152,#47153,
#47154,#47155,#47156,#47157,#47158,#47159,#47160,#47161,#47162,#47163,#47164,
#47165,#47166,#47167,#47168,#47169,#47170,#47171,#47172,#47173,#47174,#47175,
#47176,#47177,#47178,#47179,#47180,#47181,#47182,#47183,#47184,#47185,#47186,
#47187,#47188,#47189,#47190,#47191,#47192,#47193,#47194,#47195,#47196,#47197,
#47198,#47199,#47200,#47201,#47202,#47203,#47204,#47205,#47206,#47207,#47208,
#47209,#47210,#47211,#47212,#47213,#47214,#47215,#47216,#47217,#47218,#47219,
#47220,#47221,#47222,#47223,#47224,#47225,#47226,#47227,#47228,#47229,#47230,
#47231,#47232,#47233,#47234,#47235,#47236,#47237,#47238,#47239,#47240,#47241,
#47242,#47243,#47244,#47245,#47246,#47247,#47248,#47249,#47250,#47251),
 .UNSPECIFIED.,.F.,.F.,(4,2,2,2,2,2,2,2,2,2,2,2,2,2,2,2,2,2,2,2,2,2,2,2,
2,2,2,2,2,2,2,2,2,2,2,2,2,2,2,2,2,2,2,2,2,2,2,2,2,2,2,2,2,2,2,2,2,2,2,2,
2,2,2,2,2,2,2,2,2,2,2,2,2,2,2,2,2,2,2,2,2,2,2,2,2,2,2,2,2,2,2,2,2,2,2,2,
2,2,2,2,4),(-29.8748049370787,-29.8559623263054,-29.8310093407934,-29.6893565955101,
-29.5245377048083,-29.4841327566667,-29.4484770034037,-29.4099263933365,
-29.3532477761587,-29.1334555528409,-29.0344403123814,-28.9931722782713,
-28.9806683328654,-28.9750709988028,-28.9701189579125,-28.9663087516873,
-28.9638773537707,-28.9624017958589,-28.9446163187811,-28.9239575025797,
-28.8902752588268,-28.7426392944441,-28.622747079501,-28.5644150487242,
-28.5247241046179,-28.4897947109261,-28.4519297175056,-28.4056792359559,
-28.1853058710086,-28.1031483881522,-28.0507279668659,-28.0268697609116,
-28.0068883743685,-27.9771754794791,-27.8770101891862,-27.716092888132,
-27.6488512352504,-27.5924426658416,-27.5537667007694,-27.5135072819418,
-27.447781589121,-27.3257844177079,-27.174462736726,-27.1251475022996,-27.1015241115852,
-27.0813434574031,-27.0555673010956,-26.965667719789,-26.7956413031322,
-26.7484167986561,-26.6804349480034,-26.6401647951043,-26.6023882827539,
-26.5575180680391,-26.3319888718872,-26.2506379027527,-26.1985035135455,
-26.1746709129656,-26.154771559656,-26.1252144797171,-26.0217843114692,
-25.8978541335425,-25.8144945360647,-25.749142711359,-25.709129919641,-25.6711894328127,
-25.6157535961383,-25.4236732396369,-25.3312904716796,-25.274881413357,
-25.2502336066244,-25.2303427726501,-25.2015490711106,-25.109484335517,
-24.9413172978235,-24.8730218149808,-24.8161221980946,-24.7776560442992,
-24.7427880945695,-24.6843187969317,-24.5809851745903,-24.4276278117773,
-24.3764628207489,-24.3382797304737,-24.3168593827777,-24.2982644115716,
-24.2643468836702,-24.1640124207224,-24.0091390279228,-23.9639888264052,
-23.8979316861805,-23.8578560675221,-23.820091020739,-23.7653775833646,
-23.5729497659355,-23.4790726889548,-23.4221257040589,-23.3974458025519,
-23.3776043580981,-23.3490370914111,-23.3355609284769),.UNSPECIFIED.) ;
#306=B_SPLINE_CURVE_WITH_KNOTS('',3,(#47254,#47255,#47256,#47257,#47258,
#47259,#47260,#47261,#47262,#47263,#47264,#47265,#47266,#47267,#47268,#47269,
#47270,#47271,#47272,#47273,#47274,#47275,#47276,#47277,#47278,#47279,#47280,
#47281,#47282,#47283,#47284,#47285,#47286,#47287,#47288,#47289,#47290,#47291,
#47292,#47293,#47294,#47295,#47296,#47297,#47298,#47299,#47300,#47301,#47302,
#47303,#47304,#47305,#47306,#47307,#47308,#47309,#47310,#47311,#47312,#47313,
#47314,#47315,#47316,#47317,#47318,#47319,#47320,#47321,#47322,#47323,#47324,
#47325,#47326,#47327,#47328,#47329,#47330,#47331,#47332,#47333,#47334,#47335,
#47336,#47337,#47338,#47339,#47340,#47341,#47342,#47343,#47344,#47345,#47346,
#47347,#47348,#47349,#47350,#47351,#47352,#47353,#47354,#47355,#47356,#47357,
#47358,#47359,#47360,#47361,#47362,#47363,#47364,#47365),.UNSPECIFIED.,
 .F.,.F.,(4,2,2,2,2,2,2,2,2,2,2,2,2,2,2,2,2,2,2,2,2,2,2,2,2,2,2,2,2,2,2,
2,2,2,2,2,2,2,2,2,2,2,2,2,2,2,2,2,2,2,2,2,2,2,2,4),(-10.5425049368748,-10.4813665573713,
-10.3082210802619,-10.0952472441292,-9.95794965199355,-9.84959651696192,
-9.68102697606107,-9.47105758716311,-9.29704804786971,-9.08058762674709,
-8.94801017752495,-8.83790843595371,-8.66281179722811,-8.44979106049249,
-8.26875026576761,-8.02350533146686,-7.91386747822455,-7.72464433932807,
-7.45273652713729,-7.27799612001064,-7.05859100547209,-6.92228575466226,
-6.79872465568987,-6.4206733771102,-6.2299195775176,-5.99481772115077,-5.89085098224896,
-5.70306580415755,-5.43654325973892,-5.26211479592577,-5.04399855157591,
-4.90583377233716,-4.78312363312272,-4.40082965711161,-4.20706485434783,
-3.96876887000412,-3.86847375874845,-3.69017410085091,-3.41895959388069,
-3.24427481755454,-3.02508335598879,-2.8884582034516,-2.76461624729456,
-2.3882303819844,-2.19831894215256,-1.96368955992695,-1.85875788984718,
-1.66529088291307,-1.403256505249,-1.22966469894533,-1.01422844467065,-0.880428165090804,
-0.769524651617117,-0.411353224294561,-0.250713762539928,-2.85710713469914E-5),
 .UNSPECIFIED.) ;
#307=B_SPLINE_CURVE_WITH_KNOTS('',3,(#47368,#47369,#47370,#47371,#47372,
#47373,#47374,#47375,#47376,#47377,#47378,#47379,#47380,#47381,#47382,#47383,
#47384,#47385,#47386,#47387,#47388,#47389,#47390,#47391,#47392,#47393,#47394,
#47395,#47396,#47397,#47398,#47399,#47400,#47401,#47402,#47403,#47404,#47405,
#47406,#47407,#47408,#47409,#47410,#47411,#47412,#47413,#47414,#47415,#47416,
#47417,#47418,#47419,#47420,#47421,#47422,#47423,#47424,#47425,#47426,#47427,
#47428,#47429,#47430,#47431,#47432,#47433,#47434,#47435,#47436,#47437,#47438,
#47439,#47440,#47441,#47442,#47443,#47444,#47445,#47446,#47447,#47448,#47449,
#47450,#47451,#47452,#47453,#47454,#47455,#47456,#47457),.UNSPECIFIED.,
 .F.,.F.,(4,2,2,2,2,2,2,2,2,2,2,2,2,2,2,2,2,2,2,2,2,2,2,2,2,2,2,2,2,2,2,
2,2,2,2,2,2,2,2,2,2,2,2,2,4),(-80.5199172564641,-80.1644944208614,-80.0041939643627,
-79.6847223829998,-79.5240762293956,-79.4233443519087,-79.1836115690117,
-78.9943596077749,-78.65284703493,-78.5470907958417,-78.4516464435982,-78.2020394547879,
-77.9993526461617,-77.8038656449858,-77.6033858547518,-77.4865313444434,
-77.3320976775467,-77.1260689513558,-76.9553817713464,-76.6803092179975,
-76.49669658309,-76.385784272223,-76.150948460969,-75.9660559062757,-75.753224074914,
-75.575790872784,-75.4649445913754,-75.3309730714214,-75.1156319162072,
-74.9420481818352,-74.7355520721864,-74.5645322172805,-74.4555737217011,
-74.3216560757955,-74.1061821600071,-73.9323706298221,-73.7296741777522,
-73.5568647574461,-73.4473510989502,-73.3126234791358,-73.0977447422244,
-72.9241171079032,-72.7216571734284,-72.548688145428,-72.5408068653678),
 .UNSPECIFIED.) ;
#308=B_SPLINE_CURVE_WITH_KNOTS('',3,(#47460,#47461,#47462,#47463,#47464,
#47465,#47466,#47467,#47468,#47469,#47470,#47471,#47472,#47473,#47474,#47475,
#47476,#47477,#47478,#47479,#47480,#47481,#47482,#47483,#47484,#47485,#47486,
#47487,#47488,#47489,#47490,#47491,#47492,#47493,#47494,#47495,#47496,#47497,
#47498,#47499),.UNSPECIFIED.,.F.,.F.,(4,3,3,3,3,3,3,3,3,3,3,3,3,4),(38.8091570539889,
38.8694027977159,38.9296461683401,38.989896014336,39.0501473311069,39.1104107652207,
39.1514960580706,39.2116081997616,39.27171086176,39.3318070729702,39.3936353160341,
39.4537320202377,39.5164260327317,39.5791200452257),.UNSPECIFIED.) ;
#309=B_SPLINE_CURVE_WITH_KNOTS('',3,(#47503,#47504,#47505,#47506,#47507,
#47508,#47509,#47510,#47511,#47512,#47513,#47514,#47515,#47516,#47517,#47518,
#47519,#47520,#47521,#47522,#47523,#47524,#47525,#47526,#47527,#47528,#47529,
#47530,#47531,#47532,#47533,#47534,#47535,#47536,#47537,#47538,#47539,#47540,
#47541,#47542,#47543,#47544,#47545,#47546,#47547,#47548,#47549,#47550,#47551,
#47552,#47553,#47554,#47555,#47556,#47557,#47558,#47559,#47560,#47561,#47562,
#47563,#47564,#47565,#47566,#47567,#47568,#47569,#47570,#47571,#47572,#47573,
#47574,#47575,#47576,#47577,#47578,#47579,#47580,#47581,#47582,#47583,#47584,
#47585,#47586,#47587,#47588,#47589,#47590,#47591,#47592,#47593,#47594,#47595,
#47596,#47597,#47598,#47599,#47600,#47601,#47602,#47603,#47604,#47605,#47606,
#47607,#47608,#47609,#47610,#47611,#47612,#47613,#47614,#47615,#47616,#47617,
#47618,#47619,#47620,#47621,#47622,#47623,#47624,#47625,#47626,#47627,#47628,
#47629,#47630,#47631,#47632,#47633,#47634,#47635,#47636,#47637,#47638,#47639,
#47640,#47641,#47642,#47643,#47644,#47645,#47646,#47647,#47648,#47649,#47650,
#47651,#47652,#47653,#47654,#47655,#47656,#47657,#47658,#47659,#47660,#47661,
#47662,#47663,#47664,#47665,#47666,#47667,#47668,#47669,#47670,#47671,#47672,
#47673,#47674,#47675,#47676,#47677,#47678,#47679,#47680,#47681,#47682,#47683,
#47684,#47685,#47686,#47687,#47688,#47689,#47690,#47691,#47692,#47693,#47694,
#47695,#47696,#47697,#47698,#47699,#47700,#47701,#47702,#47703,#47704,#47705,
#47706,#47707,#47708,#47709,#47710,#47711,#47712,#47713,#47714,#47715,#47716,
#47717,#47718,#47719,#47720,#47721,#47722,#47723,#47724,#47725,#47726,#47727,
#47728,#47729,#47730,#47731,#47732,#47733,#47734,#47735,#47736,#47737,#47738,
#47739,#47740,#47741,#47742,#47743,#47744,#47745,#47746,#47747,#47748,#47749,
#47750,#47751,#47752,#47753,#47754,#47755,#47756,#47757,#47758,#47759,#47760,
#47761,#47762,#47763,#47764,#47765,#47766,#47767,#47768,#47769,#47770,#47771,
#47772,#47773,#47774,#47775,#47776,#47777,#47778,#47779,#47780,#47781,#47782,
#47783,#47784,#47785,#47786,#47787,#47788,#47789,#47790,#47791,#47792,#47793,
#47794,#47795,#47796,#47797,#47798,#47799,#47800,#47801,#47802,#47803,#47804,
#47805,#47806,#47807,#47808,#47809,#47810,#47811,#47812,#47813,#47814,#47815,
#47816,#47817,#47818,#47819,#47820,#47821,#47822,#47823,#47824,#47825,#47826,
#47827,#47828,#47829,#47830,#47831,#47832,#47833,#47834,#47835,#47836,#47837,
#47838,#47839,#47840,#47841,#47842,#47843,#47844,#47845,#47846,#47847,#47848,
#47849,#47850,#47851,#47852,#47853,#47854,#47855,#47856,#47857,#47858,#47859,
#47860,#47861,#47862,#47863,#47864,#47865,#47866,#47867,#47868,#47869,#47870,
#47871,#47872,#47873,#47874,#47875,#47876),.UNSPECIFIED.,.F.,.F.,(4,2,2,
2,2,2,2,2,2,2,2,2,2,2,2,2,2,2,2,2,2,2,2,2,2,2,2,2,2,2,2,2,2,2,2,2,2,2,2,
2,2,2,2,2,2,2,2,2,2,2,2,2,2,2,2,2,2,2,2,2,2,2,2,2,2,2,2,2,2,2,2,2,2,2,2,
2,2,2,2,2,2,2,2,2,2,2,2,2,2,2,2,2,2,2,2,2,2,2,2,2,2,2,2,2,2,2,2,2,2,2,2,
2,2,2,2,2,2,2,2,2,2,2,2,2,2,2,2,2,2,2,2,2,2,2,2,2,2,2,2,2,2,2,2,2,2,2,2,
2,2,2,2,2,2,2,2,2,2,2,2,2,2,2,2,2,2,2,2,2,2,2,2,2,2,2,2,2,2,2,2,2,2,2,2,
2,2,2,4),(12.2072423730149,12.2352191971208,12.2826569185805,12.3199218461975,
12.3632367703069,12.4476936178893,12.570959081202,12.736960751213,12.7712185243792,
12.7899046594911,12.8110958594259,12.8477758062442,12.9775498472711,13.186850273024,
13.2414042611081,13.2791719333704,13.3191621616987,13.3843445062427,13.4283106072689,
13.571818250311,13.703077921244,13.7390148797864,13.7579955084812,13.7788333307434,
13.8137096799704,13.9274501747456,14.1649810223736,14.2107354896485,14.2484923886513,
14.2885024925577,14.3537950693201,14.3978697781285,14.5420032459383,14.6763405085586,
14.7101190497473,14.7287234735031,14.7500338458174,14.7873103976802,14.8364313854618,
14.9720349776009,14.9951544653213,15.1331017759202,15.1792500957851,15.2170924865626,
15.2569504404925,15.3213987389577,15.3646448623818,15.504077960292,15.5393575172787,
15.6436449362394,15.6784198201109,15.6971953543804,15.7182674144656,15.7543468588177,
15.8785479367335,16.0957546475812,16.1497574669088,16.1874404271184,16.2275915897599,
16.2936677418344,16.3385182845485,16.4872119182997,16.5225488814497,16.6229804370995,
16.6526714130605,16.6726354756428,16.6963210792083,16.7464171669615,16.7864055409356,
16.962630390052,16.9924079593312,17.088306000914,17.1333446489689,17.1705248555486,
17.2158728626694,17.3139913778747,17.4768169480921,17.5819524092582,17.6167855591192,
17.6355711590667,17.6566292337011,17.6926408650967,17.8162330412686,18.0343992755267,
18.0883065109779,18.1259740276626,18.1661521329659,18.2323828326118,18.2773877277253,
18.4270102994341,18.4414035791782,18.4691306508678,18.5619445513156,18.5913834403182,
18.6113154546221,18.6351376173856,18.6860428603105,18.8442137203142,19.0099584586975,
19.0560936002452,19.093934576838,19.1338008765076,19.1982873848837,19.2415700475714,
19.3812049082807,19.4103466456513,19.4394988404435,19.5313524466272,19.5606807983543,
19.5805980985628,19.6044755801851,19.6557311127837,19.8144735380744,19.9772665517165,
20.0241117669603,20.0621065620635,20.10170899509,20.164753729605,20.206640131746,
20.3387062130429,20.3770288819941,20.4046552093695,20.4998778235861,20.5295201131088,
20.5494768264847,20.5731859404254,20.623421447614,20.6635769726289,20.8413927447492,
20.9555215426404,21.0034034723294,21.0407764988915,21.0832855070926,21.1628107718385,
21.347842788525,21.3712421860454,21.4688546884355,21.4986088990629,21.5185848426185,
21.5422513859962,21.5922080050725,21.6320278687749,21.8067026296436,21.8713843789855,
21.9449867583524,21.9868524349962,22.024353265849,22.0742603937447,22.2173877193162,
22.3441788131783,22.4383303184236,22.4678730112234,22.4878055784151,22.5115165527441,
22.561887359572,22.7206260368362,22.8857575036312,22.9324261795403,22.970362556157,
23.0028103026188,23.0530709333166,23.1155220944091,23.2491008063794,23.395836497707,
23.4315490522561,23.4504940804626,23.4704160773139,23.4722676083633,23.4741530752907,
23.4761135314339,23.4781910345803,23.4804314105348,23.4828868373316,23.4836044905581,
23.484530463745,23.4857418875848,23.4873529350992,23.4895365131139,23.5211848320784,
23.5827324207832,23.8242118109602,23.8900513082125,23.9302202891897,23.965754532381,
24.0033012563355,24.0582608056696,24.2611810843085),.UNSPECIFIED.) ;
#310=B_SPLINE_CURVE_WITH_KNOTS('',3,(#47879,#47880,#47881,#47882,#47883,
#47884,#47885,#47886,#47887,#47888,#47889,#47890,#47891,#47892,#47893,#47894,
#47895,#47896,#47897,#47898,#47899,#47900,#47901,#47902,#47903,#47904,#47905,
#47906,#47907,#47908,#47909,#47910,#47911,#47912,#47913,#47914,#47915,#47916,
#47917,#47918,#47919,#47920,#47921,#47922,#47923,#47924,#47925,#47926,#47927,
#47928,#47929,#47930,#47931,#47932,#47933,#47934,#47935,#47936,#47937,#47938,
#47939,#47940,#47941,#47942,#47943,#47944,#47945,#47946,#47947,#47948,#47949,
#47950,#47951,#47952,#47953,#47954,#47955,#47956,#47957,#47958,#47959,#47960,
#47961,#47962,#47963,#47964,#47965,#47966,#47967,#47968,#47969,#47970,#47971,
#47972,#47973,#47974,#47975,#47976,#47977,#47978,#47979,#47980,#47981,#47982,
#47983,#47984,#47985,#47986,#47987,#47988,#47989,#47990,#47991,#47992,#47993,
#47994,#47995,#47996,#47997,#47998,#47999,#48000,#48001,#48002,#48003,#48004,
#48005,#48006,#48007,#48008,#48009,#48010,#48011,#48012,#48013,#48014,#48015,
#48016,#48017,#48018,#48019,#48020,#48021,#48022,#48023,#48024,#48025,#48026,
#48027,#48028,#48029,#48030,#48031,#48032,#48033,#48034,#48035,#48036,#48037,
#48038,#48039,#48040,#48041,#48042,#48043,#48044,#48045,#48046,#48047,#48048,
#48049,#48050,#48051,#48052,#48053,#48054,#48055,#48056,#48057,#48058,#48059,
#48060,#48061,#48062,#48063,#48064,#48065,#48066,#48067,#48068,#48069,#48070,
#48071,#48072,#48073,#48074,#48075,#48076,#48077,#48078,#48079,#48080,#48081,
#48082,#48083,#48084,#48085,#48086,#48087,#48088,#48089,#48090,#48091,#48092,
#48093,#48094,#48095,#48096,#48097,#48098,#48099,#48100,#48101,#48102,#48103,
#48104,#48105,#48106,#48107,#48108,#48109,#48110,#48111,#48112,#48113,#48114,
#48115,#48116,#48117,#48118,#48119,#48120,#48121,#48122,#48123,#48124,#48125,
#48126,#48127,#48128,#48129,#48130,#48131,#48132,#48133,#48134,#48135,#48136,
#48137),.UNSPECIFIED.,.F.,.F.,(4,3,3,3,3,3,3,3,3,3,3,3,3,3,3,3,3,3,3,3,
3,3,3,3,3,3,3,3,3,3,3,3,3,3,3,3,3,3,3,3,3,3,3,3,3,3,3,3,3,3,3,3,3,3,3,3,
3,3,3,3,3,3,3,3,3,3,3,3,3,3,3,3,3,3,3,3,3,3,3,3,3,3,3,3,3,3,4),(-84.8061323363251,
-84.7434695854549,-84.6808110755322,-84.6181547160668,-84.5554984169936,
-84.4928322445765,-84.4301641985852,-84.3674819098806,-84.3072727343469,
-84.2449152840996,-84.1827586433676,-84.1206101572369,-84.0584666053991,
-83.9959532371414,-83.9338046160016,-83.8711088741851,-83.8084131323685,
-83.7460214897466,-83.6836387031221,-83.6212620261393,-83.5588887142844,
-83.4965090091967,-83.4341289979585,-83.3717356186068,-83.3095535303901,
-83.2471960801428,-83.1849129227894,-83.1226366457664,-83.0603642914639,
-82.9979467007009,-82.9356680248854,-82.8731809766486,-82.8106939284118,
-82.7483364781645,-82.6860202553423,-82.6237106902526,-82.5614048951035,
-82.499012252936,-82.4367000854348,-82.3742672059341,-82.3118343264334,
-82.2494768761861,-82.1871654863429,-82.1248607634951,-82.062559809642,
-82.0001635383452,-81.9378561629617,-81.8754154437083,-81.812974724455,
-81.7506172742077,-81.6883094565925,-81.6260083494707,-81.5637110472351,
-81.5013120660455,-81.4390083946495,-81.376561758563,-81.3141151224766,
-81.2517576722293,-81.189445700161,-81.1271403995358,-81.0648388735713,
-81.002443035303,-80.9401351071849,-80.8776953138415,-80.8152555204982,
-80.7528980702509,-80.6905887871496,-80.628286198462,-80.5659874016961,
-80.503589530902,-80.4412843477519,-80.3788401331359,-80.3163959185198,
-80.2540384682725,-80.1917278738116,-80.1294239633962,-80.0671238373162,
-80.0047269571225,-79.9424204389808,-79.8799783777611,-79.8175363165415,
-79.7551789658218,-79.6928320409426,-79.6304912444782,-79.5681557198953,
-79.5058202388051,-79.4912145662646),.UNSPECIFIED.) ;
#311=B_SPLINE_CURVE_WITH_KNOTS('',3,(#48179,#48180,#48181,#48182,#48183,
#48184,#48185,#48186,#48187,#48188,#48189,#48190,#48191,#48192,#48193,#48194,
#48195,#48196),.UNSPECIFIED.,.F.,.F.,(4,2,2,2,2,2,2,2,4),(-3.02737420106107,
-2.83815008504339,-2.64892596902571,-2.45972830991075,-2.2705306507958,
-2.08133299168085,-1.8921353325659,-1.70291121654822,-1.51368710053054),
 .UNSPECIFIED.) ;
#312=B_SPLINE_CURVE_WITH_KNOTS('',3,(#48199,#48200,#48201,#48202,#48203,
#48204,#48205,#48206,#48207,#48208,#48209,#48210,#48211,#48212,#48213,#48214,
#48215,#48216),.UNSPECIFIED.,.F.,.F.,(4,2,2,2,2,2,2,2,4),(-1.51368710053053,
-1.32446298451285,-1.13523886849517,-0.946041209380219,-0.756843550265268,
-0.567645891150316,-0.378448232035365,-0.189224116017682,0.),
 .UNSPECIFIED.) ;
#313=B_SPLINE_CURVE_WITH_KNOTS('',3,(#48271,#48272,#48273,#48274,#48275,
#48276,#48277,#48278,#48279,#48280,#48281,#48282,#48283,#48284),
 .UNSPECIFIED.,.F.,.F.,(4,2,2,2,2,2,4),(-2.86271597092642,-2.47550138268059,
-2.09247759219639,-1.63307121855681,-1.1818186467659,-0.689259812314864,
-1.00000004810141E-6),.UNSPECIFIED.) ;
#314=B_SPLINE_CURVE_WITH_KNOTS('',3,(#48285,#48286,#48287,#48288,#48289,
#48290,#48291,#48292,#48293,#48294,#48295,#48296,#48297,#48298,#48299,#48300,
#48301,#48302,#48303,#48304,#48305,#48306,#48307,#48308,#48309,#48310,#48311,
#48312,#48313,#48314,#48315,#48316,#48317,#48318,#48319,#48320,#48321,#48322,
#48323,#48324,#48325,#48326,#48327,#48328,#48329,#48330,#48331,#48332,#48333,
#48334,#48335,#48336,#48337,#48338,#48339,#48340,#48341,#48342,#48343,#48344,
#48345,#48346,#48347,#48348,#48349,#48350,#48351,#48352,#48353,#48354,#48355,
#48356,#48357,#48358,#48359,#48360,#48361,#48362,#48363,#48364,#48365,#48366,
#48367,#48368,#48369,#48370,#48371,#48372,#48373,#48374,#48375,#48376,#48377,
#48378,#48379,#48380,#48381,#48382,#48383,#48384,#48385,#48386,#48387,#48388,
#48389,#48390,#48391,#48392,#48393,#48394,#48395,#48396,#48397,#48398,#48399,
#48400,#48401,#48402,#48403,#48404,#48405,#48406,#48407,#48408,#48409,#48410,
#48411,#48412,#48413,#48414),.UNSPECIFIED.,.F.,.F.,(4,3,3,3,3,3,3,3,3,3,
3,3,3,3,3,3,3,3,3,3,3,3,3,3,3,3,3,3,3,3,3,3,3,3,3,3,3,3,3,3,3,3,3,4),(0.,
0.134956132691862,0.150548210071358,0.284576496872476,0.42651189256128,
0.561684253595667,0.696272635973996,0.82933537653257,0.852318079627691,
0.867571174403126,1.00107306380577,1.13432953696973,1.23838937708017,1.37208338021623,
1.50558528557567,1.60554221520874,1.69300452863768,1.71195887004486,1.8435302488514,
1.97562049759594,2.10733784413285,2.23767920145199,2.30524072264026,2.43707975007448,
2.52155729666941,2.54226292029336,2.67187769228001,2.80231319807097,2.93934656128157,
3.06892063981614,3.19735578614655,3.32372079372745,3.35044665091336,3.38443065417707,
3.51315247311986,3.64233608971587,3.75232450310687,3.82177124080331,3.86231291649787,
3.87975886711596,4.00788164525527,4.13559019490866,4.26173696563685,4.37270046381608),
 .UNSPECIFIED.) ;
#315=B_SPLINE_CURVE_WITH_KNOTS('',3,(#48430,#48431,#48432,#48433,#48434,
#48435,#48436,#48437,#48438,#48439,#48440,#48441,#48442,#48443,#48444,#48445,
#48446,#48447,#48448,#48449,#48450,#48451,#48452,#48453,#48454,#48455,#48456,
#48457,#48458,#48459,#48460,#48461,#48462,#48463),.UNSPECIFIED.,.T.,.F.,
(4,2,2,2,2,2,2,2,2,2,2,2,2,2,2,2,4),(0.,0.131943994423176,0.263887988846351,
0.395831447701094,0.527774906555838,0.659718365410582,0.791661824265325,
0.9236058186885,1.05554981311168,1.18749380753485,1.31943780195803,1.45138126081277,
1.58332471966751,1.71526817852226,1.847211637377,1.97915563180018,2.11109962622335),
 .UNSPECIFIED.) ;
#316=B_SPLINE_CURVE_WITH_KNOTS('',3,(#48465,#48466,#48467,#48468,#48469,
#48470,#48471,#48472,#48473,#48474,#48475,#48476,#48477,#48478,#48479,#48480,
#48481,#48482,#48483,#48484,#48485,#48486,#48487,#48488,#48489,#48490,#48491,
#48492,#48493,#48494,#48495,#48496,#48497,#48498),.UNSPECIFIED.,.T.,.F.,
(4,2,2,2,2,2,2,2,2,2,2,2,2,2,2,2,4),(0.,0.131943994423175,0.263887988846351,
0.395831447701094,0.527774906555838,0.659718365410582,0.791661824265325,
0.923605818688501,1.05554981311168,1.18749380753485,1.31943780195803,1.45138126081277,
1.58332471966751,1.71526817852226,1.847211637377,1.97915563180018,2.11109962622335),
 .UNSPECIFIED.) ;
#317=B_SPLINE_CURVE_WITH_KNOTS('',3,(#48500,#48501,#48502,#48503,#48504,
#48505,#48506,#48507,#48508,#48509,#48510,#48511,#48512,#48513,#48514,#48515,
#48516,#48517,#48518,#48519,#48520,#48521,#48522,#48523,#48524,#48525,#48526,
#48527,#48528,#48529,#48530,#48531,#48532,#48533),.UNSPECIFIED.,.T.,.F.,
(4,2,2,2,2,2,2,2,2,2,2,2,2,2,2,2,4),(0.,0.131943994423175,0.26388798884635,
0.395831447701094,0.527774906555837,0.659718365410581,0.791661824265324,
0.9236058186885,1.05554981311168,1.18749380753485,1.31943780195803,1.45138126081277,
1.58332471966751,1.71526817852226,1.847211637377,1.97915563180018,2.11109962622335),
 .UNSPECIFIED.) ;
#318=B_SPLINE_CURVE_WITH_KNOTS('',1,(#48613,#48614),.UNSPECIFIED.,.F.,.F.,
(2,2),(0.,1.00000015726815),.UNSPECIFIED.) ;
#319=B_SPLINE_CURVE_WITH_KNOTS('',3,(#48615,#48616,#48617,#48618,#48619,
#48620,#48621,#48622,#48623,#48624,#48625,#48626,#48627,#48628,#48629,#48630,
#48631,#48632,#48633,#48634,#48635,#48636,#48637,#48638,#48639,#48640,#48641,
#48642,#48643,#48644,#48645,#48646,#48647,#48648,#48649,#48650,#48651,#48652,
#48653,#48654,#48655,#48656,#48657,#48658,#48659,#48660,#48661,#48662,#48663,
#48664,#48665,#48666,#48667,#48668,#48669),.UNSPECIFIED.,.T.,.F.,(4,2,2,
2,2,2,2,2,2,2,2,3,2,2,2,2,2,2,2,2,2,2,2,2,2,2,4),(0.630282646728311,0.638093074049646,
0.647002723099591,0.666366138141934,0.696779929267916,0.740656076798668,
0.804443699294602,0.892545576433704,1.02104051551844,1.06836668156106,1.13376734398064,
1.19519452402957,1.25836937632244,1.38453630464938,1.44224028136641,1.49447273220586,
1.54567596360975,1.59097946229049,1.63573830290034,1.67109818487044,1.70152973349188,
1.72897522297272,1.75594681875993,1.77754167411064,1.80981305883969,1.82286183962224,
1.82547717075788),.UNSPECIFIED.) ;
#320=B_SPLINE_CURVE_WITH_KNOTS('',1,(#48740,#48741),.UNSPECIFIED.,.F.,.F.,
(2,2),(0.,1.00000015726814),.UNSPECIFIED.) ;
#321=B_SPLINE_CURVE_WITH_KNOTS('',3,(#48742,#48743,#48744,#48745,#48746,
#48747,#48748,#48749,#48750,#48751,#48752,#48753,#48754,#48755,#48756,#48757,
#48758,#48759,#48760,#48761,#48762,#48763,#48764,#48765,#48766,#48767,#48768,
#48769,#48770,#48771,#48772,#48773,#48774,#48775,#48776,#48777,#48778,#48779,
#48780,#48781,#48782,#48783,#48784,#48785,#48786,#48787,#48788,#48789,#48790,
#48791,#48792,#48793,#48794,#48795,#48796),.UNSPECIFIED.,.T.,.F.,(4,2,2,
2,2,2,2,2,2,2,2,3,2,2,2,2,2,2,2,2,2,2,2,2,2,2,4),(0.630282646727731,0.638093074049046,
0.647002723098976,0.666366138141306,0.696779929267319,0.74065607679813,
0.804443699294194,0.892545576433443,1.02104051551834,1.06836668156095,1.13376734398052,
1.19519452402944,1.25836937632229,1.38453630464921,1.44224028136624,1.49447273220568,
1.54567596360952,1.59097946229014,1.63573830289993,1.67109818486996,1.70152973349133,
1.72897522297213,1.7559468187593,1.77754167410999,1.80981305883899,1.82286183962152,
1.82547717075717),.UNSPECIFIED.) ;
#322=B_SPLINE_CURVE_WITH_KNOTS('',1,(#48867,#48868),.UNSPECIFIED.,.F.,.F.,
(2,2),(0.,1.00000015726815),.UNSPECIFIED.) ;
#323=B_SPLINE_CURVE_WITH_KNOTS('',3,(#48869,#48870,#48871,#48872,#48873,
#48874,#48875,#48876,#48877,#48878,#48879,#48880,#48881,#48882,#48883,#48884,
#48885,#48886,#48887,#48888,#48889,#48890,#48891,#48892,#48893,#48894,#48895,
#48896,#48897,#48898,#48899,#48900,#48901,#48902,#48903,#48904,#48905,#48906,
#48907,#48908,#48909,#48910,#48911,#48912,#48913,#48914,#48915,#48916,#48917,
#48918,#48919,#48920,#48921,#48922,#48923),.UNSPECIFIED.,.T.,.F.,(4,2,2,
2,2,2,2,2,2,2,2,3,2,2,2,2,2,2,2,2,2,2,2,2,2,2,4),(0.630282646727811,0.638093074049133,
0.647002723099068,0.66636613814141,0.696779929267413,0.740656076798171,
0.804443699294128,0.892545576433259,1.02104051551798,1.06836668156057,1.13376734398012,
1.19519452402904,1.25836937632187,1.38453630464876,1.44224028136575,1.49447273220515,
1.545675963609,1.5909794622897,1.63573830289951,1.67109818486956,1.70152973349097,
1.72897522297177,1.75594681875897,1.77754167410966,1.80981305883867,1.82286183962121,
1.82547717075685),.UNSPECIFIED.) ;
#324=B_SPLINE_CURVE_WITH_KNOTS('',3,(#49617,#49618,#49619,#49620,#49621,
#49622,#49623,#49624,#49625,#49626,#49627,#49628,#49629,#49630,#49631,#49632,
#49633,#49634,#49635,#49636,#49637,#49638,#49639,#49640,#49641,#49642,#49643,
#49644,#49645,#49646,#49647,#49648,#49649,#49650,#49651,#49652,#49653,#49654,
#49655,#49656,#49657,#49658,#49659,#49660,#49661,#49662,#49663,#49664,#49665,
#49666,#49667,#49668,#49669,#49670,#49671,#49672,#49673,#49674,#49675,#49676,
#49677,#49678,#49679,#49680,#49681,#49682,#49683,#49684,#49685,#49686,#49687,
#49688,#49689,#49690,#49691,#49692,#49693,#49694,#49695,#49696,#49697,#49698,
#49699,#49700,#49701,#49702,#49703,#49704,#49705,#49706,#49707,#49708,#49709,
#49710,#49711,#49712,#49713,#49714,#49715,#49716,#49717,#49718,#49719,#49720,
#49721,#49722,#49723,#49724,#49725,#49726,#49727,#49728,#49729,#49730,#49731,
#49732,#49733,#49734,#49735,#49736,#49737,#49738,#49739,#49740,#49741,#49742,
#49743,#49744,#49745,#49746,#49747,#49748,#49749,#49750,#49751,#49752),
 .UNSPECIFIED.,.F.,.F.,(4,3,3,3,3,3,3,3,3,3,3,3,3,3,3,3,3,3,3,3,3,3,3,3,
3,3,3,3,3,3,3,3,3,3,3,3,3,3,3,3,3,3,3,3,3,4),(2.18408295184663E-6,0.123020428160983,
0.15963065273004,0.281586707028109,0.404758111867876,0.527955343315918,
0.650212475416643,0.73717114933423,0.753380162546799,0.767542900869677,
0.772752757916178,0.895020990109926,1.01719177953705,1.12547299608439,1.2478361314004,
1.37486418901594,1.50189224663149,1.51295714877596,1.63388146162191,1.75558436713017,
1.8770599821172,1.99728332804384,2.08122088405351,2.1937412593632,2.22090947074412,
2.24234748900313,2.25711688775144,2.31417322948663,2.43433900312252,2.55521631537028,
2.67592273084785,2.79589111461474,2.91402806997879,2.98138388653104,2.99369222579519,
3.02628757255141,3.14563906826117,3.26562493318584,3.38565980391277,3.45762068722671,
3.4747197256305,3.48565352718463,3.60526986962867,3.72467353676032,3.84274714773479,
3.95993145615853),.UNSPECIFIED.) ;
#325=B_SPLINE_CURVE_WITH_KNOTS('',3,(#49754,#49755,#49756,#49757,#49758,
#49759,#49760,#49761,#49762,#49763,#49764,#49765,#49766,#49767,#49768,#49769,
#49770,#49771,#49772,#49773,#49774,#49775,#49776,#49777,#49778,#49779,#49780,
#49781,#49782,#49783,#49784,#49785,#49786,#49787,#49788,#49789,#49790,#49791,
#49792,#49793,#49794,#49795,#49796,#49797,#49798,#49799,#49800,#49801,#49802,
#49803,#49804,#49805,#49806,#49807,#49808,#49809,#49810,#49811,#49812,#49813,
#49814,#49815,#49816,#49817,#49818,#49819,#49820,#49821,#49822,#49823,#49824,
#49825,#49826,#49827,#49828,#49829,#49830,#49831,#49832,#49833,#49834,#49835,
#49836,#49837,#49838,#49839,#49840,#49841,#49842,#49843,#49844,#49845,#49846,
#49847,#49848,#49849,#49850,#49851,#49852,#49853,#49854,#49855,#49856,#49857,
#49858,#49859,#49860,#49861,#49862,#49863,#49864,#49865,#49866,#49867,#49868,
#49869,#49870,#49871,#49872,#49873,#49874,#49875,#49876,#49877,#49878,#49879,
#49880,#49881,#49882,#49883,#49884,#49885,#49886,#49887,#49888,#49889,#49890,
#49891,#49892),.UNSPECIFIED.,.F.,.F.,(4,3,3,3,3,3,3,3,3,3,3,3,3,3,3,3,3,
3,3,3,3,3,3,3,3,3,3,3,3,3,3,3,3,3,3,3,3,3,3,3,3,3,3,3,3,3,4),(0.,0.119588194315636,
0.152837981974594,0.271317579881898,0.390765157706876,0.510593513266912,
0.630145691521126,0.687516409369078,0.712777341230908,0.729146013580884,
0.746103307941794,0.866247064092426,0.986797445428536,1.08911143430474,
1.20940114144625,1.32989963245365,1.41810059920495,1.44370363426542,1.46133334350923,
1.47491872658128,1.59493286517016,1.71620190524513,1.83753914921351,1.9580232347556,
2.03550736646401,2.15666423324517,2.18484158143669,2.20157601869575,2.21395295588132,
2.33405734051309,2.45539974153245,2.57743148373137,2.69927308058649,2.82035616630182,
2.90588765281033,2.94463079271265,2.95935015045668,2.99141913931883,3.11252755730056,
3.23451829514276,3.35702313311209,3.44804384530054,3.4621411140443,3.58565221622721,
3.70869195186839,3.83243873732217,3.95618552277594),.UNSPECIFIED.) ;
#326=B_SPLINE_CURVE_WITH_KNOTS('',3,(#49893,#49894,#49895,#49896),
 .UNSPECIFIED.,.F.,.F.,(4,4),(-0.00157738977958374,0.),.UNSPECIFIED.) ;
#327=B_SPLINE_CURVE_WITH_KNOTS('',3,(#50590,#50591,#50592,#50593,#50594,
#50595,#50596,#50597,#50598,#50599,#50600,#50601,#50602,#50603,#50604,#50605,
#50606,#50607,#50608,#50609,#50610,#50611,#50612,#50613,#50614,#50615,#50616,
#50617,#50618,#50619,#50620,#50621,#50622,#50623,#50624,#50625,#50626,#50627,
#50628,#50629,#50630,#50631,#50632,#50633,#50634,#50635,#50636,#50637,#50638,
#50639,#50640,#50641,#50642,#50643,#50644,#50645,#50646,#50647,#50648,#50649,
#50650,#50651,#50652,#50653,#50654,#50655,#50656,#50657,#50658,#50659,#50660,
#50661,#50662,#50663,#50664,#50665,#50666,#50667,#50668,#50669,#50670,#50671,
#50672,#50673,#50674,#50675,#50676,#50677,#50678,#50679,#50680,#50681,#50682,
#50683,#50684,#50685,#50686,#50687,#50688,#50689,#50690,#50691,#50692,#50693,
#50694,#50695,#50696,#50697,#50698,#50699,#50700,#50701,#50702,#50703,#50704,
#50705,#50706,#50707,#50708,#50709,#50710,#50711,#50712,#50713,#50714,#50715,
#50716,#50717,#50718,#50719,#50720,#50721,#50722,#50723,#50724,#50725),
 .UNSPECIFIED.,.F.,.F.,(4,3,3,3,3,3,3,3,3,3,3,3,3,3,3,3,3,3,3,3,3,3,3,3,
3,3,3,3,3,3,3,3,3,3,3,3,3,3,3,3,3,3,3,3,3,4),(0.,0.119588186287281,0.152837981974752,
0.27074719741009,0.390267991763342,0.510094677789097,0.61965267305727,0.674431670691357,
0.708278729033239,0.729210668325444,0.735267875681489,0.855351785448358,
0.975909365301059,1.08911143430487,1.20925610650812,1.33411169372933,1.45896728095053,
1.47047783077841,1.59044520192017,1.71170224358119,1.8330458276188,1.95355177499451,
2.03550736646409,2.15666422985477,2.18484158150908,2.20157601759723,2.21395295550005,
2.33397535245444,2.45526219673935,2.57760433999465,2.69951082281856,2.82207079628956,
2.94463076976056,2.95773533199481,2.99141913931887,3.11248092205803,3.23444145233754,
3.35694954126384,3.43211505332396,3.45237084951486,3.46204675189966,3.4646398157526,
3.58757479015538,3.7106123337395,3.83339892825768,3.95618552277586),
 .UNSPECIFIED.) ;
#328=B_SPLINE_CURVE_WITH_KNOTS('',3,(#50726,#50727,#50728,#50729),
 .UNSPECIFIED.,.F.,.F.,(4,4),(0.,0.00157736468337877),.UNSPECIFIED.) ;
#329=B_SPLINE_CURVE_WITH_KNOTS('',3,(#50730,#50731,#50732,#50733,#50734,
#50735,#50736,#50737,#50738,#50739,#50740,#50741,#50742,#50743,#50744,#50745,
#50746,#50747,#50748,#50749,#50750,#50751,#50752,#50753,#50754,#50755,#50756,
#50757,#50758,#50759,#50760,#50761,#50762,#50763,#50764,#50765,#50766,#50767,
#50768,#50769,#50770,#50771,#50772,#50773,#50774,#50775,#50776,#50777,#50778,
#50779,#50780,#50781,#50782,#50783,#50784,#50785,#50786,#50787,#50788,#50789,
#50790,#50791,#50792,#50793,#50794,#50795,#50796,#50797,#50798,#50799,#50800,
#50801,#50802,#50803,#50804,#50805,#50806,#50807,#50808,#50809,#50810,#50811,
#50812,#50813,#50814,#50815,#50816,#50817,#50818,#50819,#50820,#50821,#50822,
#50823,#50824,#50825,#50826,#50827,#50828,#50829,#50830,#50831,#50832,#50833,
#50834,#50835,#50836,#50837,#50838,#50839,#50840,#50841,#50842,#50843,#50844,
#50845,#50846,#50847,#50848,#50849,#50850,#50851,#50852,#50853,#50854,#50855,
#50856,#50857,#50858,#50859),.UNSPECIFIED.,.F.,.F.,(4,3,3,3,3,3,3,3,3,3,
3,3,3,3,3,3,3,3,3,3,3,3,3,3,3,3,3,3,3,3,3,3,3,3,3,3,3,3,3,3,3,3,3,4),(0.,
0.123018240977632,0.159630652729786,0.281611310473703,0.404794365344837,
0.527980108221235,0.650146381112849,0.754308226515199,0.766561817559909,
0.888812162564381,1.01099748544193,1.12547299608417,1.24783613177185,1.37486419163187,
1.50189225149189,1.51295715334221,1.63388146506136,1.75558437158114,1.87705998894425,
1.99728334001246,2.08122088405321,2.20269423912377,2.24766412561392,2.25939910057906,
2.37910849227707,2.49977219254656,2.62076457057125,2.74102482887587,2.86028037404055,
2.94328397329584,2.97018145502892,2.98651707444645,3.00353032282715,3.02628757255113,
3.14563905790358,3.26562491787666,3.38565979382963,3.45762067936319,3.48901510291289,
3.55710178412575,3.67664845340404,3.79570446790245,3.91331257842532,3.95993145615846),
 .UNSPECIFIED.) ;
#330=B_SPLINE_CURVE_WITH_KNOTS('',3,(#51209,#51210,#51211,#51212,#51213,
#51214,#51215,#51216,#51217,#51218,#51219,#51220,#51221,#51222,#51223,#51224,
#51225,#51226,#51227,#51228,#51229,#51230,#51231,#51232,#51233,#51234,#51235,
#51236,#51237,#51238,#51239,#51240,#51241,#51242,#51243,#51244,#51245,#51246,
#51247,#51248,#51249,#51250,#51251,#51252,#51253,#51254,#51255,#51256,#51257,
#51258,#51259,#51260,#51261,#51262,#51263,#51264,#51265,#51266,#51267,#51268,
#51269,#51270,#51271,#51272,#51273,#51274,#51275,#51276,#51277,#51278,#51279,
#51280,#51281,#51282,#51283,#51284,#51285,#51286,#51287,#51288,#51289,#51290,
#51291,#51292,#51293,#51294,#51295,#51296,#51297,#51298,#51299,#51300,#51301,
#51302,#51303,#51304,#51305,#51306,#51307,#51308,#51309,#51310,#51311,#51312,
#51313,#51314,#51315,#51316,#51317,#51318,#51319,#51320,#51321,#51322,#51323,
#51324,#51325,#51326,#51327,#51328,#51329,#51330,#51331,#51332,#51333,#51334,
#51335),.UNSPECIFIED.,.F.,.F.,(4,3,3,3,3,3,3,3,3,3,3,3,3,3,3,3,3,3,3,3,
3,3,3,3,3,3,3,3,3,3,3,3,3,3,3,3,3,3,3,3,3,3,4),(6.28075782615231E-6,0.134962417714373,
0.150548210071363,0.284576510029121,0.4265119018776,0.561684260662624,0.696272643598151,
0.829335384069975,0.852318077423036,0.865259157588972,0.998756784143564,
1.13201928919157,1.2383893770802,1.37204896176997,1.50568859332497,1.63839311050962,
1.69300451064955,1.709972305995,1.84153084943448,1.97362301373667,2.10534945672862,
2.23570269565275,2.30524072264028,2.43707979046566,2.52155729901495,2.53397976802391,
2.66352086058859,2.79392303702358,2.92452377215859,3.05420467689459,3.18278646002985,
3.30927444084533,3.35044665091337,3.38440368336101,3.51310617758439,3.64228386708091,
3.77121409589701,3.85162416869255,3.8665988626213,3.99473725549904,4.12250938678091,
4.2487399621133,4.37270046381604),.UNSPECIFIED.) ;
#331=B_SPLINE_CURVE_WITH_KNOTS('',3,(#51685,#51686,#51687,#51688,#51689,
#51690,#51691,#51692,#51693,#51694,#51695,#51696,#51697,#51698,#51699,#51700,
#51701,#51702,#51703,#51704,#51705,#51706,#51707,#51708,#51709,#51710,#51711,
#51712,#51713,#51714,#51715,#51716,#51717,#51718,#51719,#51720,#51721,#51722,
#51723,#51724,#51725,#51726,#51727,#51728,#51729,#51730,#51731,#51732,#51733,
#51734,#51735,#51736,#51737,#51738,#51739,#51740,#51741,#51742,#51743,#51744,
#51745,#51746,#51747,#51748,#51749,#51750,#51751,#51752,#51753,#51754,#51755,
#51756,#51757,#51758,#51759,#51760,#51761,#51762,#51763,#51764,#51765,#51766,
#51767,#51768,#51769,#51770,#51771,#51772,#51773,#51774,#51775,#51776,#51777,
#51778,#51779,#51780,#51781,#51782,#51783,#51784,#51785,#51786,#51787,#51788,
#51789,#51790,#51791,#51792,#51793,#51794,#51795,#51796,#51797,#51798,#51799,
#51800,#51801,#51802,#51803,#51804,#51805,#51806,#51807,#51808,#51809,#51810,
#51811,#51812,#51813,#51814),.UNSPECIFIED.,.F.,.F.,(4,3,3,3,3,3,3,3,3,3,
3,3,3,3,3,3,3,3,3,3,3,3,3,3,3,3,3,3,3,3,3,3,3,3,3,3,3,3,3,3,3,3,3,4),(0.,
0.127950841635321,0.138734436835898,0.266927318078744,0.39452245359627,
0.522788716549364,0.651083437735894,0.779381949996588,0.799252792649835,
0.815195110372998,0.944426122570075,1.07435921574577,1.16427748677867,1.29343658906208,
1.42315651822206,1.55284275525532,1.60917412077767,1.62373987619339,1.7535153835574,
1.88480435100334,2.01633375694167,2.14727531103612,2.21103030364097,2.34228118872861,
2.43432232649351,2.44667434785096,2.57724334887867,2.70921236615828,2.84205677072627,
2.97499463641324,3.1073063974138,3.237949250727,3.27831317758158,3.29127088822594,
3.4254816777589,3.55892260811963,3.69298599227836,3.77698239380477,3.8058365140531,
3.83035997939428,3.96532060706772,4.10051008302849,4.23496370739636,4.36495720448964),
 .UNSPECIFIED.) ;
#332=B_SPLINE_CURVE_WITH_KNOTS('',3,(#51815,#51816,#51817,#51818),
 .UNSPECIFIED.,.F.,.F.,(4,4),(0.,0.00110748569343258),.UNSPECIFIED.) ;
#570=SHAPE_REPRESENTATION_RELATIONSHIP('SRR','None',#63884,#585) ;
#585=ADVANCED_BREP_SHAPE_REPRESENTATION('',(#615),#63814) ;
#600=STYLED_ITEM('',(#63964),#615) ;
#615=MANIFOLD_SOLID_BREP('Body1',#15499) ;
#731=FACE_BOUND('',#2733,.T.) ;
#732=FACE_BOUND('',#2739,.T.) ;
#733=FACE_BOUND('',#2741,.T.) ;
#734=FACE_BOUND('',#2745,.T.) ;
#735=FACE_BOUND('',#2751,.T.) ;
#736=FACE_BOUND('',#2755,.T.) ;
#737=FACE_BOUND('',#2758,.T.) ;
#738=FACE_BOUND('',#2759,.T.) ;
#739=FACE_BOUND('',#2760,.T.) ;
#740=FACE_BOUND('',#2762,.T.) ;
#741=FACE_BOUND('',#2765,.T.) ;
#742=FACE_BOUND('',#2775,.T.) ;
#743=FACE_BOUND('',#2779,.T.) ;
#744=FACE_BOUND('',#2787,.T.) ;
#745=FACE_BOUND('',#2792,.T.) ;
#746=FACE_BOUND('',#2795,.T.) ;
#747=FACE_BOUND('',#2798,.T.) ;
#882=PLANE('',#16082) ;
#883=PLANE('',#16097) ;
#884=PLANE('',#16105) ;
#885=PLANE('',#16118) ;
#886=PLANE('',#16125) ;
#887=PLANE('',#16133) ;
#888=PLANE('',#16137) ;
#889=PLANE('',#16142) ;
#890=PLANE('',#16143) ;
#891=PLANE('',#16145) ;
#892=PLANE('',#16148) ;
#893=PLANE('',#16151) ;
#894=PLANE('',#16154) ;
#895=PLANE('',#16160) ;
#896=PLANE('',#16164) ;
#897=PLANE('',#16167) ;
#1200=CYLINDRICAL_SURFACE('',#16026,19.425) ;
#1201=CYLINDRICAL_SURFACE('',#16028,19.425) ;
#1202=CYLINDRICAL_SURFACE('',#16029,19.425) ;
#1203=CYLINDRICAL_SURFACE('',#16030,19.425) ;
#1204=CYLINDRICAL_SURFACE('',#16031,19.425) ;
#1205=CYLINDRICAL_SURFACE('',#16032,19.425) ;
#1206=CYLINDRICAL_SURFACE('',#16033,19.425) ;
#1207=CYLINDRICAL_SURFACE('',#16034,19.425) ;
#1208=CYLINDRICAL_SURFACE('',#16035,19.425) ;
#1209=CYLINDRICAL_SURFACE('',#16036,19.425) ;
#1210=CYLINDRICAL_SURFACE('',#16037,19.425) ;
#1211=CYLINDRICAL_SURFACE('',#16038,19.425) ;
#1212=CYLINDRICAL_SURFACE('',#16039,19.425) ;
#1213=CYLINDRICAL_SURFACE('',#16040,22.12975) ;
#1214=CYLINDRICAL_SURFACE('',#16042,22.12975) ;
#1215=CYLINDRICAL_SURFACE('',#16043,22.12975) ;
#1216=CYLINDRICAL_SURFACE('',#16044,22.12975) ;
#1217=CYLINDRICAL_SURFACE('',#16045,22.12975) ;
#1218=CYLINDRICAL_SURFACE('',#16046,22.12975) ;
#1219=CYLINDRICAL_SURFACE('',#16047,22.12975) ;
#1220=CYLINDRICAL_SURFACE('',#16049,20.33524) ;
#1221=CYLINDRICAL_SURFACE('',#16051,20.33524) ;
#1222=CYLINDRICAL_SURFACE('',#16052,20.33524) ;
#1223=CYLINDRICAL_SURFACE('',#16053,20.33524) ;
#1224=CYLINDRICAL_SURFACE('',#16054,20.33524) ;
#1225=CYLINDRICAL_SURFACE('',#16055,20.33524) ;
#1226=CYLINDRICAL_SURFACE('',#16056,18.56595) ;
#1227=CYLINDRICAL_SURFACE('',#16058,18.56595) ;
#1228=CYLINDRICAL_SURFACE('',#16059,18.56595) ;
#1229=CYLINDRICAL_SURFACE('',#16060,18.56595) ;
#1230=CYLINDRICAL_SURFACE('',#16061,18.56595) ;
#1231=CYLINDRICAL_SURFACE('',#16062,18.56595) ;
#1232=CYLINDRICAL_SURFACE('',#16063,18.56595) ;
#1233=CYLINDRICAL_SURFACE('',#16064,18.56595) ;
#1234=CYLINDRICAL_SURFACE('',#16065,18.56595) ;
#1235=CYLINDRICAL_SURFACE('',#16066,18.56595) ;
#1236=CYLINDRICAL_SURFACE('',#16067,18.56595) ;
#1237=CYLINDRICAL_SURFACE('',#16068,18.56595) ;
#1238=CYLINDRICAL_SURFACE('',#16069,18.56595) ;
#1239=CYLINDRICAL_SURFACE('',#16070,18.56595) ;
#1240=CYLINDRICAL_SURFACE('',#16072,20.33524) ;
#1241=CYLINDRICAL_SURFACE('',#16074,22.12975) ;
#1242=CYLINDRICAL_SURFACE('',#16076,19.425) ;
#1243=CYLINDRICAL_SURFACE('',#16084,13.2000000000001) ;
#1244=CYLINDRICAL_SURFACE('',#16089,17.5) ;
#1245=CYLINDRICAL_SURFACE('',#16095,19.9999999999999) ;
#1246=CYLINDRICAL_SURFACE('',#16103,22.5) ;
#1247=CYLINDRICAL_SURFACE('',#16111,33.5) ;
#1248=CYLINDRICAL_SURFACE('',#16130,33.5) ;
#1249=CYLINDRICAL_SURFACE('',#16139,33.5) ;
#1250=CYLINDRICAL_SURFACE('',#16140,33.5) ;
#1251=CYLINDRICAL_SURFACE('',#16141,33.5) ;
#1252=CYLINDRICAL_SURFACE('',#16146,5.00000000000251) ;
#1253=CYLINDRICAL_SURFACE('',#16149,5.00000000000251) ;
#1254=CYLINDRICAL_SURFACE('',#16152,20.065) ;
#1255=CYLINDRICAL_SURFACE('',#16156,23.) ;
#1256=CYLINDRICAL_SURFACE('',#16157,20.065) ;
#1257=CYLINDRICAL_SURFACE('',#16158,22.5) ;
#1258=CYLINDRICAL_SURFACE('',#16162,22.25) ;
#1259=CYLINDRICAL_SURFACE('',#16165,18.) ;
#1721=FACE_OUTER_BOUND('',#2688,.T.) ;
#1722=FACE_OUTER_BOUND('',#2689,.T.) ;
#1723=FACE_OUTER_BOUND('',#2690,.T.) ;
#1724=FACE_OUTER_BOUND('',#2691,.T.) ;
#1725=FACE_OUTER_BOUND('',#2692,.T.) ;
#1726=FACE_OUTER_BOUND('',#2693,.T.) ;
#1727=FACE_OUTER_BOUND('',#2694,.T.) ;
#1728=FACE_OUTER_BOUND('',#2695,.T.) ;
#1729=FACE_OUTER_BOUND('',#2696,.T.) ;
#1730=FACE_OUTER_BOUND('',#2697,.T.) ;
#1731=FACE_OUTER_BOUND('',#2698,.T.) ;
#1732=FACE_OUTER_BOUND('',#2699,.T.) ;
#1733=FACE_OUTER_BOUND('',#2700,.T.) ;
#1734=FACE_OUTER_BOUND('',#2701,.T.) ;
#1735=FACE_OUTER_BOUND('',#2702,.T.) ;
#1736=FACE_OUTER_BOUND('',#2703,.T.) ;
#1737=FACE_OUTER_BOUND('',#2704,.T.) ;
#1738=FACE_OUTER_BOUND('',#2705,.T.) ;
#1739=FACE_OUTER_BOUND('',#2706,.T.) ;
#1740=FACE_OUTER_BOUND('',#2707,.T.) ;
#1741=FACE_OUTER_BOUND('',#2708,.T.) ;
#1742=FACE_OUTER_BOUND('',#2709,.T.) ;
#1743=FACE_OUTER_BOUND('',#2710,.T.) ;
#1744=FACE_OUTER_BOUND('',#2711,.T.) ;
#1745=FACE_OUTER_BOUND('',#2712,.T.) ;
#1746=FACE_OUTER_BOUND('',#2713,.T.) ;
#1747=FACE_OUTER_BOUND('',#2714,.T.) ;
#1748=FACE_OUTER_BOUND('',#2715,.T.) ;
#1749=FACE_OUTER_BOUND('',#2716,.T.) ;
#1750=FACE_OUTER_BOUND('',#2717,.T.) ;
#1751=FACE_OUTER_BOUND('',#2718,.T.) ;
#1752=FACE_OUTER_BOUND('',#2719,.T.) ;
#1753=FACE_OUTER_BOUND('',#2720,.T.) ;
#1754=FACE_OUTER_BOUND('',#2721,.T.) ;
#1755=FACE_OUTER_BOUND('',#2722,.T.) ;
#1756=FACE_OUTER_BOUND('',#2723,.T.) ;
#1757=FACE_OUTER_BOUND('',#2724,.T.) ;
#1758=FACE_OUTER_BOUND('',#2725,.T.) ;
#1759=FACE_OUTER_BOUND('',#2726,.T.) ;
#1760=FACE_OUTER_BOUND('',#2727,.T.) ;
#1761=FACE_OUTER_BOUND('',#2728,.T.) ;
#1762=FACE_OUTER_BOUND('',#2729,.T.) ;
#1763=FACE_OUTER_BOUND('',#2730,.T.) ;
#1764=FACE_OUTER_BOUND('',#2731,.T.) ;
#1765=FACE_OUTER_BOUND('',#2732,.T.) ;
#1766=FACE_OUTER_BOUND('',#2734,.T.) ;
#1767=FACE_OUTER_BOUND('',#2735,.T.) ;
#1768=FACE_OUTER_BOUND('',#2736,.T.) ;
#1769=FACE_OUTER_BOUND('',#2737,.T.) ;
#1770=FACE_OUTER_BOUND('',#2738,.T.) ;
#1771=FACE_OUTER_BOUND('',#2740,.T.) ;
#1772=FACE_OUTER_BOUND('',#2742,.T.) ;
#1773=FACE_OUTER_BOUND('',#2743,.T.) ;
#1774=FACE_OUTER_BOUND('',#2744,.T.) ;
#1775=FACE_OUTER_BOUND('',#2746,.T.) ;
#1776=FACE_OUTER_BOUND('',#2747,.T.) ;
#1777=FACE_OUTER_BOUND('',#2748,.T.) ;
#1778=FACE_OUTER_BOUND('',#2749,.T.) ;
#1779=FACE_OUTER_BOUND('',#2750,.T.) ;
#1780=FACE_OUTER_BOUND('',#2752,.T.) ;
#1781=FACE_OUTER_BOUND('',#2753,.T.) ;
#1782=FACE_OUTER_BOUND('',#2754,.T.) ;
#1783=FACE_OUTER_BOUND('',#2756,.T.) ;
#1784=FACE_OUTER_BOUND('',#2757,.T.) ;
#1785=FACE_OUTER_BOUND('',#2761,.T.) ;
#1786=FACE_OUTER_BOUND('',#2763,.T.) ;
#1787=FACE_OUTER_BOUND('',#2764,.T.) ;
#1788=FACE_OUTER_BOUND('',#2766,.T.) ;
#1789=FACE_OUTER_BOUND('',#2767,.T.) ;
#1790=FACE_OUTER_BOUND('',#2768,.T.) ;
#1791=FACE_OUTER_BOUND('',#2769,.T.) ;
#1792=FACE_OUTER_BOUND('',#2770,.T.) ;
#1793=FACE_OUTER_BOUND('',#2771,.T.) ;
#1794=FACE_OUTER_BOUND('',#2772,.T.) ;
#1795=FACE_OUTER_BOUND('',#2773,.T.) ;
#1796=FACE_OUTER_BOUND('',#2774,.T.) ;
#1797=FACE_OUTER_BOUND('',#2776,.T.) ;
#1798=FACE_OUTER_BOUND('',#2777,.T.) ;
#1799=FACE_OUTER_BOUND('',#2778,.T.) ;
#1800=FACE_OUTER_BOUND('',#2780,.T.) ;
#1801=FACE_OUTER_BOUND('',#2781,.T.) ;
#1802=FACE_OUTER_BOUND('',#2782,.T.) ;
#1803=FACE_OUTER_BOUND('',#2783,.T.) ;
#1804=FACE_OUTER_BOUND('',#2784,.T.) ;
#1805=FACE_OUTER_BOUND('',#2785,.T.) ;
#1806=FACE_OUTER_BOUND('',#2786,.T.) ;
#1807=FACE_OUTER_BOUND('',#2788,.T.) ;
#1808=FACE_OUTER_BOUND('',#2789,.T.) ;
#1809=FACE_OUTER_BOUND('',#2790,.T.) ;
#1810=FACE_OUTER_BOUND('',#2791,.T.) ;
#1811=FACE_OUTER_BOUND('',#2793,.T.) ;
#1812=FACE_OUTER_BOUND('',#2794,.T.) ;
#1813=FACE_OUTER_BOUND('',#2796,.T.) ;
#1814=FACE_OUTER_BOUND('',#2797,.T.) ;
#2688=EDGE_LOOP('',(#10510,#10511,#10512,#10513)) ;
#2689=EDGE_LOOP('',(#10514,#10515,#10516,#10517)) ;
#2690=EDGE_LOOP('',(#10518,#10519,#10520,#10521)) ;
#2691=EDGE_LOOP('',(#10522,#10523,#10524,#10525)) ;
#2692=EDGE_LOOP('',(#10526,#10527,#10528,#10529)) ;
#2693=EDGE_LOOP('',(#10530,#10531,#10532,#10533)) ;
#2694=EDGE_LOOP('',(#10534,#10535,#10536,#10537)) ;
#2695=EDGE_LOOP('',(#10538,#10539,#10540,#10541)) ;
#2696=EDGE_LOOP('',(#10542,#10543,#10544,#10545)) ;
#2697=EDGE_LOOP('',(#10546,#10547,#10548,#10549)) ;
#2698=EDGE_LOOP('',(#10550,#10551,#10552,#10553)) ;
#2699=EDGE_LOOP('',(#10554,#10555,#10556,#10557)) ;
#2700=EDGE_LOOP('',(#10558,#10559,#10560,#10561)) ;
#2701=EDGE_LOOP('',(#10562,#10563,#10564,#10565)) ;
#2702=EDGE_LOOP('',(#10566,#10567,#10568,#10569)) ;
#2703=EDGE_LOOP('',(#10570,#10571,#10572,#10573)) ;
#2704=EDGE_LOOP('',(#10574,#10575,#10576,#10577)) ;
#2705=EDGE_LOOP('',(#10578,#10579,#10580,#10581)) ;
#2706=EDGE_LOOP('',(#10582,#10583,#10584,#10585)) ;
#2707=EDGE_LOOP('',(#10586,#10587,#10588,#10589,#10590)) ;
#2708=EDGE_LOOP('',(#10591,#10592,#10593,#10594)) ;
#2709=EDGE_LOOP('',(#10595,#10596,#10597,#10598)) ;
#2710=EDGE_LOOP('',(#10599,#10600,#10601,#10602)) ;
#2711=EDGE_LOOP('',(#10603,#10604,#10605,#10606)) ;
#2712=EDGE_LOOP('',(#10607,#10608,#10609,#10610)) ;
#2713=EDGE_LOOP('',(#10611,#10612,#10613,#10614)) ;
#2714=EDGE_LOOP('',(#10615,#10616,#10617,#10618)) ;
#2715=EDGE_LOOP('',(#10619,#10620,#10621,#10622)) ;
#2716=EDGE_LOOP('',(#10623,#10624,#10625,#10626)) ;
#2717=EDGE_LOOP('',(#10627,#10628,#10629,#10630,#10631)) ;
#2718=EDGE_LOOP('',(#10632,#10633,#10634,#10635)) ;
#2719=EDGE_LOOP('',(#10636,#10637,#10638,#10639)) ;
#2720=EDGE_LOOP('',(#10640,#10641,#10642,#10643)) ;
#2721=EDGE_LOOP('',(#10644,#10645,#10646,#10647)) ;
#2722=EDGE_LOOP('',(#10648,#10649,#10650,#10651,#10652,#10653)) ;
#2723=EDGE_LOOP('',(#10654,#10655,#10656,#10657)) ;
#2724=EDGE_LOOP('',(#10658,#10659,#10660,#10661,#10662)) ;
#2725=EDGE_LOOP('',(#10663,#10664,#10665,#10666)) ;
#2726=EDGE_LOOP('',(#10667,#10668,#10669,#10670)) ;
#2727=EDGE_LOOP('',(#10671,#10672,#10673,#10674)) ;
#2728=EDGE_LOOP('',(#10675,#10676,#10677,#10678)) ;
#2729=EDGE_LOOP('',(#10679,#10680,#10681)) ;
#2730=EDGE_LOOP('',(#10682,#10683,#10684,#10685)) ;
#2731=EDGE_LOOP('',(#10686,#10687,#10688,#10689,#10690)) ;
#2732=EDGE_LOOP('',(#10691)) ;
#2733=EDGE_LOOP('',(#10692)) ;
#2734=EDGE_LOOP('',(#10693,#10694,#10695,#10696,#10697)) ;
#2735=EDGE_LOOP('',(#10698,#10699,#10700,#10701,#10702)) ;
#2736=EDGE_LOOP('',(#10703,#10704,#10705,#10706,#10707)) ;
#2737=EDGE_LOOP('',(#10708,#10709,#10710,#10711,#10712)) ;
#2738=EDGE_LOOP('',(#10713,#10714,#10715,#10716,#10717)) ;
#2739=EDGE_LOOP('',(#10718,#10719,#10720,#10721)) ;
#2740=EDGE_LOOP('',(#10722)) ;
#2741=EDGE_LOOP('',(#10723)) ;
#2742=EDGE_LOOP('',(#10724,#10725,#10726,#10727,#10728)) ;
#2743=EDGE_LOOP('',(#10729,#10730,#10731,#10732,#10733)) ;
#2744=EDGE_LOOP('',(#10734)) ;
#2745=EDGE_LOOP('',(#10735)) ;
#2746=EDGE_LOOP('',(#10736,#10737,#10738,#10739,#10740,#10741)) ;
#2747=EDGE_LOOP('',(#10742,#10743,#10744,#10745,#10746,#10747)) ;
#2748=EDGE_LOOP('',(#10748,#10749,#10750,#10751,#10752)) ;
#2749=EDGE_LOOP('',(#10753,#10754,#10755,#10756,#10757)) ;
#2750=EDGE_LOOP('',(#10758)) ;
#2751=EDGE_LOOP('',(#10759)) ;
#2752=EDGE_LOOP('',(#10760,#10761,#10762,#10763,#10764)) ;
#2753=EDGE_LOOP('',(#10765,#10766,#10767,#10768,#10769)) ;
#2754=EDGE_LOOP('',(#10770,#10771,#10772,#10773)) ;
#2755=EDGE_LOOP('',(#10774)) ;
#2756=EDGE_LOOP('',(#10775,#10776,#10777,#10778,#10779)) ;
#2757=EDGE_LOOP('',(#10780,#10781,#10782,#10783,#10784,#10785)) ;
#2758=EDGE_LOOP('',(#10786)) ;
#2759=EDGE_LOOP('',(#10787)) ;
#2760=EDGE_LOOP('',(#10788)) ;
#2761=EDGE_LOOP('',(#10789)) ;
#2762=EDGE_LOOP('',(#10790)) ;
#2763=EDGE_LOOP('',(#10791,#10792,#10793,#10794,#10795)) ;
#2764=EDGE_LOOP('',(#10796)) ;
#2765=EDGE_LOOP('',(#10797)) ;
#2766=EDGE_LOOP('',(#10798,#10799,#10800,#10801)) ;
#2767=EDGE_LOOP('',(#10802)) ;
#2768=EDGE_LOOP('',(#10803,#10804,#10805,#10806)) ;
#2769=EDGE_LOOP('',(#10807)) ;
#2770=EDGE_LOOP('',(#10808,#10809,#10810,#10811)) ;
#2771=EDGE_LOOP('',(#10812)) ;
#2772=EDGE_LOOP('',(#10813,#10814,#10815,#10816,#10817,#10818,#10819,#10820,
#10821,#10822,#10823,#10824,#10825,#10826,#10827,#10828,#10829,#10830,#10831,
#10832,#10833,#10834,#10835,#10836,#10837,#10838,#10839,#10840,#10841,#10842,
#10843,#10844)) ;
#2773=EDGE_LOOP('',(#10845,#10846,#10847,#10848,#10849,#10850,#10851,#10852,
#10853,#10854,#10855,#10856,#10857,#10858,#10859,#10860,#10861,#10862,#10863,
#10864,#10865,#10866,#10867,#10868,#10869,#10870,#10871,#10872,#10873,#10874,
#10875,#10876,#10877,#10878)) ;
#2774=EDGE_LOOP('',(#10879,#10880,#10881,#10882,#10883)) ;
#2775=EDGE_LOOP('',(#10884)) ;
#2776=EDGE_LOOP('',(#10885,#10886,#10887,#10888,#10889,#10890,#10891,#10892,
#10893,#10894,#10895,#10896,#10897,#10898,#10899,#10900,#10901)) ;
#2777=EDGE_LOOP('',(#10902,#10903,#10904,#10905,#10906,#10907,#10908,#10909,
#10910,#10911,#10912,#10913,#10914,#10915,#10916,#10917,#10918)) ;
#2778=EDGE_LOOP('',(#10919,#10920,#10921,#10922,#10923,#10924)) ;
#2779=EDGE_LOOP('',(#10925)) ;
#2780=EDGE_LOOP('',(#10926,#10927,#10928,#10929)) ;
#2781=EDGE_LOOP('',(#10930,#10931,#10932,#10933)) ;
#2782=EDGE_LOOP('',(#10934,#10935,#10936,#10937)) ;
#2783=EDGE_LOOP('',(#10938,#10939,#10940,#10941)) ;
#2784=EDGE_LOOP('',(#10942,#10943,#10944,#10945)) ;
#2785=EDGE_LOOP('',(#10946,#10947,#10948,#10949)) ;
#2786=EDGE_LOOP('',(#10950)) ;
#2787=EDGE_LOOP('',(#10951)) ;
#2788=EDGE_LOOP('',(#10952,#10953,#10954,#10955)) ;
#2789=EDGE_LOOP('',(#10956,#10957,#10958,#10959)) ;
#2790=EDGE_LOOP('',(#10960,#10961,#10962,#10963)) ;
#2791=EDGE_LOOP('',(#10964)) ;
#2792=EDGE_LOOP('',(#10965)) ;
#2793=EDGE_LOOP('',(#10966,#10967,#10968,#10969)) ;
#2794=EDGE_LOOP('',(#10970)) ;
#2795=EDGE_LOOP('',(#10971)) ;
#2796=EDGE_LOOP('',(#10972,#10973,#10974,#10975)) ;
#2797=EDGE_LOOP('',(#10976,#10977,#10978,#10979,#10980)) ;
#2798=EDGE_LOOP('',(#10981)) ;
#3642=CIRCLE('',#16027,19.425) ;
#3643=CIRCLE('',#16041,22.12975) ;
#3644=CIRCLE('',#16048,22.12975) ;
#3645=CIRCLE('',#16050,20.33524) ;
#3646=CIRCLE('',#16057,18.56595) ;
#3647=CIRCLE('',#16071,18.56595) ;
#3648=CIRCLE('',#16073,20.33524) ;
#3649=CIRCLE('',#16075,22.12975) ;
#3650=CIRCLE('',#16077,19.425) ;
#3651=CIRCLE('',#16079,13.2000000000001) ;
#3652=CIRCLE('',#16080,13.4500000000001) ;
#3653=CIRCLE('',#16081,13.2000000000001) ;
#3654=CIRCLE('',#16083,17.25) ;
#3655=CIRCLE('',#16085,13.2) ;
#3656=CIRCLE('',#16087,17.5) ;
#3657=CIRCLE('',#16088,17.5) ;
#3658=CIRCLE('',#16090,17.5) ;
#3659=CIRCLE('',#16092,19.9999999999999) ;
#3660=CIRCLE('',#16093,19.7499999999997) ;
#3661=CIRCLE('',#16094,19.9999999999999) ;
#3662=CIRCLE('',#16096,20.) ;
#3663=CIRCLE('',#16098,18.) ;
#3664=CIRCLE('',#16100,22.5) ;
#3665=CIRCLE('',#16101,22.25) ;
#3666=CIRCLE('',#16102,22.5) ;
#3667=CIRCLE('',#16104,22.5) ;
#3668=CIRCLE('',#16107,33.5) ;
#3669=CIRCLE('',#16108,33.2649649327684) ;
#3670=CIRCLE('',#16109,33.2649649327684) ;
#3671=CIRCLE('',#16110,33.5) ;
#3672=CIRCLE('',#16112,33.5) ;
#3673=CIRCLE('',#16113,33.5) ;
#3674=CIRCLE('',#16115,20.065) ;
#3675=CIRCLE('',#16117,33.25) ;
#3676=CIRCLE('',#16119,23.) ;
#3677=CIRCLE('',#16121,15.6275202784794) ;
#3678=CIRCLE('',#16122,15.8837) ;
#3679=CIRCLE('',#16123,15.6275202784794) ;
#3680=CIRCLE('',#16127,33.5) ;
#3681=CIRCLE('',#16128,33.25) ;
#3682=CIRCLE('',#16129,33.5) ;
#3683=CIRCLE('',#16131,33.5) ;
#3684=CIRCLE('',#16132,33.5) ;
#3685=CIRCLE('',#16134,22.5) ;
#3686=CIRCLE('',#16136,33.25) ;
#3687=CIRCLE('',#16138,20.065) ;
#3688=CIRCLE('',#16144,20.065) ;
#3689=CIRCLE('',#16147,5.00000000000251) ;
#3690=CIRCLE('',#16150,5.00000000000251) ;
#3691=CIRCLE('',#16153,20.065) ;
#3692=CIRCLE('',#16155,23.) ;
#3693=CIRCLE('',#16159,22.5) ;
#3694=CIRCLE('',#16161,22.25) ;
#3695=CIRCLE('',#16163,22.25) ;
#3696=CIRCLE('',#16166,18.) ;
#4876=LINE('',#23802,#5532) ;
#4877=LINE('',#24013,#5533) ;
#4878=LINE('',#24711,#5534) ;
#4879=LINE('',#25409,#5535) ;
#4880=LINE('',#26239,#5536) ;
#4881=LINE('',#27007,#5537) ;
#4882=LINE('',#27737,#5538) ;
#4883=LINE('',#28443,#5539) ;
#4884=LINE('',#29111,#5540) ;
#4885=LINE('',#29813,#5541) ;
#4886=LINE('',#30599,#5542) ;
#4887=LINE('',#31377,#5543) ;
#4888=LINE('',#32055,#5544) ;
#4889=LINE('',#32747,#5545) ;
#4890=LINE('',#32836,#5546) ;
#4891=LINE('',#33146,#5547) ;
#4892=LINE('',#33462,#5548) ;
#4893=LINE('',#33776,#5549) ;
#4894=LINE('',#34460,#5550) ;
#4895=LINE('',#35156,#5551) ;
#4896=LINE('',#35839,#5552) ;
#4897=LINE('',#36016,#5553) ;
#4898=LINE('',#36316,#5554) ;
#4899=LINE('',#36616,#5555) ;
#4900=LINE('',#36906,#5556) ;
#4901=LINE('',#37206,#5557) ;
#4902=LINE('',#37512,#5558) ;
#4903=LINE('',#38595,#5559) ;
#4904=LINE('',#38599,#5560) ;
#4905=LINE('',#39387,#5561) ;
#4906=LINE('',#40182,#5562) ;
#4907=LINE('',#40872,#5563) ;
#4908=LINE('',#41620,#5564) ;
#4909=LINE('',#42336,#5565) ;
#4910=LINE('',#43028,#5566) ;
#4911=LINE('',#43888,#5567) ;
#4912=LINE('',#44572,#5568) ;
#4913=LINE('',#45321,#5569) ;
#4914=LINE('',#46025,#5570) ;
#4915=LINE('',#48143,#5571) ;
#4916=LINE('',#48152,#5572) ;
#4917=LINE('',#48157,#5573) ;
#4918=LINE('',#48161,#5574) ;
#4919=LINE('',#48168,#5575) ;
#4920=LINE('',#48173,#5576) ;
#4921=LINE('',#48177,#5577) ;
#4922=LINE('',#48198,#5578) ;
#4923=LINE('',#48225,#5579) ;
#4924=LINE('',#48230,#5580) ;
#4925=LINE('',#48238,#5581) ;
#4926=LINE('',#48245,#5582) ;
#4927=LINE('',#48251,#5583) ;
#4928=LINE('',#48255,#5584) ;
#4929=LINE('',#48265,#5585) ;
#4930=LINE('',#48269,#5586) ;
#4931=LINE('',#48420,#5587) ;
#4932=LINE('',#48425,#5588) ;
#4933=LINE('',#48539,#5589) ;
#4934=LINE('',#51824,#5590) ;
#4935=LINE('',#51826,#5591) ;
#4936=LINE('',#51827,#5592) ;
#4937=LINE('',#51831,#5593) ;
#4938=LINE('',#51834,#5594) ;
#4939=LINE('',#51835,#5595) ;
#4940=LINE('',#51842,#5596) ;
#4941=LINE('',#51847,#5597) ;
#4942=LINE('',#51849,#5598) ;
#4943=LINE('',#51853,#5599) ;
#4944=LINE('',#51860,#5600) ;
#4945=LINE('',#51865,#5601) ;
#5532=VECTOR('',#18792,19.425) ;
#5533=VECTOR('',#18797,19.425) ;
#5534=VECTOR('',#18800,19.425) ;
#5535=VECTOR('',#18803,19.425) ;
#5536=VECTOR('',#18806,19.425) ;
#5537=VECTOR('',#18809,19.425) ;
#5538=VECTOR('',#18812,19.425) ;
#5539=VECTOR('',#18815,19.425) ;
#5540=VECTOR('',#18818,19.425) ;
#5541=VECTOR('',#18821,19.425) ;
#5542=VECTOR('',#18824,19.425) ;
#5543=VECTOR('',#18827,19.425) ;
#5544=VECTOR('',#18830,19.425) ;
#5545=VECTOR('',#18833,22.12975) ;
#5546=VECTOR('',#18838,22.12975) ;
#5547=VECTOR('',#18841,22.12975) ;
#5548=VECTOR('',#18844,22.12975) ;
#5549=VECTOR('',#18847,22.12975) ;
#5550=VECTOR('',#18850,22.12975) ;
#5551=VECTOR('',#18853,22.12975) ;
#5552=VECTOR('',#18858,20.33524) ;
#5553=VECTOR('',#18863,20.33524) ;
#5554=VECTOR('',#18866,20.33524) ;
#5555=VECTOR('',#18869,20.33524) ;
#5556=VECTOR('',#18872,20.33524) ;
#5557=VECTOR('',#18875,20.33524) ;
#5558=VECTOR('',#18878,18.56595) ;
#5559=VECTOR('',#18883,18.56595) ;
#5560=VECTOR('',#18886,18.56595) ;
#5561=VECTOR('',#18889,18.56595) ;
#5562=VECTOR('',#18892,18.56595) ;
#5563=VECTOR('',#18895,18.56595) ;
#5564=VECTOR('',#18898,18.56595) ;
#5565=VECTOR('',#18901,18.56595) ;
#5566=VECTOR('',#18904,18.56595) ;
#5567=VECTOR('',#18907,18.56595) ;
#5568=VECTOR('',#18910,18.56595) ;
#5569=VECTOR('',#18913,18.56595) ;
#5570=VECTOR('',#18916,18.56595) ;
#5571=VECTOR('',#18937,13.3250000000001) ;
#5572=VECTOR('',#18950,13.2000000000001) ;
#5573=VECTOR('',#18955,17.375) ;
#5574=VECTOR('',#18960,17.5) ;
#5575=VECTOR('',#18967,19.8749999999998) ;
#5576=VECTOR('',#18974,19.9999999999999) ;
#5577=VECTOR('',#18977,10.) ;
#5578=VECTOR('',#18978,10.) ;
#5579=VECTOR('',#18987,22.375) ;
#5580=VECTOR('',#18994,22.5) ;
#5581=VECTOR('',#19003,33.3824824663842) ;
#5582=VECTOR('',#19012,33.5) ;
#5583=VECTOR('',#19019,26.7825) ;
#5584=VECTOR('',#19024,33.375) ;
#5585=VECTOR('',#19035,15.7556101392397) ;
#5586=VECTOR('',#19042,14.41685) ;
#5587=VECTOR('',#19049,33.375) ;
#5588=VECTOR('',#19056,33.5) ;
#5589=VECTOR('',#19067,33.375) ;
#5590=VECTOR('',#19088,10.) ;
#5591=VECTOR('',#19089,10.) ;
#5592=VECTOR('',#19090,10.) ;
#5593=VECTOR('',#19095,10.) ;
#5594=VECTOR('',#19098,10.) ;
#5595=VECTOR('',#19099,10.) ;
#5596=VECTOR('',#19110,20.065) ;
#5597=VECTOR('',#19117,23.) ;
#5598=VECTOR('',#19120,20.065) ;
#5599=VECTOR('',#19125,22.5) ;
#5600=VECTOR('',#19134,22.25) ;
#5601=VECTOR('',#19141,18.) ;
#6252=VERTEX_POINT('',#23800) ;
#6253=VERTEX_POINT('',#23801) ;
#6254=VERTEX_POINT('',#23803) ;
#6255=VERTEX_POINT('',#23936) ;
#6256=VERTEX_POINT('',#24011) ;
#6257=VERTEX_POINT('',#24012) ;
#6258=VERTEX_POINT('',#24709) ;
#6259=VERTEX_POINT('',#24710) ;
#6260=VERTEX_POINT('',#25407) ;
#6261=VERTEX_POINT('',#25408) ;
#6262=VERTEX_POINT('',#26237) ;
#6263=VERTEX_POINT('',#26238) ;
#6264=VERTEX_POINT('',#27005) ;
#6265=VERTEX_POINT('',#27006) ;
#6266=VERTEX_POINT('',#27735) ;
#6267=VERTEX_POINT('',#27736) ;
#6268=VERTEX_POINT('',#28441) ;
#6269=VERTEX_POINT('',#28442) ;
#6270=VERTEX_POINT('',#29109) ;
#6271=VERTEX_POINT('',#29110) ;
#6272=VERTEX_POINT('',#29811) ;
#6273=VERTEX_POINT('',#29812) ;
#6274=VERTEX_POINT('',#30597) ;
#6275=VERTEX_POINT('',#30598) ;
#6276=VERTEX_POINT('',#31375) ;
#6277=VERTEX_POINT('',#31376) ;
#6278=VERTEX_POINT('',#32053) ;
#6279=VERTEX_POINT('',#32054) ;
#6280=VERTEX_POINT('',#32745) ;
#6281=VERTEX_POINT('',#32746) ;
#6282=VERTEX_POINT('',#32748) ;
#6283=VERTEX_POINT('',#32799) ;
#6284=VERTEX_POINT('',#32834) ;
#6285=VERTEX_POINT('',#32835) ;
#6286=VERTEX_POINT('',#33144) ;
#6287=VERTEX_POINT('',#33145) ;
#6288=VERTEX_POINT('',#33460) ;
#6289=VERTEX_POINT('',#33461) ;
#6290=VERTEX_POINT('',#33774) ;
#6291=VERTEX_POINT('',#33775) ;
#6292=VERTEX_POINT('',#34458) ;
#6293=VERTEX_POINT('',#34459) ;
#6294=VERTEX_POINT('',#35154) ;
#6295=VERTEX_POINT('',#35155) ;
#6296=VERTEX_POINT('',#35157) ;
#6297=VERTEX_POINT('',#35837) ;
#6298=VERTEX_POINT('',#35838) ;
#6299=VERTEX_POINT('',#35840) ;
#6300=VERTEX_POINT('',#35939) ;
#6301=VERTEX_POINT('',#36014) ;
#6302=VERTEX_POINT('',#36015) ;
#6303=VERTEX_POINT('',#36314) ;
#6304=VERTEX_POINT('',#36315) ;
#6305=VERTEX_POINT('',#36614) ;
#6306=VERTEX_POINT('',#36615) ;
#6307=VERTEX_POINT('',#36904) ;
#6308=VERTEX_POINT('',#36905) ;
#6309=VERTEX_POINT('',#37204) ;
#6310=VERTEX_POINT('',#37205) ;
#6311=VERTEX_POINT('',#37510) ;
#6312=VERTEX_POINT('',#37511) ;
#6313=VERTEX_POINT('',#37513) ;
#6314=VERTEX_POINT('',#37754) ;
#6315=VERTEX_POINT('',#37905) ;
#6316=VERTEX_POINT('',#38254) ;
#6317=VERTEX_POINT('',#38597) ;
#6318=VERTEX_POINT('',#38598) ;
#6319=VERTEX_POINT('',#39385) ;
#6320=VERTEX_POINT('',#39386) ;
#6321=VERTEX_POINT('',#39780) ;
#6322=VERTEX_POINT('',#40180) ;
#6323=VERTEX_POINT('',#40181) ;
#6324=VERTEX_POINT('',#40870) ;
#6325=VERTEX_POINT('',#40871) ;
#6326=VERTEX_POINT('',#41618) ;
#6327=VERTEX_POINT('',#41619) ;
#6328=VERTEX_POINT('',#42334) ;
#6329=VERTEX_POINT('',#42335) ;
#6330=VERTEX_POINT('',#43026) ;
#6331=VERTEX_POINT('',#43027) ;
#6332=VERTEX_POINT('',#43029) ;
#6333=VERTEX_POINT('',#43410) ;
#6334=VERTEX_POINT('',#43886) ;
#6335=VERTEX_POINT('',#43887) ;
#6336=VERTEX_POINT('',#44570) ;
#6337=VERTEX_POINT('',#44571) ;
#6338=VERTEX_POINT('',#44919) ;
#6339=VERTEX_POINT('',#45319) ;
#6340=VERTEX_POINT('',#45320) ;
#6341=VERTEX_POINT('',#46023) ;
#6342=VERTEX_POINT('',#46024) ;
#6343=VERTEX_POINT('',#46707) ;
#6344=VERTEX_POINT('',#47048) ;
#6345=VERTEX_POINT('',#47253) ;
#6346=VERTEX_POINT('',#47366) ;
#6347=VERTEX_POINT('',#47459) ;
#6348=VERTEX_POINT('',#47502) ;
#6349=VERTEX_POINT('',#47877) ;
#6350=VERTEX_POINT('',#48139) ;
#6351=VERTEX_POINT('',#48140) ;
#6352=VERTEX_POINT('',#48142) ;
#6353=VERTEX_POINT('',#48147) ;
#6354=VERTEX_POINT('',#48150) ;
#6355=VERTEX_POINT('',#48154) ;
#6356=VERTEX_POINT('',#48155) ;
#6357=VERTEX_POINT('',#48160) ;
#6358=VERTEX_POINT('',#48164) ;
#6359=VERTEX_POINT('',#48165) ;
#6360=VERTEX_POINT('',#48167) ;
#6361=VERTEX_POINT('',#48172) ;
#6362=VERTEX_POINT('',#48175) ;
#6363=VERTEX_POINT('',#48176) ;
#6364=VERTEX_POINT('',#48178) ;
#6365=VERTEX_POINT('',#48197) ;
#6366=VERTEX_POINT('',#48218) ;
#6367=VERTEX_POINT('',#48221) ;
#6368=VERTEX_POINT('',#48222) ;
#6369=VERTEX_POINT('',#48224) ;
#6370=VERTEX_POINT('',#48229) ;
#6371=VERTEX_POINT('',#48234) ;
#6372=VERTEX_POINT('',#48235) ;
#6373=VERTEX_POINT('',#48237) ;
#6374=VERTEX_POINT('',#48239) ;
#6375=VERTEX_POINT('',#48244) ;
#6376=VERTEX_POINT('',#48246) ;
#6377=VERTEX_POINT('',#48250) ;
#6378=VERTEX_POINT('',#48254) ;
#6379=VERTEX_POINT('',#48258) ;
#6380=VERTEX_POINT('',#48261) ;
#6381=VERTEX_POINT('',#48262) ;
#6382=VERTEX_POINT('',#48264) ;
#6383=VERTEX_POINT('',#48416) ;
#6384=VERTEX_POINT('',#48417) ;
#6385=VERTEX_POINT('',#48419) ;
#6386=VERTEX_POINT('',#48424) ;
#6387=VERTEX_POINT('',#48426) ;
#6388=VERTEX_POINT('',#48429) ;
#6389=VERTEX_POINT('',#48464) ;
#6390=VERTEX_POINT('',#48499) ;
#6391=VERTEX_POINT('',#48535) ;
#6392=VERTEX_POINT('',#48538) ;
#6393=VERTEX_POINT('',#48542) ;
#6394=VERTEX_POINT('',#48612) ;
#6395=VERTEX_POINT('',#48739) ;
#6396=VERTEX_POINT('',#48866) ;
#6397=VERTEX_POINT('',#49753) ;
#6398=VERTEX_POINT('',#50589) ;
#6399=VERTEX_POINT('',#51684) ;
#6400=VERTEX_POINT('',#51820) ;
#6401=VERTEX_POINT('',#51823) ;
#6402=VERTEX_POINT('',#51825) ;
#6403=VERTEX_POINT('',#51829) ;
#6404=VERTEX_POINT('',#51833) ;
#6405=VERTEX_POINT('',#51840) ;
#6406=VERTEX_POINT('',#51844) ;
#6407=VERTEX_POINT('',#51851) ;
#6408=VERTEX_POINT('',#51855) ;
#6409=VERTEX_POINT('',#51858) ;
#6410=VERTEX_POINT('',#51863) ;
#7809=EDGE_CURVE('',#6252,#6253,#4876,.T.) ;
#7810=EDGE_CURVE('',#6252,#6254,#222,.F.) ;
#7811=EDGE_CURVE('',#6254,#6255,#3642,.T.) ;
#7812=EDGE_CURVE('',#6255,#6253,#223,.T.) ;
#7813=EDGE_CURVE('',#6256,#6257,#4877,.T.) ;
#7814=EDGE_CURVE('',#6256,#6252,#224,.F.) ;
#7815=EDGE_CURVE('',#6253,#6257,#225,.T.) ;
#7816=EDGE_CURVE('',#6258,#6259,#4878,.T.) ;
#7817=EDGE_CURVE('',#6258,#6256,#226,.T.) ;
#7818=EDGE_CURVE('',#6257,#6259,#227,.T.) ;
#7819=EDGE_CURVE('',#6260,#6261,#4879,.T.) ;
#7820=EDGE_CURVE('',#6260,#6258,#228,.T.) ;
#7821=EDGE_CURVE('',#6259,#6261,#229,.T.) ;
#7822=EDGE_CURVE('',#6262,#6263,#4880,.T.) ;
#7823=EDGE_CURVE('',#6262,#6260,#230,.T.) ;
#7824=EDGE_CURVE('',#6261,#6263,#231,.T.) ;
#7825=EDGE_CURVE('',#6264,#6265,#4881,.T.) ;
#7826=EDGE_CURVE('',#6264,#6262,#232,.T.) ;
#7827=EDGE_CURVE('',#6263,#6265,#233,.T.) ;
#7828=EDGE_CURVE('',#6266,#6267,#4882,.T.) ;
#7829=EDGE_CURVE('',#6266,#6264,#234,.T.) ;
#7830=EDGE_CURVE('',#6265,#6267,#235,.T.) ;
#7831=EDGE_CURVE('',#6268,#6269,#4883,.T.) ;
#7832=EDGE_CURVE('',#6268,#6266,#236,.T.) ;
#7833=EDGE_CURVE('',#6267,#6269,#237,.T.) ;
#7834=EDGE_CURVE('',#6270,#6271,#4884,.T.) ;
#7835=EDGE_CURVE('',#6270,#6268,#238,.T.) ;
#7836=EDGE_CURVE('',#6269,#6271,#239,.T.) ;
#7837=EDGE_CURVE('',#6272,#6273,#4885,.T.) ;
#7838=EDGE_CURVE('',#6272,#6270,#240,.T.) ;
#7839=EDGE_CURVE('',#6271,#6273,#241,.T.) ;
#7840=EDGE_CURVE('',#6274,#6275,#4886,.T.) ;
#7841=EDGE_CURVE('',#6274,#6272,#242,.T.) ;
#7842=EDGE_CURVE('',#6273,#6275,#243,.T.) ;
#7843=EDGE_CURVE('',#6276,#6277,#4887,.T.) ;
#7844=EDGE_CURVE('',#6276,#6274,#244,.T.) ;
#7845=EDGE_CURVE('',#6275,#6277,#245,.T.) ;
#7846=EDGE_CURVE('',#6278,#6279,#4888,.T.) ;
#7847=EDGE_CURVE('',#6278,#6276,#246,.T.) ;
#7848=EDGE_CURVE('',#6277,#6279,#247,.T.) ;
#7849=EDGE_CURVE('',#6280,#6281,#4889,.T.) ;
#7850=EDGE_CURVE('',#6280,#6282,#248,.T.) ;
#7851=EDGE_CURVE('',#6282,#6283,#3643,.T.) ;
#7852=EDGE_CURVE('',#6283,#6281,#249,.T.) ;
#7853=EDGE_CURVE('',#6284,#6285,#4890,.T.) ;
#7854=EDGE_CURVE('',#6284,#6280,#250,.T.) ;
#7855=EDGE_CURVE('',#6281,#6285,#251,.T.) ;
#7856=EDGE_CURVE('',#6286,#6287,#4891,.T.) ;
#7857=EDGE_CURVE('',#6286,#6284,#252,.T.) ;
#7858=EDGE_CURVE('',#6285,#6287,#253,.T.) ;
#7859=EDGE_CURVE('',#6288,#6289,#4892,.T.) ;
#7860=EDGE_CURVE('',#6288,#6286,#254,.T.) ;
#7861=EDGE_CURVE('',#6287,#6289,#255,.T.) ;
#7862=EDGE_CURVE('',#6290,#6291,#4893,.T.) ;
#7863=EDGE_CURVE('',#6290,#6288,#256,.T.) ;
#7864=EDGE_CURVE('',#6289,#6291,#257,.T.) ;
#7865=EDGE_CURVE('',#6292,#6293,#4894,.T.) ;
#7866=EDGE_CURVE('',#6292,#6290,#258,.T.) ;
#7867=EDGE_CURVE('',#6291,#6293,#259,.T.) ;
#7868=EDGE_CURVE('',#6294,#6295,#4895,.T.) ;
#7869=EDGE_CURVE('',#6296,#6294,#3644,.F.) ;
#7870=EDGE_CURVE('',#6296,#6292,#260,.T.) ;
#7871=EDGE_CURVE('',#6293,#6295,#261,.T.) ;
#7872=EDGE_CURVE('',#6297,#6298,#4896,.T.) ;
#7873=EDGE_CURVE('',#6299,#6297,#262,.F.) ;
#7874=EDGE_CURVE('',#6300,#6299,#3645,.T.) ;
#7875=EDGE_CURVE('',#6300,#6298,#263,.T.) ;
#7876=EDGE_CURVE('',#6301,#6302,#4897,.T.) ;
#7877=EDGE_CURVE('',#6297,#6301,#264,.F.) ;
#7878=EDGE_CURVE('',#6298,#6302,#265,.T.) ;
#7879=EDGE_CURVE('',#6303,#6304,#4898,.T.) ;
#7880=EDGE_CURVE('',#6301,#6303,#266,.F.) ;
#7881=EDGE_CURVE('',#6302,#6304,#267,.T.) ;
#7882=EDGE_CURVE('',#6305,#6306,#4899,.T.) ;
#7883=EDGE_CURVE('',#6303,#6305,#268,.F.) ;
#7884=EDGE_CURVE('',#6304,#6306,#269,.T.) ;
#7885=EDGE_CURVE('',#6307,#6308,#4900,.T.) ;
#7886=EDGE_CURVE('',#6305,#6307,#270,.F.) ;
#7887=EDGE_CURVE('',#6306,#6308,#271,.T.) ;
#7888=EDGE_CURVE('',#6309,#6310,#4901,.T.) ;
#7889=EDGE_CURVE('',#6307,#6309,#272,.F.) ;
#7890=EDGE_CURVE('',#6308,#6310,#273,.T.) ;
#7891=EDGE_CURVE('',#6311,#6312,#4902,.T.) ;
#7892=EDGE_CURVE('',#6313,#6311,#274,.F.) ;
#7893=EDGE_CURVE('',#6314,#6313,#3646,.T.) ;
#7894=EDGE_CURVE('',#6314,#6312,#275,.T.) ;
#7895=EDGE_CURVE('',#6311,#6315,#276,.F.) ;
#7896=EDGE_CURVE('',#6312,#6316,#277,.T.) ;
#7897=EDGE_CURVE('',#6315,#6316,#4903,.T.) ;
#7898=EDGE_CURVE('',#6317,#6318,#4904,.T.) ;
#7899=EDGE_CURVE('',#6315,#6317,#278,.F.) ;
#7900=EDGE_CURVE('',#6316,#6318,#279,.T.) ;
#7901=EDGE_CURVE('',#6319,#6320,#4905,.T.) ;
#7902=EDGE_CURVE('',#6317,#6319,#280,.F.) ;
#7903=EDGE_CURVE('',#6318,#6321,#281,.T.) ;
#7904=EDGE_CURVE('',#6321,#6320,#282,.T.) ;
#7905=EDGE_CURVE('',#6322,#6323,#4906,.T.) ;
#7906=EDGE_CURVE('',#6319,#6322,#283,.F.) ;
#7907=EDGE_CURVE('',#6320,#6323,#284,.T.) ;
#7908=EDGE_CURVE('',#6324,#6325,#4907,.T.) ;
#7909=EDGE_CURVE('',#6322,#6324,#285,.F.) ;
#7910=EDGE_CURVE('',#6323,#6325,#286,.T.) ;
#7911=EDGE_CURVE('',#6326,#6327,#4908,.T.) ;
#7912=EDGE_CURVE('',#6324,#6326,#287,.F.) ;
#7913=EDGE_CURVE('',#6325,#6327,#288,.T.) ;
#7914=EDGE_CURVE('',#6328,#6329,#4909,.T.) ;
#7915=EDGE_CURVE('',#6326,#6328,#289,.F.) ;
#7916=EDGE_CURVE('',#6327,#6329,#290,.T.) ;
#7917=EDGE_CURVE('',#6330,#6331,#4910,.T.) ;
#7918=EDGE_CURVE('',#6332,#6330,#291,.F.) ;
#7919=EDGE_CURVE('',#6328,#6332,#292,.F.) ;
#7920=EDGE_CURVE('',#6329,#6333,#293,.T.) ;
#7921=EDGE_CURVE('',#6333,#6331,#294,.T.) ;
#7922=EDGE_CURVE('',#6334,#6335,#4911,.T.) ;
#7923=EDGE_CURVE('',#6330,#6334,#295,.F.) ;
#7924=EDGE_CURVE('',#6331,#6335,#296,.T.) ;
#7925=EDGE_CURVE('',#6336,#6337,#4912,.T.) ;
#7926=EDGE_CURVE('',#6334,#6336,#297,.F.) ;
#7927=EDGE_CURVE('',#6335,#6338,#298,.T.) ;
#7928=EDGE_CURVE('',#6338,#6337,#299,.T.) ;
#7929=EDGE_CURVE('',#6339,#6340,#4913,.T.) ;
#7930=EDGE_CURVE('',#6336,#6339,#300,.F.) ;
#7931=EDGE_CURVE('',#6337,#6340,#301,.T.) ;
#7932=EDGE_CURVE('',#6341,#6342,#4914,.T.) ;
#7933=EDGE_CURVE('',#6339,#6341,#302,.F.) ;
#7934=EDGE_CURVE('',#6340,#6342,#303,.T.) ;
#7935=EDGE_CURVE('',#6342,#6343,#304,.T.) ;
#7936=EDGE_CURVE('',#6344,#6343,#3647,.T.) ;
#7937=EDGE_CURVE('',#6341,#6344,#305,.F.) ;
#7938=EDGE_CURVE('',#6310,#6345,#306,.T.) ;
#7939=EDGE_CURVE('',#6346,#6345,#3648,.T.) ;
#7940=EDGE_CURVE('',#6309,#6346,#307,.F.) ;
#7941=EDGE_CURVE('',#6295,#6347,#308,.T.) ;
#7942=EDGE_CURVE('',#6294,#6347,#3649,.F.) ;
#7943=EDGE_CURVE('',#6279,#6348,#309,.T.) ;
#7944=EDGE_CURVE('',#6349,#6348,#3650,.F.) ;
#7945=EDGE_CURVE('',#6349,#6278,#310,.T.) ;
#7946=EDGE_CURVE('',#6350,#6351,#3651,.T.) ;
#7947=EDGE_CURVE('',#6351,#6352,#4915,.T.) ;
#7948=EDGE_CURVE('',#6352,#6352,#3652,.T.) ;
#7949=EDGE_CURVE('',#6351,#6350,#3653,.T.) ;
#7950=EDGE_CURVE('',#6353,#6353,#3654,.T.) ;
#7951=EDGE_CURVE('',#6354,#6354,#3655,.T.) ;
#7952=EDGE_CURVE('',#6354,#6350,#4916,.T.) ;
#7953=EDGE_CURVE('',#6355,#6356,#3656,.T.) ;
#7954=EDGE_CURVE('',#6356,#6353,#4917,.T.) ;
#7955=EDGE_CURVE('',#6356,#6355,#3657,.T.) ;
#7956=EDGE_CURVE('',#6355,#6357,#4918,.T.) ;
#7957=EDGE_CURVE('',#6357,#6357,#3658,.T.) ;
#7958=EDGE_CURVE('',#6358,#6359,#3659,.T.) ;
#7959=EDGE_CURVE('',#6359,#6360,#4919,.T.) ;
#7960=EDGE_CURVE('',#6360,#6360,#3660,.T.) ;
#7961=EDGE_CURVE('',#6359,#6358,#3661,.T.) ;
#7962=EDGE_CURVE('',#6358,#6361,#4920,.T.) ;
#7963=EDGE_CURVE('',#6361,#6361,#3662,.T.) ;
#7964=EDGE_CURVE('',#6362,#6363,#4921,.T.) ;
#7965=EDGE_CURVE('',#6363,#6364,#311,.T.) ;
#7966=EDGE_CURVE('',#6364,#6365,#4922,.T.) ;
#7967=EDGE_CURVE('',#6365,#6362,#312,.T.) ;
#7968=EDGE_CURVE('',#6366,#6366,#3663,.T.) ;
#7969=EDGE_CURVE('',#6367,#6368,#3664,.T.) ;
#7970=EDGE_CURVE('',#6368,#6369,#4923,.T.) ;
#7971=EDGE_CURVE('',#6369,#6369,#3665,.T.) ;
#7972=EDGE_CURVE('',#6368,#6367,#3666,.T.) ;
#7973=EDGE_CURVE('',#6367,#6370,#4924,.T.) ;
#7974=EDGE_CURVE('',#6370,#6370,#3667,.T.) ;
#7975=EDGE_CURVE('',#6371,#6372,#3668,.T.) ;
#7976=EDGE_CURVE('',#6372,#6373,#4925,.T.) ;
#7977=EDGE_CURVE('',#6373,#6374,#3669,.T.) ;
#7978=EDGE_CURVE('',#6374,#6373,#3670,.T.) ;
#7979=EDGE_CURVE('',#6372,#6371,#3671,.T.) ;
#7980=EDGE_CURVE('',#6371,#6375,#4926,.T.) ;
#7981=EDGE_CURVE('',#6376,#6375,#3672,.T.) ;
#7982=EDGE_CURVE('',#6375,#6376,#3673,.T.) ;
#7983=EDGE_CURVE('',#6374,#6377,#4927,.T.) ;
#7984=EDGE_CURVE('',#6377,#6377,#3674,.T.) ;
#7985=EDGE_CURVE('',#6376,#6378,#4928,.T.) ;
#7986=EDGE_CURVE('',#6378,#6378,#3675,.T.) ;
#7987=EDGE_CURVE('',#6379,#6379,#3676,.T.) ;
#7988=EDGE_CURVE('',#6380,#6381,#3677,.T.) ;
#7989=EDGE_CURVE('',#6381,#6382,#4929,.T.) ;
#7990=EDGE_CURVE('',#6382,#6382,#3678,.T.) ;
#7991=EDGE_CURVE('',#6381,#6380,#3679,.T.) ;
#7992=EDGE_CURVE('',#6354,#6380,#4930,.T.) ;
#7993=EDGE_CURVE('',#6299,#6283,#313,.F.) ;
#7994=EDGE_CURVE('',#6282,#6300,#314,.T.) ;
#7995=EDGE_CURVE('',#6383,#6384,#3680,.T.) ;
#7996=EDGE_CURVE('',#6384,#6385,#4931,.T.) ;
#7997=EDGE_CURVE('',#6385,#6385,#3681,.T.) ;
#7998=EDGE_CURVE('',#6384,#6383,#3682,.T.) ;
#7999=EDGE_CURVE('',#6383,#6386,#4932,.T.) ;
#8000=EDGE_CURVE('',#6387,#6386,#3683,.T.) ;
#8001=EDGE_CURVE('',#6386,#6387,#3684,.T.) ;
#8002=EDGE_CURVE('',#6388,#6388,#315,.T.) ;
#8003=EDGE_CURVE('',#6389,#6389,#316,.T.) ;
#8004=EDGE_CURVE('',#6390,#6390,#317,.T.) ;
#8005=EDGE_CURVE('',#6391,#6391,#3685,.T.) ;
#8006=EDGE_CURVE('',#6387,#6392,#4933,.T.) ;
#8007=EDGE_CURVE('',#6392,#6392,#3686,.T.) ;
#8008=EDGE_CURVE('',#6393,#6393,#3687,.T.) ;
#8009=EDGE_CURVE('',#6388,#6394,#318,.T.) ;
#8010=EDGE_CURVE('',#6394,#6394,#319,.T.) ;
#8011=EDGE_CURVE('',#6389,#6395,#320,.T.) ;
#8012=EDGE_CURVE('',#6395,#6395,#321,.T.) ;
#8013=EDGE_CURVE('',#6390,#6396,#322,.T.) ;
#8014=EDGE_CURVE('',#6396,#6396,#323,.T.) ;
#8015=EDGE_CURVE('',#6348,#6344,#324,.T.) ;
#8016=EDGE_CURVE('',#6397,#6255,#325,.T.) ;
#8017=EDGE_CURVE('',#6397,#6313,#326,.T.) ;
#8018=EDGE_CURVE('',#6398,#6349,#327,.T.) ;
#8019=EDGE_CURVE('',#6343,#6398,#328,.T.) ;
#8020=EDGE_CURVE('',#6254,#6314,#329,.T.) ;
#8021=EDGE_CURVE('',#6347,#6346,#330,.T.) ;
#8022=EDGE_CURVE('',#6399,#6296,#331,.T.) ;
#8023=EDGE_CURVE('',#6345,#6399,#332,.T.) ;
#8024=EDGE_CURVE('',#6400,#6400,#3688,.T.) ;
#8025=EDGE_CURVE('',#6401,#6362,#4934,.T.) ;
#8026=EDGE_CURVE('',#6402,#6401,#4935,.T.) ;
#8027=EDGE_CURVE('',#6402,#6363,#4936,.T.) ;
#8028=EDGE_CURVE('',#6403,#6402,#3689,.T.) ;
#8029=EDGE_CURVE('',#6403,#6364,#4937,.T.) ;
#8030=EDGE_CURVE('',#6404,#6403,#4938,.T.) ;
#8031=EDGE_CURVE('',#6404,#6365,#4939,.T.) ;
#8032=EDGE_CURVE('',#6401,#6404,#3690,.T.) ;
#8033=EDGE_CURVE('',#6405,#6405,#3691,.T.) ;
#8034=EDGE_CURVE('',#6405,#6400,#4940,.T.) ;
#8035=EDGE_CURVE('',#6406,#6406,#3692,.T.) ;
#8036=EDGE_CURVE('',#6379,#6406,#4941,.T.) ;
#8037=EDGE_CURVE('',#6393,#6377,#4942,.T.) ;
#8038=EDGE_CURVE('',#6407,#6407,#3693,.T.) ;
#8039=EDGE_CURVE('',#6407,#6391,#4943,.T.) ;
#8040=EDGE_CURVE('',#6408,#6408,#3694,.T.) ;
#8041=EDGE_CURVE('',#6409,#6409,#3695,.T.) ;
#8042=EDGE_CURVE('',#6409,#6408,#4944,.T.) ;
#8043=EDGE_CURVE('',#6410,#6410,#3696,.T.) ;
#8044=EDGE_CURVE('',#6410,#6366,#4945,.T.) ;
#10510=ORIENTED_EDGE('',*,*,#7809,.F.) ;
#10511=ORIENTED_EDGE('',*,*,#7810,.T.) ;
#10512=ORIENTED_EDGE('',*,*,#7811,.T.) ;
#10513=ORIENTED_EDGE('',*,*,#7812,.T.) ;
#10514=ORIENTED_EDGE('',*,*,#7813,.F.) ;
#10515=ORIENTED_EDGE('',*,*,#7814,.T.) ;
#10516=ORIENTED_EDGE('',*,*,#7809,.T.) ;
#10517=ORIENTED_EDGE('',*,*,#7815,.T.) ;
#10518=ORIENTED_EDGE('',*,*,#7816,.F.) ;
#10519=ORIENTED_EDGE('',*,*,#7817,.T.) ;
#10520=ORIENTED_EDGE('',*,*,#7813,.T.) ;
#10521=ORIENTED_EDGE('',*,*,#7818,.T.) ;
#10522=ORIENTED_EDGE('',*,*,#7819,.F.) ;
#10523=ORIENTED_EDGE('',*,*,#7820,.T.) ;
#10524=ORIENTED_EDGE('',*,*,#7816,.T.) ;
#10525=ORIENTED_EDGE('',*,*,#7821,.T.) ;
#10526=ORIENTED_EDGE('',*,*,#7822,.F.) ;
#10527=ORIENTED_EDGE('',*,*,#7823,.T.) ;
#10528=ORIENTED_EDGE('',*,*,#7819,.T.) ;
#10529=ORIENTED_EDGE('',*,*,#7824,.T.) ;
#10530=ORIENTED_EDGE('',*,*,#7825,.F.) ;
#10531=ORIENTED_EDGE('',*,*,#7826,.T.) ;
#10532=ORIENTED_EDGE('',*,*,#7822,.T.) ;
#10533=ORIENTED_EDGE('',*,*,#7827,.T.) ;
#10534=ORIENTED_EDGE('',*,*,#7828,.F.) ;
#10535=ORIENTED_EDGE('',*,*,#7829,.T.) ;
#10536=ORIENTED_EDGE('',*,*,#7825,.T.) ;
#10537=ORIENTED_EDGE('',*,*,#7830,.T.) ;
#10538=ORIENTED_EDGE('',*,*,#7831,.F.) ;
#10539=ORIENTED_EDGE('',*,*,#7832,.T.) ;
#10540=ORIENTED_EDGE('',*,*,#7828,.T.) ;
#10541=ORIENTED_EDGE('',*,*,#7833,.T.) ;
#10542=ORIENTED_EDGE('',*,*,#7834,.F.) ;
#10543=ORIENTED_EDGE('',*,*,#7835,.T.) ;
#10544=ORIENTED_EDGE('',*,*,#7831,.T.) ;
#10545=ORIENTED_EDGE('',*,*,#7836,.T.) ;
#10546=ORIENTED_EDGE('',*,*,#7837,.F.) ;
#10547=ORIENTED_EDGE('',*,*,#7838,.T.) ;
#10548=ORIENTED_EDGE('',*,*,#7834,.T.) ;
#10549=ORIENTED_EDGE('',*,*,#7839,.T.) ;
#10550=ORIENTED_EDGE('',*,*,#7840,.F.) ;
#10551=ORIENTED_EDGE('',*,*,#7841,.T.) ;
#10552=ORIENTED_EDGE('',*,*,#7837,.T.) ;
#10553=ORIENTED_EDGE('',*,*,#7842,.T.) ;
#10554=ORIENTED_EDGE('',*,*,#7843,.F.) ;
#10555=ORIENTED_EDGE('',*,*,#7844,.T.) ;
#10556=ORIENTED_EDGE('',*,*,#7840,.T.) ;
#10557=ORIENTED_EDGE('',*,*,#7845,.T.) ;
#10558=ORIENTED_EDGE('',*,*,#7846,.F.) ;
#10559=ORIENTED_EDGE('',*,*,#7847,.T.) ;
#10560=ORIENTED_EDGE('',*,*,#7843,.T.) ;
#10561=ORIENTED_EDGE('',*,*,#7848,.T.) ;
#10562=ORIENTED_EDGE('',*,*,#7849,.F.) ;
#10563=ORIENTED_EDGE('',*,*,#7850,.T.) ;
#10564=ORIENTED_EDGE('',*,*,#7851,.T.) ;
#10565=ORIENTED_EDGE('',*,*,#7852,.T.) ;
#10566=ORIENTED_EDGE('',*,*,#7853,.F.) ;
#10567=ORIENTED_EDGE('',*,*,#7854,.T.) ;
#10568=ORIENTED_EDGE('',*,*,#7849,.T.) ;
#10569=ORIENTED_EDGE('',*,*,#7855,.T.) ;
#10570=ORIENTED_EDGE('',*,*,#7856,.F.) ;
#10571=ORIENTED_EDGE('',*,*,#7857,.T.) ;
#10572=ORIENTED_EDGE('',*,*,#7853,.T.) ;
#10573=ORIENTED_EDGE('',*,*,#7858,.T.) ;
#10574=ORIENTED_EDGE('',*,*,#7859,.F.) ;
#10575=ORIENTED_EDGE('',*,*,#7860,.T.) ;
#10576=ORIENTED_EDGE('',*,*,#7856,.T.) ;
#10577=ORIENTED_EDGE('',*,*,#7861,.T.) ;
#10578=ORIENTED_EDGE('',*,*,#7862,.F.) ;
#10579=ORIENTED_EDGE('',*,*,#7863,.T.) ;
#10580=ORIENTED_EDGE('',*,*,#7859,.T.) ;
#10581=ORIENTED_EDGE('',*,*,#7864,.T.) ;
#10582=ORIENTED_EDGE('',*,*,#7865,.F.) ;
#10583=ORIENTED_EDGE('',*,*,#7866,.T.) ;
#10584=ORIENTED_EDGE('',*,*,#7862,.T.) ;
#10585=ORIENTED_EDGE('',*,*,#7867,.T.) ;
#10586=ORIENTED_EDGE('',*,*,#7868,.F.) ;
#10587=ORIENTED_EDGE('',*,*,#7869,.F.) ;
#10588=ORIENTED_EDGE('',*,*,#7870,.T.) ;
#10589=ORIENTED_EDGE('',*,*,#7865,.T.) ;
#10590=ORIENTED_EDGE('',*,*,#7871,.T.) ;
#10591=ORIENTED_EDGE('',*,*,#7872,.F.) ;
#10592=ORIENTED_EDGE('',*,*,#7873,.F.) ;
#10593=ORIENTED_EDGE('',*,*,#7874,.F.) ;
#10594=ORIENTED_EDGE('',*,*,#7875,.T.) ;
#10595=ORIENTED_EDGE('',*,*,#7876,.F.) ;
#10596=ORIENTED_EDGE('',*,*,#7877,.F.) ;
#10597=ORIENTED_EDGE('',*,*,#7872,.T.) ;
#10598=ORIENTED_EDGE('',*,*,#7878,.T.) ;
#10599=ORIENTED_EDGE('',*,*,#7879,.F.) ;
#10600=ORIENTED_EDGE('',*,*,#7880,.F.) ;
#10601=ORIENTED_EDGE('',*,*,#7876,.T.) ;
#10602=ORIENTED_EDGE('',*,*,#7881,.T.) ;
#10603=ORIENTED_EDGE('',*,*,#7882,.F.) ;
#10604=ORIENTED_EDGE('',*,*,#7883,.F.) ;
#10605=ORIENTED_EDGE('',*,*,#7879,.T.) ;
#10606=ORIENTED_EDGE('',*,*,#7884,.T.) ;
#10607=ORIENTED_EDGE('',*,*,#7885,.F.) ;
#10608=ORIENTED_EDGE('',*,*,#7886,.F.) ;
#10609=ORIENTED_EDGE('',*,*,#7882,.T.) ;
#10610=ORIENTED_EDGE('',*,*,#7887,.T.) ;
#10611=ORIENTED_EDGE('',*,*,#7888,.F.) ;
#10612=ORIENTED_EDGE('',*,*,#7889,.F.) ;
#10613=ORIENTED_EDGE('',*,*,#7885,.T.) ;
#10614=ORIENTED_EDGE('',*,*,#7890,.T.) ;
#10615=ORIENTED_EDGE('',*,*,#7891,.F.) ;
#10616=ORIENTED_EDGE('',*,*,#7892,.F.) ;
#10617=ORIENTED_EDGE('',*,*,#7893,.F.) ;
#10618=ORIENTED_EDGE('',*,*,#7894,.T.) ;
#10619=ORIENTED_EDGE('',*,*,#7895,.F.) ;
#10620=ORIENTED_EDGE('',*,*,#7891,.T.) ;
#10621=ORIENTED_EDGE('',*,*,#7896,.T.) ;
#10622=ORIENTED_EDGE('',*,*,#7897,.F.) ;
#10623=ORIENTED_EDGE('',*,*,#7898,.F.) ;
#10624=ORIENTED_EDGE('',*,*,#7899,.F.) ;
#10625=ORIENTED_EDGE('',*,*,#7897,.T.) ;
#10626=ORIENTED_EDGE('',*,*,#7900,.T.) ;
#10627=ORIENTED_EDGE('',*,*,#7901,.F.) ;
#10628=ORIENTED_EDGE('',*,*,#7902,.F.) ;
#10629=ORIENTED_EDGE('',*,*,#7898,.T.) ;
#10630=ORIENTED_EDGE('',*,*,#7903,.T.) ;
#10631=ORIENTED_EDGE('',*,*,#7904,.T.) ;
#10632=ORIENTED_EDGE('',*,*,#7905,.F.) ;
#10633=ORIENTED_EDGE('',*,*,#7906,.F.) ;
#10634=ORIENTED_EDGE('',*,*,#7901,.T.) ;
#10635=ORIENTED_EDGE('',*,*,#7907,.T.) ;
#10636=ORIENTED_EDGE('',*,*,#7908,.F.) ;
#10637=ORIENTED_EDGE('',*,*,#7909,.F.) ;
#10638=ORIENTED_EDGE('',*,*,#7905,.T.) ;
#10639=ORIENTED_EDGE('',*,*,#7910,.T.) ;
#10640=ORIENTED_EDGE('',*,*,#7911,.F.) ;
#10641=ORIENTED_EDGE('',*,*,#7912,.F.) ;
#10642=ORIENTED_EDGE('',*,*,#7908,.T.) ;
#10643=ORIENTED_EDGE('',*,*,#7913,.T.) ;
#10644=ORIENTED_EDGE('',*,*,#7914,.F.) ;
#10645=ORIENTED_EDGE('',*,*,#7915,.F.) ;
#10646=ORIENTED_EDGE('',*,*,#7911,.T.) ;
#10647=ORIENTED_EDGE('',*,*,#7916,.T.) ;
#10648=ORIENTED_EDGE('',*,*,#7917,.F.) ;
#10649=ORIENTED_EDGE('',*,*,#7918,.F.) ;
#10650=ORIENTED_EDGE('',*,*,#7919,.F.) ;
#10651=ORIENTED_EDGE('',*,*,#7914,.T.) ;
#10652=ORIENTED_EDGE('',*,*,#7920,.T.) ;
#10653=ORIENTED_EDGE('',*,*,#7921,.T.) ;
#10654=ORIENTED_EDGE('',*,*,#7922,.F.) ;
#10655=ORIENTED_EDGE('',*,*,#7923,.F.) ;
#10656=ORIENTED_EDGE('',*,*,#7917,.T.) ;
#10657=ORIENTED_EDGE('',*,*,#7924,.T.) ;
#10658=ORIENTED_EDGE('',*,*,#7925,.F.) ;
#10659=ORIENTED_EDGE('',*,*,#7926,.F.) ;
#10660=ORIENTED_EDGE('',*,*,#7922,.T.) ;
#10661=ORIENTED_EDGE('',*,*,#7927,.T.) ;
#10662=ORIENTED_EDGE('',*,*,#7928,.T.) ;
#10663=ORIENTED_EDGE('',*,*,#7929,.F.) ;
#10664=ORIENTED_EDGE('',*,*,#7930,.F.) ;
#10665=ORIENTED_EDGE('',*,*,#7925,.T.) ;
#10666=ORIENTED_EDGE('',*,*,#7931,.T.) ;
#10667=ORIENTED_EDGE('',*,*,#7932,.F.) ;
#10668=ORIENTED_EDGE('',*,*,#7933,.F.) ;
#10669=ORIENTED_EDGE('',*,*,#7929,.T.) ;
#10670=ORIENTED_EDGE('',*,*,#7934,.T.) ;
#10671=ORIENTED_EDGE('',*,*,#7932,.T.) ;
#10672=ORIENTED_EDGE('',*,*,#7935,.T.) ;
#10673=ORIENTED_EDGE('',*,*,#7936,.F.) ;
#10674=ORIENTED_EDGE('',*,*,#7937,.F.) ;
#10675=ORIENTED_EDGE('',*,*,#7888,.T.) ;
#10676=ORIENTED_EDGE('',*,*,#7938,.T.) ;
#10677=ORIENTED_EDGE('',*,*,#7939,.F.) ;
#10678=ORIENTED_EDGE('',*,*,#7940,.F.) ;
#10679=ORIENTED_EDGE('',*,*,#7868,.T.) ;
#10680=ORIENTED_EDGE('',*,*,#7941,.T.) ;
#10681=ORIENTED_EDGE('',*,*,#7942,.F.) ;
#10682=ORIENTED_EDGE('',*,*,#7846,.T.) ;
#10683=ORIENTED_EDGE('',*,*,#7943,.T.) ;
#10684=ORIENTED_EDGE('',*,*,#7944,.F.) ;
#10685=ORIENTED_EDGE('',*,*,#7945,.T.) ;
#10686=ORIENTED_EDGE('',*,*,#7946,.T.) ;
#10687=ORIENTED_EDGE('',*,*,#7947,.T.) ;
#10688=ORIENTED_EDGE('',*,*,#7948,.T.) ;
#10689=ORIENTED_EDGE('',*,*,#7947,.F.) ;
#10690=ORIENTED_EDGE('',*,*,#7949,.T.) ;
#10691=ORIENTED_EDGE('',*,*,#7950,.F.) ;
#10692=ORIENTED_EDGE('',*,*,#7948,.F.) ;
#10693=ORIENTED_EDGE('',*,*,#7951,.F.) ;
#10694=ORIENTED_EDGE('',*,*,#7952,.T.) ;
#10695=ORIENTED_EDGE('',*,*,#7949,.F.) ;
#10696=ORIENTED_EDGE('',*,*,#7946,.F.) ;
#10697=ORIENTED_EDGE('',*,*,#7952,.F.) ;
#10698=ORIENTED_EDGE('',*,*,#7953,.T.) ;
#10699=ORIENTED_EDGE('',*,*,#7954,.T.) ;
#10700=ORIENTED_EDGE('',*,*,#7950,.T.) ;
#10701=ORIENTED_EDGE('',*,*,#7954,.F.) ;
#10702=ORIENTED_EDGE('',*,*,#7955,.T.) ;
#10703=ORIENTED_EDGE('',*,*,#7953,.F.) ;
#10704=ORIENTED_EDGE('',*,*,#7956,.T.) ;
#10705=ORIENTED_EDGE('',*,*,#7957,.T.) ;
#10706=ORIENTED_EDGE('',*,*,#7956,.F.) ;
#10707=ORIENTED_EDGE('',*,*,#7955,.F.) ;
#10708=ORIENTED_EDGE('',*,*,#7958,.T.) ;
#10709=ORIENTED_EDGE('',*,*,#7959,.T.) ;
#10710=ORIENTED_EDGE('',*,*,#7960,.T.) ;
#10711=ORIENTED_EDGE('',*,*,#7959,.F.) ;
#10712=ORIENTED_EDGE('',*,*,#7961,.T.) ;
#10713=ORIENTED_EDGE('',*,*,#7958,.F.) ;
#10714=ORIENTED_EDGE('',*,*,#7962,.T.) ;
#10715=ORIENTED_EDGE('',*,*,#7963,.T.) ;
#10716=ORIENTED_EDGE('',*,*,#7962,.F.) ;
#10717=ORIENTED_EDGE('',*,*,#7961,.F.) ;
#10718=ORIENTED_EDGE('',*,*,#7964,.T.) ;
#10719=ORIENTED_EDGE('',*,*,#7965,.T.) ;
#10720=ORIENTED_EDGE('',*,*,#7966,.T.) ;
#10721=ORIENTED_EDGE('',*,*,#7967,.T.) ;
#10722=ORIENTED_EDGE('',*,*,#7960,.F.) ;
#10723=ORIENTED_EDGE('',*,*,#7968,.F.) ;
#10724=ORIENTED_EDGE('',*,*,#7969,.T.) ;
#10725=ORIENTED_EDGE('',*,*,#7970,.T.) ;
#10726=ORIENTED_EDGE('',*,*,#7971,.T.) ;
#10727=ORIENTED_EDGE('',*,*,#7970,.F.) ;
#10728=ORIENTED_EDGE('',*,*,#7972,.T.) ;
#10729=ORIENTED_EDGE('',*,*,#7969,.F.) ;
#10730=ORIENTED_EDGE('',*,*,#7973,.T.) ;
#10731=ORIENTED_EDGE('',*,*,#7974,.T.) ;
#10732=ORIENTED_EDGE('',*,*,#7973,.F.) ;
#10733=ORIENTED_EDGE('',*,*,#7972,.F.) ;
#10734=ORIENTED_EDGE('',*,*,#7971,.F.) ;
#10735=ORIENTED_EDGE('',*,*,#7963,.F.) ;
#10736=ORIENTED_EDGE('',*,*,#7975,.T.) ;
#10737=ORIENTED_EDGE('',*,*,#7976,.T.) ;
#10738=ORIENTED_EDGE('',*,*,#7977,.T.) ;
#10739=ORIENTED_EDGE('',*,*,#7978,.T.) ;
#10740=ORIENTED_EDGE('',*,*,#7976,.F.) ;
#10741=ORIENTED_EDGE('',*,*,#7979,.T.) ;
#10742=ORIENTED_EDGE('',*,*,#7975,.F.) ;
#10743=ORIENTED_EDGE('',*,*,#7980,.T.) ;
#10744=ORIENTED_EDGE('',*,*,#7981,.F.) ;
#10745=ORIENTED_EDGE('',*,*,#7982,.F.) ;
#10746=ORIENTED_EDGE('',*,*,#7980,.F.) ;
#10747=ORIENTED_EDGE('',*,*,#7979,.F.) ;
#10748=ORIENTED_EDGE('',*,*,#7978,.F.) ;
#10749=ORIENTED_EDGE('',*,*,#7983,.T.) ;
#10750=ORIENTED_EDGE('',*,*,#7984,.F.) ;
#10751=ORIENTED_EDGE('',*,*,#7983,.F.) ;
#10752=ORIENTED_EDGE('',*,*,#7977,.F.) ;
#10753=ORIENTED_EDGE('',*,*,#7981,.T.) ;
#10754=ORIENTED_EDGE('',*,*,#7982,.T.) ;
#10755=ORIENTED_EDGE('',*,*,#7985,.T.) ;
#10756=ORIENTED_EDGE('',*,*,#7986,.T.) ;
#10757=ORIENTED_EDGE('',*,*,#7985,.F.) ;
#10758=ORIENTED_EDGE('',*,*,#7986,.F.) ;
#10759=ORIENTED_EDGE('',*,*,#7987,.T.) ;
#10760=ORIENTED_EDGE('',*,*,#7988,.T.) ;
#10761=ORIENTED_EDGE('',*,*,#7989,.T.) ;
#10762=ORIENTED_EDGE('',*,*,#7990,.T.) ;
#10763=ORIENTED_EDGE('',*,*,#7989,.F.) ;
#10764=ORIENTED_EDGE('',*,*,#7991,.T.) ;
#10765=ORIENTED_EDGE('',*,*,#7951,.T.) ;
#10766=ORIENTED_EDGE('',*,*,#7992,.T.) ;
#10767=ORIENTED_EDGE('',*,*,#7991,.F.) ;
#10768=ORIENTED_EDGE('',*,*,#7988,.F.) ;
#10769=ORIENTED_EDGE('',*,*,#7992,.F.) ;
#10770=ORIENTED_EDGE('',*,*,#7993,.T.) ;
#10771=ORIENTED_EDGE('',*,*,#7851,.F.) ;
#10772=ORIENTED_EDGE('',*,*,#7994,.T.) ;
#10773=ORIENTED_EDGE('',*,*,#7874,.T.) ;
#10774=ORIENTED_EDGE('',*,*,#7990,.F.) ;
#10775=ORIENTED_EDGE('',*,*,#7995,.T.) ;
#10776=ORIENTED_EDGE('',*,*,#7996,.T.) ;
#10777=ORIENTED_EDGE('',*,*,#7997,.T.) ;
#10778=ORIENTED_EDGE('',*,*,#7996,.F.) ;
#10779=ORIENTED_EDGE('',*,*,#7998,.T.) ;
#10780=ORIENTED_EDGE('',*,*,#7995,.F.) ;
#10781=ORIENTED_EDGE('',*,*,#7999,.T.) ;
#10782=ORIENTED_EDGE('',*,*,#8000,.F.) ;
#10783=ORIENTED_EDGE('',*,*,#8001,.F.) ;
#10784=ORIENTED_EDGE('',*,*,#7999,.F.) ;
#10785=ORIENTED_EDGE('',*,*,#7998,.F.) ;
#10786=ORIENTED_EDGE('',*,*,#8002,.T.) ;
#10787=ORIENTED_EDGE('',*,*,#8003,.T.) ;
#10788=ORIENTED_EDGE('',*,*,#8004,.T.) ;
#10789=ORIENTED_EDGE('',*,*,#7997,.F.) ;
#10790=ORIENTED_EDGE('',*,*,#8005,.F.) ;
#10791=ORIENTED_EDGE('',*,*,#8000,.T.) ;
#10792=ORIENTED_EDGE('',*,*,#8001,.T.) ;
#10793=ORIENTED_EDGE('',*,*,#8006,.T.) ;
#10794=ORIENTED_EDGE('',*,*,#8007,.T.) ;
#10795=ORIENTED_EDGE('',*,*,#8006,.F.) ;
#10796=ORIENTED_EDGE('',*,*,#8007,.F.) ;
#10797=ORIENTED_EDGE('',*,*,#8008,.T.) ;
#10798=ORIENTED_EDGE('',*,*,#8002,.F.) ;
#10799=ORIENTED_EDGE('',*,*,#8009,.T.) ;
#10800=ORIENTED_EDGE('',*,*,#8010,.T.) ;
#10801=ORIENTED_EDGE('',*,*,#8009,.F.) ;
#10802=ORIENTED_EDGE('',*,*,#8010,.F.) ;
#10803=ORIENTED_EDGE('',*,*,#8003,.F.) ;
#10804=ORIENTED_EDGE('',*,*,#8011,.T.) ;
#10805=ORIENTED_EDGE('',*,*,#8012,.T.) ;
#10806=ORIENTED_EDGE('',*,*,#8011,.F.) ;
#10807=ORIENTED_EDGE('',*,*,#8012,.F.) ;
#10808=ORIENTED_EDGE('',*,*,#8004,.F.) ;
#10809=ORIENTED_EDGE('',*,*,#8013,.T.) ;
#10810=ORIENTED_EDGE('',*,*,#8014,.T.) ;
#10811=ORIENTED_EDGE('',*,*,#8013,.F.) ;
#10812=ORIENTED_EDGE('',*,*,#8014,.F.) ;
#10813=ORIENTED_EDGE('',*,*,#7899,.T.) ;
#10814=ORIENTED_EDGE('',*,*,#7902,.T.) ;
#10815=ORIENTED_EDGE('',*,*,#7906,.T.) ;
#10816=ORIENTED_EDGE('',*,*,#7909,.T.) ;
#10817=ORIENTED_EDGE('',*,*,#7912,.T.) ;
#10818=ORIENTED_EDGE('',*,*,#7915,.T.) ;
#10819=ORIENTED_EDGE('',*,*,#7919,.T.) ;
#10820=ORIENTED_EDGE('',*,*,#7918,.T.) ;
#10821=ORIENTED_EDGE('',*,*,#7923,.T.) ;
#10822=ORIENTED_EDGE('',*,*,#7926,.T.) ;
#10823=ORIENTED_EDGE('',*,*,#7930,.T.) ;
#10824=ORIENTED_EDGE('',*,*,#7933,.T.) ;
#10825=ORIENTED_EDGE('',*,*,#7937,.T.) ;
#10826=ORIENTED_EDGE('',*,*,#8015,.F.) ;
#10827=ORIENTED_EDGE('',*,*,#7943,.F.) ;
#10828=ORIENTED_EDGE('',*,*,#7848,.F.) ;
#10829=ORIENTED_EDGE('',*,*,#7845,.F.) ;
#10830=ORIENTED_EDGE('',*,*,#7842,.F.) ;
#10831=ORIENTED_EDGE('',*,*,#7839,.F.) ;
#10832=ORIENTED_EDGE('',*,*,#7836,.F.) ;
#10833=ORIENTED_EDGE('',*,*,#7833,.F.) ;
#10834=ORIENTED_EDGE('',*,*,#7830,.F.) ;
#10835=ORIENTED_EDGE('',*,*,#7827,.F.) ;
#10836=ORIENTED_EDGE('',*,*,#7824,.F.) ;
#10837=ORIENTED_EDGE('',*,*,#7821,.F.) ;
#10838=ORIENTED_EDGE('',*,*,#7818,.F.) ;
#10839=ORIENTED_EDGE('',*,*,#7815,.F.) ;
#10840=ORIENTED_EDGE('',*,*,#7812,.F.) ;
#10841=ORIENTED_EDGE('',*,*,#8016,.F.) ;
#10842=ORIENTED_EDGE('',*,*,#8017,.T.) ;
#10843=ORIENTED_EDGE('',*,*,#7892,.T.) ;
#10844=ORIENTED_EDGE('',*,*,#7895,.T.) ;
#10845=ORIENTED_EDGE('',*,*,#8018,.F.) ;
#10846=ORIENTED_EDGE('',*,*,#8019,.F.) ;
#10847=ORIENTED_EDGE('',*,*,#7935,.F.) ;
#10848=ORIENTED_EDGE('',*,*,#7934,.F.) ;
#10849=ORIENTED_EDGE('',*,*,#7931,.F.) ;
#10850=ORIENTED_EDGE('',*,*,#7928,.F.) ;
#10851=ORIENTED_EDGE('',*,*,#7927,.F.) ;
#10852=ORIENTED_EDGE('',*,*,#7924,.F.) ;
#10853=ORIENTED_EDGE('',*,*,#7921,.F.) ;
#10854=ORIENTED_EDGE('',*,*,#7920,.F.) ;
#10855=ORIENTED_EDGE('',*,*,#7916,.F.) ;
#10856=ORIENTED_EDGE('',*,*,#7913,.F.) ;
#10857=ORIENTED_EDGE('',*,*,#7910,.F.) ;
#10858=ORIENTED_EDGE('',*,*,#7907,.F.) ;
#10859=ORIENTED_EDGE('',*,*,#7904,.F.) ;
#10860=ORIENTED_EDGE('',*,*,#7903,.F.) ;
#10861=ORIENTED_EDGE('',*,*,#7900,.F.) ;
#10862=ORIENTED_EDGE('',*,*,#7896,.F.) ;
#10863=ORIENTED_EDGE('',*,*,#7894,.F.) ;
#10864=ORIENTED_EDGE('',*,*,#8020,.F.) ;
#10865=ORIENTED_EDGE('',*,*,#7810,.F.) ;
#10866=ORIENTED_EDGE('',*,*,#7814,.F.) ;
#10867=ORIENTED_EDGE('',*,*,#7817,.F.) ;
#10868=ORIENTED_EDGE('',*,*,#7820,.F.) ;
#10869=ORIENTED_EDGE('',*,*,#7823,.F.) ;
#10870=ORIENTED_EDGE('',*,*,#7826,.F.) ;
#10871=ORIENTED_EDGE('',*,*,#7829,.F.) ;
#10872=ORIENTED_EDGE('',*,*,#7832,.F.) ;
#10873=ORIENTED_EDGE('',*,*,#7835,.F.) ;
#10874=ORIENTED_EDGE('',*,*,#7838,.F.) ;
#10875=ORIENTED_EDGE('',*,*,#7841,.F.) ;
#10876=ORIENTED_EDGE('',*,*,#7844,.F.) ;
#10877=ORIENTED_EDGE('',*,*,#7847,.F.) ;
#10878=ORIENTED_EDGE('',*,*,#7945,.F.) ;
#10879=ORIENTED_EDGE('',*,*,#8015,.T.) ;
#10880=ORIENTED_EDGE('',*,*,#7936,.T.) ;
#10881=ORIENTED_EDGE('',*,*,#8019,.T.) ;
#10882=ORIENTED_EDGE('',*,*,#8018,.T.) ;
#10883=ORIENTED_EDGE('',*,*,#7944,.T.) ;
#10884=ORIENTED_EDGE('',*,*,#7957,.F.) ;
#10885=ORIENTED_EDGE('',*,*,#8021,.F.) ;
#10886=ORIENTED_EDGE('',*,*,#7941,.F.) ;
#10887=ORIENTED_EDGE('',*,*,#7871,.F.) ;
#10888=ORIENTED_EDGE('',*,*,#7867,.F.) ;
#10889=ORIENTED_EDGE('',*,*,#7864,.F.) ;
#10890=ORIENTED_EDGE('',*,*,#7861,.F.) ;
#10891=ORIENTED_EDGE('',*,*,#7858,.F.) ;
#10892=ORIENTED_EDGE('',*,*,#7855,.F.) ;
#10893=ORIENTED_EDGE('',*,*,#7852,.F.) ;
#10894=ORIENTED_EDGE('',*,*,#7993,.F.) ;
#10895=ORIENTED_EDGE('',*,*,#7873,.T.) ;
#10896=ORIENTED_EDGE('',*,*,#7877,.T.) ;
#10897=ORIENTED_EDGE('',*,*,#7880,.T.) ;
#10898=ORIENTED_EDGE('',*,*,#7883,.T.) ;
#10899=ORIENTED_EDGE('',*,*,#7886,.T.) ;
#10900=ORIENTED_EDGE('',*,*,#7889,.T.) ;
#10901=ORIENTED_EDGE('',*,*,#7940,.T.) ;
#10902=ORIENTED_EDGE('',*,*,#8022,.F.) ;
#10903=ORIENTED_EDGE('',*,*,#8023,.F.) ;
#10904=ORIENTED_EDGE('',*,*,#7938,.F.) ;
#10905=ORIENTED_EDGE('',*,*,#7890,.F.) ;
#10906=ORIENTED_EDGE('',*,*,#7887,.F.) ;
#10907=ORIENTED_EDGE('',*,*,#7884,.F.) ;
#10908=ORIENTED_EDGE('',*,*,#7881,.F.) ;
#10909=ORIENTED_EDGE('',*,*,#7878,.F.) ;
#10910=ORIENTED_EDGE('',*,*,#7875,.F.) ;
#10911=ORIENTED_EDGE('',*,*,#7994,.F.) ;
#10912=ORIENTED_EDGE('',*,*,#7850,.F.) ;
#10913=ORIENTED_EDGE('',*,*,#7854,.F.) ;
#10914=ORIENTED_EDGE('',*,*,#7857,.F.) ;
#10915=ORIENTED_EDGE('',*,*,#7860,.F.) ;
#10916=ORIENTED_EDGE('',*,*,#7863,.F.) ;
#10917=ORIENTED_EDGE('',*,*,#7866,.F.) ;
#10918=ORIENTED_EDGE('',*,*,#7870,.F.) ;
#10919=ORIENTED_EDGE('',*,*,#8021,.T.) ;
#10920=ORIENTED_EDGE('',*,*,#7939,.T.) ;
#10921=ORIENTED_EDGE('',*,*,#8023,.T.) ;
#10922=ORIENTED_EDGE('',*,*,#8022,.T.) ;
#10923=ORIENTED_EDGE('',*,*,#7869,.T.) ;
#10924=ORIENTED_EDGE('',*,*,#7942,.T.) ;
#10925=ORIENTED_EDGE('',*,*,#8024,.F.) ;
#10926=ORIENTED_EDGE('',*,*,#7964,.F.) ;
#10927=ORIENTED_EDGE('',*,*,#8025,.F.) ;
#10928=ORIENTED_EDGE('',*,*,#8026,.F.) ;
#10929=ORIENTED_EDGE('',*,*,#8027,.T.) ;
#10930=ORIENTED_EDGE('',*,*,#7965,.F.) ;
#10931=ORIENTED_EDGE('',*,*,#8027,.F.) ;
#10932=ORIENTED_EDGE('',*,*,#8028,.F.) ;
#10933=ORIENTED_EDGE('',*,*,#8029,.T.) ;
#10934=ORIENTED_EDGE('',*,*,#7966,.F.) ;
#10935=ORIENTED_EDGE('',*,*,#8029,.F.) ;
#10936=ORIENTED_EDGE('',*,*,#8030,.F.) ;
#10937=ORIENTED_EDGE('',*,*,#8031,.T.) ;
#10938=ORIENTED_EDGE('',*,*,#7967,.F.) ;
#10939=ORIENTED_EDGE('',*,*,#8031,.F.) ;
#10940=ORIENTED_EDGE('',*,*,#8032,.F.) ;
#10941=ORIENTED_EDGE('',*,*,#8025,.T.) ;
#10942=ORIENTED_EDGE('',*,*,#8028,.T.) ;
#10943=ORIENTED_EDGE('',*,*,#8026,.T.) ;
#10944=ORIENTED_EDGE('',*,*,#8032,.T.) ;
#10945=ORIENTED_EDGE('',*,*,#8030,.T.) ;
#10946=ORIENTED_EDGE('',*,*,#8033,.F.) ;
#10947=ORIENTED_EDGE('',*,*,#8034,.T.) ;
#10948=ORIENTED_EDGE('',*,*,#8024,.T.) ;
#10949=ORIENTED_EDGE('',*,*,#8034,.F.) ;
#10950=ORIENTED_EDGE('',*,*,#8035,.F.) ;
#10951=ORIENTED_EDGE('',*,*,#8033,.T.) ;
#10952=ORIENTED_EDGE('',*,*,#7987,.F.) ;
#10953=ORIENTED_EDGE('',*,*,#8036,.T.) ;
#10954=ORIENTED_EDGE('',*,*,#8035,.T.) ;
#10955=ORIENTED_EDGE('',*,*,#8036,.F.) ;
#10956=ORIENTED_EDGE('',*,*,#8008,.F.) ;
#10957=ORIENTED_EDGE('',*,*,#8037,.T.) ;
#10958=ORIENTED_EDGE('',*,*,#7984,.T.) ;
#10959=ORIENTED_EDGE('',*,*,#8037,.F.) ;
#10960=ORIENTED_EDGE('',*,*,#8038,.F.) ;
#10961=ORIENTED_EDGE('',*,*,#8039,.T.) ;
#10962=ORIENTED_EDGE('',*,*,#8005,.T.) ;
#10963=ORIENTED_EDGE('',*,*,#8039,.F.) ;
#10964=ORIENTED_EDGE('',*,*,#8038,.T.) ;
#10965=ORIENTED_EDGE('',*,*,#8040,.F.) ;
#10966=ORIENTED_EDGE('',*,*,#8041,.F.) ;
#10967=ORIENTED_EDGE('',*,*,#8042,.T.) ;
#10968=ORIENTED_EDGE('',*,*,#8040,.T.) ;
#10969=ORIENTED_EDGE('',*,*,#8042,.F.) ;
#10970=ORIENTED_EDGE('',*,*,#7974,.F.) ;
#10971=ORIENTED_EDGE('',*,*,#8041,.T.) ;
#10972=ORIENTED_EDGE('',*,*,#8043,.F.) ;
#10973=ORIENTED_EDGE('',*,*,#8044,.T.) ;
#10974=ORIENTED_EDGE('',*,*,#7968,.T.) ;
#10975=ORIENTED_EDGE('',*,*,#8044,.F.) ;
#10976=ORIENTED_EDGE('',*,*,#8016,.T.) ;
#10977=ORIENTED_EDGE('',*,*,#7811,.F.) ;
#10978=ORIENTED_EDGE('',*,*,#8020,.T.) ;
#10979=ORIENTED_EDGE('',*,*,#7893,.T.) ;
#10980=ORIENTED_EDGE('',*,*,#8017,.F.) ;
#10981=ORIENTED_EDGE('',*,*,#8043,.T.) ;
#14538=CONICAL_SURFACE('',#16078,13.3250000000001,0.785398163397564) ;
#14539=CONICAL_SURFACE('',#16086,17.375,0.785398163397199) ;
#14540=CONICAL_SURFACE('',#16091,19.8749999999998,0.785398163397706) ;
#14541=CONICAL_SURFACE('',#16099,22.375,0.785398163397484) ;
#14542=CONICAL_SURFACE('',#16106,33.3824824663842,0.611520837079942) ;
#14543=CONICAL_SURFACE('',#16114,26.7825,1.22304167415987) ;
#14544=CONICAL_SURFACE('',#16116,33.375,0.785398163397448) ;
#14545=CONICAL_SURFACE('',#16120,15.7556101392397,0.797758865436123) ;
#14546=CONICAL_SURFACE('',#16124,14.41685,0.0247214040773807) ;
#14547=CONICAL_SURFACE('',#16126,33.375,0.785398163397439) ;
#14548=CONICAL_SURFACE('',#16135,33.375,0.785398163397439) ;
#14809=ADVANCED_FACE('',(#1721),#1200,.T.) ;
#14810=ADVANCED_FACE('',(#1722),#1201,.T.) ;
#14811=ADVANCED_FACE('',(#1723),#1202,.T.) ;
#14812=ADVANCED_FACE('',(#1724),#1203,.T.) ;
#14813=ADVANCED_FACE('',(#1725),#1204,.T.) ;
#14814=ADVANCED_FACE('',(#1726),#1205,.T.) ;
#14815=ADVANCED_FACE('',(#1727),#1206,.T.) ;
#14816=ADVANCED_FACE('',(#1728),#1207,.T.) ;
#14817=ADVANCED_FACE('',(#1729),#1208,.T.) ;
#14818=ADVANCED_FACE('',(#1730),#1209,.T.) ;
#14819=ADVANCED_FACE('',(#1731),#1210,.T.) ;
#14820=ADVANCED_FACE('',(#1732),#1211,.T.) ;
#14821=ADVANCED_FACE('',(#1733),#1212,.T.) ;
#14822=ADVANCED_FACE('',(#1734),#1213,.T.) ;
#14823=ADVANCED_FACE('',(#1735),#1214,.T.) ;
#14824=ADVANCED_FACE('',(#1736),#1215,.T.) ;
#14825=ADVANCED_FACE('',(#1737),#1216,.T.) ;
#14826=ADVANCED_FACE('',(#1738),#1217,.T.) ;
#14827=ADVANCED_FACE('',(#1739),#1218,.T.) ;
#14828=ADVANCED_FACE('',(#1740),#1219,.T.) ;
#14829=ADVANCED_FACE('',(#1741),#1220,.T.) ;
#14830=ADVANCED_FACE('',(#1742),#1221,.T.) ;
#14831=ADVANCED_FACE('',(#1743),#1222,.T.) ;
#14832=ADVANCED_FACE('',(#1744),#1223,.T.) ;
#14833=ADVANCED_FACE('',(#1745),#1224,.T.) ;
#14834=ADVANCED_FACE('',(#1746),#1225,.T.) ;
#14835=ADVANCED_FACE('',(#1747),#1226,.T.) ;
#14836=ADVANCED_FACE('',(#1748),#1227,.T.) ;
#14837=ADVANCED_FACE('',(#1749),#1228,.T.) ;
#14838=ADVANCED_FACE('',(#1750),#1229,.T.) ;
#14839=ADVANCED_FACE('',(#1751),#1230,.T.) ;
#14840=ADVANCED_FACE('',(#1752),#1231,.T.) ;
#14841=ADVANCED_FACE('',(#1753),#1232,.T.) ;
#14842=ADVANCED_FACE('',(#1754),#1233,.T.) ;
#14843=ADVANCED_FACE('',(#1755),#1234,.T.) ;
#14844=ADVANCED_FACE('',(#1756),#1235,.T.) ;
#14845=ADVANCED_FACE('',(#1757),#1236,.T.) ;
#14846=ADVANCED_FACE('',(#1758),#1237,.T.) ;
#14847=ADVANCED_FACE('',(#1759),#1238,.T.) ;
#14848=ADVANCED_FACE('',(#1760),#1239,.T.) ;
#14849=ADVANCED_FACE('',(#1761),#1240,.T.) ;
#14850=ADVANCED_FACE('',(#1762),#1241,.T.) ;
#14851=ADVANCED_FACE('',(#1763),#1242,.T.) ;
#14852=ADVANCED_FACE('',(#1764),#14538,.F.) ;
#14853=ADVANCED_FACE('',(#1765,#731),#882,.T.) ;
#14854=ADVANCED_FACE('',(#1766),#1243,.F.) ;
#14855=ADVANCED_FACE('',(#1767),#14539,.T.) ;
#14856=ADVANCED_FACE('',(#1768),#1244,.T.) ;
#14857=ADVANCED_FACE('',(#1769),#14540,.T.) ;
#14858=ADVANCED_FACE('',(#1770,#732),#1245,.T.) ;
#14859=ADVANCED_FACE('',(#1771,#733),#883,.T.) ;
#14860=ADVANCED_FACE('',(#1772),#14541,.T.) ;
#14861=ADVANCED_FACE('',(#1773),#1246,.T.) ;
#14862=ADVANCED_FACE('',(#1774,#734),#884,.T.) ;
#14863=ADVANCED_FACE('',(#1775),#14542,.T.) ;
#14864=ADVANCED_FACE('',(#1776),#1247,.T.) ;
#14865=ADVANCED_FACE('',(#1777),#14543,.T.) ;
#14866=ADVANCED_FACE('',(#1778),#14544,.T.) ;
#14867=ADVANCED_FACE('',(#1779,#735),#885,.T.) ;
#14868=ADVANCED_FACE('',(#1780),#14545,.F.) ;
#14869=ADVANCED_FACE('',(#1781),#14546,.F.) ;
#14870=ADVANCED_FACE('',(#1782,#736),#886,.T.) ;
#14871=ADVANCED_FACE('',(#1783),#14547,.T.) ;
#14872=ADVANCED_FACE('',(#1784,#737,#738,#739),#1248,.T.) ;
#14873=ADVANCED_FACE('',(#1785,#740),#887,.T.) ;
#14874=ADVANCED_FACE('',(#1786),#14548,.T.) ;
#14875=ADVANCED_FACE('',(#1787,#741),#888,.T.) ;
#14876=ADVANCED_FACE('',(#1788),#215,.F.) ;
#14877=ADVANCED_FACE('',(#1789),#1249,.T.) ;
#14878=ADVANCED_FACE('',(#1790),#216,.F.) ;
#14879=ADVANCED_FACE('',(#1791),#1250,.T.) ;
#14880=ADVANCED_FACE('',(#1792),#217,.F.) ;
#14881=ADVANCED_FACE('',(#1793),#1251,.T.) ;
#14882=ADVANCED_FACE('',(#1794),#218,.F.) ;
#14883=ADVANCED_FACE('',(#1795),#219,.F.) ;
#14884=ADVANCED_FACE('',(#1796,#742),#889,.T.) ;
#14885=ADVANCED_FACE('',(#1797),#220,.F.) ;
#14886=ADVANCED_FACE('',(#1798),#221,.F.) ;
#14887=ADVANCED_FACE('',(#1799,#743),#890,.T.) ;
#14888=ADVANCED_FACE('',(#1800),#891,.F.) ;
#14889=ADVANCED_FACE('',(#1801),#1252,.F.) ;
#14890=ADVANCED_FACE('',(#1802),#892,.F.) ;
#14891=ADVANCED_FACE('',(#1803),#1253,.F.) ;
#14892=ADVANCED_FACE('',(#1804),#893,.T.) ;
#14893=ADVANCED_FACE('',(#1805),#1254,.T.) ;
#14894=ADVANCED_FACE('',(#1806,#744),#894,.T.) ;
#14895=ADVANCED_FACE('',(#1807),#1255,.T.) ;
#14896=ADVANCED_FACE('',(#1808),#1256,.T.) ;
#14897=ADVANCED_FACE('',(#1809),#1257,.T.) ;
#14898=ADVANCED_FACE('',(#1810,#745),#895,.T.) ;
#14899=ADVANCED_FACE('',(#1811),#1258,.T.) ;
#14900=ADVANCED_FACE('',(#1812,#746),#896,.T.) ;
#14901=ADVANCED_FACE('',(#1813),#1259,.T.) ;
#14902=ADVANCED_FACE('',(#1814,#747),#897,.T.) ;
#15499=CLOSED_SHELL('',(#14809,#14810,#14811,#14812,#14813,#14814,#14815,
#14816,#14817,#14818,#14819,#14820,#14821,#14822,#14823,#14824,#14825,#14826,
#14827,#14828,#14829,#14830,#14831,#14832,#14833,#14834,#14835,#14836,#14837,
#14838,#14839,#14840,#14841,#14842,#14843,#14844,#14845,#14846,#14847,#14848,
#14849,#14850,#14851,#14852,#14853,#14854,#14855,#14856,#14857,#14858,#14859,
#14860,#14861,#14862,#14863,#14864,#14865,#14866,#14867,#14868,#14869,#14870,
#14871,#14872,#14873,#14874,#14875,#14876,#14877,#14878,#14879,#14880,#14881,
#14882,#14883,#14884,#14885,#14886,#14887,#14888,#14889,#14890,#14891,#14892,
#14893,#14894,#14895,#14896,#14897,#14898,#14899,#14900,#14901,#14902)) ;
#16025=AXIS2_PLACEMENT_3D('',#23798,#18788,#18789) ;
#16026=AXIS2_PLACEMENT_3D('',#23799,#18790,#18791) ;
#16027=AXIS2_PLACEMENT_3D('',#23937,#18793,#18794) ;
#16028=AXIS2_PLACEMENT_3D('',#24010,#18795,#18796) ;
#16029=AXIS2_PLACEMENT_3D('',#24708,#18798,#18799) ;
#16030=AXIS2_PLACEMENT_3D('',#25406,#18801,#18802) ;
#16031=AXIS2_PLACEMENT_3D('',#26236,#18804,#18805) ;
#16032=AXIS2_PLACEMENT_3D('',#27004,#18807,#18808) ;
#16033=AXIS2_PLACEMENT_3D('',#27734,#18810,#18811) ;
#16034=AXIS2_PLACEMENT_3D('',#28440,#18813,#18814) ;
#16035=AXIS2_PLACEMENT_3D('',#29108,#18816,#18817) ;
#16036=AXIS2_PLACEMENT_3D('',#29810,#18819,#18820) ;
#16037=AXIS2_PLACEMENT_3D('',#30596,#18822,#18823) ;
#16038=AXIS2_PLACEMENT_3D('',#31374,#18825,#18826) ;
#16039=AXIS2_PLACEMENT_3D('',#32052,#18828,#18829) ;
#16040=AXIS2_PLACEMENT_3D('',#32744,#18831,#18832) ;
#16041=AXIS2_PLACEMENT_3D('',#32800,#18834,#18835) ;
#16042=AXIS2_PLACEMENT_3D('',#32833,#18836,#18837) ;
#16043=AXIS2_PLACEMENT_3D('',#33143,#18839,#18840) ;
#16044=AXIS2_PLACEMENT_3D('',#33459,#18842,#18843) ;
#16045=AXIS2_PLACEMENT_3D('',#33773,#18845,#18846) ;
#16046=AXIS2_PLACEMENT_3D('',#34457,#18848,#18849) ;
#16047=AXIS2_PLACEMENT_3D('',#35153,#18851,#18852) ;
#16048=AXIS2_PLACEMENT_3D('',#35158,#18854,#18855) ;
#16049=AXIS2_PLACEMENT_3D('',#35836,#18856,#18857) ;
#16050=AXIS2_PLACEMENT_3D('',#35940,#18859,#18860) ;
#16051=AXIS2_PLACEMENT_3D('',#36013,#18861,#18862) ;
#16052=AXIS2_PLACEMENT_3D('',#36313,#18864,#18865) ;
#16053=AXIS2_PLACEMENT_3D('',#36613,#18867,#18868) ;
#16054=AXIS2_PLACEMENT_3D('',#36903,#18870,#18871) ;
#16055=AXIS2_PLACEMENT_3D('',#37203,#18873,#18874) ;
#16056=AXIS2_PLACEMENT_3D('',#37509,#18876,#18877) ;
#16057=AXIS2_PLACEMENT_3D('',#37755,#18879,#18880) ;
#16058=AXIS2_PLACEMENT_3D('',#37904,#18881,#18882) ;
#16059=AXIS2_PLACEMENT_3D('',#38596,#18884,#18885) ;
#16060=AXIS2_PLACEMENT_3D('',#39384,#18887,#18888) ;
#16061=AXIS2_PLACEMENT_3D('',#40179,#18890,#18891) ;
#16062=AXIS2_PLACEMENT_3D('',#40869,#18893,#18894) ;
#16063=AXIS2_PLACEMENT_3D('',#41617,#18896,#18897) ;
#16064=AXIS2_PLACEMENT_3D('',#42333,#18899,#18900) ;
#16065=AXIS2_PLACEMENT_3D('',#43025,#18902,#18903) ;
#16066=AXIS2_PLACEMENT_3D('',#43885,#18905,#18906) ;
#16067=AXIS2_PLACEMENT_3D('',#44569,#18908,#18909) ;
#16068=AXIS2_PLACEMENT_3D('',#45318,#18911,#18912) ;
#16069=AXIS2_PLACEMENT_3D('',#46022,#18914,#18915) ;
#16070=AXIS2_PLACEMENT_3D('',#46706,#18917,#18918) ;
#16071=AXIS2_PLACEMENT_3D('',#47049,#18919,#18920) ;
#16072=AXIS2_PLACEMENT_3D('',#47252,#18921,#18922) ;
#16073=AXIS2_PLACEMENT_3D('',#47367,#18923,#18924) ;
#16074=AXIS2_PLACEMENT_3D('',#47458,#18925,#18926) ;
#16075=AXIS2_PLACEMENT_3D('',#47500,#18927,#18928) ;
#16076=AXIS2_PLACEMENT_3D('',#47501,#18929,#18930) ;
#16077=AXIS2_PLACEMENT_3D('',#47878,#18931,#18932) ;
#16078=AXIS2_PLACEMENT_3D('',#48138,#18933,#18934) ;
#16079=AXIS2_PLACEMENT_3D('',#48141,#18935,#18936) ;
#16080=AXIS2_PLACEMENT_3D('',#48144,#18938,#18939) ;
#16081=AXIS2_PLACEMENT_3D('',#48145,#18940,#18941) ;
#16082=AXIS2_PLACEMENT_3D('',#48146,#18942,#18943) ;
#16083=AXIS2_PLACEMENT_3D('',#48148,#18944,#18945) ;
#16084=AXIS2_PLACEMENT_3D('',#48149,#18946,#18947) ;
#16085=AXIS2_PLACEMENT_3D('',#48151,#18948,#18949) ;
#16086=AXIS2_PLACEMENT_3D('',#48153,#18951,#18952) ;
#16087=AXIS2_PLACEMENT_3D('',#48156,#18953,#18954) ;
#16088=AXIS2_PLACEMENT_3D('',#48158,#18956,#18957) ;
#16089=AXIS2_PLACEMENT_3D('',#48159,#18958,#18959) ;
#16090=AXIS2_PLACEMENT_3D('',#48162,#18961,#18962) ;
#16091=AXIS2_PLACEMENT_3D('',#48163,#18963,#18964) ;
#16092=AXIS2_PLACEMENT_3D('',#48166,#18965,#18966) ;
#16093=AXIS2_PLACEMENT_3D('',#48169,#18968,#18969) ;
#16094=AXIS2_PLACEMENT_3D('',#48170,#18970,#18971) ;
#16095=AXIS2_PLACEMENT_3D('',#48171,#18972,#18973) ;
#16096=AXIS2_PLACEMENT_3D('',#48174,#18975,#18976) ;
#16097=AXIS2_PLACEMENT_3D('',#48217,#18979,#18980) ;
#16098=AXIS2_PLACEMENT_3D('',#48219,#18981,#18982) ;
#16099=AXIS2_PLACEMENT_3D('',#48220,#18983,#18984) ;
#16100=AXIS2_PLACEMENT_3D('',#48223,#18985,#18986) ;
#16101=AXIS2_PLACEMENT_3D('',#48226,#18988,#18989) ;
#16102=AXIS2_PLACEMENT_3D('',#48227,#18990,#18991) ;
#16103=AXIS2_PLACEMENT_3D('',#48228,#18992,#18993) ;
#16104=AXIS2_PLACEMENT_3D('',#48231,#18995,#18996) ;
#16105=AXIS2_PLACEMENT_3D('',#48232,#18997,#18998) ;
#16106=AXIS2_PLACEMENT_3D('',#48233,#18999,#19000) ;
#16107=AXIS2_PLACEMENT_3D('',#48236,#19001,#19002) ;
#16108=AXIS2_PLACEMENT_3D('',#48240,#19004,#19005) ;
#16109=AXIS2_PLACEMENT_3D('',#48241,#19006,#19007) ;
#16110=AXIS2_PLACEMENT_3D('',#48242,#19008,#19009) ;
#16111=AXIS2_PLACEMENT_3D('',#48243,#19010,#19011) ;
#16112=AXIS2_PLACEMENT_3D('',#48247,#19013,#19014) ;
#16113=AXIS2_PLACEMENT_3D('',#48248,#19015,#19016) ;
#16114=AXIS2_PLACEMENT_3D('',#48249,#19017,#19018) ;
#16115=AXIS2_PLACEMENT_3D('',#48252,#19020,#19021) ;
#16116=AXIS2_PLACEMENT_3D('',#48253,#19022,#19023) ;
#16117=AXIS2_PLACEMENT_3D('',#48256,#19025,#19026) ;
#16118=AXIS2_PLACEMENT_3D('',#48257,#19027,#19028) ;
#16119=AXIS2_PLACEMENT_3D('',#48259,#19029,#19030) ;
#16120=AXIS2_PLACEMENT_3D('',#48260,#19031,#19032) ;
#16121=AXIS2_PLACEMENT_3D('',#48263,#19033,#19034) ;
#16122=AXIS2_PLACEMENT_3D('',#48266,#19036,#19037) ;
#16123=AXIS2_PLACEMENT_3D('',#48267,#19038,#19039) ;
#16124=AXIS2_PLACEMENT_3D('',#48268,#19040,#19041) ;
#16125=AXIS2_PLACEMENT_3D('',#48270,#19043,#19044) ;
#16126=AXIS2_PLACEMENT_3D('',#48415,#19045,#19046) ;
#16127=AXIS2_PLACEMENT_3D('',#48418,#19047,#19048) ;
#16128=AXIS2_PLACEMENT_3D('',#48421,#19050,#19051) ;
#16129=AXIS2_PLACEMENT_3D('',#48422,#19052,#19053) ;
#16130=AXIS2_PLACEMENT_3D('',#48423,#19054,#19055) ;
#16131=AXIS2_PLACEMENT_3D('',#48427,#19057,#19058) ;
#16132=AXIS2_PLACEMENT_3D('',#48428,#19059,#19060) ;
#16133=AXIS2_PLACEMENT_3D('',#48534,#19061,#19062) ;
#16134=AXIS2_PLACEMENT_3D('',#48536,#19063,#19064) ;
#16135=AXIS2_PLACEMENT_3D('',#48537,#19065,#19066) ;
#16136=AXIS2_PLACEMENT_3D('',#48540,#19068,#19069) ;
#16137=AXIS2_PLACEMENT_3D('',#48541,#19070,#19071) ;
#16138=AXIS2_PLACEMENT_3D('',#48543,#19072,#19073) ;
#16139=AXIS2_PLACEMENT_3D('',#48670,#19074,#19075) ;
#16140=AXIS2_PLACEMENT_3D('',#48797,#19076,#19077) ;
#16141=AXIS2_PLACEMENT_3D('',#48924,#19078,#19079) ;
#16142=AXIS2_PLACEMENT_3D('',#50860,#19080,#19081) ;
#16143=AXIS2_PLACEMENT_3D('',#51819,#19082,#19083) ;
#16144=AXIS2_PLACEMENT_3D('',#51821,#19084,#19085) ;
#16145=AXIS2_PLACEMENT_3D('',#51822,#19086,#19087) ;
#16146=AXIS2_PLACEMENT_3D('',#51828,#19091,#19092) ;
#16147=AXIS2_PLACEMENT_3D('',#51830,#19093,#19094) ;
#16148=AXIS2_PLACEMENT_3D('',#51832,#19096,#19097) ;
#16149=AXIS2_PLACEMENT_3D('',#51836,#19100,#19101) ;
#16150=AXIS2_PLACEMENT_3D('',#51837,#19102,#19103) ;
#16151=AXIS2_PLACEMENT_3D('',#51838,#19104,#19105) ;
#16152=AXIS2_PLACEMENT_3D('',#51839,#19106,#19107) ;
#16153=AXIS2_PLACEMENT_3D('',#51841,#19108,#19109) ;
#16154=AXIS2_PLACEMENT_3D('',#51843,#19111,#19112) ;
#16155=AXIS2_PLACEMENT_3D('',#51845,#19113,#19114) ;
#16156=AXIS2_PLACEMENT_3D('',#51846,#19115,#19116) ;
#16157=AXIS2_PLACEMENT_3D('',#51848,#19118,#19119) ;
#16158=AXIS2_PLACEMENT_3D('',#51850,#19121,#19122) ;
#16159=AXIS2_PLACEMENT_3D('',#51852,#19123,#19124) ;
#16160=AXIS2_PLACEMENT_3D('',#51854,#19126,#19127) ;
#16161=AXIS2_PLACEMENT_3D('',#51856,#19128,#19129) ;
#16162=AXIS2_PLACEMENT_3D('',#51857,#19130,#19131) ;
#16163=AXIS2_PLACEMENT_3D('',#51859,#19132,#19133) ;
#16164=AXIS2_PLACEMENT_3D('',#51861,#19135,#19136) ;
#16165=AXIS2_PLACEMENT_3D('',#51862,#19137,#19138) ;
#16166=AXIS2_PLACEMENT_3D('',#51864,#19139,#19140) ;
#16167=AXIS2_PLACEMENT_3D('',#51866,#19142,#19143) ;
#18788=DIRECTION('axis',(0.,0.,1.)) ;
#18789=DIRECTION('refdir',(1.,0.,0.)) ;
#18790=DIRECTION('center_axis',(0.,0.,-1.)) ;
#18791=DIRECTION('ref_axis',(0.,1.,0.)) ;
#18792=DIRECTION('',(0.,0.,1.)) ;
#18793=DIRECTION('center_axis',(0.,0.,-1.)) ;
#18794=DIRECTION('ref_axis',(0.,1.,0.)) ;
#18795=DIRECTION('center_axis',(0.,0.,-1.)) ;
#18796=DIRECTION('ref_axis',(0.,1.,0.)) ;
#18797=DIRECTION('',(0.,0.,1.)) ;
#18798=DIRECTION('center_axis',(0.,0.,-1.)) ;
#18799=DIRECTION('ref_axis',(0.,1.,0.)) ;
#18800=DIRECTION('',(0.,0.,1.)) ;
#18801=DIRECTION('center_axis',(0.,0.,-1.)) ;
#18802=DIRECTION('ref_axis',(0.,1.,0.)) ;
#18803=DIRECTION('',(0.,0.,1.)) ;
#18804=DIRECTION('center_axis',(0.,0.,-1.)) ;
#18805=DIRECTION('ref_axis',(0.,1.,0.)) ;
#18806=DIRECTION('',(0.,0.,1.)) ;
#18807=DIRECTION('center_axis',(0.,0.,-1.)) ;
#18808=DIRECTION('ref_axis',(0.,1.,0.)) ;
#18809=DIRECTION('',(0.,0.,1.)) ;
#18810=DIRECTION('center_axis',(0.,0.,-1.)) ;
#18811=DIRECTION('ref_axis',(0.,1.,0.)) ;
#18812=DIRECTION('',(0.,0.,1.)) ;
#18813=DIRECTION('center_axis',(0.,0.,-1.)) ;
#18814=DIRECTION('ref_axis',(0.,1.,0.)) ;
#18815=DIRECTION('',(0.,0.,1.)) ;
#18816=DIRECTION('center_axis',(0.,0.,-1.)) ;
#18817=DIRECTION('ref_axis',(0.,1.,0.)) ;
#18818=DIRECTION('',(0.,0.,1.)) ;
#18819=DIRECTION('center_axis',(0.,0.,-1.)) ;
#18820=DIRECTION('ref_axis',(0.,1.,0.)) ;
#18821=DIRECTION('',(0.,0.,1.)) ;
#18822=DIRECTION('center_axis',(0.,0.,-1.)) ;
#18823=DIRECTION('ref_axis',(0.,1.,0.)) ;
#18824=DIRECTION('',(0.,0.,1.)) ;
#18825=DIRECTION('center_axis',(0.,0.,-1.)) ;
#18826=DIRECTION('ref_axis',(0.,1.,0.)) ;
#18827=DIRECTION('',(0.,0.,1.)) ;
#18828=DIRECTION('center_axis',(0.,0.,-1.)) ;
#18829=DIRECTION('ref_axis',(0.,1.,0.)) ;
#18830=DIRECTION('',(0.,0.,1.)) ;
#18831=DIRECTION('center_axis',(0.,0.,-1.)) ;
#18832=DIRECTION('ref_axis',(0.849891577299213,-0.526957594912394,0.)) ;
#18833=DIRECTION('',(0.,0.,1.)) ;
#18834=DIRECTION('center_axis',(0.,0.,-1.)) ;
#18835=DIRECTION('ref_axis',(0.,1.,0.)) ;
#18836=DIRECTION('center_axis',(0.,0.,-1.)) ;
#18837=DIRECTION('ref_axis',(0.,1.,0.)) ;
#18838=DIRECTION('',(0.,0.,1.)) ;
#18839=DIRECTION('center_axis',(0.,0.,-1.)) ;
#18840=DIRECTION('ref_axis',(0.,1.,0.)) ;
#18841=DIRECTION('',(0.,0.,1.)) ;
#18842=DIRECTION('center_axis',(0.,0.,-1.)) ;
#18843=DIRECTION('ref_axis',(0.,1.,0.)) ;
#18844=DIRECTION('',(0.,0.,1.)) ;
#18845=DIRECTION('center_axis',(0.,0.,-1.)) ;
#18846=DIRECTION('ref_axis',(0.,1.,0.)) ;
#18847=DIRECTION('',(0.,0.,1.)) ;
#18848=DIRECTION('center_axis',(0.,0.,-1.)) ;
#18849=DIRECTION('ref_axis',(0.,1.,0.)) ;
#18850=DIRECTION('',(0.,0.,1.)) ;
#18851=DIRECTION('center_axis',(0.,0.,-1.)) ;
#18852=DIRECTION('ref_axis',(0.,1.,0.)) ;
#18853=DIRECTION('',(0.,0.,1.)) ;
#18854=DIRECTION('center_axis',(0.,0.,1.)) ;
#18855=DIRECTION('ref_axis',(0.,1.,0.)) ;
#18856=DIRECTION('center_axis',(0.,0.,-1.)) ;
#18857=DIRECTION('ref_axis',(-0.891629331176974,0.45276609389938,0.)) ;
#18858=DIRECTION('',(0.,0.,1.)) ;
#18859=DIRECTION('center_axis',(0.,0.,1.)) ;
#18860=DIRECTION('ref_axis',(1.95976813240396E-14,1.,0.)) ;
#18861=DIRECTION('center_axis',(0.,0.,-1.)) ;
#18862=DIRECTION('ref_axis',(-0.891629331176974,0.45276609389938,0.)) ;
#18863=DIRECTION('',(0.,0.,1.)) ;
#18864=DIRECTION('center_axis',(0.,0.,-1.)) ;
#18865=DIRECTION('ref_axis',(-0.891629331176974,0.45276609389938,0.)) ;
#18866=DIRECTION('',(0.,0.,1.)) ;
#18867=DIRECTION('center_axis',(0.,0.,-1.)) ;
#18868=DIRECTION('ref_axis',(-0.891629331176974,0.45276609389938,0.)) ;
#18869=DIRECTION('',(0.,0.,1.)) ;
#18870=DIRECTION('center_axis',(0.,0.,-1.)) ;
#18871=DIRECTION('ref_axis',(-0.891629331176974,0.45276609389938,0.)) ;
#18872=DIRECTION('',(0.,0.,1.)) ;
#18873=DIRECTION('center_axis',(0.,0.,-1.)) ;
#18874=DIRECTION('ref_axis',(-0.891629331176974,0.45276609389938,0.)) ;
#18875=DIRECTION('',(0.,0.,1.)) ;
#18876=DIRECTION('center_axis',(0.,0.,-1.)) ;
#18877=DIRECTION('ref_axis',(-0.998852985909418,0.04788227793077,0.)) ;
#18878=DIRECTION('',(0.,0.,1.)) ;
#18879=DIRECTION('center_axis',(0.,0.,1.)) ;
#18880=DIRECTION('ref_axis',(7.83153288810636E-14,1.,0.)) ;
#18881=DIRECTION('center_axis',(0.,0.,-1.)) ;
#18882=DIRECTION('ref_axis',(-0.998852985909418,0.04788227793077,0.)) ;
#18883=DIRECTION('',(0.,0.,1.)) ;
#18884=DIRECTION('center_axis',(0.,0.,-1.)) ;
#18885=DIRECTION('ref_axis',(-0.998852985909418,0.04788227793077,0.)) ;
#18886=DIRECTION('',(0.,0.,1.)) ;
#18887=DIRECTION('center_axis',(0.,0.,-1.)) ;
#18888=DIRECTION('ref_axis',(-0.998852985909418,0.04788227793077,0.)) ;
#18889=DIRECTION('',(0.,0.,1.)) ;
#18890=DIRECTION('center_axis',(0.,0.,-1.)) ;
#18891=DIRECTION('ref_axis',(-0.998852985909418,0.04788227793077,0.)) ;
#18892=DIRECTION('',(0.,0.,1.)) ;
#18893=DIRECTION('center_axis',(0.,0.,-1.)) ;
#18894=DIRECTION('ref_axis',(-0.998852985909418,0.04788227793077,0.)) ;
#18895=DIRECTION('',(0.,0.,1.)) ;
#18896=DIRECTION('center_axis',(0.,0.,-1.)) ;
#18897=DIRECTION('ref_axis',(-0.998852985909418,0.04788227793077,0.)) ;
#18898=DIRECTION('',(0.,0.,1.)) ;
#18899=DIRECTION('center_axis',(0.,0.,-1.)) ;
#18900=DIRECTION('ref_axis',(-0.998852985909418,0.04788227793077,0.)) ;
#18901=DIRECTION('',(0.,0.,1.)) ;
#18902=DIRECTION('center_axis',(0.,0.,-1.)) ;
#18903=DIRECTION('ref_axis',(-0.998852985909418,0.04788227793077,0.)) ;
#18904=DIRECTION('',(0.,0.,1.)) ;
#18905=DIRECTION('center_axis',(0.,0.,-1.)) ;
#18906=DIRECTION('ref_axis',(-0.998852985909418,0.04788227793077,0.)) ;
#18907=DIRECTION('',(0.,0.,1.)) ;
#18908=DIRECTION('center_axis',(0.,0.,-1.)) ;
#18909=DIRECTION('ref_axis',(-0.998852985909418,0.04788227793077,0.)) ;
#18910=DIRECTION('',(0.,0.,1.)) ;
#18911=DIRECTION('center_axis',(0.,0.,-1.)) ;
#18912=DIRECTION('ref_axis',(-0.998852985909418,0.04788227793077,0.)) ;
#18913=DIRECTION('',(0.,0.,1.)) ;
#18914=DIRECTION('center_axis',(0.,0.,-1.)) ;
#18915=DIRECTION('ref_axis',(-0.998852985909418,0.04788227793077,0.)) ;
#18916=DIRECTION('',(0.,0.,1.)) ;
#18917=DIRECTION('center_axis',(0.,0.,-1.)) ;
#18918=DIRECTION('ref_axis',(-0.998852985909418,0.04788227793077,0.)) ;
#18919=DIRECTION('center_axis',(0.,0.,-1.)) ;
#18920=DIRECTION('ref_axis',(7.83153288810636E-14,1.,0.)) ;
#18921=DIRECTION('center_axis',(0.,0.,-1.)) ;
#18922=DIRECTION('ref_axis',(-0.891629331176974,0.45276609389938,0.)) ;
#18923=DIRECTION('center_axis',(0.,0.,-1.)) ;
#18924=DIRECTION('ref_axis',(1.95976813240396E-14,1.,0.)) ;
#18925=DIRECTION('center_axis',(0.,0.,-1.)) ;
#18926=DIRECTION('ref_axis',(0.,1.,0.)) ;
#18927=DIRECTION('center_axis',(0.,0.,1.)) ;
#18928=DIRECTION('ref_axis',(0.,1.,0.)) ;
#18929=DIRECTION('center_axis',(0.,0.,-1.)) ;
#18930=DIRECTION('ref_axis',(0.,1.,0.)) ;
#18931=DIRECTION('center_axis',(0.,0.,1.)) ;
#18932=DIRECTION('ref_axis',(0.,1.,0.)) ;
#18933=DIRECTION('center_axis',(0.,0.,-1.)) ;
#18934=DIRECTION('ref_axis',(0.,-1.,0.)) ;
#18935=DIRECTION('center_axis',(0.,0.,1.)) ;
#18936=DIRECTION('ref_axis',(0.,-1.,0.)) ;
#18937=DIRECTION('',(8.65956056235593E-17,0.707106781186629,-0.707106781186466)) ;
#18938=DIRECTION('center_axis',(0.,0.,-1.)) ;
#18939=DIRECTION('ref_axis',(0.,-1.,0.)) ;
#18940=DIRECTION('center_axis',(0.,0.,1.)) ;
#18941=DIRECTION('ref_axis',(0.,-1.,0.)) ;
#18942=DIRECTION('center_axis',(0.,0.,-1.)) ;
#18943=DIRECTION('ref_axis',(-1.,0.,0.)) ;
#18944=DIRECTION('center_axis',(0.,0.,1.)) ;
#18945=DIRECTION('ref_axis',(0.,-1.,0.)) ;
#18946=DIRECTION('center_axis',(0.,0.,-1.)) ;
#18947=DIRECTION('ref_axis',(0.,1.,0.)) ;
#18948=DIRECTION('center_axis',(0.,0.,-1.)) ;
#18949=DIRECTION('ref_axis',(1.,0.,0.)) ;
#18950=DIRECTION('',(0.,0.,-1.)) ;
#18951=DIRECTION('center_axis',(0.,0.,1.)) ;
#18952=DIRECTION('ref_axis',(0.,-1.,0.)) ;
#18953=DIRECTION('center_axis',(0.,0.,-1.)) ;
#18954=DIRECTION('ref_axis',(0.,-1.,0.)) ;
#18955=DIRECTION('',(8.65956056235278E-17,-0.707106781186371,-0.707106781186724)) ;
#18956=DIRECTION('center_axis',(0.,0.,-1.)) ;
#18957=DIRECTION('ref_axis',(0.,-1.,0.)) ;
#18958=DIRECTION('center_axis',(0.,0.,-1.)) ;
#18959=DIRECTION('ref_axis',(0.,1.,0.)) ;
#18960=DIRECTION('',(0.,0.,1.)) ;
#18961=DIRECTION('center_axis',(0.,0.,-1.)) ;
#18962=DIRECTION('ref_axis',(1.,0.,0.)) ;
#18963=DIRECTION('center_axis',(0.,0.,1.)) ;
#18964=DIRECTION('ref_axis',(0.,-1.,0.)) ;
#18965=DIRECTION('center_axis',(0.,0.,-1.)) ;
#18966=DIRECTION('ref_axis',(0.,-1.,0.)) ;
#18967=DIRECTION('',(8.65956056235716E-17,-0.70710678118673,-0.707106781186365)) ;
#18968=DIRECTION('center_axis',(0.,0.,1.)) ;
#18969=DIRECTION('ref_axis',(0.,-1.,0.)) ;
#18970=DIRECTION('center_axis',(0.,0.,-1.)) ;
#18971=DIRECTION('ref_axis',(0.,-1.,0.)) ;
#18972=DIRECTION('center_axis',(0.,0.,-1.)) ;
#18973=DIRECTION('ref_axis',(0.,1.,0.)) ;
#18974=DIRECTION('',(0.,0.,1.)) ;
#18975=DIRECTION('center_axis',(0.,0.,-1.)) ;
#18976=DIRECTION('ref_axis',(1.,0.,0.)) ;
#18977=DIRECTION('',(0.,0.,1.)) ;
#18978=DIRECTION('',(0.,0.,-1.)) ;
#18979=DIRECTION('center_axis',(0.,0.,-1.)) ;
#18980=DIRECTION('ref_axis',(-1.,0.,0.)) ;
#18981=DIRECTION('center_axis',(0.,0.,-1.)) ;
#18982=DIRECTION('ref_axis',(1.,0.,0.)) ;
#18983=DIRECTION('center_axis',(0.,0.,1.)) ;
#18984=DIRECTION('ref_axis',(0.,-1.,0.)) ;
#18985=DIRECTION('center_axis',(0.,0.,-1.)) ;
#18986=DIRECTION('ref_axis',(0.,-1.,0.)) ;
#18987=DIRECTION('',(8.65956056235524E-17,-0.707106781186573,-0.707106781186522)) ;
#18988=DIRECTION('center_axis',(0.,0.,1.)) ;
#18989=DIRECTION('ref_axis',(0.,-1.,0.)) ;
#18990=DIRECTION('center_axis',(0.,0.,-1.)) ;
#18991=DIRECTION('ref_axis',(0.,-1.,0.)) ;
#18992=DIRECTION('center_axis',(0.,0.,-1.)) ;
#18993=DIRECTION('ref_axis',(0.,1.,0.)) ;
#18994=DIRECTION('',(0.,0.,1.)) ;
#18995=DIRECTION('center_axis',(0.,0.,-1.)) ;
#18996=DIRECTION('ref_axis',(1.,0.,0.)) ;
#18997=DIRECTION('center_axis',(0.,0.,-1.)) ;
#18998=DIRECTION('ref_axis',(-1.,0.,0.)) ;
#18999=DIRECTION('center_axis',(6.07670133222886E-15,0.,1.)) ;
#19000=DIRECTION('ref_axis',(-3.05083907927506E-17,-1.,1.85390378974466E-31)) ;
#19001=DIRECTION('center_axis',(0.,0.,-1.)) ;
#19002=DIRECTION('ref_axis',(0.,-1.,0.)) ;
#19003=DIRECTION('',(-4.92266285732438E-15,-0.57411334821253,-0.818775832205738)) ;
#19004=DIRECTION('center_axis',(0.,0.,1.)) ;
#19005=DIRECTION('ref_axis',(-6.12323399573677E-17,-1.,0.)) ;
#19006=DIRECTION('center_axis',(0.,0.,1.)) ;
#19007=DIRECTION('ref_axis',(-6.12323399573677E-17,-1.,0.)) ;
#19008=DIRECTION('center_axis',(0.,0.,-1.)) ;
#19009=DIRECTION('ref_axis',(0.,-1.,0.)) ;
#19010=DIRECTION('center_axis',(0.,0.,-1.)) ;
#19011=DIRECTION('ref_axis',(0.,1.,0.)) ;
#19012=DIRECTION('',(0.,0.,1.)) ;
#19013=DIRECTION('center_axis',(0.,0.,1.)) ;
#19014=DIRECTION('ref_axis',(0.,-1.,0.)) ;
#19015=DIRECTION('center_axis',(0.,0.,1.)) ;
#19016=DIRECTION('ref_axis',(0.,-1.,0.)) ;
#19017=DIRECTION('center_axis',(0.,0.,1.)) ;
#19018=DIRECTION('ref_axis',(0.,1.,0.)) ;
#19019=DIRECTION('',(-1.15133977109009E-16,0.940140268926269,-0.340787726808409)) ;
#19020=DIRECTION('center_axis',(0.,0.,-1.)) ;
#19021=DIRECTION('ref_axis',(1.,0.,0.)) ;
#19022=DIRECTION('center_axis',(0.,0.,-1.)) ;
#19023=DIRECTION('ref_axis',(0.,-1.,0.)) ;
#19024=DIRECTION('',(-8.65956056235493E-17,-0.707106781186547,0.707106781186548)) ;
#19025=DIRECTION('center_axis',(0.,0.,-1.)) ;
#19026=DIRECTION('ref_axis',(0.,-1.,0.)) ;
#19027=DIRECTION('center_axis',(0.,0.,1.)) ;
#19028=DIRECTION('ref_axis',(1.,0.,0.)) ;
#19029=DIRECTION('center_axis',(0.,0.,-1.)) ;
#19030=DIRECTION('ref_axis',(1.,0.,0.)) ;
#19031=DIRECTION('center_axis',(3.82880846191654E-15,0.,1.)) ;
#19032=DIRECTION('ref_axis',(-3.03672668314921E-17,-1.,1.16270448209694E-31)) ;
#19033=DIRECTION('center_axis',(0.,0.,-1.)) ;
#19034=DIRECTION('ref_axis',(-6.12323399573677E-17,-1.,0.)) ;
#19035=DIRECTION('',(2.60778271056638E-15,0.715792877193627,0.698312649863132)) ;
#19036=DIRECTION('center_axis',(0.,0.,1.)) ;
#19037=DIRECTION('ref_axis',(0.,-1.,0.)) ;
#19038=DIRECTION('center_axis',(0.,0.,-1.)) ;
#19039=DIRECTION('ref_axis',(-6.12323399573677E-17,-1.,0.)) ;
#19040=DIRECTION('center_axis',(0.,0.,1.)) ;
#19041=DIRECTION('ref_axis',(0.,1.,0.)) ;
#19042=DIRECTION('',(3.02719047191673E-18,-0.0247188860822922,0.999694441652473)) ;
#19043=DIRECTION('center_axis',(0.,0.,1.)) ;
#19044=DIRECTION('ref_axis',(1.,0.,0.)) ;
#19045=DIRECTION('center_axis',(0.,0.,1.)) ;
#19046=DIRECTION('ref_axis',(0.,-1.,0.)) ;
#19047=DIRECTION('center_axis',(0.,0.,-1.)) ;
#19048=DIRECTION('ref_axis',(0.,-1.,0.)) ;
#19049=DIRECTION('',(8.65956056235485E-17,-0.707106781186541,-0.707106781186554)) ;
#19050=DIRECTION('center_axis',(0.,0.,1.)) ;
#19051=DIRECTION('ref_axis',(0.,-1.,0.)) ;
#19052=DIRECTION('center_axis',(0.,0.,-1.)) ;
#19053=DIRECTION('ref_axis',(0.,-1.,0.)) ;
#19054=DIRECTION('center_axis',(0.,0.,-1.)) ;
#19055=DIRECTION('ref_axis',(0.,1.,0.)) ;
#19056=DIRECTION('',(0.,0.,1.)) ;
#19057=DIRECTION('center_axis',(0.,0.,1.)) ;
#19058=DIRECTION('ref_axis',(0.,-1.,0.)) ;
#19059=DIRECTION('center_axis',(0.,0.,1.)) ;
#19060=DIRECTION('ref_axis',(0.,-1.,0.)) ;
#19061=DIRECTION('center_axis',(0.,0.,-1.)) ;
#19062=DIRECTION('ref_axis',(-1.,0.,0.)) ;
#19063=DIRECTION('center_axis',(0.,0.,-1.)) ;
#19064=DIRECTION('ref_axis',(1.,0.,0.)) ;
#19065=DIRECTION('center_axis',(0.,0.,-1.)) ;
#19066=DIRECTION('ref_axis',(0.,-1.,0.)) ;
#19067=DIRECTION('',(-8.65956056235485E-17,-0.707106781186541,0.707106781186554)) ;
#19068=DIRECTION('center_axis',(0.,0.,-1.)) ;
#19069=DIRECTION('ref_axis',(0.,-1.,0.)) ;
#19070=DIRECTION('center_axis',(0.,0.,1.)) ;
#19071=DIRECTION('ref_axis',(1.,0.,0.)) ;
#19072=DIRECTION('center_axis',(0.,0.,-1.)) ;
#19073=DIRECTION('ref_axis',(1.,0.,0.)) ;
#19074=DIRECTION('center_axis',(0.,0.,-1.)) ;
#19075=DIRECTION('ref_axis',(0.,1.,0.)) ;
#19076=DIRECTION('center_axis',(0.,0.,-1.)) ;
#19077=DIRECTION('ref_axis',(0.,1.,0.)) ;
#19078=DIRECTION('center_axis',(0.,0.,-1.)) ;
#19079=DIRECTION('ref_axis',(0.,1.,0.)) ;
#19080=DIRECTION('center_axis',(0.,0.,-1.)) ;
#19081=DIRECTION('ref_axis',(-1.,0.,0.)) ;
#19082=DIRECTION('center_axis',(0.,0.,-1.)) ;
#19083=DIRECTION('ref_axis',(-1.,0.,0.)) ;
#19084=DIRECTION('center_axis',(0.,0.,-1.)) ;
#19085=DIRECTION('ref_axis',(1.,0.,0.)) ;
#19086=DIRECTION('center_axis',(1.,0.,-7.40148683083438E-17)) ;
#19087=DIRECTION('ref_axis',(-7.40148683083438E-17,0.,-1.)) ;
#19088=DIRECTION('',(0.,1.,0.)) ;
#19089=DIRECTION('',(-7.40148683083438E-17,0.,-1.)) ;
#19090=DIRECTION('',(0.,1.,0.)) ;
#19091=DIRECTION('center_axis',(0.,1.,0.)) ;
#19092=DIRECTION('ref_axis',(-1.,0.,0.)) ;
#19093=DIRECTION('center_axis',(0.,1.,0.)) ;
#19094=DIRECTION('ref_axis',(-1.,0.,0.)) ;
#19095=DIRECTION('',(0.,1.,0.)) ;
#19096=DIRECTION('center_axis',(-1.,0.,-2.46716227694479E-17)) ;
#19097=DIRECTION('ref_axis',(-2.46716227694479E-17,0.,1.)) ;
#19098=DIRECTION('',(-2.46716227694479E-17,0.,1.)) ;
#19099=DIRECTION('',(0.,1.,0.)) ;
#19100=DIRECTION('center_axis',(0.,1.,0.)) ;
#19101=DIRECTION('ref_axis',(1.,0.,0.)) ;
#19102=DIRECTION('center_axis',(0.,1.,0.)) ;
#19103=DIRECTION('ref_axis',(1.,0.,0.)) ;
#19104=DIRECTION('center_axis',(0.,1.,0.)) ;
#19105=DIRECTION('ref_axis',(1.,0.,0.)) ;
#19106=DIRECTION('center_axis',(0.,0.,-1.)) ;
#19107=DIRECTION('ref_axis',(0.,1.,0.)) ;
#19108=DIRECTION('center_axis',(0.,0.,-1.)) ;
#19109=DIRECTION('ref_axis',(1.,0.,0.)) ;
#19110=DIRECTION('',(0.,0.,1.)) ;
#19111=DIRECTION('center_axis',(0.,0.,1.)) ;
#19112=DIRECTION('ref_axis',(1.,0.,0.)) ;
#19113=DIRECTION('center_axis',(0.,0.,-1.)) ;
#19114=DIRECTION('ref_axis',(1.,0.,0.)) ;
#19115=DIRECTION('center_axis',(0.,0.,-1.)) ;
#19116=DIRECTION('ref_axis',(0.,1.,0.)) ;
#19117=DIRECTION('',(0.,0.,1.)) ;
#19118=DIRECTION('center_axis',(0.,0.,-1.)) ;
#19119=DIRECTION('ref_axis',(0.,1.,0.)) ;
#19120=DIRECTION('',(0.,0.,1.)) ;
#19121=DIRECTION('center_axis',(0.,0.,-1.)) ;
#19122=DIRECTION('ref_axis',(0.,1.,0.)) ;
#19123=DIRECTION('center_axis',(0.,0.,-1.)) ;
#19124=DIRECTION('ref_axis',(1.,0.,0.)) ;
#19125=DIRECTION('',(0.,0.,1.)) ;
#19126=DIRECTION('center_axis',(0.,0.,-1.)) ;
#19127=DIRECTION('ref_axis',(-1.,0.,0.)) ;
#19128=DIRECTION('center_axis',(0.,0.,-1.)) ;
#19129=DIRECTION('ref_axis',(1.,0.,0.)) ;
#19130=DIRECTION('center_axis',(0.,0.,-1.)) ;
#19131=DIRECTION('ref_axis',(0.,1.,0.)) ;
#19132=DIRECTION('center_axis',(0.,0.,-1.)) ;
#19133=DIRECTION('ref_axis',(1.,0.,0.)) ;
#19134=DIRECTION('',(0.,0.,1.)) ;
#19135=DIRECTION('center_axis',(0.,0.,1.)) ;
#19136=DIRECTION('ref_axis',(1.,0.,0.)) ;
#19137=DIRECTION('center_axis',(0.,0.,-1.)) ;
#19138=DIRECTION('ref_axis',(0.,1.,0.)) ;
#19139=DIRECTION('center_axis',(0.,0.,-1.)) ;
#19140=DIRECTION('ref_axis',(1.,0.,0.)) ;
#19141=DIRECTION('',(0.,0.,1.)) ;
#19142=DIRECTION('center_axis',(0.,0.,1.)) ;
#19143=DIRECTION('ref_axis',(1.,0.,0.)) ;
#23798=CARTESIAN_POINT('',(0.,0.,0.)) ;
#23799=CARTESIAN_POINT('Origin',(0.,0.,-328.125)) ;
#23800=CARTESIAN_POINT('',(-3.75195406107394E-8,-19.425,-318.731323220285)) ;
#23801=CARTESIAN_POINT('',(9.76712332682731E-9,-19.425,-318.518971385864)) ;
#23802=CARTESIAN_POINT('',(-2.37887640734373E-15,-19.425,-328.125)) ;
#23803=CARTESIAN_POINT('',(17.5361854501357,8.35622174666851,-318.250211755085)) ;
#23804=CARTESIAN_POINT('Ctrl Pts',(17.5359434890344,8.35591472846589,-318.250416135478)) ;
#23805=CARTESIAN_POINT('Ctrl Pts',(17.8361640444519,7.72586393628701,-318.258588076908)) ;
#23806=CARTESIAN_POINT('Ctrl Pts',(18.1022112467557,7.08008972097568,-318.266685027288)) ;
#23807=CARTESIAN_POINT('Ctrl Pts',(18.3886374715729,6.26235086001032,-318.277016532212)) ;
#23808=CARTESIAN_POINT('Ctrl Pts',(18.4422758795157,6.10258032632359,-318.279037530685)) ;
#23809=CARTESIAN_POINT('Ctrl Pts',(18.5317424236186,5.82413163966269,-318.282568096761)) ;
#23810=CARTESIAN_POINT('Ctrl Pts',(18.5685261696438,5.70577097810744,-318.284071416777)) ;
#23811=CARTESIAN_POINT('Ctrl Pts',(18.6384663337505,5.47287970534842,-318.287035700646)) ;
#23812=CARTESIAN_POINT('Ctrl Pts',(18.6717060340157,5.35837972543229,-318.288496034413)) ;
#23813=CARTESIAN_POINT('Ctrl Pts',(18.7405266390085,5.11289615809773,-318.291633941726)) ;
#23814=CARTESIAN_POINT('Ctrl Pts',(18.7757930869953,4.98183096105143,-318.293313533209)) ;
#23815=CARTESIAN_POINT('Ctrl Pts',(18.8670348664502,4.62799901878173,-318.297859564765)) ;
#23816=CARTESIAN_POINT('Ctrl Pts',(18.9204374156704,4.40459161454828,-318.300742488007)) ;
#23817=CARTESIAN_POINT('Ctrl Pts',(19.1395387183558,3.41032516101798,-318.313619447152)) ;
#23818=CARTESIAN_POINT('Ctrl Pts',(19.2621762184986,2.63074481189291,-318.323872053442)) ;
#23819=CARTESIAN_POINT('Ctrl Pts',(19.3564723693809,1.64291578597717,-318.336600535357)) ;
#23820=CARTESIAN_POINT('Ctrl Pts',(19.3726502454238,1.43965881836873,-318.339203483527)) ;
#23821=CARTESIAN_POINT('Ctrl Pts',(19.3923133935744,1.13130489355929,-318.343111699114)) ;
#23822=CARTESIAN_POINT('Ctrl Pts',(19.3981501515743,1.02637237507932,-318.344434517958)) ;
#23823=CARTESIAN_POINT('Ctrl Pts',(19.4034726746178,0.914288693855463,-318.345838106023)) ;
#23824=CARTESIAN_POINT('Ctrl Pts',(19.4038063482354,0.907179613167534,-318.345927090444)) ;
#23825=CARTESIAN_POINT('Ctrl Pts',(19.4043797672481,0.894817578832296,-318.346081755098)) ;
#23826=CARTESIAN_POINT('Ctrl Pts',(19.404621286705,0.889564708458132,-318.346147452837)) ;
#23827=CARTESIAN_POINT('Ctrl Pts',(19.4050409056885,0.88035681542777,-318.346262576645)) ;
#23828=CARTESIAN_POINT('Ctrl Pts',(19.405219929107,0.876401835293624,-318.346312011936)) ;
#23829=CARTESIAN_POINT('Ctrl Pts',(19.4055338043819,0.86942046457019,-318.346399252918)) ;
#23830=CARTESIAN_POINT('Ctrl Pts',(19.4056691573984,0.866394096712561,-318.346437063653)) ;
#23831=CARTESIAN_POINT('Ctrl Pts',(19.4059082495824,0.861020052690169,-318.346504192271)) ;
#23832=CARTESIAN_POINT('Ctrl Pts',(19.4060122706947,0.858672389210068,-318.346533513009)) ;
#23833=CARTESIAN_POINT('Ctrl Pts',(19.4064760354284,0.84816250658705,-318.346664753903)) ;
#23834=CARTESIAN_POINT('Ctrl Pts',(19.4068310555369,0.840000079229425,-318.346766625959)) ;
#23835=CARTESIAN_POINT('Ctrl Pts',(19.407500239987,0.824387673207127,-318.346961371011)) ;
#23836=CARTESIAN_POINT('Ctrl Pts',(19.4078152645099,0.816937732942163,-318.347054252894)) ;
#23837=CARTESIAN_POINT('Ctrl Pts',(19.4084142279498,0.802577095756465,-318.347233202422)) ;
#23838=CARTESIAN_POINT('Ctrl Pts',(19.40869876572,0.795666424998969,-318.347319276348)) ;
#23839=CARTESIAN_POINT('Ctrl Pts',(19.4092447198009,0.782232084142982,-318.347486523887)) ;
#23840=CARTESIAN_POINT('Ctrl Pts',(19.4095065381935,0.775708431318012,-318.347567701776)) ;
#23841=CARTESIAN_POINT('Ctrl Pts',(19.4100137933671,0.7629082489646,-318.347726909552)) ;
#23842=CARTESIAN_POINT('Ctrl Pts',(19.4102594748316,0.756631729946837,-318.347804942071)) ;
#23843=CARTESIAN_POINT('Ctrl Pts',(19.4107404722003,0.744189087075131,-318.347959565718)) ;
#23844=CARTESIAN_POINT('Ctrl Pts',(19.4109758944565,0.738022967989215,-318.348036158001)) ;
#23845=CARTESIAN_POINT('Ctrl Pts',(19.4137091817322,0.665527346705117,-318.34893626181)) ;
#23846=CARTESIAN_POINT('Ctrl Pts',(19.4158699937519,0.599185489183012,-318.349756037201)) ;
#23847=CARTESIAN_POINT('Ctrl Pts',(19.419423420364,0.469690434818989,-318.351347653963)) ;
#23848=CARTESIAN_POINT('Ctrl Pts',(19.4208481061199,0.406538970002123,-318.352119923812)) ;
#23849=CARTESIAN_POINT('Ctrl Pts',(19.4240711038294,0.224243411802522,-318.35433919791)) ;
#23850=CARTESIAN_POINT('Ctrl Pts',(19.4250812068003,0.105088182032955,-318.355777493511)) ;
#23851=CARTESIAN_POINT('Ctrl Pts',(19.4246389057749,-0.505599037037676,
-318.363101020354)) ;
#23852=CARTESIAN_POINT('Ctrl Pts',(19.4056265118234,-0.996939939709481,
-318.368838635994)) ;
#23853=CARTESIAN_POINT('Ctrl Pts',(19.3340458606877,-1.92925034319463,-318.379759743753)) ;
#23854=CARTESIAN_POINT('Ctrl Pts',(19.2849577239435,-2.37017749952631,-318.384938958872)) ;
#23855=CARTESIAN_POINT('Ctrl Pts',(19.1907765657816,-3.01461168345414,-318.392653256337)) ;
#23856=CARTESIAN_POINT('Ctrl Pts',(19.1574365658758,-3.21969142248208,-318.395129309198)) ;
#23857=CARTESIAN_POINT('Ctrl Pts',(19.091327592596,-3.58884584990186,-318.399634297491)) ;
#23858=CARTESIAN_POINT('Ctrl Pts',(19.0597164221864,-3.75310719037178,-318.401656097661)) ;
#23859=CARTESIAN_POINT('Ctrl Pts',(19.0042060176744,-4.02274123847243,-318.405006281912)) ;
#23860=CARTESIAN_POINT('Ctrl Pts',(18.9815421653682,-4.12835929006944,-318.406326541001)) ;
#23861=CARTESIAN_POINT('Ctrl Pts',(18.930433014569,-4.35721543798472,-318.409205254106)) ;
#23862=CARTESIAN_POINT('Ctrl Pts',(18.9016626882452,-4.48037588405983,-318.410765808215)) ;
#23863=CARTESIAN_POINT('Ctrl Pts',(18.834800682221,-4.7544865949519,-318.414264842707)) ;
#23864=CARTESIAN_POINT('Ctrl Pts',(18.7960929691439,-4.90527761966604,-318.416207281625)) ;
#23865=CARTESIAN_POINT('Ctrl Pts',(18.6123990748495,-5.58675833213696,-318.425064621203)) ;
#23866=CARTESIAN_POINT('Ctrl Pts',(18.4467215570834,-6.11160604010705,-318.432111733988)) ;
#23867=CARTESIAN_POINT('Ctrl Pts',(18.0783812130823,-7.12621109985498,-318.446026883841)) ;
#23868=CARTESIAN_POINT('Ctrl Pts',(17.877512153499,-7.61612181226138,-318.452884693635)) ;
#23869=CARTESIAN_POINT('Ctrl Pts',(17.5869727219576,-8.24967559074662,-318.461730250758)) ;
#23870=CARTESIAN_POINT('Ctrl Pts',(17.5150853350643,-8.40122269285768,-318.463843721782)) ;
#23871=CARTESIAN_POINT('Ctrl Pts',(17.4064633805098,-8.62275472449833,-318.466919799804)) ;
#23872=CARTESIAN_POINT('Ctrl Pts',(17.3712500550719,-8.69347674990476,-318.467899764193)) ;
#23873=CARTESIAN_POINT('Ctrl Pts',(17.3056289315658,-8.82327869990995,-318.469693205862)) ;
#23874=CARTESIAN_POINT('Ctrl Pts',(17.2753476360861,-8.88242105382913,-318.470508222507)) ;
#23875=CARTESIAN_POINT('Ctrl Pts',(17.1994145935773,-9.02886862829517,-318.472521891028)) ;
#23876=CARTESIAN_POINT('Ctrl Pts',(17.1534009480539,-9.11598414992153,-318.473715902887)) ;
#23877=CARTESIAN_POINT('Ctrl Pts',(16.9577496167712,-9.47967492743655,-318.478691632871)) ;
#23878=CARTESIAN_POINT('Ctrl Pts',(16.8020697987869,-9.75294622576759,-318.482408942612)) ;
#23879=CARTESIAN_POINT('Ctrl Pts',(16.5426809640306,-10.1836035601808,-318.488311133754)) ;
#23880=CARTESIAN_POINT('Ctrl Pts',(16.4431973381435,-10.3434682917478,-318.490511919025)) ;
#23881=CARTESIAN_POINT('Ctrl Pts',(16.0911232605261,-10.8913126181413,-318.498118923141)) ;
#23882=CARTESIAN_POINT('Ctrl Pts',(15.8269989726428,-11.2716920415504,-318.503518932264)) ;
#23883=CARTESIAN_POINT('Ctrl Pts',(15.4633360303461,-11.7574040645809,-318.510701428245)) ;
#23884=CARTESIAN_POINT('Ctrl Pts',(15.3758574189166,-11.8715761424008,-318.512411095488)) ;
#23885=CARTESIAN_POINT('Ctrl Pts',(15.1547786925007,-12.1535722008268,-318.516692273301)) ;
#23886=CARTESIAN_POINT('Ctrl Pts',(15.0196516279904,-12.3201744801037,-318.519274310003)) ;
#23887=CARTESIAN_POINT('Ctrl Pts',(14.7964408248314,-12.5862464781808,-318.523491569587)) ;
#23888=CARTESIAN_POINT('Ctrl Pts',(14.7100472522316,-12.687110438287,-318.525112693334)) ;
#23889=CARTESIAN_POINT('Ctrl Pts',(14.5395638958167,-12.8820661524688,-318.528291319787)) ;
#23890=CARTESIAN_POINT('Ctrl Pts',(14.4555780735056,-12.9762401776811,-318.529847886303)) ;
#23891=CARTESIAN_POINT('Ctrl Pts',(14.267065028334,-13.1835198982721,-318.533321653275)) ;
#23892=CARTESIAN_POINT('Ctrl Pts',(14.162098234109,-13.2962143090171,-318.535242593247)) ;
#23893=CARTESIAN_POINT('Ctrl Pts',(13.6772898161035,-13.8044593913075,-318.54405376234)) ;
#23894=CARTESIAN_POINT('Ctrl Pts',(13.2821443593885,-14.1850623421511,-318.551075665434)) ;
#23895=CARTESIAN_POINT('Ctrl Pts',(12.4755358261488,-14.8986926287413,-318.564956089729)) ;
#23896=CARTESIAN_POINT('Ctrl Pts',(12.0655115682462,-15.2326447829125,-318.57180454189)) ;
#23897=CARTESIAN_POINT('Ctrl Pts',(11.505796574595,-15.6517214019043,-318.580680703614)) ;
#23898=CARTESIAN_POINT('Ctrl Pts',(11.3678723738325,-15.7521812937659,-318.582831255241)) ;
#23899=CARTESIAN_POINT('Ctrl Pts',(11.1637120153642,-15.8968075622017,-318.585950979884)) ;
#23900=CARTESIAN_POINT('Ctrl Pts',(11.0984995132176,-15.942404624404,-318.586938120349)) ;
#23901=CARTESIAN_POINT('Ctrl Pts',(10.9783446230289,-16.0253232590335,-318.588738433228)) ;
#23902=CARTESIAN_POINT('Ctrl Pts',(10.9234876020961,-16.0627661010884,-318.589553224272)) ;
#23903=CARTESIAN_POINT('Ctrl Pts',(10.787308577303,-16.1546953073578,-318.591559071098)) ;
#23904=CARTESIAN_POINT('Ctrl Pts',(10.7057646774855,-16.2088497285502,-318.592745594856)) ;
#23905=CARTESIAN_POINT('Ctrl Pts',(10.3667465054018,-16.4303219284505,-318.597625436801)) ;
#23906=CARTESIAN_POINT('Ctrl Pts',(10.1057316969341,-16.5921396875327,-318.601257392169)) ;
#23907=CARTESIAN_POINT('Ctrl Pts',(9.47635769564765,-16.9619613836531,-318.609831168774)) ;
#23908=CARTESIAN_POINT('Ctrl Pts',(9.10482459956954,-17.1642552598683,-318.614749280166)) ;
#23909=CARTESIAN_POINT('Ctrl Pts',(8.29507997240903,-17.5714537898474,-318.62536471977)) ;
#23910=CARTESIAN_POINT('Ctrl Pts',(7.85521804294205,-17.7724474425252,-318.631070562401)) ;
#23911=CARTESIAN_POINT('Ctrl Pts',(7.25416743233182,-18.0204186077575,-318.638897510944)) ;
#23912=CARTESIAN_POINT('Ctrl Pts',(7.09920454975442,-18.0820277233927,-318.64091754488)) ;
#23913=CARTESIAN_POINT('Ctrl Pts',(6.82669164795596,-18.1863283928655,-318.644476427079)) ;
#23914=CARTESIAN_POINT('Ctrl Pts',(6.70948677342134,-18.2298943074088,-318.646009128314)) ;
#23915=CARTESIAN_POINT('Ctrl Pts',(6.46080727354764,-18.3196071804636,-318.649266252274)) ;
#23916=CARTESIAN_POINT('Ctrl Pts',(6.32924021215035,-18.3654772914714,-318.650992475406)) ;
#23917=CARTESIAN_POINT('Ctrl Pts',(5.96577894148348,-18.4878264385583,-318.655769724322)) ;
#23918=CARTESIAN_POINT('Ctrl Pts',(5.73291888797409,-18.5613546244059,-318.658840020083)) ;
#23919=CARTESIAN_POINT('Ctrl Pts',(5.29162843691991,-18.6916003365817,-318.664671321594)) ;
#23920=CARTESIAN_POINT('Ctrl Pts',(5.08351716581555,-18.7492695245115,-318.667426575661)) ;
#23921=CARTESIAN_POINT('Ctrl Pts',(4.30906359933547,-18.9500339164173,-318.677682130067)) ;
#23922=CARTESIAN_POINT('Ctrl Pts',(3.73731666048703,-19.0710324107846,-318.685266965197)) ;
#23923=CARTESIAN_POINT('Ctrl Pts',(2.89879228028493,-19.2093270458025,-318.696150089002)) ;
#23924=CARTESIAN_POINT('Ctrl Pts',(2.6357350103506,-19.247185343998,-318.699528560866)) ;
#23925=CARTESIAN_POINT('Ctrl Pts',(2.28062245314534,-19.290875030694,-318.704007561273)) ;
#23926=CARTESIAN_POINT('Ctrl Pts',(2.18918235324355,-19.3014657184243,-318.705153577779)) ;
#23927=CARTESIAN_POINT('Ctrl Pts',(2.03837205828987,-19.3178472436615,-318.707029707136)) ;
#23928=CARTESIAN_POINT('Ctrl Pts',(1.97904441178138,-19.324015266403,-318.707764148417)) ;
#23929=CARTESIAN_POINT('Ctrl Pts',(1.84031778419984,-19.3377924643283,-318.709472733874)) ;
#23930=CARTESIAN_POINT('Ctrl Pts',(1.7608985974158,-19.3451860443713,-318.710444365842)) ;
#23931=CARTESIAN_POINT('Ctrl Pts',(1.51018394198892,-19.3669697720635,-318.713494019274)) ;
#23932=CARTESIAN_POINT('Ctrl Pts',(1.33874158295967,-19.3795754553743,-318.715553508113)) ;
#23933=CARTESIAN_POINT('Ctrl Pts',(0.778478482824912,-19.4132998882475,
-318.722227322384)) ;
#23934=CARTESIAN_POINT('Ctrl Pts',(0.389251165707532,-19.4250000007518,
-318.726776673746)) ;
#23935=CARTESIAN_POINT('Ctrl Pts',(-3.75195408075513E-8,-19.425,-318.731323220285)) ;
#23936=CARTESIAN_POINT('',(17.5359809117572,-8.35583619169778,-318.25)) ;
#23937=CARTESIAN_POINT('Origin',(0.,0.,-318.25)) ;
#23938=CARTESIAN_POINT('Ctrl Pts',(17.5359809117572,-8.35583619169781,-318.25)) ;
#23939=CARTESIAN_POINT('Ctrl Pts',(17.5198792059969,-8.38962804668179,-318.250460037632)) ;
#23940=CARTESIAN_POINT('Ctrl Pts',(17.5036798636303,-8.42337327821063,-318.250921300259)) ;
#23941=CARTESIAN_POINT('Ctrl Pts',(17.4683361610756,-8.49645636247359,-318.251924139912)) ;
#23942=CARTESIAN_POINT('Ctrl Pts',(17.4491562426748,-8.53577678780645,-318.252466131549)) ;
#23943=CARTESIAN_POINT('Ctrl Pts',(17.3747570462932,-8.68700262016844,-318.254559570065)) ;
#23944=CARTESIAN_POINT('Ctrl Pts',(17.318592799099,-8.79843965357187,-318.2561211156)) ;
#23945=CARTESIAN_POINT('Ctrl Pts',(16.9574819793595,-9.49807307940423,-318.266027876778)) ;
#23946=CARTESIAN_POINT('Ctrl Pts',(16.6236830848865,-10.0708862132213,-318.274585351295)) ;
#23947=CARTESIAN_POINT('Ctrl Pts',(16.0460907785041,-10.9548319601542,-318.288061387794)) ;
#23948=CARTESIAN_POINT('Ctrl Pts',(15.8209570947634,-11.2775303285937,-318.293046457475)) ;
#23949=CARTESIAN_POINT('Ctrl Pts',(15.5094952734983,-11.6962682575552,-318.299568971753)) ;
#23950=CARTESIAN_POINT('Ctrl Pts',(15.4317888945073,-11.798602728926,-318.301167631723)) ;
#23951=CARTESIAN_POINT('Ctrl Pts',(15.2792878999389,-11.9953529513281,-318.304249729324)) ;
#23952=CARTESIAN_POINT('Ctrl Pts',(15.2046191254482,-12.0898589093431,-318.305734047246)) ;
#23953=CARTESIAN_POINT('Ctrl Pts',(15.05458867922,-12.2761593510363,-318.308667868868)) ;
#23954=CARTESIAN_POINT('Ctrl Pts',(14.9792544271018,-12.3679693386124,-318.310117507856)) ;
#23955=CARTESIAN_POINT('Ctrl Pts',(14.774242130377,-12.6131972834278,-318.314000571655)) ;
#23956=CARTESIAN_POINT('Ctrl Pts',(14.6430183721534,-12.76530412388,-318.316420816178)) ;
#23957=CARTESIAN_POINT('Ctrl Pts',(14.11937145961,-13.3535835191081,-318.325837903387)) ;
#23958=CARTESIAN_POINT('Ctrl Pts',(13.7096294855631,-13.7739211730652,-318.3326820739)) ;
#23959=CARTESIAN_POINT('Ctrl Pts',(12.9412265317647,-14.4938851277888,-318.34489605397)) ;
#23960=CARTESIAN_POINT('Ctrl Pts',(12.58959139021,-14.8003458594248,-318.350279025558)) ;
#23961=CARTESIAN_POINT('Ctrl Pts',(12.097352808699,-15.1990998134531,-318.35772399782)) ;
#23962=CARTESIAN_POINT('Ctrl Pts',(11.9660813985514,-15.302662381079,-318.359701577825)) ;
#23963=CARTESIAN_POINT('Ctrl Pts',(11.7781452047365,-15.4470317870343,-318.362532484224)) ;
#23964=CARTESIAN_POINT('Ctrl Pts',(11.7225721416481,-15.4892478146926,-318.363369557972)) ;
#23965=CARTESIAN_POINT('Ctrl Pts',(11.6116381886808,-15.5725797064156,-318.365041613266)) ;
#23966=CARTESIAN_POINT('Ctrl Pts',(11.5562834452924,-15.6137020932165,-318.365876489156)) ;
#23967=CARTESIAN_POINT('Ctrl Pts',(11.4523687553509,-15.6900437593506,-318.367445857157)) ;
#23968=CARTESIAN_POINT('Ctrl Pts',(11.4038623722044,-15.725334536324,-318.368179319703)) ;
#23969=CARTESIAN_POINT('Ctrl Pts',(11.2982164897377,-15.801451220993,-318.369779202226)) ;
#23970=CARTESIAN_POINT('Ctrl Pts',(11.2410176229562,-15.8421930086534,-318.370646780637)) ;
#23971=CARTESIAN_POINT('Ctrl Pts',(11.0868475315197,-15.9507504192236,-318.372987401497)) ;
#23972=CARTESIAN_POINT('Ctrl Pts',(10.9894755363776,-16.017991587524,-318.374468024141)) ;
#23973=CARTESIAN_POINT('Ctrl Pts',(10.5266240762749,-16.3314110326398,-318.381505375013)) ;
#23974=CARTESIAN_POINT('Ctrl Pts',(10.1534516232657,-16.5659958926339,-318.387174199619)) ;
#23975=CARTESIAN_POINT('Ctrl Pts',(9.3715428916209,-17.0211688971527,-318.398831704899)) ;
#23976=CARTESIAN_POINT('Ctrl Pts',(8.962220594579,-17.2402033077897,-318.404816939237)) ;
#23977=CARTESIAN_POINT('Ctrl Pts',(8.35539662660272,-17.5374672915959,-318.413419660947)) ;
#23978=CARTESIAN_POINT('Ctrl Pts',(8.16383713678824,-17.6274551535937,-318.416098111544)) ;
#23979=CARTESIAN_POINT('Ctrl Pts',(7.86067880717831,-17.7638663493227,-318.420274185247)) ;
#23980=CARTESIAN_POINT('Ctrl Pts',(7.75005213757438,-17.8124089020029,-318.421785206438)) ;
#23981=CARTESIAN_POINT('Ctrl Pts',(7.60390051266738,-17.8749203541796,-318.423764273037)) ;
#23982=CARTESIAN_POINT('Ctrl Pts',(7.56877710392898,-17.889820955705,-318.424238590433)) ;
#23983=CARTESIAN_POINT('Ctrl Pts',(7.42632280512932,-17.9497605273382,-318.426157089413)) ;
#23984=CARTESIAN_POINT('Ctrl Pts',(7.31863194284603,-17.9939378658013,-318.427595353699)) ;
#23985=CARTESIAN_POINT('Ctrl Pts',(7.09350300785435,-18.0839356773858,-318.430577222018)) ;
#23986=CARTESIAN_POINT('Ctrl Pts',(6.97600279352915,-18.1295863046937,-318.432119592422)) ;
#23987=CARTESIAN_POINT('Ctrl Pts',(6.68748025904288,-18.2384614516959,-318.435873898971)) ;
#23988=CARTESIAN_POINT('Ctrl Pts',(6.51599603297857,-18.300427977921,-318.43807711471)) ;
#23989=CARTESIAN_POINT('Ctrl Pts',(5.68044058268022,-18.5891257963158,-318.448687554087)) ;
#23990=CARTESIAN_POINT('Ctrl Pts',(5.00528602135639,-18.7821754793875,-318.456860865535)) ;
#23991=CARTESIAN_POINT('Ctrl Pts',(3.89849440260567,-19.0347136373014,-318.470116949714)) ;
#23992=CARTESIAN_POINT('Ctrl Pts',(3.47270829007892,-19.1169787680542,-318.475189009329)) ;
#23993=CARTESIAN_POINT('Ctrl Pts',(2.92407062282469,-19.2040441445099,-318.481844724358)) ;
#23994=CARTESIAN_POINT('Ctrl Pts',(2.80343553201976,-19.2220251186595,-318.483315786842)) ;
#23995=CARTESIAN_POINT('Ctrl Pts',(2.61309447505108,-19.2485659928119,-318.485653829477)) ;
#23996=CARTESIAN_POINT('Ctrl Pts',(2.54349761241096,-19.2578860576797,-318.486512290162)) ;
#23997=CARTESIAN_POINT('Ctrl Pts',(2.40300201308118,-19.2759256267124,-318.488253724751)) ;
#23998=CARTESIAN_POINT('Ctrl Pts',(2.33210269302313,-19.2846318205587,-318.489136781985)) ;
#23999=CARTESIAN_POINT('Ctrl Pts',(2.13717099809704,-19.3074780543583,-318.491574837144)) ;
#24000=CARTESIAN_POINT('Ctrl Pts',(2.01304789948299,-19.320813822877,-318.493138550738)) ;
#24001=CARTESIAN_POINT('Ctrl Pts',(1.58957877219779,-19.362186222767,-318.498502211751)) ;
#24002=CARTESIAN_POINT('Ctrl Pts',(1.28971446400269,-19.3844693528092,-318.502348628073)) ;
#24003=CARTESIAN_POINT('Ctrl Pts',(0.934551723804926,-19.4025838549164,
-318.506921303889)) ;
#24004=CARTESIAN_POINT('Ctrl Pts',(0.879637174321103,-19.4051510071819,
-318.507628821915)) ;
#24005=CARTESIAN_POINT('Ctrl Pts',(0.735946097340056,-19.4112570958334,
-318.509480978891)) ;
#24006=CARTESIAN_POINT('Ctrl Pts',(0.647154892522766,-19.4144201366001,
-318.51062632345)) ;
#24007=CARTESIAN_POINT('Ctrl Pts',(0.372263752904269,-19.4223247735594,
-318.514172668865)) ;
#24008=CARTESIAN_POINT('Ctrl Pts',(0.18612948495482,-19.4249999999064,-318.516574511693)) ;
#24009=CARTESIAN_POINT('Ctrl Pts',(9.76712256212098E-9,-19.425,-318.518971385864)) ;
#24010=CARTESIAN_POINT('Origin',(0.,0.,-328.125)) ;
#24011=CARTESIAN_POINT('',(-0.000449417202212064,-19.4250824346375,-320.231292904519)) ;
#24012=CARTESIAN_POINT('',(-0.000295851126506864,-19.4249999967644,-320.018354299106)) ;
#24013=CARTESIAN_POINT('',(-2.37887640734373E-15,-19.425,-328.125)) ;
#24014=CARTESIAN_POINT('Ctrl Pts',(-3.75195408769402E-8,-19.425,-318.731323220285)) ;
#24015=CARTESIAN_POINT('Ctrl Pts',(-0.286007459534617,-19.4249999994476,
-318.734663854929)) ;
#24016=CARTESIAN_POINT('Ctrl Pts',(-0.572027782392097,-19.4186833807807,
-318.738002522882)) ;
#24017=CARTESIAN_POINT('Ctrl Pts',(-1.14627823685766,-19.393298418784,-318.744751765226)) ;
#24018=CARTESIAN_POINT('Ctrl Pts',(-1.43438419233051,-19.3741198251488,
-318.748161338625)) ;
#24019=CARTESIAN_POINT('Ctrl Pts',(-1.94585854290658,-19.3286002949899,
-318.754288319144)) ;
#24020=CARTESIAN_POINT('Ctrl Pts',(-2.16939892445428,-19.3047886001703,
-318.756991228773)) ;
#24021=CARTESIAN_POINT('Ctrl Pts',(-2.52608639503362,-19.2605202271534,
-318.761352659256)) ;
#24022=CARTESIAN_POINT('Ctrl Pts',(-2.65952133422362,-19.2425491583177,
-318.762995115991)) ;
#24023=CARTESIAN_POINT('Ctrl Pts',(-2.91804790595291,-19.2049902411333,
-318.76619964914)) ;
#24024=CARTESIAN_POINT('Ctrl Pts',(-3.04315622115263,-19.1855636849058,
-318.767760595865)) ;
#24025=CARTESIAN_POINT('Ctrl Pts',(-3.34410870049375,-19.13581459057,-318.771540576724)) ;
#24026=CARTESIAN_POINT('Ctrl Pts',(-3.51974228862563,-19.1042894956005,
-318.773767293134)) ;
#24027=CARTESIAN_POINT('Ctrl Pts',(-4.41580901212489,-18.9306748653615,
-318.785231997198)) ;
#24028=CARTESIAN_POINT('Ctrl Pts',(-5.12819980772471,-18.7502367586556,
-318.794718262101)) ;
#24029=CARTESIAN_POINT('Ctrl Pts',(-6.21820311983242,-18.407371765267,-318.809451024768)) ;
#24030=CARTESIAN_POINT('Ctrl Pts',(-6.60378877473305,-18.2725849320413,
-318.814700814828)) ;
#24031=CARTESIAN_POINT('Ctrl Pts',(-7.09646490993294,-18.0827299214219,
-318.821351819026)) ;
#24032=CARTESIAN_POINT('Ctrl Pts',(-7.20769100613827,-18.0386841552426,
-318.822849343208)) ;
#24033=CARTESIAN_POINT('Ctrl Pts',(-7.38344274293308,-17.9672010350083,
-318.82520527028)) ;
#24034=CARTESIAN_POINT('Ctrl Pts',(-7.44823886926803,-17.9404369384148,
-318.82607159725)) ;
#24035=CARTESIAN_POINT('Ctrl Pts',(-7.57068731491574,-17.889081778305,-318.82770344851)) ;
#24036=CARTESIAN_POINT('Ctrl Pts',(-7.62836824756348,-17.8645613207162,
-318.828469946132)) ;
#24037=CARTESIAN_POINT('Ctrl Pts',(-7.79288254156359,-17.7936833985481,
-318.830651070199)) ;
#24038=CARTESIAN_POINT('Ctrl Pts',(-7.89941913751624,-17.7466437543245,
-318.832057440686)) ;
#24039=CARTESIAN_POINT('Ctrl Pts',(-8.32919216631633,-17.5522470329059,
-318.837717218088)) ;
#24040=CARTESIAN_POINT('Ctrl Pts',(-8.64878179349487,-17.3969937795925,
-318.841895786816)) ;
#24041=CARTESIAN_POINT('Ctrl Pts',(-9.58321805118889,-16.9109382977038,
-318.85422563345)) ;
#24042=CARTESIAN_POINT('Ctrl Pts',(-10.1846887237055,-16.5556642431838,
-318.862326688989)) ;
#24043=CARTESIAN_POINT('Ctrl Pts',(-10.9534643882013,-16.0437873841392,
-318.873345983863)) ;
#24044=CARTESIAN_POINT('Ctrl Pts',(-11.1390100224788,-15.9155254769109,
-318.876057792405)) ;
#24045=CARTESIAN_POINT('Ctrl Pts',(-11.4318026969099,-15.705498387101,-318.880430034651)) ;
#24046=CARTESIAN_POINT('Ctrl Pts',(-11.540504887464,-15.6257972395733,-318.882074260238)) ;
#24047=CARTESIAN_POINT('Ctrl Pts',(-11.7496542862082,-15.4690745761243,
-318.885280056272)) ;
#24048=CARTESIAN_POINT('Ctrl Pts',(-11.8501956218692,-15.3921898299445,
-318.886840472017)) ;
#24049=CARTESIAN_POINT('Ctrl Pts',(-12.0903676936717,-15.2047802985234,
-318.890615372731)) ;
#24050=CARTESIAN_POINT('Ctrl Pts',(-12.2292439161095,-15.0933073910411,
-318.892837481342)) ;
#24051=CARTESIAN_POINT('Ctrl Pts',(-12.6698705757445,-14.72955165818,-318.90001399427)) ;
#24052=CARTESIAN_POINT('Ctrl Pts',(-12.9654982953675,-14.4700091632262,
-318.905024752178)) ;
#24053=CARTESIAN_POINT('Ctrl Pts',(-13.6543603084029,-13.8271611091469,
-318.917123217825)) ;
#24054=CARTESIAN_POINT('Ctrl Pts',(-14.0396227635746,-13.435807810924,-318.924246579844)) ;
#24055=CARTESIAN_POINT('Ctrl Pts',(-14.4943566837919,-12.9329388101128,
-318.932924486614)) ;
#24056=CARTESIAN_POINT('Ctrl Pts',(-14.5799644230022,-12.8363514837939,
-318.934570405797)) ;
#24057=CARTESIAN_POINT('Ctrl Pts',(-14.7717783066041,-12.6155419555065,
-318.93828005332)) ;
#24058=CARTESIAN_POINT('Ctrl Pts',(-14.8773922409784,-12.4908179645103,
-318.940338213387)) ;
#24059=CARTESIAN_POINT('Ctrl Pts',(-15.0312891342176,-12.3043532871932,
-318.943351536856)) ;
#24060=CARTESIAN_POINT('Ctrl Pts',(-15.0807924992862,-12.2436293829311,
-318.944323056544)) ;
#24061=CARTESIAN_POINT('Ctrl Pts',(-15.1717600805074,-12.130654154376,-318.946111130847)) ;
#24062=CARTESIAN_POINT('Ctrl Pts',(-15.2133250264288,-12.0784856577575,
-318.946929098896)) ;
#24063=CARTESIAN_POINT('Ctrl Pts',(-15.3166239120342,-11.9474552520882,
-318.948965292312)) ;
#24064=CARTESIAN_POINT('Ctrl Pts',(-15.3780182482045,-11.8683280145292,
-318.950178634034)) ;
#24065=CARTESIAN_POINT('Ctrl Pts',(-15.6676038787213,-11.4890798474374,
-318.955925392695)) ;
#24066=CARTESIAN_POINT('Ctrl Pts',(-15.8876381157418,-11.1828316396753,
-318.960364475648)) ;
#24067=CARTESIAN_POINT('Ctrl Pts',(-16.2606980124245,-10.6303437739049,
-318.968170767709)) ;
#24068=CARTESIAN_POINT('Ctrl Pts',(-16.417386715422,-10.386718544207,-318.971546590227)) ;
#24069=CARTESIAN_POINT('Ctrl Pts',(-16.7564710752746,-9.83264365093919,
-318.979143420769)) ;
#24070=CARTESIAN_POINT('Ctrl Pts',(-16.9358015468594,-9.52044271824114,
-318.983369685163)) ;
#24071=CARTESIAN_POINT('Ctrl Pts',(-17.2294095101058,-8.97471617269769,
-318.990734379051)) ;
#24072=CARTESIAN_POINT('Ctrl Pts',(-17.3478660158323,-8.74354772326497,
-318.993846875203)) ;
#24073=CARTESIAN_POINT('Ctrl Pts',(-17.5233251881918,-8.38352654107101,
-318.998697116442)) ;
#24074=CARTESIAN_POINT('Ctrl Pts',(-17.583621526928,-8.25631254541748,-319.00041140313)) ;
#24075=CARTESIAN_POINT('Ctrl Pts',(-17.6947151141119,-8.01518775241271,
-319.003663016634)) ;
#24076=CARTESIAN_POINT('Ctrl Pts',(-17.7458085444244,-7.90142118440228,
-319.005198129967)) ;
#24077=CARTESIAN_POINT('Ctrl Pts',(-17.8603827240459,-7.63958802068494,
-319.008733909052)) ;
#24078=CARTESIAN_POINT('Ctrl Pts',(-17.9231241475552,-7.49120797109105,
-319.010739625042)) ;
#24079=CARTESIAN_POINT('Ctrl Pts',(-18.1466380638239,-6.94372205674883,
-319.0181469038)) ;
#24080=CARTESIAN_POINT('Ctrl Pts',(-18.2959833775576,-6.54008712519531,
-319.02362366026)) ;
#24081=CARTESIAN_POINT('Ctrl Pts',(-18.6052207054103,-5.61054354314534,
-319.036202366919)) ;
#24082=CARTESIAN_POINT('Ctrl Pts',(-18.7564471686972,-5.08213784282851,
-319.043331739021)) ;
#24083=CARTESIAN_POINT('Ctrl Pts',(-18.915303677657,-4.42250862607873,-319.0520162424)) ;
#24084=CARTESIAN_POINT('Ctrl Pts',(-18.944281581646,-4.29668374092105,-319.053662866711)) ;
#24085=CARTESIAN_POINT('Ctrl Pts',(-19.0070998763694,-4.01092274747163,
-319.0573737716)) ;
#24086=CARTESIAN_POINT('Ctrl Pts',(-19.0401801607921,-3.85082933730122,
-319.05943248372)) ;
#24087=CARTESIAN_POINT('Ctrl Pts',(-19.0861197738805,-3.61341873825023,
-319.062446363266)) ;
#24088=CARTESIAN_POINT('Ctrl Pts',(-19.1005382664594,-3.53641074437951,
-319.063417899645)) ;
#24089=CARTESIAN_POINT('Ctrl Pts',(-19.1263680184581,-3.39368821649319,
-319.065205913583)) ;
#24090=CARTESIAN_POINT('Ctrl Pts',(-19.1379074354898,-3.32799823764049,
-319.066023805766)) ;
#24091=CARTESIAN_POINT('Ctrl Pts',(-19.165922711895,-3.16355113880511,-319.068059572948)) ;
#24092=CARTESIAN_POINT('Ctrl Pts',(-19.1819737961618,-3.06472356481236,
-319.06927256835)) ;
#24093=CARTESIAN_POINT('Ctrl Pts',(-19.2545953664382,-2.59464926943222,
-319.075001102468)) ;
#24094=CARTESIAN_POINT('Ctrl Pts',(-19.3011565997644,-2.22193672053857,
-319.079423081229)) ;
#24095=CARTESIAN_POINT('Ctrl Pts',(-19.3770393798232,-1.4279701314104,-319.088763113019)) ;
#24096=CARTESIAN_POINT('Ctrl Pts',(-19.4034904314886,-1.00663452578914,
-319.093673030672)) ;
#24097=CARTESIAN_POINT('Ctrl Pts',(-19.4248948166236,-0.295944930719285,
-319.102021365853)) ;
#24098=CARTESIAN_POINT('Ctrl Pts',(-19.4271478415352,-0.0069595709563066,
-319.10543382954)) ;
#24099=CARTESIAN_POINT('Ctrl Pts',(-19.4196884454123,0.506870156982208,
-319.11156535498)) ;
#24100=CARTESIAN_POINT('Ctrl Pts',(-19.4125174538411,0.731698390769262,
-319.114269886848)) ;
#24101=CARTESIAN_POINT('Ctrl Pts',(-19.3948134566833,1.09085846674695,-319.118633375426)) ;
#24102=CARTESIAN_POINT('Ctrl Pts',(-19.3867846151373,1.22529320652801,-319.120276243922)) ;
#24103=CARTESIAN_POINT('Ctrl Pts',(-19.3684965380784,1.48593303008581,-319.123481250528)) ;
#24104=CARTESIAN_POINT('Ctrl Pts',(-19.3584000000183,1.61214283027296,-319.125042255054)) ;
#24105=CARTESIAN_POINT('Ctrl Pts',(-19.3336303569957,1.88783473977934,-319.128472339184)) ;
#24106=CARTESIAN_POINT('Ctrl Pts',(-19.318455932172,2.03726363082032,-319.130344543198)) ;
#24107=CARTESIAN_POINT('Ctrl Pts',(-19.25314781647,2.61377727702371,-319.137617418963)) ;
#24108=CARTESIAN_POINT('Ctrl Pts',(-19.1905711747549,3.03932703729421,-319.143094303266)) ;
#24109=CARTESIAN_POINT('Ctrl Pts',(-19.0173764027594,3.9954228492101,-319.155574852306)) ;
#24110=CARTESIAN_POINT('Ctrl Pts',(-18.8985791057416,4.52412599122849,-319.162602881702)) ;
#24111=CARTESIAN_POINT('Ctrl Pts',(-18.724527504751,5.170989811772,-319.171176061958)) ;
#24112=CARTESIAN_POINT('Ctrl Pts',(-18.6899865524383,5.29447529288879,-319.172811095647)) ;
#24113=CARTESIAN_POINT('Ctrl Pts',(-18.6088454376086,5.57386504444546,-319.176500694777)) ;
#24114=CARTESIAN_POINT('Ctrl Pts',(-18.5615038098253,5.72954418035052,-319.178549686023)) ;
#24115=CARTESIAN_POINT('Ctrl Pts',(-18.4885163252147,5.95915323007896,-319.181552393243)) ;
#24116=CARTESIAN_POINT('Ctrl Pts',(-18.4643707752617,6.03355243794713,-319.182522309887)) ;
#24117=CARTESIAN_POINT('Ctrl Pts',(-18.4187930541865,6.17115394140327,-319.184309172572)) ;
#24118=CARTESIAN_POINT('Ctrl Pts',(-18.3974833250131,6.23439538672314,-319.185127510836)) ;
#24119=CARTESIAN_POINT('Ctrl Pts',(-18.3433008693072,6.39249693441792,-319.187166994278)) ;
#24120=CARTESIAN_POINT('Ctrl Pts',(-18.310017830893,6.48721441840174,-319.188383218009)) ;
#24121=CARTESIAN_POINT('Ctrl Pts',(-18.1531698348957,6.92275044755156,-319.193958018758)) ;
#24122=CARTESIAN_POINT('Ctrl Pts',(-18.0208131590611,7.26032665209868,-319.198229971217)) ;
#24123=CARTESIAN_POINT('Ctrl Pts',(-17.8384470777989,7.6896838442158,-319.203694955434)) ;
#24124=CARTESIAN_POINT('Ctrl Pts',(-17.7970392699325,7.78503853579107,-319.204910594097)) ;
#24125=CARTESIAN_POINT('Ctrl Pts',(-17.5584583825457,8.32259461867351,-319.211783085014)) ;
#24126=CARTESIAN_POINT('Ctrl Pts',(-17.345572051133,8.75763506388627,-319.217424338588)) ;
#24127=CARTESIAN_POINT('Ctrl Pts',(-16.9707337335858,9.45621874933345,-319.226803067271)) ;
#24128=CARTESIAN_POINT('Ctrl Pts',(-16.818351950779,9.72465493470311,-319.230486730623)) ;
#24129=CARTESIAN_POINT('Ctrl Pts',(-16.5832574868462,10.1167315595443,-319.236011605052)) ;
#24130=CARTESIAN_POINT('Ctrl Pts',(-16.5054168849176,10.2432367785327,-319.237816995416)) ;
#24131=CARTESIAN_POINT('Ctrl Pts',(-16.3665888869429,10.4631657107685,-319.240997555763)) ;
#24132=CARTESIAN_POINT('Ctrl Pts',(-16.3062332163227,10.5569800012248,-319.242367856849)) ;
#24133=CARTESIAN_POINT('Ctrl Pts',(-16.1644949881051,10.7731762133207,-319.245557877206)) ;
#24134=CARTESIAN_POINT('Ctrl Pts',(-16.0825249525402,10.8951647540438,-319.247382074004)) ;
#24135=CARTESIAN_POINT('Ctrl Pts',(-15.830094880295,11.2617766245844,-319.252938310712)) ;
#24136=CARTESIAN_POINT('Ctrl Pts',(-15.6553802985389,11.5034161787677,-319.256702401312)) ;
#24137=CARTESIAN_POINT('Ctrl Pts',(-15.2005919979552,12.1028510703977,-319.266284355565)) ;
#24138=CARTESIAN_POINT('Ctrl Pts',(-14.9133993252527,12.4550198886634,-319.27214469337)) ;
#24139=CARTESIAN_POINT('Ctrl Pts',(-14.3014337225396,13.153893498165,-319.284129349596)) ;
#24140=CARTESIAN_POINT('Ctrl Pts',(-13.9757578203743,13.4994116575871,-319.290249774535)) ;
#24141=CARTESIAN_POINT('Ctrl Pts',(-13.5526641681001,13.916543997344,-319.297733878049)) ;
#24142=CARTESIAN_POINT('Ctrl Pts',(-13.4668022349233,13.9996478710047,-319.299229649769)) ;
#24143=CARTESIAN_POINT('Ctrl Pts',(-13.3343548476939,14.1254947315382,-319.301498226729)) ;
#24144=CARTESIAN_POINT('Ctrl Pts',(-13.2883184836089,14.1688112593946,-319.302279711851)) ;
#24145=CARTESIAN_POINT('Ctrl Pts',(-13.1912193463019,14.2592842788769,-319.303912487723)) ;
#24146=CARTESIAN_POINT('Ctrl Pts',(-13.1401132729873,14.3063929472702,-319.304762904417)) ;
#24147=CARTESIAN_POINT('Ctrl Pts',(-13.0026594517259,14.4317375502826,-319.307027912034)) ;
#24148=CARTESIAN_POINT('Ctrl Pts',(-12.9158586748178,14.5094726399239,-319.30843500956)) ;
#24149=CARTESIAN_POINT('Ctrl Pts',(-12.2152370283555,15.1256504256142,-319.319630140021)) ;
#24150=CARTESIAN_POINT('Ctrl Pts',(-11.5687193323299,15.6256859697436,-319.329009437447)) ;
#24151=CARTESIAN_POINT('Ctrl Pts',(-10.581632880336,16.2941945412504,-319.343037871547)) ;
#24152=CARTESIAN_POINT('Ctrl Pts',(-10.2645659281097,16.4957696275153,-319.347497290025)) ;
#24153=CARTESIAN_POINT('Ctrl Pts',(-9.80522660530929,16.7694200485499,-319.353941284508)) ;
#24154=CARTESIAN_POINT('Ctrl Pts',(-9.667604152967,16.8491349153244,-319.355869657371)) ;
#24155=CARTESIAN_POINT('Ctrl Pts',(-9.42052513919147,16.9882262797459,-319.359330097166)) ;
#24156=CARTESIAN_POINT('Ctrl Pts',(-9.31144720129368,17.0482573009866,-319.360857201268)) ;
#24157=CARTESIAN_POINT('Ctrl Pts',(-9.07673726510174,17.1745052760715,-319.364142671045)) ;
#24158=CARTESIAN_POINT('Ctrl Pts',(-8.95094096972081,17.2404015772406,-319.365903276137)) ;
#24159=CARTESIAN_POINT('Ctrl Pts',(-8.58654913872108,17.4262188413609,-319.371002531296)) ;
#24160=CARTESIAN_POINT('Ctrl Pts',(-8.34618911471716,17.5426068772734,-319.374365648693)) ;
#24161=CARTESIAN_POINT('Ctrl Pts',(-7.34958317248912,18.0000670383572,-319.388291465842)) ;
#24162=CARTESIAN_POINT('Ctrl Pts',(-6.57427009648635,18.2974793099848,-319.399120297439)) ;
#24163=CARTESIAN_POINT('Ctrl Pts',(-5.57823854312572,18.6080515203548,-319.412430109452)) ;
#24164=CARTESIAN_POINT('Ctrl Pts',(-5.3731133531913,18.668314862405,-319.415137404912)) ;
#24165=CARTESIAN_POINT('Ctrl Pts',(-5.08338582086082,18.7482624151904,-319.418895210974)) ;
#24166=CARTESIAN_POINT('Ctrl Pts',(-4.99958272234323,18.770783884055,-319.41997441577)) ;
#24167=CARTESIAN_POINT('Ctrl Pts',(-4.85210862625507,18.8093587905659,-319.421858268555)) ;
#24168=CARTESIAN_POINT('Ctrl Pts',(-4.78850208370146,18.8256522873235,-319.422665692023)) ;
#24169=CARTESIAN_POINT('Ctrl Pts',(-4.64100228455089,18.8626400298758,-319.424526291629)) ;
#24170=CARTESIAN_POINT('Ctrl Pts',(-4.55705128569807,18.8830975930296,-319.425576703793)) ;
#24171=CARTESIAN_POINT('Ctrl Pts',(-4.26191973839969,18.9529338055533,-319.429243483035)) ;
#24172=CARTESIAN_POINT('Ctrl Pts',(-4.05005102379226,18.9993354280094,-319.431829396955)) ;
#24173=CARTESIAN_POINT('Ctrl Pts',(-3.45867597488227,19.1185114874035,-319.438965655464)) ;
#24174=CARTESIAN_POINT('Ctrl Pts',(-3.07770871133181,19.18352498438,-319.443471370064)) ;
#24175=CARTESIAN_POINT('Ctrl Pts',(-2.50189577599105,19.2641943980974,-319.450262618639)) ;
#24176=CARTESIAN_POINT('Ctrl Pts',(-2.30833870158,19.2883446849052,-319.45254192553)) ;
#24177=CARTESIAN_POINT('Ctrl Pts',(-1.67336492210439,19.3578760347954,-319.460033375713)) ;
#24178=CARTESIAN_POINT('Ctrl Pts',(-1.23075434875401,19.3910483792836,-319.465280469474)) ;
#24179=CARTESIAN_POINT('Ctrl Pts',(-0.623320616382399,19.4156911297978,
-319.472599739241)) ;
#24180=CARTESIAN_POINT('Ctrl Pts',(-0.459165776355288,19.4202666646659,
-319.474589088276)) ;
#24181=CARTESIAN_POINT('Ctrl Pts',(-0.16991243671988,19.4246595459666,-319.478117245155)) ;
#24182=CARTESIAN_POINT('Ctrl Pts',(-0.0448367083294808,19.4253509192243,
-319.479650332151)) ;
#24183=CARTESIAN_POINT('Ctrl Pts',(0.21935368510912,19.4242596456323,-319.482905152556)) ;
#24184=CARTESIAN_POINT('Ctrl Pts',(0.358460185782071,19.4221905317047,-319.484628652571)) ;
#24185=CARTESIAN_POINT('Ctrl Pts',(0.747493509970748,19.4122229552821,-319.489476103244)) ;
#24186=CARTESIAN_POINT('Ctrl Pts',(0.997307315390067,19.4009928708691,-319.492620766601)) ;
#24187=CARTESIAN_POINT('Ctrl Pts',(1.58522149112291,19.3631783933155,-319.500089585227)) ;
#24188=CARTESIAN_POINT('Ctrl Pts',(1.92298031716225,19.3325567558531,-319.504434253006)) ;
#24189=CARTESIAN_POINT('Ctrl Pts',(2.93072117525097,19.2145220741525,-319.517496453928)) ;
#24190=CARTESIAN_POINT('Ctrl Pts',(3.59712195098988,19.1009868442836,-319.5262798367)) ;
#24191=CARTESIAN_POINT('Ctrl Pts',(4.36775995916229,18.9279253875368,-319.536218792138)) ;
#24192=CARTESIAN_POINT('Ctrl Pts',(4.47904679191005,18.9019000745747,-319.537648164129)) ;
#24193=CARTESIAN_POINT('Ctrl Pts',(4.65063233290984,18.8601729863577,-319.539839477076)) ;
#24194=CARTESIAN_POINT('Ctrl Pts',(4.71109597756533,18.8451606751506,-319.5406092371)) ;
#24195=CARTESIAN_POINT('Ctrl Pts',(4.83992806172283,18.8125146220046,-319.542243423241)) ;
#24196=CARTESIAN_POINT('Ctrl Pts',(4.90827470886859,18.7947984676675,-319.543106761882)) ;
#24197=CARTESIAN_POINT('Ctrl Pts',(5.09457423403305,18.7454221966875,-319.545451928985)) ;
#24198=CARTESIAN_POINT('Ctrl Pts',(5.21232763872753,18.7130216857496,-319.546925321088)) ;
#24199=CARTESIAN_POINT('Ctrl Pts',(5.74454508610029,18.5611657237391,-319.55355860564)) ;
#24200=CARTESIAN_POINT('Ctrl Pts',(6.155266552297,18.4290359668572,-319.558608190151)) ;
#24201=CARTESIAN_POINT('Ctrl Pts',(7.21925500414974,18.0472079326958,-319.571816545702)) ;
#24202=CARTESIAN_POINT('Ctrl Pts',(7.86403413150695,17.7757228640842,-319.579964169707)) ;
#24203=CARTESIAN_POINT('Ctrl Pts',(8.65627264809483,17.3905899661984,-319.590539817958)) ;
#24204=CARTESIAN_POINT('Ctrl Pts',(8.81865051146814,17.3088150533775,-319.592737096492)) ;
#24205=CARTESIAN_POINT('Ctrl Pts',(9.09147400862782,17.1665829427565,-319.596483433851)) ;
#24206=CARTESIAN_POINT('Ctrl Pts',(9.20252330661169,17.1073093829274,-319.598023862791)) ;
#24207=CARTESIAN_POINT('Ctrl Pts',(9.42996686121904,16.9830538481456,-319.601211861457)) ;
#24208=CARTESIAN_POINT('Ctrl Pts',(9.54628416540355,16.9179446620544,-319.602860311755)) ;
#24209=CARTESIAN_POINT('Ctrl Pts',(9.85043698043884,16.7435580642309,-319.607218931059)) ;
#24210=CARTESIAN_POINT('Ctrl Pts',(10.037124720128,16.6323171106734,-319.609943317031)) ;
#24211=CARTESIAN_POINT('Ctrl Pts',(10.3465566923133,16.4408295884237,-319.614539446108)) ;
#24212=CARTESIAN_POINT('Ctrl Pts',(10.4703296399019,16.3622831570724,-319.616399948199)) ;
#24213=CARTESIAN_POINT('Ctrl Pts',(10.9943619232276,16.0213506831903,-319.624366904326)) ;
#24214=CARTESIAN_POINT('Ctrl Pts',(11.3857393299431,15.7456219411165,-319.630547899466)) ;
#24215=CARTESIAN_POINT('Ctrl Pts',(12.116032479166,15.1896454514303,-319.642386349653)) ;
#24216=CARTESIAN_POINT('Ctrl Pts',(12.4564073416982,14.911790272916,-319.648040808461)) ;
#24217=CARTESIAN_POINT('Ctrl Pts',(12.8763387012517,14.5445725085118,-319.655066458539)) ;
#24218=CARTESIAN_POINT('Ctrl Pts',(12.9648910773246,14.4656934579686,-319.65655069805)) ;
#24219=CARTESIAN_POINT('Ctrl Pts',(13.0994104250053,14.3436413398267,-319.658805835417)) ;
#24220=CARTESIAN_POINT('Ctrl Pts',(13.1458986479478,14.3010471335973,-319.659585261497)) ;
#24221=CARTESIAN_POINT('Ctrl Pts',(13.2433232408229,14.210906710811,-319.661218038106)) ;
#24222=CARTESIAN_POINT('Ctrl Pts',(13.2942128092271,14.1633112579453,-319.662070478705)) ;
#24223=CARTESIAN_POINT('Ctrl Pts',(13.4301638188544,14.0347821586678,-319.664348217855)) ;
#24224=CARTESIAN_POINT('Ctrl Pts',(13.5147494761151,13.953349314783,-319.665765874823)) ;
#24225=CARTESIAN_POINT('Ctrl Pts',(14.0191878154656,13.4588229937113,-319.674240296478)) ;
#24226=CARTESIAN_POINT('Ctrl Pts',(14.4208137413924,13.0275737888171,-319.681081538056)) ;
#24227=CARTESIAN_POINT('Ctrl Pts',(14.9722594784799,12.3786517725441,-319.691032954735)) ;
#24228=CARTESIAN_POINT('Ctrl Pts',(15.1382199895028,12.1751332232697,-319.694107094242)) ;
#24229=CARTESIAN_POINT('Ctrl Pts',(15.5134298944664,11.6954739098415,-319.701285857854)) ;
#24230=CARTESIAN_POINT('Ctrl Pts',(15.7195195733131,11.4169751131098,-319.705405497076)) ;
#24231=CARTESIAN_POINT('Ctrl Pts',(16.0085774286592,11.0036821824669,-319.71148753106)) ;
#24232=CARTESIAN_POINT('Ctrl Pts',(16.0975210870838,10.8731498482114,-319.713403808928)) ;
#24233=CARTESIAN_POINT('Ctrl Pts',(16.2535385579529,10.638069998087,-319.716849015764)) ;
#24234=CARTESIAN_POINT('Ctrl Pts',(16.3212203108627,10.5339364179202,-319.718373110447)) ;
#24235=CARTESIAN_POINT('Ctrl Pts',(16.4654702984172,10.3072686946033,-319.721686940702)) ;
#24236=CARTESIAN_POINT('Ctrl Pts',(16.5416794251544,10.1845148049907,-319.723479304229)) ;
#24237=CARTESIAN_POINT('Ctrl Pts',(16.7626753827012,9.81952023836204,-319.728802147479)) ;
#24238=CARTESIAN_POINT('Ctrl Pts',(16.9035606429977,9.57496218182493,-319.732360677361)) ;
#24239=CARTESIAN_POINT('Ctrl Pts',(17.3549922644091,8.75029982847682,-319.744316544545)) ;
#24240=CARTESIAN_POINT('Ctrl Pts',(17.6413915214249,8.15749990096506,-319.752854497285)) ;
#24241=CARTESIAN_POINT('Ctrl Pts',(18.0279101210599,7.24142332345096,-319.76563659963)) ;
#24242=CARTESIAN_POINT('Ctrl Pts',(18.1505922341871,6.92818572287452,-319.769934179204)) ;
#24243=CARTESIAN_POINT('Ctrl Pts',(18.2986470218039,6.519192244981,-319.775388638042)) ;
#24244=CARTESIAN_POINT('Ctrl Pts',(18.331507948968,6.42620935781394,-319.776618274191)) ;
#24245=CARTESIAN_POINT('Ctrl Pts',(18.385338365181,6.27011800760672,-319.77866268873)) ;
#24246=CARTESIAN_POINT('Ctrl Pts',(18.4066944075146,6.20714488752647,-319.779482061991)) ;
#24247=CARTESIAN_POINT('Ctrl Pts',(18.4527532675439,6.06900176175195,-319.781267087575)) ;
#24248=CARTESIAN_POINT('Ctrl Pts',(18.4773209549008,5.99378810833174,-319.782231158767)) ;
#24249=CARTESIAN_POINT('Ctrl Pts',(18.5526270616485,5.75837577893185,-319.785227071815)) ;
#24250=CARTESIAN_POINT('Ctrl Pts',(18.6017467860728,5.59766729655617,-319.787241281824)) ;
#24251=CARTESIAN_POINT('Ctrl Pts',(18.7965748415917,4.92933096199668,-319.795523127758)) ;
#24252=CARTESIAN_POINT('Ctrl Pts',(18.9236369358729,4.41650280620033,-319.801659121554)) ;
#24253=CARTESIAN_POINT('Ctrl Pts',(19.1407324677365,3.35697276733582,-319.814302166083)) ;
#24254=CARTESIAN_POINT('Ctrl Pts',(19.2285998746394,2.81031150364746,-319.820808521203)) ;
#24255=CARTESIAN_POINT('Ctrl Pts',(19.310926550977,2.107712269778,-319.829317575429)) ;
#24256=CARTESIAN_POINT('Ctrl Pts',(19.3270275158075,1.95456966864444,-319.831180468447)) ;
#24257=CARTESIAN_POINT('Ctrl Pts',(19.3530051756656,1.6756293138922,-319.834591018595)) ;
#24258=CARTESIAN_POINT('Ctrl Pts',(19.3634802149994,1.54989575190196,-319.83613473974)) ;
#24259=CARTESIAN_POINT('Ctrl Pts',(19.3824641648942,1.29164219627096,-319.839319501247)) ;
#24260=CARTESIAN_POINT('Ctrl Pts',(19.39084061465,1.15911900456988,-319.84096131771)) ;
#24261=CARTESIAN_POINT('Ctrl Pts',(19.4091907277486,0.812362275099774,-319.845277357797)) ;
#24262=CARTESIAN_POINT('Ctrl Pts',(19.416976473909,0.598031398985461,-319.847965278672)) ;
#24263=CARTESIAN_POINT('Ctrl Pts',(19.4240515196692,0.239845096497573,-319.852488637292)) ;
#24264=CARTESIAN_POINT('Ctrl Pts',(19.425294797375,0.0960473048833851,-319.854312971843)) ;
#24265=CARTESIAN_POINT('Ctrl Pts',(19.4238035592789,-0.510584409799216,
-319.862040189592)) ;
#24266=CARTESIAN_POINT('Ctrl Pts',(19.4061244350911,-0.973228774394006,
-319.868013287343)) ;
#24267=CARTESIAN_POINT('Ctrl Pts',(19.3573626930666,-1.63158588178593,-319.876529758202)) ;
#24268=CARTESIAN_POINT('Ctrl Pts',(19.3397897050108,-1.82814035011033,-319.879073856347)) ;
#24269=CARTESIAN_POINT('Ctrl Pts',(19.2872448141822,-2.32958775406388,-319.885547524391)) ;
#24270=CARTESIAN_POINT('Ctrl Pts',(19.2480369977297,-2.63398253625553,-319.889461733029)) ;
#24271=CARTESIAN_POINT('Ctrl Pts',(19.1868400664284,-3.03403455816125,-319.894535741393)) ;
#24272=CARTESIAN_POINT('Ctrl Pts',(19.1713150346135,-3.13063528946316,-319.895755464012)) ;
#24273=CARTESIAN_POINT('Ctrl Pts',(19.1440301423152,-3.29258917814907,-319.897788763722)) ;
#24274=CARTESIAN_POINT('Ctrl Pts',(19.1326638120382,-3.35800671164288,-319.898606816706)) ;
#24275=CARTESIAN_POINT('Ctrl Pts',(19.1069434318142,-3.50166607401071,-319.900395601994)) ;
#24276=CARTESIAN_POINT('Ctrl Pts',(19.0924437541368,-3.57988046125007,-319.90136468146)) ;
#24277=CARTESIAN_POINT('Ctrl Pts',(19.0453427895433,-3.82552454708578,-319.904395924486)) ;
#24278=CARTESIAN_POINT('Ctrl Pts',(19.011016352351,-3.99261536397352,-319.906439868259)) ;
#24279=CARTESIAN_POINT('Ctrl Pts',(18.8612998114041,-4.67562491496626,-319.914755429211)) ;
#24280=CARTESIAN_POINT('Ctrl Pts',(18.7270724414509,-5.18718219041252,-319.920896964146)) ;
#24281=CARTESIAN_POINT('Ctrl Pts',(18.4113633395472,-6.21718044863164,-319.933491337464)) ;
#24282=CARTESIAN_POINT('Ctrl Pts',(18.2284293175958,-6.73468601389578,-319.939942712156)) ;
#24283=CARTESIAN_POINT('Ctrl Pts',(17.9663481508599,-7.38679396782988,-319.948396081849)) ;
#24284=CARTESIAN_POINT('Ctrl Pts',(17.9071589631958,-7.52914661728683,-319.950261103953)) ;
#24285=CARTESIAN_POINT('Ctrl Pts',(17.7964438069221,-7.786728505083,-319.953674257314)) ;
#24286=CARTESIAN_POINT('Ctrl Pts',(17.7454772322504,-7.90218898381787,-319.955218430139)) ;
#24287=CARTESIAN_POINT('Ctrl Pts',(17.6386136913809,-8.13803083715431,-319.958402788484)) ;
#24288=CARTESIAN_POINT('Ctrl Pts',(17.5826008338157,-8.2583525428472,-319.96004373622)) ;
#24289=CARTESIAN_POINT('Ctrl Pts',(17.4330234286783,-8.57123979643036,-319.964354199776)) ;
#24290=CARTESIAN_POINT('Ctrl Pts',(17.3375008366692,-8.76284896724658,-319.967037345288)) ;
#24291=CARTESIAN_POINT('Ctrl Pts',(17.1727224004742,-9.08013238251074,-319.971551198128)) ;
#24292=CARTESIAN_POINT('Ctrl Pts',(17.105206232086,-9.20668878731601,-319.973370820631)) ;
#24293=CARTESIAN_POINT('Ctrl Pts',(16.8148983557659,-9.73664090089767,-319.981067326744)) ;
#24294=CARTESIAN_POINT('Ctrl Pts',(16.5791906918577,-10.1327892236922,-319.987013880993)) ;
#24295=CARTESIAN_POINT('Ctrl Pts',(16.2347365115245,-10.6674574852521,-319.995219045869)) ;
#24296=CARTESIAN_POINT('Ctrl Pts',(16.1378655561486,-10.8134459874558,-319.997478108299)) ;
#24297=CARTESIAN_POINT('Ctrl Pts',(15.8532660786967,-11.2300053106622,-320.003962314034)) ;
#24298=CARTESIAN_POINT('Ctrl Pts',(15.6606147021019,-11.4971393196055,-320.008168610392)) ;
#24299=CARTESIAN_POINT('Ctrl Pts',(15.401255676348,-11.8381491529765,-320.013541816394)) ;
#24300=CARTESIAN_POINT('Ctrl Pts',(15.340642454738,-11.9165909928463,-320.014777984915)) ;
#24301=CARTESIAN_POINT('Ctrl Pts',(15.2383304843045,-12.0469224113029,-320.01682974958)) ;
#24302=CARTESIAN_POINT('Ctrl Pts',(15.1969607062318,-12.0990677682819,-320.017650019072)) ;
#24303=CARTESIAN_POINT('Ctrl Pts',(15.1059979787026,-12.2125209500564,-320.019432696106)) ;
#24304=CARTESIAN_POINT('Ctrl Pts',(15.0562981778349,-12.2737414054994,-320.020393568594)) ;
#24305=CARTESIAN_POINT('Ctrl Pts',(14.9005404323206,-12.4632347953278,-320.023367103946)) ;
#24306=CARTESIAN_POINT('Ctrl Pts',(14.7932055954489,-12.5904485663399,-320.025362502473)) ;
#24307=CARTESIAN_POINT('Ctrl Pts',(14.5974159250915,-12.8165388336824,-320.028921331156)) ;
#24308=CARTESIAN_POINT('Ctrl Pts',(14.5095579535376,-12.915918372653,-320.030490098249)) ;
#24309=CARTESIAN_POINT('Ctrl Pts',(14.0312113165347,-13.4459538114782,-320.038900796939)) ;
#24310=CARTESIAN_POINT('Ctrl Pts',(13.6225568993258,-13.8598163825987,-320.045635080711)) ;
#24311=CARTESIAN_POINT('Ctrl Pts',(12.906066784318,-14.5230892005215,-320.057113830224)) ;
#24312=CARTESIAN_POINT('Ctrl Pts',(12.6080563836265,-14.7825435233644,-320.061799326824)) ;
#24313=CARTESIAN_POINT('Ctrl Pts',(12.1790461947006,-15.1336328199938,-320.068480156693)) ;
#24314=CARTESIAN_POINT('Ctrl Pts',(12.0545124738968,-15.2330147202168,-320.070411896682)) ;
#24315=CARTESIAN_POINT('Ctrl Pts',(11.8304864172023,-15.4073269615523,-320.073876027723)) ;
#24316=CARTESIAN_POINT('Ctrl Pts',(11.7314693973193,-15.4828537001632,-320.075403414269)) ;
#24317=CARTESIAN_POINT('Ctrl Pts',(11.6040727697785,-15.5781036372578,-320.077364289323)) ;
#24318=CARTESIAN_POINT('Ctrl Pts',(11.5763573826724,-15.5987104443636,-320.077790623979)) ;
#24319=CARTESIAN_POINT('Ctrl Pts',(11.536965465186,-15.6278361188462,-320.078396214306)) ;
#24320=CARTESIAN_POINT('Ctrl Pts',(11.5253341519739,-15.6364160403744,-320.078574983567)) ;
#24321=CARTESIAN_POINT('Ctrl Pts',(11.5013343520194,-15.6540783373441,-320.078943761192)) ;
#24322=CARTESIAN_POINT('Ctrl Pts',(11.4889646574522,-15.6631590545577,-320.079133782508)) ;
#24323=CARTESIAN_POINT('Ctrl Pts',(11.3494818178547,-15.7653006805766,-320.081275938116)) ;
#24324=CARTESIAN_POINT('Ctrl Pts',(11.2212519883264,-15.8568265048196,-320.083240115295)) ;
#24325=CARTESIAN_POINT('Ctrl Pts',(10.9334497031553,-16.0570098881476,-320.087636653383)) ;
#24326=CARTESIAN_POINT('Ctrl Pts',(10.7733421362647,-16.1648689453075,-320.090074571522)) ;
#24327=CARTESIAN_POINT('Ctrl Pts',(10.2898271280426,-16.4802218539497,-320.097407787465)) ;
#24328=CARTESIAN_POINT('Ctrl Pts',(9.96184416019737,-16.6805250139656,-320.102345417078)) ;
#24329=CARTESIAN_POINT('Ctrl Pts',(9.10076366196011,-17.1719373173476,-320.115128779555)) ;
#24330=CARTESIAN_POINT('Ctrl Pts',(8.55956732940584,-17.4480124475641,-320.122998913466)) ;
#24331=CARTESIAN_POINT('Ctrl Pts',(7.90699649753113,-17.7432217520323,-320.132001980529)) ;
#24332=CARTESIAN_POINT('Ctrl Pts',(7.80728493739994,-17.7873217126604,-320.133364258878)) ;
#24333=CARTESIAN_POINT('Ctrl Pts',(7.65082907614626,-17.8549492246879,-320.135477957095)) ;
#24334=CARTESIAN_POINT('Ctrl Pts',(7.59433550681355,-17.8790510261955,-320.136236353435)) ;
#24335=CARTESIAN_POINT('Ctrl Pts',(7.49133427772186,-17.9224180769281,-320.137609682883)) ;
#24336=CARTESIAN_POINT('Ctrl Pts',(7.44486426451642,-17.9417712356788,-320.138225831955)) ;
#24337=CARTESIAN_POINT('Ctrl Pts',(7.32828074780718,-17.9897933290309,-320.139763597955)) ;
#24338=CARTESIAN_POINT('Ctrl Pts',(7.2580737654951,-18.0182332089402,-320.140682406149)) ;
#24339=CARTESIAN_POINT('Ctrl Pts',(6.950268086372,-18.1408300983097,-320.144682484297)) ;
#24340=CARTESIAN_POINT('Ctrl Pts',(6.71099026965467,-18.2307035849578,-320.147719048505)) ;
#24341=CARTESIAN_POINT('Ctrl Pts',(5.96525904222833,-18.4941307713049,-320.157042646806)) ;
#24342=CARTESIAN_POINT('Ctrl Pts',(5.45335437292572,-18.6514909847323,-320.163251148029)) ;
#24343=CARTESIAN_POINT('Ctrl Pts',(4.50900273328787,-18.899578534748,-320.174703850276)) ;
#24344=CARTESIAN_POINT('Ctrl Pts',(4.07870795394553,-18.9970870043679,-320.179920710947)) ;
#24345=CARTESIAN_POINT('Ctrl Pts',(3.48464881511938,-19.1105901213535,-320.187203008135)) ;
#24346=CARTESIAN_POINT('Ctrl Pts',(3.32344711824944,-19.1392824134687,-320.189186663364)) ;
#24347=CARTESIAN_POINT('Ctrl Pts',(3.03855365646183,-19.1862827463981,-320.192708423543)) ;
#24348=CARTESIAN_POINT('Ctrl Pts',(2.91501170326987,-19.2054409131982,-320.194240878757)) ;
#24349=CARTESIAN_POINT('Ctrl Pts',(2.67617180461992,-19.2401211510786,-320.197214383535)) ;
#24350=CARTESIAN_POINT('Ctrl Pts',(2.5609023354619,-19.2558026741529,-320.198654322613)) ;
#24351=CARTESIAN_POINT('Ctrl Pts',(2.30827514732471,-19.28786210294,-320.201820904053)) ;
#24352=CARTESIAN_POINT('Ctrl Pts',(2.17086927092872,-19.3038101214256,-320.203550195971)) ;
#24353=CARTESIAN_POINT('Ctrl Pts',(1.35770446560157,-19.3893980313548,-320.213823603408)) ;
#24354=CARTESIAN_POINT('Ctrl Pts',(0.678840956636049,-19.4250170068381,
-320.222580491791)) ;
#24355=CARTESIAN_POINT('Ctrl Pts',(-0.000486475511301404,-19.4249999939084,
-320.231344117963)) ;
#24356=CARTESIAN_POINT('Ctrl Pts',(9.76712100086985E-9,-19.425,-318.518971385864)) ;
#24357=CARTESIAN_POINT('Ctrl Pts',(-0.281309642560281,-19.4250000001414,
-318.522593938602)) ;
#24358=CARTESIAN_POINT('Ctrl Pts',(-0.562608351426869,-19.4188891791731,
-318.52620480889)) ;
#24359=CARTESIAN_POINT('Ctrl Pts',(-0.98839503799673,-19.4003782790569,
-318.531633105823)) ;
#24360=CARTESIAN_POINT('Ctrl Pts',(-1.13301837794897,-19.3924694543237,
-318.53347047545)) ;
#24361=CARTESIAN_POINT('Ctrl Pts',(-1.49304367215994,-19.3687400017827,
-318.538025821844)) ;
#24362=CARTESIAN_POINT('Ctrl Pts',(-1.7082958740376,-19.3509429770943,-318.54073264566)) ;
#24363=CARTESIAN_POINT('Ctrl Pts',(-2.05644308952404,-19.3163038514045,
-318.545081253135)) ;
#24364=CARTESIAN_POINT('Ctrl Pts',(-2.18953891826495,-19.30167018793,-318.546736780915)) ;
#24365=CARTESIAN_POINT('Ctrl Pts',(-2.44903474289518,-19.2704204422533,
-318.549951299789)) ;
#24366=CARTESIAN_POINT('Ctrl Pts',(-2.57544357055276,-19.253933770986,-318.551511038845)) ;
#24367=CARTESIAN_POINT('Ctrl Pts',(-2.85626281090689,-19.2144933483132,
-318.554963303093)) ;
#24368=CARTESIAN_POINT('Ctrl Pts',(-3.01057738304826,-19.1909201390506,
-318.556851771086)) ;
#24369=CARTESIAN_POINT('Ctrl Pts',(-3.70461599907052,-19.0763210064208,
-318.565312913879)) ;
#24370=CARTESIAN_POINT('Ctrl Pts',(-4.24063143112721,-18.964367890893,-318.571751450696)) ;
#24371=CARTESIAN_POINT('Ctrl Pts',(-5.19254844379973,-18.7231673640123,
-318.583240523233)) ;
#24372=CARTESIAN_POINT('Ctrl Pts',(-5.61019155372591,-18.6022930116724,
-318.588302851206)) ;
#24373=CARTESIAN_POINT('Ctrl Pts',(-6.1763337479905,-18.4176381295371,-318.595341812481)) ;
#24374=CARTESIAN_POINT('Ctrl Pts',(-6.32861531634097,-18.3658683679347,
-318.59725336271)) ;
#24375=CARTESIAN_POINT('Ctrl Pts',(-6.59606307380386,-18.2712252690202,
-318.600654534087)) ;
#24376=CARTESIAN_POINT('Ctrl Pts',(-6.71149835490394,-18.2291390545479,
-318.602137165154)) ;
#24377=CARTESIAN_POINT('Ctrl Pts',(-6.89323042781999,-18.1609216627391,
-318.604499547196)) ;
#24378=CARTESIAN_POINT('Ctrl Pts',(-6.95979611729777,-18.1355159662169,
-318.605370888983)) ;
#24379=CARTESIAN_POINT('Ctrl Pts',(-7.08445107702869,-18.0871523229644,
-318.607015200005)) ;
#24380=CARTESIAN_POINT('Ctrl Pts',(-7.14257231876875,-18.0642793067054,
-318.607787063708)) ;
#24381=CARTESIAN_POINT('Ctrl Pts',(-7.30763223389162,-17.9984005220407,
-318.609992827469)) ;
#24382=CARTESIAN_POINT('Ctrl Pts',(-7.41429979558313,-17.9547227408593,
-318.611434720101)) ;
#24383=CARTESIAN_POINT('Ctrl Pts',(-8.05855226592651,-17.6841967435869,
-318.620229844747)) ;
#24384=CARTESIAN_POINT('Ctrl Pts',(-8.58608043785829,-17.4341704987621,
-318.627788409611)) ;
#24385=CARTESIAN_POINT('Ctrl Pts',(-9.5766023086422,-16.9088280443761,-318.642248496006)) ;
#24386=CARTESIAN_POINT('Ctrl Pts',(-10.0409869559877,-16.6372582347089,
-318.649149546914)) ;
#24387=CARTESIAN_POINT('Ctrl Pts',(-10.6539918496282,-16.243751158889,-318.658318004136)) ;
#24388=CARTESIAN_POINT('Ctrl Pts',(-10.8129520876239,-16.1383723268202,
-318.660701979693)) ;
#24389=CARTESIAN_POINT('Ctrl Pts',(-11.0760522722631,-15.9583238825469,
-318.664657495471)) ;
#24390=CARTESIAN_POINT('Ctrl Pts',(-11.1810513870136,-15.884933900105,-318.666238760988)) ;
#24391=CARTESIAN_POINT('Ctrl Pts',(-11.3790104965478,-15.7436335116766,
-318.669225437135)) ;
#24392=CARTESIAN_POINT('Ctrl Pts',(-11.4721077802981,-15.6759248258178,
-318.670632366494)) ;
#24393=CARTESIAN_POINT('Ctrl Pts',(-11.716685426649,-15.4947003137914,-318.674335661906)) ;
#24394=CARTESIAN_POINT('Ctrl Pts',(-11.8671178731669,-15.3797909198352,
-318.676620704043)) ;
#24395=CARTESIAN_POINT('Ctrl Pts',(-12.4100687898402,-14.9523426553508,
-318.684904697639)) ;
#24396=CARTESIAN_POINT('Ctrl Pts',(-12.7921186309444,-14.6268267404817,
-318.690800061353)) ;
#24397=CARTESIAN_POINT('Ctrl Pts',(-13.4933998368074,-13.9808036454977,
-318.701941583293)) ;
#24398=CARTESIAN_POINT('Ctrl Pts',(-13.8148835074953,-13.6632244498188,
-318.707191682889)) ;
#24399=CARTESIAN_POINT('Ctrl Pts',(-14.286815456577,-13.163323743258,-318.715306283102)) ;
#24400=CARTESIAN_POINT('Ctrl Pts',(-14.4454956396309,-12.9889893062894,
-318.718111007086)) ;
#24401=CARTESIAN_POINT('Ctrl Pts',(-14.6592687562269,-12.7453630525265,
-318.722026148711)) ;
#24402=CARTESIAN_POINT('Ctrl Pts',(-14.7171198130982,-12.6785182173073,
-318.723099953692)) ;
#24403=CARTESIAN_POINT('Ctrl Pts',(-14.8169737794786,-12.5615361527424,
-318.724980614691)) ;
#24404=CARTESIAN_POINT('Ctrl Pts',(-14.8591833934123,-12.5115774931384,
-318.725784347021)) ;
#24405=CARTESIAN_POINT('Ctrl Pts',(-14.9550834583552,-12.3969018107208,
-318.727630644818)) ;
#24406=CARTESIAN_POINT('Ctrl Pts',(-15.0086074605848,-12.3320475923666,
-318.728675615809)) ;
#24407=CARTESIAN_POINT('Ctrl Pts',(-15.1834832746546,-12.1173283289809,
-318.732134973936)) ;
#24408=CARTESIAN_POINT('Ctrl Pts',(-15.303024574892,-11.9660038788156,-318.734572358845)) ;
#24409=CARTESIAN_POINT('Ctrl Pts',(-15.9423061939397,-11.1315018639262,
-318.747956071733)) ;
#24410=CARTESIAN_POINT('Ctrl Pts',(-16.4185784480342,-10.4162254875563,
-318.75917431441)) ;
#24411=CARTESIAN_POINT('Ctrl Pts',(-16.9790078444991,-9.44009013957686,
-318.773468010337)) ;
#24412=CARTESIAN_POINT('Ctrl Pts',(-17.1072426802417,-9.20566442663661,
-318.776832953415)) ;
#24413=CARTESIAN_POINT('Ctrl Pts',(-17.2962768300287,-8.84249209513793,
-318.781937011439)) ;
#24414=CARTESIAN_POINT('Ctrl Pts',(-17.3605645323641,-8.71559853486529,
-318.783700558217)) ;
#24415=CARTESIAN_POINT('Ctrl Pts',(-17.4786392289392,-8.47604724865055,
-318.786992917104)) ;
#24416=CARTESIAN_POINT('Ctrl Pts',(-17.5327452632324,-8.36355485654717,
-318.78852395679)) ;
#24417=CARTESIAN_POINT('Ctrl Pts',(-17.6535782295364,-8.10600350792921,
-318.791995949859)) ;
#24418=CARTESIAN_POINT('Ctrl Pts',(-17.7196085051241,-7.96062759433623,
-318.793931894104)) ;
#24419=CARTESIAN_POINT('Ctrl Pts',(-17.9372022810921,-7.46543590598969,
-318.800450722183)) ;
#24420=CARTESIAN_POINT('Ctrl Pts',(-18.0802578902136,-7.1119782376013,-318.804975637053)) ;
#24421=CARTESIAN_POINT('Ctrl Pts',(-18.417471675483,-6.20272105639672,-318.816386168539)) ;
#24422=CARTESIAN_POINT('Ctrl Pts',(-18.5969383397456,-5.64188745504251,
-318.823205571547)) ;
#24423=CARTESIAN_POINT('Ctrl Pts',(-18.7854897387201,-4.94507596005149,
-318.83171059127)) ;
#24424=CARTESIAN_POINT('Ctrl Pts',(-18.8189884364033,-4.81602275262298,
-318.833287606221)) ;
#24425=CARTESIAN_POINT('Ctrl Pts',(-18.8914683970381,-4.52448500263164,
-318.836862583972)) ;
#24426=CARTESIAN_POINT('Ctrl Pts',(-18.9296870891624,-4.36182178552562,
-318.838865854972)) ;
#24427=CARTESIAN_POINT('Ctrl Pts',(-18.9829081362497,-4.12141803792854,
-318.841850821195)) ;
#24428=CARTESIAN_POINT('Ctrl Pts',(-18.9995415128459,-4.04404626993299,
-318.842815202196)) ;
#24429=CARTESIAN_POINT('Ctrl Pts',(-19.0293177693786,-3.90129934197765,
-318.844602882531)) ;
#24430=CARTESIAN_POINT('Ctrl Pts',(-19.0425976989024,-3.83595414033837,
-318.845424628392)) ;
#24431=CARTESIAN_POINT('Ctrl Pts',(-19.0748294395548,-3.6730615720313,-318.847480901521)) ;
#24432=CARTESIAN_POINT('Ctrl Pts',(-19.0933696769462,-3.5754347708675,-318.84872012183)) ;
#24433=CARTESIAN_POINT('Ctrl Pts',(-19.1699793297289,-3.15443471089505,
-318.854087102997)) ;
#24434=CARTESIAN_POINT('Ctrl Pts',(-19.2205886007562,-2.82975952166295,
-318.85828365467)) ;
#24435=CARTESIAN_POINT('Ctrl Pts',(-19.3472024779211,-1.8557195114113,-318.870907862588)) ;
#24436=CARTESIAN_POINT('Ctrl Pts',(-19.3986906192923,-1.20363816396453,
-318.879391869552)) ;
#24437=CARTESIAN_POINT('Ctrl Pts',(-19.4229942398794,-0.345942738703501,
-318.890309916632)) ;
#24438=CARTESIAN_POINT('Ctrl Pts',(-19.4255586998374,-0.141601557501543,
-318.89289464664)) ;
#24439=CARTESIAN_POINT('Ctrl Pts',(-19.4243293951762,0.238989545311665,
-318.897673544698)) ;
#24440=CARTESIAN_POINT('Ctrl Pts',(-19.4213614348628,0.415221148313284,
-318.899872358371)) ;
#24441=CARTESIAN_POINT('Ctrl Pts',(-19.4121531722439,0.717539689643196,
-318.903619567498)) ;
#24442=CARTESIAN_POINT('Ctrl Pts',(-19.407081366212,0.843650924975231,-318.905175322758)) ;
#24443=CARTESIAN_POINT('Ctrl Pts',(-19.3940307038812,1.10475439300562,-318.908381531465)) ;
#24444=CARTESIAN_POINT('Ctrl Pts',(-19.3858705420236,1.23973085745001,-318.910030725909)) ;
#24445=CARTESIAN_POINT('Ctrl Pts',(-19.3601426778081,1.60238675401459,-318.91444132033)) ;
#24446=CARTESIAN_POINT('Ctrl Pts',(-19.3399684821758,1.82985987867593,-318.917185930809)) ;
#24447=CARTESIAN_POINT('Ctrl Pts',(-19.2315153508163,2.848301551117,-318.929400602154)) ;
#24448=CARTESIAN_POINT('Ctrl Pts',(-19.0986877147631,3.63374849181006,-318.938588139787)) ;
#24449=CARTESIAN_POINT('Ctrl Pts',(-18.8716089887424,4.60813179505011,-318.950346886867)) ;
#24450=CARTESIAN_POINT('Ctrl Pts',(-18.8220148624354,4.80668917155145,-318.952764524926)) ;
#24451=CARTESIAN_POINT('Ctrl Pts',(-18.7318332272153,5.14491890736277,-318.956942448483)) ;
#24452=CARTESIAN_POINT('Ctrl Pts',(-18.6927974746998,5.2849871408575,-318.958690325869)) ;
#24453=CARTESIAN_POINT('Ctrl Pts',(-18.6312341767884,5.49666905831746,-318.961366781977)) ;
#24454=CARTESIAN_POINT('Ctrl Pts',(-18.609857994836,5.56861231194216,-318.962282579803)) ;
#24455=CARTESIAN_POINT('Ctrl Pts',(-18.5686016729175,5.70457273291662,-318.964026421333)) ;
#24456=CARTESIAN_POINT('Ctrl Pts',(-18.5488060791336,5.76861431843191,-318.964853487191)) ;
#24457=CARTESIAN_POINT('Ctrl Pts',(-18.4966253480309,5.93438052676743,-318.967007935004)) ;
#24458=CARTESIAN_POINT('Ctrl Pts',(-18.463732406974,6.03594293036196,-318.968341255345)) ;
#24459=CARTESIAN_POINT('Ctrl Pts',(-18.2309585715872,6.73495917707555,-318.977597716277)) ;
#24460=CARTESIAN_POINT('Ctrl Pts',(-18.0029523526304,7.32265194850747,-318.985770355803)) ;
#24461=CARTESIAN_POINT('Ctrl Pts',(-17.5949113088679,8.23949358284055,-318.998706344651)) ;
#24462=CARTESIAN_POINT('Ctrl Pts',(-17.4332163546212,8.5763119587949,-319.003503551503)) ;
#24463=CARTESIAN_POINT('Ctrl Pts',(-17.1400142964417,9.14446202074354,-319.01162184168)) ;
#24464=CARTESIAN_POINT('Ctrl Pts',(-17.0132826723432,9.37813888071287,-319.014969188932)) ;
#24465=CARTESIAN_POINT('Ctrl Pts',(-16.8116435982421,9.73238796335473,-319.020050470095)) ;
#24466=CARTESIAN_POINT('Ctrl Pts',(-16.7401440448032,9.85486242278771,-319.021808590269)) ;
#24467=CARTESIAN_POINT('Ctrl Pts',(-16.6033408972646,10.0834125749074,-319.025092136772)) ;
#24468=CARTESIAN_POINT('Ctrl Pts',(-16.5383456404657,10.1896644512946,-319.026619769169)) ;
#24469=CARTESIAN_POINT('Ctrl Pts',(-16.3878492836484,10.4304568480525,-319.030085119356)) ;
#24470=CARTESIAN_POINT('Ctrl Pts',(-16.3017048851415,10.5645848065078,-319.032017823272)) ;
#24471=CARTESIAN_POINT('Ctrl Pts',(-15.9972008075659,11.0261076984492,-319.038681319967)) ;
#24472=CARTESIAN_POINT('Ctrl Pts',(-15.7705506164876,11.3479169398191,-319.043349155503)) ;
#24473=CARTESIAN_POINT('Ctrl Pts',(-15.184940038922,12.1279337945308,-319.054817237063)) ;
#24474=CARTESIAN_POINT('Ctrl Pts',(-14.8148679480065,12.5773156145039,-319.061557857873)) ;
#24475=CARTESIAN_POINT('Ctrl Pts',(-14.3363224859771,13.1079398816237,-319.069975444417)) ;
#24476=CARTESIAN_POINT('Ctrl Pts',(-14.2464527234643,13.2055600074209,-319.071544724529)) ;
#24477=CARTESIAN_POINT('Ctrl Pts',(-14.041585663632,13.4235692720284,-319.075104557132)) ;
#24478=CARTESIAN_POINT('Ctrl Pts',(-13.9260266340707,13.543416185919,-319.077100443237)) ;
#24479=CARTESIAN_POINT('Ctrl Pts',(-13.7534666466554,13.7178351715603,-319.080074754697)) ;
#24480=CARTESIAN_POINT('Ctrl Pts',(-13.6976507680253,13.7735692545961,-319.081035916552)) ;
#24481=CARTESIAN_POINT('Ctrl Pts',(-13.5940957996483,13.8757204367483,-319.082819134496)) ;
#24482=CARTESIAN_POINT('Ctrl Pts',(-13.5464546343919,13.9222349158385,-319.083639655415)) ;
#24483=CARTESIAN_POINT('Ctrl Pts',(-13.4272529093993,14.0374264579817,-319.085692330991)) ;
#24484=CARTESIAN_POINT('Ctrl Pts',(-13.3554037623734,14.1058020885596,-319.086929164425)) ;
#24485=CARTESIAN_POINT('Ctrl Pts',(-13.0430800892332,14.3985011130801,-319.092297491269)) ;
#24486=CARTESIAN_POINT('Ctrl Pts',(-12.7974544051356,14.6172477753458,-319.096498007817)) ;
#24487=CARTESIAN_POINT('Ctrl Pts',(-12.4521047642065,14.9094254161017,-319.102312037758)) ;
#24488=CARTESIAN_POINT('Ctrl Pts',(-12.3570560226559,14.988296959111,-319.103903099836)) ;
#24489=CARTESIAN_POINT('Ctrl Pts',(-11.9657294571611,15.3067673999572,-319.110408627166)) ;
#24490=CARTESIAN_POINT('Ctrl Pts',(-11.6631843900081,15.5385308191745,-319.115332337856)) ;
#24491=CARTESIAN_POINT('Ctrl Pts',(-11.032465958419,15.9928850761558,-319.12529673545)) ;
#24492=CARTESIAN_POINT('Ctrl Pts',(-10.7038988152191,16.2146301114938,-319.130331621717)) ;
#24493=CARTESIAN_POINT('Ctrl Pts',(-10.2339196797603,16.5112975471355,-319.137288657613)) ;
#24494=CARTESIAN_POINT('Ctrl Pts',(-10.0980172924047,16.5947613891119,-319.139273005091)) ;
#24495=CARTESIAN_POINT('Ctrl Pts',(-9.85437637253241,16.7402910866508,-319.142781867258)) ;
#24496=CARTESIAN_POINT('Ctrl Pts',(-9.74704073897626,16.8030139033719,-319.144311232173)) ;
#24497=CARTESIAN_POINT('Ctrl Pts',(-9.51455649186934,16.9358915135056,-319.147589070207)) ;
#24498=CARTESIAN_POINT('Ctrl Pts',(-9.38921772309961,17.0056989627636,-319.149334899365)) ;
#24499=CARTESIAN_POINT('Ctrl Pts',(-9.02067087819596,17.2056445089635,-319.15440884559)) ;
#24500=CARTESIAN_POINT('Ctrl Pts',(-8.77545035467825,17.3319986599757,-319.157709701277)) ;
#24501=CARTESIAN_POINT('Ctrl Pts',(-7.90574916523827,17.7569368184926,-319.169194684422)) ;
#24502=CARTESIAN_POINT('Ctrl Pts',(-7.26808256790414,18.0273306093729,-319.177204314309)) ;
#24503=CARTESIAN_POINT('Ctrl Pts',(-6.32345454911503,18.3696015485612,-319.189001075838)) ;
#24504=CARTESIAN_POINT('Ctrl Pts',(-6.02703321474957,18.4689796230911,-319.192696813909)) ;
#24505=CARTESIAN_POINT('Ctrl Pts',(-5.63427989693023,18.590191118835,-319.197649238454)) ;
#24506=CARTESIAN_POINT('Ctrl Pts',(-5.53999659840101,18.6185056716164,-319.198842335518)) ;
#24507=CARTESIAN_POINT('Ctrl Pts',(-5.38169521646288,18.6647368098396,-319.20085544333)) ;
#24508=CARTESIAN_POINT('Ctrl Pts',(-5.31779301641488,18.6830436767091,-319.201670833769)) ;
#24509=CARTESIAN_POINT('Ctrl Pts',(-5.17753837271423,18.7224463123878,-319.203467236348)) ;
#24510=CARTESIAN_POINT('Ctrl Pts',(-5.10114848518211,18.7434037365707,-319.204449810701)) ;
#24511=CARTESIAN_POINT('Ctrl Pts',(-4.8617830801725,18.8075014801824,-319.207539290597)) ;
#24512=CARTESIAN_POINT('Ctrl Pts',(-4.69837293282371,18.8489877254449,-319.209663710756)) ;
#24513=CARTESIAN_POINT('Ctrl Pts',(-4.02151656785325,19.0114777528298,-319.2184980939)) ;
#24514=CARTESIAN_POINT('Ctrl Pts',(-3.50378669144107,19.1136694631686,-319.225331953445)) ;
#24515=CARTESIAN_POINT('Ctrl Pts',(-2.43577292500802,19.2796216008331,-319.239263664763)) ;
#24516=CARTESIAN_POINT('Ctrl Pts',(-1.8856225545396,19.3411796397485,-319.246350370911)) ;
#24517=CARTESIAN_POINT('Ctrl Pts',(-1.18002345020777,19.3897360898768,-319.255222727326)) ;
#24518=CARTESIAN_POINT('Ctrl Pts',(-1.02633135182892,19.3984784202595,-319.257142841635)) ;
#24519=CARTESIAN_POINT('Ctrl Pts',(-0.746531880739883,19.4110594300021,
-319.26061536971)) ;
#24520=CARTESIAN_POINT('Ctrl Pts',(-0.620460002500041,19.415498125939,-319.262171518501)) ;
#24521=CARTESIAN_POINT('Ctrl Pts',(-0.361615415586241,19.4220876884012,
-319.265349473588)) ;
#24522=CARTESIAN_POINT('Ctrl Pts',(-0.228845829115496,19.4241057844961,
-319.266970342065)) ;
#24523=CARTESIAN_POINT('Ctrl Pts',(0.118422270441552,19.4258232120628,-319.271187264693)) ;
#24524=CARTESIAN_POINT('Ctrl Pts',(0.332913498290453,19.423331334148,-319.273769216686)) ;
#24525=CARTESIAN_POINT('Ctrl Pts',(0.691097371376012,19.4132351215999,-319.278050392725)) ;
#24526=CARTESIAN_POINT('Ctrl Pts',(0.834825746196516,19.4075856172344,-319.279760140831)) ;
#24527=CARTESIAN_POINT('Ctrl Pts',(1.44092500563573,19.3770163131899,-319.286943841325)) ;
#24528=CARTESIAN_POINT('Ctrl Pts',(1.90239030063177,19.3371646729517,-319.292344948641)) ;
#24529=CARTESIAN_POINT('Ctrl Pts',(2.54927461513781,19.2579185282765,-319.299957837074)) ;
#24530=CARTESIAN_POINT('Ctrl Pts',(2.73621542702979,19.2322477154015,-319.302163367099)) ;
#24531=CARTESIAN_POINT('Ctrl Pts',(3.23294661115451,19.1566471614693,-319.308062367286)) ;
#24532=CARTESIAN_POINT('Ctrl Pts',(3.54195087193586,19.1019281088195,-319.31177164361)) ;
#24533=CARTESIAN_POINT('Ctrl Pts',(3.94607148523922,19.0202222257233,-319.316739172532)) ;
#24534=CARTESIAN_POINT('Ctrl Pts',(4.04249990231068,18.9999612679811,-319.317933340458)) ;
#24535=CARTESIAN_POINT('Ctrl Pts',(4.20372436194343,18.9648028255723,-319.31994762389)) ;
#24536=CARTESIAN_POINT('Ctrl Pts',(4.26860563362978,18.9503047647362,-319.320763104396)) ;
#24537=CARTESIAN_POINT('Ctrl Pts',(4.41057961537276,18.9178138081743,-319.322558982284)) ;
#24538=CARTESIAN_POINT('Ctrl Pts',(4.48763917291356,18.8996821787261,-319.323540933839)) ;
#24539=CARTESIAN_POINT('Ctrl Pts',(4.7281420408479,18.8415395331534,-319.326625760228)) ;
#24540=CARTESIAN_POINT('Ctrl Pts',(4.89117753658232,18.7998755657682,-319.328746074956)) ;
#24541=CARTESIAN_POINT('Ctrl Pts',(5.56334159726219,18.6187674092852,-319.33758068225)) ;
#24542=CARTESIAN_POINT('Ctrl Pts',(6.0672224142105,18.4607172509099,-319.344419276832)) ;
#24543=CARTESIAN_POINT('Ctrl Pts',(7.0849251195189,18.0953242375593,-319.358357129462)) ;
#24544=CARTESIAN_POINT('Ctrl Pts',(7.59758239100315,17.8861306180735,-319.365445277847)) ;
#24545=CARTESIAN_POINT('Ctrl Pts',(8.24053287680013,17.5911325318351,-319.374319232124)) ;
#24546=CARTESIAN_POINT('Ctrl Pts',(8.37969030386068,17.5252707923306,-319.376239541859)) ;
#24547=CARTESIAN_POINT('Ctrl Pts',(8.6314383181823,17.4024370490482,-319.379712491934)) ;
#24548=CARTESIAN_POINT('Ctrl Pts',(8.74428481201609,17.3460089317986,-319.381268866787)) ;
#24549=CARTESIAN_POINT('Ctrl Pts',(8.9747747816275,17.2279331524601,-319.384447379039)) ;
#24550=CARTESIAN_POINT('Ctrl Pts',(9.09235189995542,17.1661702213987,-319.386068577443)) ;
#24551=CARTESIAN_POINT('Ctrl Pts',(9.39820217234182,17.0014839796763,-319.390286683647)) ;
#24552=CARTESIAN_POINT('Ctrl Pts',(9.5854197004372,16.8966384515679,-319.392869480552)) ;
#24553=CARTESIAN_POINT('Ctrl Pts',(9.89523116576786,16.7163312944322,-319.397152253011)) ;
#24554=CARTESIAN_POINT('Ctrl Pts',(10.0187922188998,16.6425699426894,-319.398862753759)) ;
#24555=CARTESIAN_POINT('Ctrl Pts',(10.5367482879582,16.3255105618358,-319.406051458614)) ;
#24556=CARTESIAN_POINT('Ctrl Pts',(10.9231907820573,16.0695134679488,-319.411456733147)) ;
#24557=CARTESIAN_POINT('Ctrl Pts',(11.4393971990231,15.7003229998558,-319.418870291716)) ;
#24558=CARTESIAN_POINT('Ctrl Pts',(11.5773630273631,15.5988658520796,-319.420871955883)) ;
#24559=CARTESIAN_POINT('Ctrl Pts',(11.9765916353141,15.297067129635,-319.426743336963)) ;
#24560=CARTESIAN_POINT('Ctrl Pts',(12.2341240503698,15.0918924515503,-319.430631320507)) ;
#24561=CARTESIAN_POINT('Ctrl Pts',(12.5622626184348,14.8165452073739,-319.435791589205)) ;
#24562=CARTESIAN_POINT('Ctrl Pts',(12.6377194030083,14.7522371940441,-319.436992976174)) ;
#24563=CARTESIAN_POINT('Ctrl Pts',(12.763012126789,14.6437897283367,-319.439015543221)) ;
#24564=CARTESIAN_POINT('Ctrl Pts',(12.8131194532447,14.5999666452216,-319.439831995936)) ;
#24565=CARTESIAN_POINT('Ctrl Pts',(12.9220889498549,14.5036705745683,-319.441624961875)) ;
#24566=CARTESIAN_POINT('Ctrl Pts',(12.9808587361702,14.4510950939438,-319.442602975731)) ;
#24567=CARTESIAN_POINT('Ctrl Pts',(13.1626774036782,14.2864359408839,-319.445660845915)) ;
#24568=CARTESIAN_POINT('Ctrl Pts',(13.2846068537678,14.173127704085,-319.447757731575)) ;
#24569=CARTESIAN_POINT('Ctrl Pts',(13.501065969841,13.9667261222266,-319.451552621445)) ;
#24570=CARTESIAN_POINT('Ctrl Pts',(13.5961268684638,13.8742046626275,-319.453245088027)) ;
#24571=CARTESIAN_POINT('Ctrl Pts',(14.1026834695256,13.3709741176509,-319.46238856836)) ;
#24572=CARTESIAN_POINT('Ctrl Pts',(14.496531456211,12.942921118733,-319.469937593148)) ;
#24573=CARTESIAN_POINT('Ctrl Pts',(15.124775587694,12.1954037912678,-319.482456125675)) ;
#24574=CARTESIAN_POINT('Ctrl Pts',(15.3696779437044,11.885272879332,-319.487476581644)) ;
#24575=CARTESIAN_POINT('Ctrl Pts',(15.699803610784,11.4399370657213,-319.494417871668)) ;
#24576=CARTESIAN_POINT('Ctrl Pts',(15.7930770486984,11.3108227338175,-319.496400326873)) ;
#24577=CARTESIAN_POINT('Ctrl Pts',(15.9564245101839,11.0787475722964,-319.499910428903)) ;
#24578=CARTESIAN_POINT('Ctrl Pts',(16.0271161498356,10.9762324541092,-319.501442864822)) ;
#24579=CARTESIAN_POINT('Ctrl Pts',(16.1762175280855,10.7554978102815,-319.504704586036)) ;
#24580=CARTESIAN_POINT('Ctrl Pts',(16.2543279150401,10.6370846927523,-319.506431482649)) ;
#24581=CARTESIAN_POINT('Ctrl Pts',(16.4752218762355,10.2941004329853,-319.511370527203)) ;
#24582=CARTESIAN_POINT('Ctrl Pts',(16.6146969759507,10.0674368322498,-319.514557737471)) ;
#24583=CARTESIAN_POINT('Ctrl Pts',(16.9390313838352,9.51524722024922,-319.522163407105)) ;
#24584=CARTESIAN_POINT('Ctrl Pts',(17.1192242493347,9.18710375889944,-319.526553240275)) ;
#24585=CARTESIAN_POINT('Ctrl Pts',(17.5762887518579,8.29455790863486,-319.538274792425)) ;
#24586=CARTESIAN_POINT('Ctrl Pts',(17.835434727826,7.72158530093575,-319.545564656954)) ;
#24587=CARTESIAN_POINT('Ctrl Pts',(18.1055920530098,7.03772475473517,-319.554405862526)) ;
#24588=CARTESIAN_POINT('Ctrl Pts',(18.1440156535216,6.93806379558523,-319.555698077377)) ;
#24589=CARTESIAN_POINT('Ctrl Pts',(18.2052237415366,6.77531926819771,-319.557817831679)) ;
#24590=CARTESIAN_POINT('Ctrl Pts',(18.2285069520863,6.71242556551517,-319.558639365612)) ;
#24591=CARTESIAN_POINT('Ctrl Pts',(18.2772007207493,6.57876976234691,-319.560391185835)) ;
#24592=CARTESIAN_POINT('Ctrl Pts',(18.3025270558299,6.5079782670706,-319.56132243007)) ;
#24593=CARTESIAN_POINT('Ctrl Pts',(18.3757438360789,6.2995166226579,-319.564072687228)) ;
#24594=CARTESIAN_POINT('Ctrl Pts',(18.4224964161285,6.16145249913778,-319.565904363065)) ;
#24595=CARTESIAN_POINT('Ctrl Pts',(18.5015169430172,5.91915517059847,-319.569128821231)) ;
#24596=CARTESIAN_POINT('Ctrl Pts',(18.5344688824556,5.81515178982918,-319.570516063413)) ;
#24597=CARTESIAN_POINT('Ctrl Pts',(18.684680673011,5.32680053795363,-319.577036745979)) ;
#24598=CARTESIAN_POINT('Ctrl Pts',(18.7908721890419,4.93915153764358,-319.582230471955)) ;
#24599=CARTESIAN_POINT('Ctrl Pts',(18.9276947719951,4.37107506445579,-319.58976736749)) ;
#24600=CARTESIAN_POINT('Ctrl Pts',(18.9679231742898,4.1930677438476,-319.592118989836)) ;
#24601=CARTESIAN_POINT('Ctrl Pts',(19.0957257404718,3.58802175684998,-319.60006284774)) ;
#24602=CARTESIAN_POINT('Ctrl Pts',(19.1714323752068,3.15861110030695,-319.60561513026)) ;
#24603=CARTESIAN_POINT('Ctrl Pts',(19.255610793609,2.56493228343429,-319.613129698851)) ;
#24604=CARTESIAN_POINT('Ctrl Pts',(19.2765431084871,2.40256332806498,-319.615168827079)) ;
#24605=CARTESIAN_POINT('Ctrl Pts',(19.3098362399808,2.11576887111567,-319.618741893899)) ;
#24606=CARTESIAN_POINT('Ctrl Pts',(19.3230528431689,1.99145233401034,-319.620281258418)) ;
#24607=CARTESIAN_POINT('Ctrl Pts',(19.3484645527746,1.72828536821113,-319.623520490304)) ;
#24608=CARTESIAN_POINT('Ctrl Pts',(19.3603671214867,1.58941368103535,-319.625218378177)) ;
#24609=CARTESIAN_POINT('Ctrl Pts',(19.3895556127815,1.19959459489223,-319.629954464472)) ;
#24610=CARTESIAN_POINT('Ctrl Pts',(19.4034633545706,0.948421966995108,-319.632971044759)) ;
#24611=CARTESIAN_POINT('Ctrl Pts',(19.4247704260956,0.355030743297774,-319.640033855164)) ;
#24612=CARTESIAN_POINT('Ctrl Pts',(19.4280104723781,0.0127464750800942,
-319.644057303709)) ;
#24613=CARTESIAN_POINT('Ctrl Pts',(19.4109258119925,-0.994469447955966,
-319.65584664851)) ;
#24614=CARTESIAN_POINT('Ctrl Pts',(19.3654968887435,-1.65847345045228,-319.663542447662)) ;
#24615=CARTESIAN_POINT('Ctrl Pts',(19.2721535258711,-2.43482484567934,-319.672924137038)) ;
#24616=CARTESIAN_POINT('Ctrl Pts',(19.2571613486127,-2.55068819893634,-319.674334881957)) ;
#24617=CARTESIAN_POINT('Ctrl Pts',(19.2325126297362,-2.72855628319807,-319.676521203806)) ;
#24618=CARTESIAN_POINT('Ctrl Pts',(19.2235993182903,-2.79066133423313,-319.677288462859)) ;
#24619=CARTESIAN_POINT('Ctrl Pts',(19.2040999190519,-2.9219986890197,-319.678920192542)) ;
#24620=CARTESIAN_POINT('Ctrl Pts',(19.1934399819546,-2.99121909490093,-319.679785621922)) ;
#24621=CARTESIAN_POINT('Ctrl Pts',(19.1636187141323,-3.17813824201646,-319.682135859549)) ;
#24622=CARTESIAN_POINT('Ctrl Pts',(19.1437475537222,-3.29572062565021,-319.683628527363)) ;
#24623=CARTESIAN_POINT('Ctrl Pts',(19.0516453757676,-3.81174554693782,-319.6902310191)) ;
#24624=CARTESIAN_POINT('Ctrl Pts',(18.9680483907105,-4.20805595952492,-319.69543564422)) ;
#24625=CARTESIAN_POINT('Ctrl Pts',(18.696546370881,-5.3215759478819,-319.710212277407)) ;
#24626=CARTESIAN_POINT('Ctrl Pts',(18.479892395138,-6.03105317827658,-319.719789401176)) ;
#24627=CARTESIAN_POINT('Ctrl Pts',(18.1618668340894,-6.89264958180068,-319.731323128647)) ;
#24628=CARTESIAN_POINT('Ctrl Pts',(18.0982345214657,-7.05804027300622,-319.733534096698)) ;
#24629=CARTESIAN_POINT('Ctrl Pts',(17.9853395516464,-7.33990263142604,-319.737296169189)) ;
#24630=CARTESIAN_POINT('Ctrl Pts',(17.937186216287,-7.45680629481606,-319.738854764944)) ;
#24631=CARTESIAN_POINT('Ctrl Pts',(17.835238496018,-7.69760575949502,-319.742061997978)) ;
#24632=CARTESIAN_POINT('Ctrl Pts',(17.7812862177421,-7.82142743621631,-319.743709426064)) ;
#24633=CARTESIAN_POINT('Ctrl Pts',(17.6331611894406,-8.15192185233348,-319.748103536506)) ;
#24634=CARTESIAN_POINT('Ctrl Pts',(17.5366479334065,-8.35752253527709,-319.750833701538)) ;
#24635=CARTESIAN_POINT('Ctrl Pts',(17.3676193906738,-8.70177470242162,-319.755408402899)) ;
#24636=CARTESIAN_POINT('Ctrl Pts',(17.2969940729034,-8.84132808906969,-319.757263924998)) ;
#24637=CARTESIAN_POINT('Ctrl Pts',(16.9754634801301,-9.45806048023715,-319.765480305192)) ;
#24638=CARTESIAN_POINT('Ctrl Pts',(16.7064424421542,-9.92552513051495,-319.771744703688)) ;
#24639=CARTESIAN_POINT('Ctrl Pts',(16.2286623120334,-10.6811560918468,-319.782210097808)) ;
#24640=CARTESIAN_POINT('Ctrl Pts',(16.0308128962793,-10.9758650115822,-319.786384723742)) ;
#24641=CARTESIAN_POINT('Ctrl Pts',(15.7574815395629,-11.3598396332507,-319.792040093532)) ;
#24642=CARTESIAN_POINT('Ctrl Pts',(15.689109800906,-11.454082877267,-319.793446143421)) ;
#24643=CARTESIAN_POINT('Ctrl Pts',(15.5826388633039,-11.5980997861228,-319.795626875622)) ;
#24644=CARTESIAN_POINT('Ctrl Pts',(15.5451390825901,-11.6483133321948,-319.796393306092)) ;
#24645=CARTESIAN_POINT('Ctrl Pts',(15.4651690207367,-11.754322135218,-319.798025258767)) ;
#24646=CARTESIAN_POINT('Ctrl Pts',(15.422638318519,-11.8100706589939,-319.798891756021)) ;
#24647=CARTESIAN_POINT('Ctrl Pts',(15.3067061273003,-11.9603383706976,-319.801248414546)) ;
#24648=CARTESIAN_POINT('Ctrl Pts',(15.2327315358329,-12.0544114871995,-319.802746505928)) ;
#24649=CARTESIAN_POINT('Ctrl Pts',(14.9022893818169,-12.4667337797591,-319.80940263346)) ;
#24650=CARTESIAN_POINT('Ctrl Pts',(14.6366840169162,-12.7775255823434,-319.814657122216)) ;
#24651=CARTESIAN_POINT('Ctrl Pts',(13.8676023164714,-13.6219747008256,-319.829383771116)) ;
#24652=CARTESIAN_POINT('Ctrl Pts',(13.3434123698215,-14.1358389693269,-319.838859027163)) ;
#24653=CARTESIAN_POINT('Ctrl Pts',(12.6570262819971,-14.736424319879,-319.850315376833)) ;
#24654=CARTESIAN_POINT('Ctrl Pts',(12.5210150489641,-14.8521614022319,-319.85254399068)) ;
#24655=CARTESIAN_POINT('Ctrl Pts',(12.2858598279487,-15.0467375248484,-319.85632626538)) ;
#24656=CARTESIAN_POINT('Ctrl Pts',(12.1875052902613,-15.1265123773828,-319.857887629423)) ;
#24657=CARTESIAN_POINT('Ctrl Pts',(11.997661978307,-15.2774396630474,-319.86086265066)) ;
#24658=CARTESIAN_POINT('Ctrl Pts',(11.9063026660171,-15.3487462832055,-319.862277542121)) ;
#24659=CARTESIAN_POINT('Ctrl Pts',(11.6709892955055,-15.5290448493576,-319.865880176186)) ;
#24660=CARTESIAN_POINT('Ctrl Pts',(11.5261437010686,-15.636855073254,-319.868058406599)) ;
#24661=CARTESIAN_POINT('Ctrl Pts',(11.1927040063727,-15.877887371847,-319.87298960823)) ;
#24662=CARTESIAN_POINT('Ctrl Pts',(11.0031952466678,-16.0097977796998,-319.875733059635)) ;
#24663=CARTESIAN_POINT('Ctrl Pts',(10.3488665902215,-16.4481460757579,-319.885033523324)) ;
#24664=CARTESIAN_POINT('Ctrl Pts',(9.87324753800785,-16.7379667709284,-319.891497081867)) ;
#24665=CARTESIAN_POINT('Ctrl Pts',(9.06903814116813,-17.181795687896,-319.902258499843)) ;
#24666=CARTESIAN_POINT('Ctrl Pts',(8.74741430706783,-17.347746182655,-319.906522608289)) ;
#24667=CARTESIAN_POINT('Ctrl Pts',(8.33090634608313,-17.5481251578087,-319.912088834451)) ;
#24668=CARTESIAN_POINT('Ctrl Pts',(8.24013246321081,-17.5909327225883,-319.913304658191)) ;
#24669=CARTESIAN_POINT('Ctrl Pts',(8.08942883746605,-17.660579753382,-319.915330616156)) ;
#24670=CARTESIAN_POINT('Ctrl Pts',(8.02968740904654,-17.687822258951,-319.916135703589)) ;
#24671=CARTESIAN_POINT('Ctrl Pts',(7.92432589743704,-17.7352240328544,-319.917559677219)) ;
#24672=CARTESIAN_POINT('Ctrl Pts',(7.87876427070972,-17.7555114256233,-319.91817671134)) ;
#24673=CARTESIAN_POINT('Ctrl Pts',(7.82757692958262,-17.7780679819389,-319.918871132564)) ;
#24674=CARTESIAN_POINT('Ctrl Pts',(7.82202767007425,-17.7805102538582,-319.918946431086)) ;
#24675=CARTESIAN_POINT('Ctrl Pts',(7.81074339996243,-17.7854702431278,-319.919099579988)) ;
#24676=CARTESIAN_POINT('Ctrl Pts',(7.8050083132647,-17.7879877855563,-319.919177432436)) ;
#24677=CARTESIAN_POINT('Ctrl Pts',(7.79323018271909,-17.7931512621709,-319.91933735082)) ;
#24678=CARTESIAN_POINT('Ctrl Pts',(7.78718700660935,-17.7957968926211,-319.919419420311)) ;
#24679=CARTESIAN_POINT('Ctrl Pts',(7.77466165931191,-17.8012727385397,-319.919589557151)) ;
#24680=CARTESIAN_POINT('Ctrl Pts',(7.76817928770987,-17.8041024930389,-319.919677629826)) ;
#24681=CARTESIAN_POINT('Ctrl Pts',(7.75462795187441,-17.8100092578932,-319.919861785609)) ;
#24682=CARTESIAN_POINT('Ctrl Pts',(7.74755869847941,-17.8130856016534,-319.919957876307)) ;
#24683=CARTESIAN_POINT('Ctrl Pts',(7.73266172770501,-17.819557806239,-319.920160414594)) ;
#24684=CARTESIAN_POINT('Ctrl Pts',(7.72483360061325,-17.8229527196764,-319.920266872797)) ;
#24685=CARTESIAN_POINT('Ctrl Pts',(7.71387065905006,-17.8276985645229,-319.920415999903)) ;
#24686=CARTESIAN_POINT('Ctrl Pts',(7.7107377209296,-17.8290538293841,-319.920458620996)) ;
#24687=CARTESIAN_POINT('Ctrl Pts',(7.70343575019896,-17.8322102743221,-319.920557968169)) ;
#24688=CARTESIAN_POINT('Ctrl Pts',(7.69926644293814,-17.8340108182575,-319.920614701209)) ;
#24689=CARTESIAN_POINT('Ctrl Pts',(7.60415275072753,-17.8750467479181,-319.921909108167)) ;
#24690=CARTESIAN_POINT('Ctrl Pts',(7.51291029900293,-17.9135874157695,-319.923154281409)) ;
#24691=CARTESIAN_POINT('Ctrl Pts',(7.25010073708382,-18.0222366455581,-319.926746682547)) ;
#24692=CARTESIAN_POINT('Ctrl Pts',(7.07781985777919,-18.0905898278586,-319.929108699088)) ;
#24693=CARTESIAN_POINT('Ctrl Pts',(6.34432215931883,-18.3695261993673,-319.939159988119)) ;
#24694=CARTESIAN_POINT('Ctrl Pts',(5.77449513429753,-18.5565385838466,-319.946945282641)) ;
#24695=CARTESIAN_POINT('Ctrl Pts',(4.83650765202176,-18.8169801384299,-319.959413796065)) ;
#24696=CARTESIAN_POINT('Ctrl Pts',(4.47326465659935,-18.9066245590628,-319.964162979456)) ;
#24697=CARTESIAN_POINT('Ctrl Pts',(3.9524197161255,-19.0193120515089,-319.970834996176)) ;
#24698=CARTESIAN_POINT('Ctrl Pts',(3.79677353791587,-19.0509937620902,-319.972811781925)) ;
#24699=CARTESIAN_POINT('Ctrl Pts',(3.51847864256827,-19.10409456639,-319.976315703288)) ;
#24700=CARTESIAN_POINT('Ctrl Pts',(3.39597955153457,-19.1262501314918,-319.977847563879)) ;
#24701=CARTESIAN_POINT('Ctrl Pts',(3.15827358304186,-19.1668866803756,-319.980800302581)) ;
#24702=CARTESIAN_POINT('Ctrl Pts',(3.04309642511415,-19.185510189436,-319.982222054245)) ;
#24703=CARTESIAN_POINT('Ctrl Pts',(2.78826725108276,-19.2243621692534,-319.985348862049)) ;
#24704=CARTESIAN_POINT('Ctrl Pts',(2.64854841155588,-19.2441088765399,-319.987050791772)) ;
#24705=CARTESIAN_POINT('Ctrl Pts',(1.67666385417762,-19.3706821099435,-319.998811253086)) ;
#24706=CARTESIAN_POINT('Ctrl Pts',(0.838559641495929,-19.4250183449035,
-320.008511425644)) ;
#24707=CARTESIAN_POINT('Ctrl Pts',(-0.00042484694712408,-19.4249999953541,
-320.018354222948)) ;
#24708=CARTESIAN_POINT('Origin',(0.,0.,-328.125)) ;
#24709=CARTESIAN_POINT('',(0.000290047970874232,-19.4246600253745,-321.730568038795)) ;
#24710=CARTESIAN_POINT('',(0.0001668108406198,-19.4249999992838,-321.519753599958)) ;
#24711=CARTESIAN_POINT('',(-2.37887640734373E-15,-19.425,-328.125)) ;
#24712=CARTESIAN_POINT('Ctrl Pts',(0.000290047970874162,-19.4246600253745,
-321.730568038795)) ;
#24713=CARTESIAN_POINT('Ctrl Pts',(0.414032815414898,-19.4247115091692,
-321.725584231456)) ;
#24714=CARTESIAN_POINT('Ctrl Pts',(0.827728246191239,-19.4115727824527,
-321.720657750041)) ;
#24715=CARTESIAN_POINT('Ctrl Pts',(1.24054323851937,-19.3852594821658,-321.715754611829)) ;
#24716=CARTESIAN_POINT('Ctrl Pts',(1.67062772321509,-19.3578454046617,-321.710646358227)) ;
#24717=CARTESIAN_POINT('Ctrl Pts',(2.09975668298582,-19.3161309520273,-321.705563481343)) ;
#24718=CARTESIAN_POINT('Ctrl Pts',(2.52698399798445,-19.260178292411,-321.700440001018)) ;
#24719=CARTESIAN_POINT('Ctrl Pts',(2.95421131298308,-19.2042256327946,-321.695316520694)) ;
#24720=CARTESIAN_POINT('Ctrl Pts',(3.37953703303916,-19.1340344813326,-321.690152193862)) ;
#24721=CARTESIAN_POINT('Ctrl Pts',(3.80200981619182,-19.049715863574,-321.68485585614)) ;
#24722=CARTESIAN_POINT('Ctrl Pts',(4.19783357195257,-18.9707159533011,-321.679893604435)) ;
#24723=CARTESIAN_POINT('Ctrl Pts',(4.59123122171946,-18.8792986800034,-321.674814568772)) ;
#24724=CARTESIAN_POINT('Ctrl Pts',(4.98142637903984,-18.775681116706,-321.669695206077)) ;
#24725=CARTESIAN_POINT('Ctrl Pts',(5.37132596310663,-18.6721420438249,-321.664579721305)) ;
#24726=CARTESIAN_POINT('Ctrl Pts',(5.75802798036154,-18.556421336585,-321.659424136884)) ;
#24727=CARTESIAN_POINT('Ctrl Pts',(6.14077663098242,-18.4287730500008,-321.654284881139)) ;
#24728=CARTESIAN_POINT('Ctrl Pts',(6.52348420669083,-18.3011384620729,-321.649146176917)) ;
#24729=CARTESIAN_POINT('Ctrl Pts',(6.9022393361505,-18.1615789550527,-321.644023901516)) ;
#24730=CARTESIAN_POINT('Ctrl Pts',(7.27630416981867,-18.0103839021878,-321.638952587994)) ;
#24731=CARTESIAN_POINT('Ctrl Pts',(7.65034627061387,-17.8591980378316,-321.63388158267)) ;
#24732=CARTESIAN_POINT('Ctrl Pts',(8.01969870178435,-17.6963780755871,-321.628861579192)) ;
#24733=CARTESIAN_POINT('Ctrl Pts',(8.38364048306132,-17.5222477356751,-321.623904110283)) ;
#24734=CARTESIAN_POINT('Ctrl Pts',(8.74815140582929,-17.3478450862719,-321.618938888757)) ;
#24735=CARTESIAN_POINT('Ctrl Pts',(9.1072347687062,-17.1620966214322,-321.614036396023)) ;
#24736=CARTESIAN_POINT('Ctrl Pts',(9.46018237293682,-16.9653621203275,-321.609184808469)) ;
#24737=CARTESIAN_POINT('Ctrl Pts',(9.81261504025612,-16.768914647255,-321.604340299193)) ;
#24738=CARTESIAN_POINT('Ctrl Pts',(10.1589298376583,-16.561513099192,-321.59954647939)) ;
#24739=CARTESIAN_POINT('Ctrl Pts',(10.4984375697143,-16.3435508740133,-321.59476878525)) ;
#24740=CARTESIAN_POINT('Ctrl Pts',(10.838689380338,-16.1251109542049,-321.589980620126)) ;
#24741=CARTESIAN_POINT('Ctrl Pts',(11.1721041965684,-15.896063872729,-321.585208539037)) ;
#24742=CARTESIAN_POINT('Ctrl Pts',(11.4980047302109,-15.6568426433194,-321.58039616376)) ;
#24743=CARTESIAN_POINT('Ctrl Pts',(11.8239052638534,-15.4176214139098,-321.575583788484)) ;
#24744=CARTESIAN_POINT('Ctrl Pts',(12.1422913996453,-15.1682258645773,-321.570730933245)) ;
#24745=CARTESIAN_POINT('Ctrl Pts',(12.4525035634766,-14.9091283489994,-321.565761898795)) ;
#24746=CARTESIAN_POINT('Ctrl Pts',(12.7622922869302,-14.6503845021767,-321.560799647089)) ;
#24747=CARTESIAN_POINT('Ctrl Pts',(13.064009807143,-14.3818973205538,-321.555720611426)) ;
#24748=CARTESIAN_POINT('Ctrl Pts',(13.3570782099071,-14.1042288644385,-321.550601248731)) ;
#24749=CARTESIAN_POINT('Ctrl Pts',(13.6499246130387,-13.8267707424795,-321.545485763959)) ;
#24750=CARTESIAN_POINT('Ctrl Pts',(13.9341351493772,-13.5401453715385,-321.540330179538)) ;
#24751=CARTESIAN_POINT('Ctrl Pts',(14.2091676755129,-13.2449374377241,-321.535190923794)) ;
#24752=CARTESIAN_POINT('Ctrl Pts',(14.4841706863594,-12.9497611843355,-321.530052219571)) ;
#24753=CARTESIAN_POINT('Ctrl Pts',(14.7499977679495,-12.6460042637827,-321.52492994417)) ;
#24754=CARTESIAN_POINT('Ctrl Pts',(15.0061394366358,-12.3342737882764,-321.519858630649)) ;
#24755=CARTESIAN_POINT('Ctrl Pts',(15.2622655389404,-12.0225622574252,-321.514787625324)) ;
#24756=CARTESIAN_POINT('Ctrl Pts',(15.5087074709339,-11.7028781435391,-321.509767621847)) ;
#24757=CARTESIAN_POINT('Ctrl Pts',(15.7449869947941,-11.3758506492204,-321.504810152937)) ;
#24758=CARTESIAN_POINT('Ctrl Pts',(15.9816360186343,-11.0483117409178,-321.499844931411)) ;
#24759=CARTESIAN_POINT('Ctrl Pts',(16.2080908308918,-10.7134064234155,-321.494942438677)) ;
#24760=CARTESIAN_POINT('Ctrl Pts',(16.4239016690412,-10.3717894487278,-321.490090851123)) ;
#24761=CARTESIAN_POINT('Ctrl Pts',(16.6393976475192,-10.0306708800022,-321.485246341847)) ;
#24762=CARTESIAN_POINT('Ctrl Pts',(16.844280651551,-9.68286016179965,-321.480452522044)) ;
#24763=CARTESIAN_POINT('Ctrl Pts',(17.0381336899874,-9.32903247602731,-321.475674827904)) ;
#24764=CARTESIAN_POINT('Ctrl Pts',(17.2324115844077,-8.97442932750882,-321.470886662781)) ;
#24765=CARTESIAN_POINT('Ctrl Pts',(17.4156109923312,-8.61378271078743,-321.466114581691)) ;
#24766=CARTESIAN_POINT('Ctrl Pts',(17.5873443318877,-8.24779689888392,-321.461302206415)) ;
#24767=CARTESIAN_POINT('Ctrl Pts',(17.7590776714444,-7.88181108697985,-321.456489831139)) ;
#24768=CARTESIAN_POINT('Ctrl Pts',(17.9193447591344,-7.51048598400925,-321.4516369759)) ;
#24769=CARTESIAN_POINT('Ctrl Pts',(18.0677923895257,-7.1345519336756,-321.446667941449)) ;
#24770=CARTESIAN_POINT('Ctrl Pts',(18.2160373885304,-6.75913103426062,-321.441705689744)) ;
#24771=CARTESIAN_POINT('Ctrl Pts',(18.3525333826738,-6.37901569349928,-321.436626654081)) ;
#24772=CARTESIAN_POINT('Ctrl Pts',(18.4770417922726,-5.99497596097233,-321.431507291386)) ;
#24773=CARTESIAN_POINT('Ctrl Pts',(18.6014558866162,-5.61122713895869,-321.426391806614)) ;
#24774=CARTESIAN_POINT('Ctrl Pts',(18.7139007423434,-5.22355990194548,-321.421236222193)) ;
#24775=CARTESIAN_POINT('Ctrl Pts',(18.8141800158724,-4.8327470542551,-321.416096966448)) ;
#24776=CARTESIAN_POINT('Ctrl Pts',(18.9144485278681,-4.4419761468915,-321.410958262225)) ;
#24777=CARTESIAN_POINT('Ctrl Pts',(19.002554191957,-4.04806029795157,-321.405835986825)) ;
#24778=CARTESIAN_POINT('Ctrl Pts',(19.0783400732297,-3.65177637953315,-321.400764673303)) ;
#24779=CARTESIAN_POINT('Ctrl Pts',(19.154121348801,-3.25551654429931,-321.395693667978)) ;
#24780=CARTESIAN_POINT('Ctrl Pts',(19.2175843977007,-2.85688889856963,-321.390673664501)) ;
#24781=CARTESIAN_POINT('Ctrl Pts',(19.2686102914582,-2.45667476388441,-321.385716195592)) ;
#24782=CARTESIAN_POINT('Ctrl Pts',(19.3197159808173,-2.05583476406919,-321.380750974066)) ;
#24783=CARTESIAN_POINT('Ctrl Pts',(19.3583455699864,-1.65340326862375,-321.375848481332)) ;
#24784=CARTESIAN_POINT('Ctrl Pts',(19.3844173589335,-1.25017041148229,-321.370996893778)) ;
#24785=CARTESIAN_POINT('Ctrl Pts',(19.4104511101483,-0.847525855492989,
-321.366152384502)) ;
#24786=CARTESIAN_POINT('Ctrl Pts',(19.4239636157988,-0.444082237091322,
-321.361358564699)) ;
#24787=CARTESIAN_POINT('Ctrl Pts',(19.4249117274997,-0.0406319516599588,
-321.356580870559)) ;
#24788=CARTESIAN_POINT('Ctrl Pts',(19.4258619171197,0.363702551368296,-321.351792705436)) ;
#24789=CARTESIAN_POINT('Ctrl Pts',(19.4141924266424,0.768043778808558,-321.347020624346)) ;
#24790=CARTESIAN_POINT('Ctrl Pts',(19.3898998507143,1.17158785965311,-321.34220824907)) ;
#24791=CARTESIAN_POINT('Ctrl Pts',(19.3656072747863,1.57513194049767,-321.337395873794)) ;
#24792=CARTESIAN_POINT('Ctrl Pts',(19.3286914063978,1.9778788711547,-321.332543018555)) ;
#24793=CARTESIAN_POINT('Ctrl Pts',(19.2791914999854,2.37901833372837,-321.327573984104)) ;
#24794=CARTESIAN_POINT('Ctrl Pts',(19.229759161069,2.7796102399332,-321.322611732398)) ;
#24795=CARTESIAN_POINT('Ctrl Pts',(19.1677637480264,3.17870345894468,-321.317532696735)) ;
#24796=CARTESIAN_POINT('Ctrl Pts',(19.0933641677198,3.57550764575502,-321.312413334041)) ;
#24797=CARTESIAN_POINT('Ctrl Pts',(19.0190209451758,3.97201125296411,-321.307297849269)) ;
#24798=CARTESIAN_POINT('Ctrl Pts',(18.9322925248851,4.36622935674251,-321.302142264847)) ;
#24799=CARTESIAN_POINT('Ctrl Pts',(18.8333762203775,4.7573893998477,-321.297003009103)) ;
#24800=CARTESIAN_POINT('Ctrl Pts',(18.7344705311356,5.14850746536595,-321.29186430488)) ;
#24801=CARTESIAN_POINT('Ctrl Pts',(18.6233796788519,5.53656819080653,-321.286742029479)) ;
#24802=CARTESIAN_POINT('Ctrl Pts',(18.5003375290666,5.92081430096648,-321.281670715958)) ;
#24803=CARTESIAN_POINT('Ctrl Pts',(18.3773028568661,6.30503705951135,-321.276599710633)) ;
#24804=CARTESIAN_POINT('Ctrl Pts',(18.2423183775642,6.6854457198535,-321.271579707156)) ;
#24805=CARTESIAN_POINT('Ctrl Pts',(18.0956534599684,7.06129728281752,-321.266622238246)) ;
#24806=CARTESIAN_POINT('Ctrl Pts',(17.9487591840125,7.43773661209638,-321.26165701672)) ;
#24807=CARTESIAN_POINT('Ctrl Pts',(17.790147875683,7.80960460824021,-321.256754523986)) ;
#24808=CARTESIAN_POINT('Ctrl Pts',(17.6201258112138,8.17616834465075,-321.251902936432)) ;
#24809=CARTESIAN_POINT('Ctrl Pts',(17.4503518023654,8.54219727873751,-321.247058427156)) ;
#24810=CARTESIAN_POINT('Ctrl Pts',(17.2692002371063,8.9029374226659,-321.242264607353)) ;
#24811=CARTESIAN_POINT('Ctrl Pts',(17.0770123269122,9.25767230804478,-321.237486913213)) ;
#24812=CARTESIAN_POINT('Ctrl Pts',(16.8844032100947,9.61318464442543,-321.23269874809)) ;
#24813=CARTESIAN_POINT('Ctrl Pts',(16.6807091725345,9.96266532240178,-321.227926667)) ;
#24814=CARTESIAN_POINT('Ctrl Pts',(16.4663118154245,10.305406810545,-321.223114291724)) ;
#24815=CARTESIAN_POINT('Ctrl Pts',(16.2519144583145,10.6481482986883,-321.218301916447)) ;
#24816=CARTESIAN_POINT('Ctrl Pts',(16.0268136015923,10.9841504948062,-321.213449061208)) ;
#24817=CARTESIAN_POINT('Ctrl Pts',(15.7914313915858,11.312720615757,-321.208480026758)) ;
#24818=CARTESIAN_POINT('Ctrl Pts',(15.5563704788845,11.6408422376712,-321.203517775052)) ;
#24819=CARTESIAN_POINT('Ctrl Pts',(15.3109945784651,11.9616373376846,-321.198438739389)) ;
#24820=CARTESIAN_POINT('Ctrl Pts',(15.05582135137,12.2744879160667,-321.193319376694)) ;
#24821=CARTESIAN_POINT('Ctrl Pts',(14.8008414182699,12.5871015097979,-321.188203891922)) ;
#24822=CARTESIAN_POINT('Ctrl Pts',(14.536079127922,12.8917827560929,-321.183048307501)) ;
#24823=CARTESIAN_POINT('Ctrl Pts',(14.2620773572675,13.1879476498576,-321.177909051757)) ;
#24824=CARTESIAN_POINT('Ctrl Pts',(13.9881049912851,13.4840807605007,-321.172770347534)) ;
#24825=CARTESIAN_POINT('Ctrl Pts',(13.7048951897873,13.7716994532655,-321.167648072133)) ;
#24826=CARTESIAN_POINT('Ctrl Pts',(13.4130156157825,14.0502506300313,-321.162576758612)) ;
#24827=CARTESIAN_POINT('Ctrl Pts',(13.1211537800441,14.3287848785315,-321.157505753287)) ;
#24828=CARTESIAN_POINT('Ctrl Pts',(12.8206232331792,14.5982527781373,-321.15248574981)) ;
#24829=CARTESIAN_POINT('Ctrl Pts',(12.5120159846361,14.8581307525481,-321.147528280901)) ;
#24830=CARTESIAN_POINT('Ctrl Pts',(12.2029261281643,15.1184151307991,-321.142563059374)) ;
#24831=CARTESIAN_POINT('Ctrl Pts',(11.8857342464352,15.3690795755255,-321.13766056664)) ;
#24832=CARTESIAN_POINT('Ctrl Pts',(11.561059939402,15.6096270128608,-321.132808979086)) ;
#24833=CARTESIAN_POINT('Ctrl Pts',(11.2368593196308,15.8498235007846,-321.127964469811)) ;
#24834=CARTESIAN_POINT('Ctrl Pts',(10.9051980271681,16.0799324491565,-321.123170650007)) ;
#24835=CARTESIAN_POINT('Ctrl Pts',(10.566718465597,16.2994879504073,-321.118392955867)) ;
#24836=CARTESIAN_POINT('Ctrl Pts',(10.2274970788384,16.5195246381739,-321.113604790744)) ;
#24837=CARTESIAN_POINT('Ctrl Pts',(9.88142739749476,16.7289614564954,-321.108832709654)) ;
#24838=CARTESIAN_POINT('Ctrl Pts',(9.52918301685861,16.927359669034,-321.104020334378)) ;
#24839=CARTESIAN_POINT('Ctrl Pts',(9.176938636223,17.1257578815723,-321.099207959102)) ;
#24840=CARTESIAN_POINT('Ctrl Pts',(8.8185194470681,17.3131173124428,-321.094355103863)) ;
#24841=CARTESIAN_POINT('Ctrl Pts',(8.45462759259423,17.489031573986,-321.089386069413)) ;
#24842=CARTESIAN_POINT('Ctrl Pts',(8.09123245140864,17.6647057121238,-321.084423817707)) ;
#24843=CARTESIAN_POINT('Ctrl Pts',(7.72228461027938,17.8290112787533,-321.079344782044)) ;
#24844=CARTESIAN_POINT('Ctrl Pts',(7.3485343084101,17.9816532522498,-321.074225419349)) ;
#24845=CARTESIAN_POINT('Ctrl Pts',(6.97506712280469,18.1341795992839,-321.069109934577)) ;
#24846=CARTESIAN_POINT('Ctrl Pts',(6.59680479711167,18.2750602054356,-321.063954350156)) ;
#24847=CARTESIAN_POINT('Ctrl Pts',(6.21450344947429,18.4040419646482,-321.058815094411)) ;
#24848=CARTESIAN_POINT('Ctrl Pts',(5.83224312874678,18.533009882102,-321.053676390189)) ;
#24849=CARTESIAN_POINT('Ctrl Pts',(5.44594465608023,18.6500816297685,-321.048554114788)) ;
#24850=CARTESIAN_POINT('Ctrl Pts',(5.05637112832498,18.7550431001519,-321.043482801267)) ;
#24851=CARTESIAN_POINT('Ctrl Pts',(4.66682127594615,18.8599981917593,-321.038411795942)) ;
#24852=CARTESIAN_POINT('Ctrl Pts',(4.27399674213582,18.9528445387418,-321.033391792465)) ;
#24853=CARTESIAN_POINT('Ctrl Pts',(3.87866787909253,19.0334056054948,-321.028434323556)) ;
#24854=CARTESIAN_POINT('Ctrl Pts',(3.48272079062339,19.1140926557123,-321.023469102029)) ;
#24855=CARTESIAN_POINT('Ctrl Pts',(3.08426149227695,19.1824559591042,-321.018566609295)) ;
#24856=CARTESIAN_POINT('Ctrl Pts',(2.68407188485392,19.2383554525851,-321.013715021741)) ;
#24857=CARTESIAN_POINT('Ctrl Pts',(2.28446613860959,19.2941733908642,-321.008870512465)) ;
#24858=CARTESIAN_POINT('Ctrl Pts',(1.88313508674887,19.3375638027708,-321.004076692662)) ;
#24859=CARTESIAN_POINT('Ctrl Pts',(1.48086574387704,19.3684249030544,-320.999298998522)) ;
#24860=CARTESIAN_POINT('Ctrl Pts',(1.07771477159253,19.3993536397468,-320.994510833399)) ;
#24861=CARTESIAN_POINT('Ctrl Pts',(0.673621351637577,19.4176979351181,-320.989738752309)) ;
#24862=CARTESIAN_POINT('Ctrl Pts',(0.269386889573299,19.4233947866315,-320.984926377033)) ;
#24863=CARTESIAN_POINT('Ctrl Pts',(-0.134847572490978,19.4290916381448,
-320.980114001757)) ;
#24864=CARTESIAN_POINT('Ctrl Pts',(-0.53922308843213,19.4221408390945,-320.975261146517)) ;
#24865=CARTESIAN_POINT('Ctrl Pts',(-0.942928660350018,19.4025214512654,
-320.970292112067)) ;
#24866=CARTESIAN_POINT('Ctrl Pts',(-1.34608317314376,19.3829288439501,-320.965329860361)) ;
#24867=CARTESIAN_POINT('Ctrl Pts',(-1.7486746688856,19.3506966200822,-320.960250824698)) ;
#24868=CARTESIAN_POINT('Ctrl Pts',(-2.14990319542456,19.3059246454638,-320.955131462003)) ;
#24869=CARTESIAN_POINT('Ctrl Pts',(-2.55082779093171,19.2611865856635,-320.950015977231)) ;
#24870=CARTESIAN_POINT('Ctrl Pts',(-2.95039152971364,19.2039279540645,-320.94486039281)) ;
#24871=CARTESIAN_POINT('Ctrl Pts',(-3.34780935058607,19.1342882363624,-320.939721137065)) ;
#24872=CARTESIAN_POINT('Ctrl Pts',(-3.74518452231466,19.0646559920904,-320.934582432843)) ;
#24873=CARTESIAN_POINT('Ctrl Pts',(-4.14041429297184,18.9826454288304,-320.929460157441)) ;
#24874=CARTESIAN_POINT('Ctrl Pts',(-4.53272613103421,18.8884336168186,-320.92438884392)) ;
#24875=CARTESIAN_POINT('Ctrl Pts',(-4.92501412730606,18.7942275302987,-320.919317838595)) ;
#24876=CARTESIAN_POINT('Ctrl Pts',(-5.31438459612526,18.6878217196654,-320.914297835118)) ;
#24877=CARTESIAN_POINT('Ctrl Pts',(-5.70007661014937,18.5694297192463,-320.909340366208)) ;
#24878=CARTESIAN_POINT('Ctrl Pts',(-6.08637177921826,18.4508525743862,-320.904375144682)) ;
#24879=CARTESIAN_POINT('Ctrl Pts',(-6.46897701035329,18.3202516908264,-320.899472651948)) ;
#24880=CARTESIAN_POINT('Ctrl Pts',(-6.84713868439783,18.177878155596,-320.894621064394)) ;
#24881=CARTESIAN_POINT('Ctrl Pts',(-7.22474863519534,18.0357123378434,-320.889776555118)) ;
#24882=CARTESIAN_POINT('Ctrl Pts',(-7.59792799415087,17.8818081238135,-320.884982735315)) ;
#24883=CARTESIAN_POINT('Ctrl Pts',(-7.9659369645801,17.7164526599707,-320.880205041174)) ;
#24884=CARTESIAN_POINT('Ctrl Pts',(-8.33475247799237,17.5507347965677,-320.875416876051)) ;
#24885=CARTESIAN_POINT('Ctrl Pts',(-8.69837487756646,17.3735152837348,-320.870644794961)) ;
#24886=CARTESIAN_POINT('Ctrl Pts',(-9.05607028410433,17.1851222091369,-320.865832419686)) ;
#24887=CARTESIAN_POINT('Ctrl Pts',(-9.41376569064274,16.9967291345388,-320.86102004441)) ;
#24888=CARTESIAN_POINT('Ctrl Pts',(-9.76553401558552,16.7971623110319,-320.856167189171)) ;
#24889=CARTESIAN_POINT('Ctrl Pts',(-10.110653081025,16.5867913533777,-320.851198154721)) ;
#24890=CARTESIAN_POINT('Ctrl Pts',(-10.4553010580933,16.376707552597,-320.846235903015)) ;
#24891=CARTESIAN_POINT('Ctrl Pts',(-10.7934075323238,16.1557939025365,-320.841156867352)) ;
#24892=CARTESIAN_POINT('Ctrl Pts',(-11.1243178209923,15.9245208148808,-320.836037504658)) ;
#24893=CARTESIAN_POINT('Ctrl Pts',(-11.4549774447451,15.693422916849,-320.830922019886)) ;
#24894=CARTESIAN_POINT('Ctrl Pts',(-11.7784519136435,15.4519814121514,-320.825766435465)) ;
#24895=CARTESIAN_POINT('Ctrl Pts',(-12.0941185762736,15.2006943796362,-320.820627179721)) ;
#24896=CARTESIAN_POINT('Ctrl Pts',(-12.4097513629371,14.949434314147,-320.815488475499)) ;
#24897=CARTESIAN_POINT('Ctrl Pts',(-12.7175781210385,14.6883309034558,-320.810366200098)) ;
#24898=CARTESIAN_POINT('Ctrl Pts',(-13.0170051831817,14.41790923598,-320.805294886577)) ;
#24899=CARTESIAN_POINT('Ctrl Pts',(-13.3164140483794,14.147504002718,-320.800223881253)) ;
#24900=CARTESIAN_POINT('Ctrl Pts',(-13.6074243028103,13.8677816576701,-320.795203877776)) ;
#24901=CARTESIAN_POINT('Ctrl Pts',(-13.8894699143559,13.5792937576966,-320.790246408867)) ;
#24902=CARTESIAN_POINT('Ctrl Pts',(-14.1719565960832,13.2903547129251,-320.785281187341)) ;
#24903=CARTESIAN_POINT('Ctrl Pts',(-14.4454505869314,12.9926226342601,-320.780378694607)) ;
#24904=CARTESIAN_POINT('Ctrl Pts',(-14.7094102384387,12.6866785582528,-320.775527107052)) ;
#24905=CARTESIAN_POINT('Ctrl Pts',(-14.9729847829978,12.3811808428493,-320.770682597777)) ;
#24906=CARTESIAN_POINT('Ctrl Pts',(-15.2270527619927,12.0674950078586,-320.765888777975)) ;
#24907=CARTESIAN_POINT('Ctrl Pts',(-15.4711019165878,11.7462271416504,-320.761111083835)) ;
#24908=CARTESIAN_POINT('Ctrl Pts',(-15.7156859389862,11.424255172049,-320.756322918711)) ;
#24909=CARTESIAN_POINT('Ctrl Pts',(-15.9502070688235,11.0946677862201,-320.751550837621)) ;
#24910=CARTESIAN_POINT('Ctrl Pts',(-16.1741778308489,10.7581041931066,-320.746738462345)) ;
#24911=CARTESIAN_POINT('Ctrl Pts',(-16.3981485928743,10.4215405999931,-320.741926087068)) ;
#24912=CARTESIAN_POINT('Ctrl Pts',(-16.611568819787,10.0780006776278,-320.737073231829)) ;
#24913=CARTESIAN_POINT('Ctrl Pts',(-16.8139811791531,9.72815450290812,-320.732104197378)) ;
#24914=CARTESIAN_POINT('Ctrl Pts',(-17.0161172451294,9.37878586911457,-320.727141945672)) ;
#24915=CARTESIAN_POINT('Ctrl Pts',(-17.2073277650371,9.02303684834942,-320.722062910009)) ;
#24916=CARTESIAN_POINT('Ctrl Pts',(-17.3872628996133,8.66163373883787,-320.716943547313)) ;
#24917=CARTESIAN_POINT('Ctrl Pts',(-17.5670617331351,8.30050439256336,-320.711828062541)) ;
#24918=CARTESIAN_POINT('Ctrl Pts',(-17.7356024416079,7.93372958177536,-320.706672478119)) ;
#24919=CARTESIAN_POINT('Ctrl Pts',(-17.8925765500298,7.56204457546894,-320.701533222374)) ;
#24920=CARTESIAN_POINT('Ctrl Pts',(-18.0495338126759,7.19039945677411,-320.69639451815)) ;
#24921=CARTESIAN_POINT('Ctrl Pts',(-18.1949270805422,6.81384520868004,-320.691272242749)) ;
#24922=CARTESIAN_POINT('Ctrl Pts',(-18.3284862523631,6.43312695139845,-320.686200929227)) ;
#24923=CARTESIAN_POINT('Ctrl Pts',(-18.462037307453,6.0524318313348,-320.681129923901)) ;
#24924=CARTESIAN_POINT('Ctrl Pts',(-18.5837557672299,5.66757318835785,-320.676109920424)) ;
#24925=CARTESIAN_POINT('Ctrl Pts',(-18.6934084609089,5.27930616398755,-320.671152451514)) ;
#24926=CARTESIAN_POINT('Ctrl Pts',(-18.8032326322779,4.89043195770348,-320.666187229987)) ;
#24927=CARTESIAN_POINT('Ctrl Pts',(-18.9009532611929,4.49813865880138,-320.661284737252)) ;
#24928=CARTESIAN_POINT('Ctrl Pts',(-18.9863726926629,4.10319563002595,-320.656433149698)) ;
#24929=CARTESIAN_POINT('Ctrl Pts',(-19.0716675004877,3.70882880784667,-320.651588640422)) ;
#24930=CARTESIAN_POINT('Ctrl Pts',(-19.1446969235176,3.31181993588284,-320.646794820618)) ;
#24931=CARTESIAN_POINT('Ctrl Pts',(-19.2053011000377,2.91294631488644,-320.642017126478)) ;
#24932=CARTESIAN_POINT('Ctrl Pts',(-19.2660380990631,2.51319850671871,-320.637228961355)) ;
#24933=CARTESIAN_POINT('Ctrl Pts',(-19.3142951818603,2.11157771646767,-320.632456880265)) ;
#24934=CARTESIAN_POINT('Ctrl Pts',(-19.3499500955848,1.70887847193987,-320.627644504989)) ;
#24935=CARTESIAN_POINT('Ctrl Pts',(-19.3856050093094,1.30617922741152,-320.622832129714)) ;
#24936=CARTESIAN_POINT('Ctrl Pts',(-19.4086575486974,0.902401501544134,
-320.617979274475)) ;
#24937=CARTESIAN_POINT('Ctrl Pts',(-19.4190266981606,0.498352507120491,
-320.613010240025)) ;
#24938=CARTESIAN_POINT('Ctrl Pts',(-19.4293816937094,0.0948550405670599,
-320.60804798832)) ;
#24939=CARTESIAN_POINT('Ctrl Pts',(-19.4270901203735,-0.30901817888565,
-320.602968952658)) ;
#24940=CARTESIAN_POINT('Ctrl Pts',(-19.412192253063,-0.712461996250404,
-320.597849589965)) ;
#24941=CARTESIAN_POINT('Ctrl Pts',(-19.3973056709019,-1.11560020451891,
-320.592734105193)) ;
#24942=CARTESIAN_POINT('Ctrl Pts',(-19.3698320775587,-1.51830969525372,
-320.587578520773)) ;
#24943=CARTESIAN_POINT('Ctrl Pts',(-19.329852362925,-1.91979722564955,-320.582439265029)) ;
#24944=CARTESIAN_POINT('Ctrl Pts',(-19.2898769387396,-2.3212416701581,-320.577300560808)) ;
#24945=CARTESIAN_POINT('Ctrl Pts',(-19.2373981910851,-2.72146446456308,
-320.572178285407)) ;
#24946=CARTESIAN_POINT('Ctrl Pts',(-19.1725354199955,-3.11968207435652,
-320.567106971887)) ;
#24947=CARTESIAN_POINT('Ctrl Pts',(-19.1076765907817,-3.5178754834518,-320.562035966563)) ;
#24948=CARTESIAN_POINT('Ctrl Pts',(-19.0304352886145,-3.91406399891133,
-320.557015963087)) ;
#24949=CARTESIAN_POINT('Ctrl Pts',(-18.9409680376835,-4.3074729546733,-320.552058494178)) ;
#24950=CARTESIAN_POINT('Ctrl Pts',(-18.8513608755838,-4.70149713339378,
-320.547093272653)) ;
#24951=CARTESIAN_POINT('Ctrl Pts',(-18.7494894677073,-5.09273308511964,
-320.542190779921)) ;
#24952=CARTESIAN_POINT('Ctrl Pts',(-18.6355483294643,-5.48041064734489,
-320.537339192368)) ;
#24953=CARTESIAN_POINT('Ctrl Pts',(-18.5217734269216,-5.86752260304727,
-320.532494683093)) ;
#24954=CARTESIAN_POINT('Ctrl Pts',(-18.3959639164691,-6.25108655878862,
-320.527700863289)) ;
#24955=CARTESIAN_POINT('Ctrl Pts',(-18.258351298614,-6.63034346269879,-320.522923169149)) ;
#24956=CARTESIAN_POINT('Ctrl Pts',(-18.1204370835338,-7.01043156095392,
-320.518135004027)) ;
#24957=CARTESIAN_POINT('Ctrl Pts',(-17.9706678151123,-7.38619368172872,
-320.513362922937)) ;
#24958=CARTESIAN_POINT('Ctrl Pts',(-17.8093162611297,-7.75687363858416,
-320.508550547661)) ;
#24959=CARTESIAN_POINT('Ctrl Pts',(-17.647964707147,-8.1275535954396,-320.503738172385)) ;
#24960=CARTESIAN_POINT('Ctrl Pts',(-17.4750306744082,-8.49315131393668,
-320.498885317146)) ;
#24961=CARTESIAN_POINT('Ctrl Pts',(-17.2908292111163,-8.85291919750511,
-320.493916282695)) ;
#24962=CARTESIAN_POINT('Ctrl Pts',(-17.1068791832579,-9.21219599706071,
-320.488954030987)) ;
#24963=CARTESIAN_POINT('Ctrl Pts',(-16.9116440705943,-9.5657523284759,-320.483874995323)) ;
#24964=CARTESIAN_POINT('Ctrl Pts',(-16.7055444454999,-9.91290043052715,
-320.478755632626)) ;
#24965=CARTESIAN_POINT('Ctrl Pts',(-16.4996009411783,-10.2597855673743,
-320.473640147854)) ;
#24966=CARTESIAN_POINT('Ctrl Pts',(-16.2828095297037,-10.60027230135,-320.468484563432)) ;
#24967=CARTESIAN_POINT('Ctrl Pts',(-16.0556207495516,-10.9337027628606,
-320.463345307687)) ;
#24968=CARTESIAN_POINT('Ctrl Pts',(-15.8284563503074,-11.26709744207,-320.458206603465)) ;
#24969=CARTESIAN_POINT('Ctrl Pts',(-15.5908968908092,-11.5934374597872,
-320.453084328063)) ;
#24970=CARTESIAN_POINT('Ctrl Pts',(-15.3434219938976,-11.9120918479036,
-320.448013014542)) ;
#24971=CARTESIAN_POINT('Ctrl Pts',(-15.0959621366668,-12.23072687058,-320.442942009217)) ;
#24972=CARTESIAN_POINT('Ctrl Pts',(-14.8385880643354,-12.5416772609582,
-320.43792200574)) ;
#24973=CARTESIAN_POINT('Ctrl Pts',(-14.5718078444623,-12.8443376475125,
-320.43296453683)) ;
#24974=CARTESIAN_POINT('Ctrl Pts',(-14.3046104266468,-13.14747134236,-320.4279993153)) ;
#24975=CARTESIAN_POINT('Ctrl Pts',(-14.0279773782128,-13.44228910014,-320.423096822563)) ;
#24976=CARTESIAN_POINT('Ctrl Pts',(-13.7424479732906,-13.7282076799566,
-320.418245235006)) ;
#24977=CARTESIAN_POINT('Ctrl Pts',(-13.4573351449372,-14.0137091154131,
-320.413400725732)) ;
#24978=CARTESIAN_POINT('Ctrl Pts',(-13.1633518315393,-14.2903372997161,
-320.40860690593)) ;
#24979=CARTESIAN_POINT('Ctrl Pts',(-12.8610644693045,-14.5575364431122,
-320.403829211792)) ;
#24980=CARTESIAN_POINT('Ctrl Pts',(-12.5581146018111,-14.8253211910017,
-320.399041046665)) ;
#24981=CARTESIAN_POINT('Ctrl Pts',(-12.2468241247313,-15.0836354265973,
-320.394268965572)) ;
#24982=CARTESIAN_POINT('Ctrl Pts',(-11.9277943413587,-15.3319456196343,
-320.389456590294)) ;
#24983=CARTESIAN_POINT('Ctrl Pts',(-11.6087645579866,-15.580255812671,-320.384644215016)) ;
#24984=CARTESIAN_POINT('Ctrl Pts',(-11.2819953342844,-15.8185618053519,
-320.379791359776)) ;
#24985=CARTESIAN_POINT('Ctrl Pts',(-10.9481209915988,-16.0463578384104,
-320.374822325325)) ;
#24986=CARTESIAN_POINT('Ctrl Pts',(-10.6147023884452,-16.2738429291644,
-320.369860073621)) ;
#24987=CARTESIAN_POINT('Ctrl Pts',(-10.2741108398708,-16.4909056522041,
-320.364781037961)) ;
#24988=CARTESIAN_POINT('Ctrl Pts',(-9.92704470433196,-16.6971432767429,
-320.35966167527)) ;
#24989=CARTESIAN_POINT('Ctrl Pts',(-9.58024147137529,-16.9032246762903,
-320.354546190495)) ;
#24990=CARTESIAN_POINT('Ctrl Pts',(-9.22697353177151,-17.0984975505992,
-320.349390606071)) ;
#24991=CARTESIAN_POINT('Ctrl Pts',(-8.86795125718945,-17.2825997540949,
-320.344251350324)) ;
#24992=CARTESIAN_POINT('Ctrl Pts',(-8.50896751130765,-17.4666822005474,
-320.339112646099)) ;
#24993=CARTESIAN_POINT('Ctrl Pts',(-8.14423068681169,-17.6395964952344,
-320.333990370695)) ;
#24994=CARTESIAN_POINT('Ctrl Pts',(-7.77446382485693,-17.8010180302188,
-320.328919057171)) ;
#24995=CARTESIAN_POINT('Ctrl Pts',(-7.40471943457631,-17.9624297552054,
-320.323848051844)) ;
#24996=CARTESIAN_POINT('Ctrl Pts',(-7.02994560305102,-18.1123501810341,
-320.318828048364)) ;
#24997=CARTESIAN_POINT('Ctrl Pts',(-6.65087810353198,-18.2504907855099,
-320.313870579451)) ;
#24998=CARTESIAN_POINT('Ctrl Pts',(-6.27121780928545,-18.3888474175324,
-320.308905357931)) ;
#24999=CARTESIAN_POINT('Ctrl Pts',(-5.8872503642293,-18.5153873501159,-320.304002865202)) ;
#25000=CARTESIAN_POINT('Ctrl Pts',(-5.49972835716007,-18.6298564245958,
-320.299151277653)) ;
#25001=CARTESIAN_POINT('Ctrl Pts',(-5.11277172896239,-18.7441584933445,
-320.294306768373)) ;
#25002=CARTESIAN_POINT('Ctrl Pts',(-4.72227085317129,-18.8464248485324,
-320.289512948564)) ;
#25003=CARTESIAN_POINT('Ctrl Pts',(-4.32898903709246,-18.936438432132,-320.284735254419)) ;
#25004=CARTESIAN_POINT('Ctrl Pts',(-3.93484529019412,-19.0266492927953,
-320.279947089303)) ;
#25005=CARTESIAN_POINT('Ctrl Pts',(-3.53790833891072,-19.1045534731966,
-320.275175008221)) ;
#25006=CARTESIAN_POINT('Ctrl Pts',(-3.13896145884664,-19.1699701432719,
-320.270362632951)) ;
#25007=CARTESIAN_POINT('Ctrl Pts',(-2.74001457878256,-19.2353868133472,
-320.265550257682)) ;
#25008=CARTESIAN_POINT('Ctrl Pts',(-2.33905772772985,-19.2883157704039,
-320.260697402449)) ;
#25009=CARTESIAN_POINT('Ctrl Pts',(-1.93688988906811,-19.328616367532,-320.255728368006)) ;
#25010=CARTESIAN_POINT('Ctrl Pts',(-1.51041267919678,-19.3713529679437,
-320.250458976121)) ;
#25011=CARTESIAN_POINT('Ctrl Pts',(-1.08250600421025,-19.3998956153957,
-320.245058602151)) ;
#25012=CARTESIAN_POINT('Ctrl Pts',(-0.654080804362692,-19.4142304696164,
-320.239617595496)) ;
#25013=CARTESIAN_POINT('Ctrl Pts',(-0.436310818107926,-19.4215169247729,
-320.236851913307)) ;
#25014=CARTESIAN_POINT('Ctrl Pts',(-0.218406684945227,-19.425133126111,
-320.234075356998)) ;
#25015=CARTESIAN_POINT('Ctrl Pts',(-0.000487082238699813,-19.4250810872335,
-320.231297307284)) ;
#25016=CARTESIAN_POINT('Ctrl Pts',(-0.000424878507915977,-19.4249999953534,
-320.018354223318)) ;
#25017=CARTESIAN_POINT('Ctrl Pts',(-0.220439294652272,-19.4249951830292,
-320.020935388206)) ;
#25018=CARTESIAN_POINT('Ctrl Pts',(-0.440437550926895,-19.421252428869,
-320.023528335593)) ;
#25019=CARTESIAN_POINT('Ctrl Pts',(-0.78548262287532,-19.4095163454399,
-320.027639313526)) ;
#25020=CARTESIAN_POINT('Ctrl Pts',(-0.910596685962431,-19.4040490962108,
-320.029139135506)) ;
#25021=CARTESIAN_POINT('Ctrl Pts',(-1.10739528474174,-19.3935417830338,
-320.031517929406)) ;
#25022=CARTESIAN_POINT('Ctrl Pts',(-1.1791197437356,-19.3893131343616,-320.032389010415)) ;
#25023=CARTESIAN_POINT('Ctrl Pts',(-1.31120037394053,-19.3807904809346,
-320.034001899657)) ;
#25024=CARTESIAN_POINT('Ctrl Pts',(-1.37156315633409,-19.376612206174,-320.034742400884)) ;
#25025=CARTESIAN_POINT('Ctrl Pts',(-1.4941388467024,-19.3675519431011,-320.036253803258)) ;
#25026=CARTESIAN_POINT('Ctrl Pts',(-1.55634972259543,-19.3626520572994,
-320.037024904116)) ;
#25027=CARTESIAN_POINT('Ctrl Pts',(-1.73302778372234,-19.3478794637681,
-320.03922516689)) ;
#25028=CARTESIAN_POINT('Ctrl Pts',(-1.84743241083146,-19.3372908773168,
-320.040662246313)) ;
#25029=CARTESIAN_POINT('Ctrl Pts',(-2.51899856859356,-19.269120696112,-320.049157452439)) ;
#25030=CARTESIAN_POINT('Ctrl Pts',(-3.07355301092097,-19.1884766746646,
-320.05640503644)) ;
#25031=CARTESIAN_POINT('Ctrl Pts',(-4.16681678102497,-18.9808775350747,
-320.070759059273)) ;
#25032=CARTESIAN_POINT('Ctrl Pts',(-4.70514252555136,-18.8546469368251,
-320.077859132195)) ;
#25033=CARTESIAN_POINT('Ctrl Pts',(-5.34313834958395,-18.6760157813397,
-320.086203723355)) ;
#25034=CARTESIAN_POINT('Ctrl Pts',(-5.44867097281211,-18.6455001957067,
-320.087582024436)) ;
#25035=CARTESIAN_POINT('Ctrl Pts',(-5.63606412821575,-18.5895871686054,
-320.090025512931)) ;
#25036=CARTESIAN_POINT('Ctrl Pts',(-5.71802610910746,-18.5645400532082,
-320.091092896228)) ;
#25037=CARTESIAN_POINT('Ctrl Pts',(-5.91077804529786,-18.5042385586038,
-320.093599832642)) ;
#25038=CARTESIAN_POINT('Ctrl Pts',(-6.02142259752397,-18.4685303063039,
-320.095036323819)) ;
#25039=CARTESIAN_POINT('Ctrl Pts',(-6.2515509311789,-18.391973228862,-320.098018954803)) ;
#25040=CARTESIAN_POINT('Ctrl Pts',(-6.37097048712458,-18.3509482969429,
-320.09956381738)) ;
#25041=CARTESIAN_POINT('Ctrl Pts',(-6.6355446054671,-18.2571636282723,-320.102980938717)) ;
#25042=CARTESIAN_POINT('Ctrl Pts',(-6.78048715562218,-18.2038311895277,
-320.1048492048)) ;
#25043=CARTESIAN_POINT('Ctrl Pts',(-7.73899609875098,-17.8381061373385,
-320.117188268857)) ;
#25044=CARTESIAN_POINT('Ctrl Pts',(-8.5313808885285,-17.472997089213,-320.127261194052)) ;
#25045=CARTESIAN_POINT('Ctrl Pts',(-9.49596775878819,-16.9472356014124,
-320.140149965992)) ;
#25046=CARTESIAN_POINT('Ctrl Pts',(-9.69344674455519,-16.835061276245,-320.142826951084)) ;
#25047=CARTESIAN_POINT('Ctrl Pts',(-9.9853888452008,-16.6623887308148,-320.146868864881)) ;
#25048=CARTESIAN_POINT('Ctrl Pts',(-10.0813688111153,-16.6044931104927,
-320.148211648081)) ;
#25049=CARTESIAN_POINT('Ctrl Pts',(-10.2547772128668,-16.4978344338597,
-320.150667449441)) ;
#25050=CARTESIAN_POINT('Ctrl Pts',(-10.3323724986371,-16.4493487777329,
-320.15177733462)) ;
#25051=CARTESIAN_POINT('Ctrl Pts',(-10.4496130117665,-16.3749337849397,
-320.153473094128)) ;
#25052=CARTESIAN_POINT('Ctrl Pts',(-10.489510801058,-16.3494046286352,-320.15405351154)) ;
#25053=CARTESIAN_POINT('Ctrl Pts',(-10.5820760261814,-16.2896971715659,
-320.155408340507)) ;
#25054=CARTESIAN_POINT('Ctrl Pts',(-10.634671893511,-16.2554089666032,-320.156184354536)) ;
#25055=CARTESIAN_POINT('Ctrl Pts',(-10.78487021505,-16.1564509623323,-320.158417125532)) ;
#25056=CARTESIAN_POINT('Ctrl Pts',(-10.8820553881146,-16.0911529643991,
-320.159882160242)) ;
#25057=CARTESIAN_POINT('Ctrl Pts',(-11.4454807756514,-15.7051526904405,
-320.168481132176)) ;
#25058=CARTESIAN_POINT('Ctrl Pts',(-11.8981183463151,-15.3650782661189,
-320.175806095342)) ;
#25059=CARTESIAN_POINT('Ctrl Pts',(-12.6441351764165,-14.7518250170382,
-320.188261826382)) ;
#25060=CARTESIAN_POINT('Ctrl Pts',(-12.9450959374776,-14.4884432500845,
-320.193404852506)) ;
#25061=CARTESIAN_POINT('Ctrl Pts',(-13.3819765467053,-14.0816258454257,
-320.200992949248)) ;
#25062=CARTESIAN_POINT('Ctrl Pts',(-13.5241861620525,-13.9451020636554,
-320.203483890397)) ;
#25063=CARTESIAN_POINT('Ctrl Pts',(-13.6755581650385,-13.7952885097983,
-320.206155988898)) ;
#25064=CARTESIAN_POINT('Ctrl Pts',(-13.6868093607018,-13.7841258597643,
-320.206354727402)) ;
#25065=CARTESIAN_POINT('Ctrl Pts',(-13.7077210526861,-13.7633278935611,
-320.206724341157)) ;
#25066=CARTESIAN_POINT('Ctrl Pts',(-13.7173850829667,-13.753696145022,-320.20689524621)) ;
#25067=CARTESIAN_POINT('Ctrl Pts',(-13.7354298052367,-13.7356737622817,
-320.207214535239)) ;
#25068=CARTESIAN_POINT('Ctrl Pts',(-13.7438129768697,-13.727285620081,-320.207362940261)) ;
#25069=CARTESIAN_POINT('Ctrl Pts',(-13.7595397355717,-13.7115206891985,
-320.207641479)) ;
#25070=CARTESIAN_POINT('Ctrl Pts',(-13.7668850850061,-13.7041456647745,
-320.207771627753)) ;
#25071=CARTESIAN_POINT('Ctrl Pts',(-13.7807298950954,-13.6902225576755,
-320.208017039606)) ;
#25072=CARTESIAN_POINT('Ctrl Pts',(-13.7872306253495,-13.6836757416896,
-320.208132313584)) ;
#25073=CARTESIAN_POINT('Ctrl Pts',(-13.7995408367887,-13.6712605812803,
-320.208350684669)) ;
#25074=CARTESIAN_POINT('Ctrl Pts',(-13.8053512449818,-13.6653931590042,
-320.208453789746)) ;
#25075=CARTESIAN_POINT('Ctrl Pts',(-13.8164050986895,-13.654216595234,-320.208650004132)) ;
#25076=CARTESIAN_POINT('Ctrl Pts',(-13.8216492297861,-13.6489081339652,
-320.208743119351)) ;
#25077=CARTESIAN_POINT('Ctrl Pts',(-13.8316712536273,-13.6387514701631,
-320.208921124481)) ;
#25078=CARTESIAN_POINT('Ctrl Pts',(-13.8364496593592,-13.6339037754167,
-320.209006018826)) ;
#25079=CARTESIAN_POINT('Ctrl Pts',(-13.8456226649469,-13.6245879679506,
-320.209169033249)) ;
#25080=CARTESIAN_POINT('Ctrl Pts',(-13.8500176524653,-13.6201202381962,
-320.209247156683)) ;
#25081=CARTESIAN_POINT('Ctrl Pts',(-13.8584920525939,-13.6114972334455,
-320.209397831947)) ;
#25082=CARTESIAN_POINT('Ctrl Pts',(-13.8625717603932,-13.6073422495304,
-320.209470386336)) ;
#25083=CARTESIAN_POINT('Ctrl Pts',(-13.870472820545,-13.5992881629975,-320.209610933356)) ;
#25084=CARTESIAN_POINT('Ctrl Pts',(-13.874294398633,-13.595389282613,-320.209678927948)) ;
#25085=CARTESIAN_POINT('Ctrl Pts',(-13.8817279186758,-13.5877990000008,
-320.209811216274)) ;
#25086=CARTESIAN_POINT('Ctrl Pts',(-13.8853400331506,-13.5841077674006,
-320.209875511509)) ;
#25087=CARTESIAN_POINT('Ctrl Pts',(-13.8923968514882,-13.5768906241003,
-320.210001148208)) ;
#25088=CARTESIAN_POINT('Ctrl Pts',(-13.8958416861789,-13.5733648418761,
-320.21006249081)) ;
#25089=CARTESIAN_POINT('Ctrl Pts',(-13.9026013145281,-13.5664411038134,
-320.210182884267)) ;
#25090=CARTESIAN_POINT('Ctrl Pts',(-13.9059162054164,-13.5630432433836,
-320.210241935968)) ;
#25091=CARTESIAN_POINT('Ctrl Pts',(-13.9124498383915,-13.5563411646504,
-320.210358348851)) ;
#25092=CARTESIAN_POINT('Ctrl Pts',(-13.9156686496936,-13.5530370142669,
-320.210415710636)) ;
#25093=CARTESIAN_POINT('Ctrl Pts',(-13.9220417488101,-13.5464902837687,
-320.210529305494)) ;
#25094=CARTESIAN_POINT('Ctrl Pts',(-13.9251960814809,-13.5432477477215,
-320.210585538957)) ;
#25095=CARTESIAN_POINT('Ctrl Pts',(-13.931470705277,-13.5367931594415,-320.210697419456)) ;
#25096=CARTESIAN_POINT('Ctrl Pts',(-13.9345910189265,-13.5335811294995,
-320.210753066688)) ;
#25097=CARTESIAN_POINT('Ctrl Pts',(-13.9408280595978,-13.5271563178918,
-320.210864317331)) ;
#25098=CARTESIAN_POINT('Ctrl Pts',(-13.94394478741,-13.5239435373567,-320.210919920748)) ;
#25099=CARTESIAN_POINT('Ctrl Pts',(-13.9502062814313,-13.517484608186,-320.211031648037)) ;
#25100=CARTESIAN_POINT('Ctrl Pts',(-13.9533510257801,-13.5142384387133,
-320.211087771715)) ;
#25101=CARTESIAN_POINT('Ctrl Pts',(-13.9597027356755,-13.5076772912768,
-320.211201150284)) ;
#25102=CARTESIAN_POINT('Ctrl Pts',(-13.9629096531327,-13.5043622689905,
-320.211258404742)) ;
#25103=CARTESIAN_POINT('Ctrl Pts',(-14.0477157293653,-13.4166348857031,
-320.212772766915)) ;
#25104=CARTESIAN_POINT('Ctrl Pts',(-14.1285491719186,-13.3314855588383,
-320.214223113798)) ;
#25105=CARTESIAN_POINT('Ctrl Pts',(-14.2950132691316,-13.1529190013186,
-320.217224662025)) ;
#25106=CARTESIAN_POINT('Ctrl Pts',(-14.3805117772377,-13.0593860381604,
-320.218774661054)) ;
#25107=CARTESIAN_POINT('Ctrl Pts',(-14.5695101725081,-12.8485203431736,
-320.22222086208)) ;
#25108=CARTESIAN_POINT('Ctrl Pts',(-14.6725201117514,-12.7307602024706,
-320.224112820286)) ;
#25109=CARTESIAN_POINT('Ctrl Pts',(-15.1257546229923,-12.1998171908184,
-320.232505599874)) ;
#25110=CARTESIAN_POINT('Ctrl Pts',(-15.4600296210871,-11.7733375947971,
-320.238874299523)) ;
#25111=CARTESIAN_POINT('Ctrl Pts',(-16.0847629805207,-10.9037150388822,
-320.251392503876)) ;
#25112=CARTESIAN_POINT('Ctrl Pts',(-16.3757928387318,-10.4615490395309,
-320.257539348988)) ;
#25113=CARTESIAN_POINT('Ctrl Pts',(-16.7364408429045,-9.86161087493845,
-320.265863726232)) ;
#25114=CARTESIAN_POINT('Ctrl Pts',(-16.822538826032,-9.71401093370881,-320.267911140453)) ;
#25115=CARTESIAN_POINT('Ctrl Pts',(-16.9458726195778,-9.49601819646844,
-320.270946504288)) ;
#25116=CARTESIAN_POINT('Ctrl Pts',(-16.9846409317898,-9.42650162167603,
-320.271916164946)) ;
#25117=CARTESIAN_POINT('Ctrl Pts',(-17.0549583465851,-9.29857128701474,
-320.273705393738)) ;
#25118=CARTESIAN_POINT('Ctrl Pts',(-17.0866372854264,-9.24023043142591,
-320.274523300756)) ;
#25119=CARTESIAN_POINT('Ctrl Pts',(-17.1642209598768,-9.0955867902831,-320.276555344582)) ;
#25120=CARTESIAN_POINT('Ctrl Pts',(-17.2097744780778,-9.00909776812452,
-320.277773943801)) ;
#25121=CARTESIAN_POINT('Ctrl Pts',(-17.3952865766884,-8.65033804646379,
-320.282837554016)) ;
#25122=CARTESIAN_POINT('Ctrl Pts',(-17.529451757974,-8.3751217203075,-320.286742212298)) ;
#25123=CARTESIAN_POINT('Ctrl Pts',(-17.6975743034572,-8.00849160484377,
-320.29192075144)) ;
#25124=CARTESIAN_POINT('Ctrl Pts',(-17.7374285037688,-7.91982980088143,
-320.29317139258)) ;
#25125=CARTESIAN_POINT('Ctrl Pts',(-17.9907817222782,-7.34470069695094,
-320.301266648444)) ;
#25126=CARTESIAN_POINT('Ctrl Pts',(-18.1849138053504,-6.84994649390582,
-320.308143566171)) ;
#25127=CARTESIAN_POINT('Ctrl Pts',(-18.4092407782897,-6.20117468916909,
-320.316902899096)) ;
#25128=CARTESIAN_POINT('Ctrl Pts',(-18.4582001039537,-6.05388821777947,
-320.318875229424)) ;
#25129=CARTESIAN_POINT('Ctrl Pts',(-18.5740815675654,-5.6907963777677,-320.323694232786)) ;
#25130=CARTESIAN_POINT('Ctrl Pts',(-18.6390138265115,-5.47437972134774,
-320.32652927465)) ;
#25131=CARTESIAN_POINT('Ctrl Pts',(-18.7366499761192,-5.12706126631921,
-320.331017010084)) ;
#25132=CARTESIAN_POINT('Ctrl Pts',(-18.7717909360028,-4.99686648520311,
-320.332685539864)) ;
#25133=CARTESIAN_POINT('Ctrl Pts',(-18.8372701690078,-4.74382610384772,
-320.335902121334)) ;
#25134=CARTESIAN_POINT('Ctrl Pts',(-18.8677694392615,-4.62102910178874,
-320.337451177583)) ;
#25135=CARTESIAN_POINT('Ctrl Pts',(-18.9382459441969,-4.32493835977142,
-320.341158712292)) ;
#25136=CARTESIAN_POINT('Ctrl Pts',(-18.977047324828,-4.15137642439419,-320.343309341665)) ;
#25137=CARTESIAN_POINT('Ctrl Pts',(-19.1644758795531,-3.25537664385854,
-320.354306568579)) ;
#25138=CARTESIAN_POINT('Ctrl Pts',(-19.2742525205538,-2.52543123931449,
-320.362889314961)) ;
#25139=CARTESIAN_POINT('Ctrl Pts',(-19.3797590953652,-1.38600334350933,
-320.376265983712)) ;
#25140=CARTESIAN_POINT('Ctrl Pts',(-19.4045313966715,-0.9799120643945,-320.381035322936)) ;
#25141=CARTESIAN_POINT('Ctrl Pts',(-19.4200624875907,-0.453945494692689,
-320.387345207962)) ;
#25142=CARTESIAN_POINT('Ctrl Pts',(-19.422486762598,-0.334516708063532,
-320.38878697328)) ;
#25143=CARTESIAN_POINT('Ctrl Pts',(-19.4245851967156,-0.145001878873325,
-320.391093834141)) ;
#25144=CARTESIAN_POINT('Ctrl Pts',(-19.4249818940004,-0.0749267703727497,
-320.391950946931)) ;
#25145=CARTESIAN_POINT('Ctrl Pts',(-19.4250150541863,0.0578554226074442,
-320.393584052569)) ;
#25146=CARTESIAN_POINT('Ctrl Pts',(-19.4247270765315,0.120561588172162,
-320.39435905633)) ;
#25147=CARTESIAN_POINT('Ctrl Pts',(-19.4230350858568,0.299894348324802,
-320.396585174918)) ;
#25148=CARTESIAN_POINT('Ctrl Pts',(-19.4208843005822,0.416511092955219,
-320.398044493412)) ;
#25149=CARTESIAN_POINT('Ctrl Pts',(-19.407867602269,0.890631409744478,-320.404015682221)) ;
#25150=CARTESIAN_POINT('Ctrl Pts',(-19.3881791064578,1.2478218379844,-320.408601230701)) ;
#25151=CARTESIAN_POINT('Ctrl Pts',(-19.3539944761441,1.66032754171005,-320.413931910504)) ;
#25152=CARTESIAN_POINT('Ctrl Pts',(-19.3491049124066,1.71637082702257,-320.414656923074)) ;
#25153=CARTESIAN_POINT('Ctrl Pts',(-19.2985323575846,2.26832211220699,-320.42180323578)) ;
#25154=CARTESIAN_POINT('Ctrl Pts',(-19.234037892802,2.76232225453438,-320.428240690546)) ;
#25155=CARTESIAN_POINT('Ctrl Pts',(-19.1255278930104,3.40106964613538,-320.436501444459)) ;
#25156=CARTESIAN_POINT('Ctrl Pts',(-19.0987148116955,3.54854681973166,-320.438404787465)) ;
#25157=CARTESIAN_POINT('Ctrl Pts',(-19.0282202711361,3.91230610441283,-320.443086677832)) ;
#25158=CARTESIAN_POINT('Ctrl Pts',(-18.9825555397607,4.12818255053048,-320.445853828238)) ;
#25159=CARTESIAN_POINT('Ctrl Pts',(-18.9032850203652,4.47374217000043,-320.450262368057)) ;
#25160=CARTESIAN_POINT('Ctrl Pts',(-18.8719982506986,4.60393697273755,-320.451918592634)) ;
#25161=CARTESIAN_POINT('Ctrl Pts',(-18.8087689258819,4.85557435039479,-320.455110716123)) ;
#25162=CARTESIAN_POINT('Ctrl Pts',(-18.7769899514861,4.97705125441319,-320.456647614805)) ;
#25163=CARTESIAN_POINT('Ctrl Pts',(-18.6968582450071,5.27166271158064,-320.460366005653)) ;
#25164=CARTESIAN_POINT('Ctrl Pts',(-18.6472757201289,5.44445078285908,-320.462539193127)) ;
#25165=CARTESIAN_POINT('Ctrl Pts',(-18.3852249421365,6.31205354173321,-320.473423790023)) ;
#25166=CARTESIAN_POINT('Ctrl Pts',(-18.1362902433041,6.99524786991735,-320.481881513887)) ;
#25167=CARTESIAN_POINT('Ctrl Pts',(-17.6870524790589,8.04168730111593,-320.495192208871)) ;
#25168=CARTESIAN_POINT('Ctrl Pts',(-17.512416229709,8.41521457284197,-320.500024121433)) ;
#25169=CARTESIAN_POINT('Ctrl Pts',(-17.271743548073,8.88998957720645,-320.506406327701)) ;
#25170=CARTESIAN_POINT('Ctrl Pts',(-17.2164666140466,8.99657252163222,-320.507855314791)) ;
#25171=CARTESIAN_POINT('Ctrl Pts',(-17.1273110968125,9.16464767802948,-320.510170913391)) ;
#25172=CARTESIAN_POINT('Ctrl Pts',(-17.0940811056974,9.22648056486171,-320.511029439188)) ;
#25173=CARTESIAN_POINT('Ctrl Pts',(-17.0305798548991,9.34312018154654,-320.512662730162)) ;
#25174=CARTESIAN_POINT('Ctrl Pts',(-17.0003773554791,9.39796332623511,-320.513436483261)) ;
#25175=CARTESIAN_POINT('Ctrl Pts',(-16.9134239713994,9.55406660408195,-320.515654344184)) ;
#25176=CARTESIAN_POINT('Ctrl Pts',(-16.8560299035658,9.65496529993548,-320.51710656398)) ;
#25177=CARTESIAN_POINT('Ctrl Pts',(-16.6219016059835,10.0581110375445,-320.522975151342)) ;
#25178=CARTESIAN_POINT('Ctrl Pts',(-16.4379148097202,10.3560690711576,-320.527462080836)) ;
#25179=CARTESIAN_POINT('Ctrl Pts',(-16.183145035555,10.7447465239927,-320.533445816465)) ;
#25180=CARTESIAN_POINT('Ctrl Pts',(-16.1194665204469,10.8400442893461,-320.53492379121)) ;
#25181=CARTESIAN_POINT('Ctrl Pts',(-15.7932932387923,11.3189472579906,-320.542398623993)) ;
#25182=CARTESIAN_POINT('Ctrl Pts',(-15.5179327601823,11.693606908471,-320.548397870096)) ;
#25183=CARTESIAN_POINT('Ctrl Pts',(-15.1399147823498,12.1710470397806,-320.556155319313)) ;
#25184=CARTESIAN_POINT('Ctrl Pts',(-15.0491755006971,12.2830664929547,-320.557984274607)) ;
#25185=CARTESIAN_POINT('Ctrl Pts',(-14.820130974883,12.5594781532492,-320.562516949373)) ;
#25186=CARTESIAN_POINT('Ctrl Pts',(-14.6803295910188,12.7226057442818,-320.565209547733)) ;
#25187=CARTESIAN_POINT('Ctrl Pts',(-14.4497402194546,12.982807156562,-320.569531050511)) ;
#25188=CARTESIAN_POINT('Ctrl Pts',(-14.36061156515,13.0813267525219,-320.571173718456)) ;
#25189=CARTESIAN_POINT('Ctrl Pts',(-14.1849078035738,13.2715833175637,-320.574358881148)) ;
#25190=CARTESIAN_POINT('Ctrl Pts',(-14.0984358871806,13.3634067039217,-320.575902165546)) ;
#25191=CARTESIAN_POINT('Ctrl Pts',(-13.8840386402038,13.5866749438975,-320.57967063276)) ;
#25192=CARTESIAN_POINT('Ctrl Pts',(-13.7551340939057,13.717162650893,-320.581886926964)) ;
#25193=CARTESIAN_POINT('Ctrl Pts',(-13.3626674665425,14.1033534505857,-320.588495604519)) ;
#25194=CARTESIAN_POINT('Ctrl Pts',(-13.0936836223788,14.3534285210378,-320.592840551551)) ;
#25195=CARTESIAN_POINT('Ctrl Pts',(-12.6501488333504,14.742934814927,-320.599772645628)) ;
#25196=CARTESIAN_POINT('Ctrl Pts',(-12.4800008388558,14.8872419066598,-320.6023803057)) ;
#25197=CARTESIAN_POINT('Ctrl Pts',(-12.0045330680007,15.2766181495714,-320.609558733597)) ;
#25198=CARTESIAN_POINT('Ctrl Pts',(-11.6942327495527,15.5154373416621,-320.61412263542)) ;
#25199=CARTESIAN_POINT('Ctrl Pts',(-11.1998693891695,15.8726579323129,-320.621336503789)) ;
#25200=CARTESIAN_POINT('Ctrl Pts',(-11.0206641396424,15.9976031260581,-320.623940760451)) ;
#25201=CARTESIAN_POINT('Ctrl Pts',(-10.767516506604,16.1678296302479,-320.627628782987)) ;
#25202=CARTESIAN_POINT('Ctrl Pts',(-10.6953204971953,16.215679020884,-320.628681631217)) ;
#25203=CARTESIAN_POINT('Ctrl Pts',(-10.5678376678042,16.2989491328382,-320.63054461717)) ;
#25204=CARTESIAN_POINT('Ctrl Pts',(-10.5126869062606,16.3345752869121,-320.631351958675)) ;
#25205=CARTESIAN_POINT('Ctrl Pts',(-10.3844049497662,16.4165237660093,-320.633233095546)) ;
#25206=CARTESIAN_POINT('Ctrl Pts',(-10.3111427893368,16.4626380957567,-320.634309634482)) ;
#25207=CARTESIAN_POINT('Ctrl Pts',(-10.0663560550385,16.6144422445951,-320.637910687091)) ;
#25208=CARTESIAN_POINT('Ctrl Pts',(-9.89349586864448,16.7179530620042,-320.640460125705)) ;
#25209=CARTESIAN_POINT('Ctrl Pts',(-9.46068789989389,16.9680598712658,-320.646831379844)) ;
#25210=CARTESIAN_POINT('Ctrl Pts',(-9.19891270728211,17.111390243241,-320.650673969133)) ;
#25211=CARTESIAN_POINT('Ctrl Pts',(-8.50643326368547,17.4700603984397,-320.660732148367)) ;
#25212=CARTESIAN_POINT('Ctrl Pts',(-8.07084131796425,17.6755180700317,-320.666950914658)) ;
#25213=CARTESIAN_POINT('Ctrl Pts',(-7.49279887847604,17.9223386716356,-320.674961274767)) ;
#25214=CARTESIAN_POINT('Ctrl Pts',(-7.35687912924018,17.9785591200967,-320.676828208443)) ;
#25215=CARTESIAN_POINT('Ctrl Pts',(-7.01813428340084,18.1141893332621,-320.681437243097)) ;
#25216=CARTESIAN_POINT('Ctrl Pts',(-6.81458710223585,18.1917417221992,-320.684168079149)) ;
#25217=CARTESIAN_POINT('Ctrl Pts',(-6.48435098185485,18.3112427076819,-320.688534230011)) ;
#25218=CARTESIAN_POINT('Ctrl Pts',(-6.35845907498211,18.3553375181483,-320.690183854407)) ;
#25219=CARTESIAN_POINT('Ctrl Pts',(-6.11294839453315,18.4385010000557,-320.693372456054)) ;
#25220=CARTESIAN_POINT('Ctrl Pts',(-5.99338437971331,18.4777109223086,-320.694912332072)) ;
#25221=CARTESIAN_POINT('Ctrl Pts',(-5.72816570492207,18.5618418644861,-320.698300422973)) ;
#25222=CARTESIAN_POINT('Ctrl Pts',(-5.58234615835567,18.6062158214463,-320.7001448955)) ;
#25223=CARTESIAN_POINT('Ctrl Pts',(-5.031149864548,18.7668858183006,-320.7070531202)) ;
#25224=CARTESIAN_POINT('Ctrl Pts',(-4.62254402445215,18.8716867317456,-320.712042307311)) ;
#25225=CARTESIAN_POINT('Ctrl Pts',(-3.68041795441686,19.0808904778501,-320.72336645772)) ;
#25226=CARTESIAN_POINT('Ctrl Pts',(-3.14527728659802,19.1763679315871,-320.729666785354)) ;
#25227=CARTESIAN_POINT('Ctrl Pts',(-2.47958132787475,19.2665200110759,-320.737585055342)) ;
#25228=CARTESIAN_POINT('Ctrl Pts',(-2.35215451189201,19.2824916959373,-320.73910479281)) ;
#25229=CARTESIAN_POINT('Ctrl Pts',(-2.06277002532154,19.3158519059493,-320.742572734726)) ;
#25230=CARTESIAN_POINT('Ctrl Pts',(-1.9007332172356,19.3324692712325,-320.744526328699)) ;
#25231=CARTESIAN_POINT('Ctrl Pts',(-1.6605742559612,19.3540497229004,-320.74745006302)) ;
#25232=CARTESIAN_POINT('Ctrl Pts',(-1.58260008586275,19.3605817186337,-320.748403743372)) ;
#25233=CARTESIAN_POINT('Ctrl Pts',(-1.43806326557867,19.3718107409448,-320.750181301689)) ;
#25234=CARTESIAN_POINT('Ctrl Pts',(-1.37151190847322,19.3766362505788,-320.751003749072)) ;
#25235=CARTESIAN_POINT('Ctrl Pts',(-1.20483191954692,19.3878588687708,-320.753072811733)) ;
#25236=CARTESIAN_POINT('Ctrl Pts',(-1.10467614605483,19.3938232961496,-320.754324284472)) ;
#25237=CARTESIAN_POINT('Ctrl Pts',(-0.658880831897908,19.4169065307049,
-320.759924364044)) ;
#25238=CARTESIAN_POINT('Ctrl Pts',(-0.312866875711771,19.4255629692898,
-320.764349425013)) ;
#25239=CARTESIAN_POINT('Ctrl Pts',(0.482373129114524,19.4242041047214,-320.774577596747)) ;
#25240=CARTESIAN_POINT('Ctrl Pts',(0.931392678153338,19.407856583598,-320.780393716816)) ;
#25241=CARTESIAN_POINT('Ctrl Pts',(1.66863256945528,19.3553699574858,-320.789881491135)) ;
#25242=CARTESIAN_POINT('Ctrl Pts',(1.95732760782233,19.3283095464456,-320.793582032926)) ;
#25243=CARTESIAN_POINT('Ctrl Pts',(2.46923212070005,19.268739925995,-320.800097748586)) ;
#25244=CARTESIAN_POINT('Ctrl Pts',(2.69268498215345,19.2387861741158,-320.802926427065)) ;
#25245=CARTESIAN_POINT('Ctrl Pts',(3.04880044857383,19.1847231241589,-320.807406743242)) ;
#25246=CARTESIAN_POINT('Ctrl Pts',(3.18182084892681,19.1631104383089,-320.809074122292)) ;
#25247=CARTESIAN_POINT('Ctrl Pts',(3.43931513789248,19.1185186468174,-320.812290028276)) ;
#25248=CARTESIAN_POINT('Ctrl Pts',(3.56381063411769,19.0957036445271,-320.813839542661)) ;
#25249=CARTESIAN_POINT('Ctrl Pts',(3.86294437716483,19.0378572536076,-320.817550782408)) ;
#25250=CARTESIAN_POINT('Ctrl Pts',(4.03734118130923,19.0016374132105,-320.819704616067)) ;
#25251=CARTESIAN_POINT('Ctrl Pts',(4.92975510516644,18.8034545099332,-320.830686450593)) ;
#25252=CARTESIAN_POINT('Ctrl Pts',(5.63864549327814,18.6031734997548,-320.839252016077)) ;
#25253=CARTESIAN_POINT('Ctrl Pts',(6.71965995391897,18.2302724701753,-320.852619371356)) ;
#25254=CARTESIAN_POINT('Ctrl Pts',(7.10058737682417,18.0853067888293,-320.857397067941)) ;
#25255=CARTESIAN_POINT('Ctrl Pts',(7.58699604262701,17.8824607981219,-320.863716616174)) ;
#25256=CARTESIAN_POINT('Ctrl Pts',(7.6968929435045,17.8354352932725,-320.865159351578)) ;
#25257=CARTESIAN_POINT('Ctrl Pts',(7.87053150959296,17.7592306034609,-320.867467385938)) ;
#25258=CARTESIAN_POINT('Ctrl Pts',(7.93456141983906,17.7307155224725,-320.868324688334)) ;
#25259=CARTESIAN_POINT('Ctrl Pts',(8.05556749265163,17.6760399360573,-320.869957816896)) ;
#25260=CARTESIAN_POINT('Ctrl Pts',(8.11257407251907,17.649948933542,-320.870732650869)) ;
#25261=CARTESIAN_POINT('Ctrl Pts',(8.27520288293987,17.5745619640171,-320.872957649764)) ;
#25262=CARTESIAN_POINT('Ctrl Pts',(8.38050900071584,17.5245907173459,-320.874416005902)) ;
#25263=CARTESIAN_POINT('Ctrl Pts',(8.80617290665142,17.3178848565147,-320.880373255798)) ;
#25264=CARTESIAN_POINT('Ctrl Pts',(9.12263530593281,17.1532895233577,-320.884945401344)) ;
#25265=CARTESIAN_POINT('Ctrl Pts',(9.90441567756516,16.7189205744363,-320.896462937509)) ;
#25266=CARTESIAN_POINT('Ctrl Pts',(10.3634000346301,16.4383605213242,-320.903425238555)) ;
#25267=CARTESIAN_POINT('Ctrl Pts',(10.9399206035668,16.0522010041459,-320.912280742381)) ;
#25268=CARTESIAN_POINT('Ctrl Pts',(11.0686358361182,15.9637188866114,-320.914265845197)) ;
#25269=CARTESIAN_POINT('Ctrl Pts',(11.3816877466164,15.7429124556655,-320.9191101012)) ;
#25270=CARTESIAN_POINT('Ctrl Pts',(11.5647999683402,15.6088920334019,-320.92195758217)) ;
#25271=CARTESIAN_POINT('Ctrl Pts',(11.8530671083957,15.3900505744603,-320.926459818943)) ;
#25272=CARTESIAN_POINT('Ctrl Pts',(11.9597576369989,15.3072876070451,-320.928130596986)) ;
#25273=CARTESIAN_POINT('Ctrl Pts',(12.1646731335807,15.1448783845089,-320.931348517156)) ;
#25274=CARTESIAN_POINT('Ctrl Pts',(12.2630004098689,15.0653720407055,-320.93289669708)) ;
#25275=CARTESIAN_POINT('Ctrl Pts',(12.4973284444706,14.872082802104,-320.936597098772)) ;
#25276=CARTESIAN_POINT('Ctrl Pts',(12.6325612651791,14.7573866632655,-320.938741553452)) ;
#25277=CARTESIAN_POINT('Ctrl Pts',(13.3243672541349,14.1541611685139,-320.949769471832)) ;
#25278=CARTESIAN_POINT('Ctrl Pts',(13.8542418026504,13.6359460795332,-320.958386272018)) ;
#25279=CARTESIAN_POINT('Ctrl Pts',(14.6263055216565,12.7892944932996,-320.971781120459)) ;
#25280=CARTESIAN_POINT('Ctrl Pts',(14.8899398949859,12.4813683265295,-320.976533581835)) ;
#25281=CARTESIAN_POINT('Ctrl Pts',(15.218453677588,12.0724281539511,-320.982823948413)) ;
#25282=CARTESIAN_POINT('Ctrl Pts',(15.2923007197748,11.9787475348052,-320.984263749828)) ;
#25283=CARTESIAN_POINT('Ctrl Pts',(15.4081331432415,11.8289882949567,-320.986568235784)) ;
#25284=CARTESIAN_POINT('Ctrl Pts',(15.4506861856761,11.7733524294485,-320.987424965514)) ;
#25285=CARTESIAN_POINT('Ctrl Pts',(15.5307792179003,11.6674529082228,-320.989058027819)) ;
#25286=CARTESIAN_POINT('Ctrl Pts',(15.5683784395538,11.6172351802214,-320.989833377618)) ;
#25287=CARTESIAN_POINT('Ctrl Pts',(15.6752763756413,11.4730107189607,-320.992061776468)) ;
#25288=CARTESIAN_POINT('Ctrl Pts',(15.7439714073125,11.3785600440571,-320.993523054556)) ;
#25289=CARTESIAN_POINT('Ctrl Pts',(16.1982568333234,10.7419598992156,-321.00336923584)) ;
#25290=CARTESIAN_POINT('Ctrl Pts',(16.5566275747158,10.1809287656804,-321.012016483889)) ;
#25291=CARTESIAN_POINT('Ctrl Pts',(17.0546710893243,9.30515560641771,-321.024988502965)) ;
#25292=CARTESIAN_POINT('Ctrl Pts',(17.2159463323272,9.00327270330376,-321.029374058005)) ;
#25293=CARTESIAN_POINT('Ctrl Pts',(17.4817758696224,8.47239031804388,-321.036902211097)) ;
#25294=CARTESIAN_POINT('Ctrl Pts',(17.590010344414,8.24532726473637,-321.04006581322)) ;
#25295=CARTESIAN_POINT('Ctrl Pts',(17.7513209149935,7.88927471557962,-321.044935165623)) ;
#25296=CARTESIAN_POINT('Ctrl Pts',(17.8074687467393,7.76170771574798,-321.046661943751)) ;
#25297=CARTESIAN_POINT('Ctrl Pts',(17.9113660019189,7.51859170549954,-321.049919341564)) ;
#25298=CARTESIAN_POINT('Ctrl Pts',(17.9593822581987,7.40316433965779,-321.051451770685)) ;
#25299=CARTESIAN_POINT('Ctrl Pts',(18.0676960301773,7.1355298002507,-321.054973261379)) ;
#25300=CARTESIAN_POINT('Ctrl Pts',(18.1271903107961,6.98300772633619,-321.05695667622)) ;
#25301=CARTESIAN_POINT('Ctrl Pts',(18.338879915505,6.41936755279624,-321.064206214334)) ;
#25302=CARTESIAN_POINT('Ctrl Pts',(18.4790742807123,6.00388301523535,-321.06939175138)) ;
#25303=CARTESIAN_POINT('Ctrl Pts',(18.6567789996028,5.4117974458981,-321.076643444932)) ;
#25304=CARTESIAN_POINT('Ctrl Pts',(18.7060726261176,5.238874036943,-321.078745564338)) ;
#25305=CARTESIAN_POINT('Ctrl Pts',(18.8577797882252,4.67721667632012,-321.08554193106)) ;
#25306=CARTESIAN_POINT('Ctrl Pts',(18.9505295115635,4.28598236151558,-321.090226089239)) ;
#25307=CARTESIAN_POINT('Ctrl Pts',(19.0620323075173,3.74077828601382,-321.096805966126)) ;
#25308=CARTESIAN_POINT('Ctrl Pts',(19.0911836958801,3.58903926837595,-321.098643072822)) ;
#25309=CARTESIAN_POINT('Ctrl Pts',(19.1396044020693,3.31969370155706,-321.10192490535)) ;
#25310=CARTESIAN_POINT('Ctrl Pts',(19.1596076150798,3.20222718020609,-321.10336317344)) ;
#25311=CARTESIAN_POINT('Ctrl Pts',(19.1896471867596,3.01545491216939,-321.105665805395)) ;
#25312=CARTESIAN_POINT('Ctrl Pts',(19.2003917668734,2.94626602204398,-321.106522236242)) ;
#25313=CARTESIAN_POINT('Ctrl Pts',(19.2200565493901,2.81495814737294,-321.10815526651)) ;
#25314=CARTESIAN_POINT('Ctrl Pts',(19.2290502633462,2.75285108421927,-321.108930888095)) ;
#25315=CARTESIAN_POINT('Ctrl Pts',(19.2539367053128,2.57492017768091,-321.111161076743)) ;
#25316=CARTESIAN_POINT('Ctrl Pts',(19.2690849759452,2.45899505969869,-321.112623892772)) ;
#25317=CARTESIAN_POINT('Ctrl Pts',(19.3582208492366,1.72537691252049,-321.121928203184)) ;
#25318=CARTESIAN_POINT('Ctrl Pts',(19.403545405867,1.10456562239607,-321.130000011575)) ;
#25319=CARTESIAN_POINT('Ctrl Pts',(19.4202525282254,0.432372943579887,-321.138665586218)) ;
#25320=CARTESIAN_POINT('Ctrl Pts',(19.4213069343574,0.382088451540699,-321.139313465365)) ;
#25321=CARTESIAN_POINT('Ctrl Pts',(19.4279410211256,-0.00624237521102015,
-321.144313284482)) ;
#25322=CARTESIAN_POINT('Ctrl Pts',(19.4248895804184,-0.344378745654854,
-321.148644917905)) ;
#25323=CARTESIAN_POINT('Ctrl Pts',(19.4042491011218,-0.931679827234011,
-321.156094792291)) ;
#25324=CARTESIAN_POINT('Ctrl Pts',(19.3906775309003,-1.18090462179393,-321.159233390272)) ;
#25325=CARTESIAN_POINT('Ctrl Pts',(19.3620736666084,-1.56845761567121,-321.164073822586)) ;
#25326=CARTESIAN_POINT('Ctrl Pts',(19.3503513763003,-1.70700253145772,-321.165796269144)) ;
#25327=CARTESIAN_POINT('Ctrl Pts',(19.3252584801268,-1.96993866947141,-321.169050264869)) ;
#25328=CARTESIAN_POINT('Ctrl Pts',(19.3121716016006,-2.0943499619186,-321.170583566854)) ;
#25329=CARTESIAN_POINT('Ctrl Pts',(19.2791097642132,-2.38192588923135,-321.174113888364)) ;
#25330=CARTESIAN_POINT('Ctrl Pts',(19.2582636068129,-2.54498078475231,-321.176105162949)) ;
#25331=CARTESIAN_POINT('Ctrl Pts',(19.1715556450661,-3.16093759698802,-321.18359390797)) ;
#25332=CARTESIAN_POINT('Ctrl Pts',(19.0917650809629,-3.61172808235323,-321.189002233231)) ;
#25333=CARTESIAN_POINT('Ctrl Pts',(18.8872496816849,-4.56879467090951,-321.200474374697)) ;
#25334=CARTESIAN_POINT('Ctrl Pts',(18.7579163564014,-5.07372229097116,-321.206519474545)) ;
#25335=CARTESIAN_POINT('Ctrl Pts',(18.5723616818639,-5.69331386978618,-321.214146099337)) ;
#25336=CARTESIAN_POINT('Ctrl Pts',(18.5351124996305,-5.8134366637237,-321.215634965401)) ;
#25337=CARTESIAN_POINT('Ctrl Pts',(18.4476431837861,-6.08612199518491,-321.219045306086)) ;
#25338=CARTESIAN_POINT('Ctrl Pts',(18.3966921353373,-6.23844037526806,-321.220972195144)) ;
#25339=CARTESIAN_POINT('Ctrl Pts',(18.3182471264915,-6.46362966199304,-321.223864064886)) ;
#25340=CARTESIAN_POINT('Ctrl Pts',(18.2921943926042,-6.53699552376028,-321.224813090462)) ;
#25341=CARTESIAN_POINT('Ctrl Pts',(18.2429555709759,-6.67305513481332,-321.226587461614)) ;
#25342=CARTESIAN_POINT('Ctrl Pts',(18.2198856220572,-6.73578953642069,-321.227411444905)) ;
#25343=CARTESIAN_POINT('Ctrl Pts',(18.1610926427764,-6.89315383377966,-321.22949230542)) ;
#25344=CARTESIAN_POINT('Ctrl Pts',(18.124953443956,-6.98762608969736,-321.230754165314)) ;
#25345=CARTESIAN_POINT('Ctrl Pts',(17.9542214534666,-7.42370286227686,-321.236630324036)) ;
#25346=CARTESIAN_POINT('Ctrl Pts',(17.8106985502113,-7.76172973170638,-321.241330907462)) ;
#25347=CARTESIAN_POINT('Ctrl Pts',(17.4277487012324,-8.59701101715748,-321.253157920627)) ;
#25348=CARTESIAN_POINT('Ctrl Pts',(17.1765516085091,-9.08851472944457,-321.260305682385)) ;
#25349=CARTESIAN_POINT('Ctrl Pts',(16.826810817791,-9.70639545373984,-321.269369310531)) ;
#25350=CARTESIAN_POINT('Ctrl Pts',(16.7471663224401,-9.84317505923139,-321.271381466083)) ;
#25351=CARTESIAN_POINT('Ctrl Pts',(16.6104204286298,-10.0715542089393,-321.274748298252)) ;
#25352=CARTESIAN_POINT('Ctrl Pts',(16.554211111639,-10.1636787384439,-321.276108433978)) ;
#25353=CARTESIAN_POINT('Ctrl Pts',(16.404548137358,-10.4044340847362,-321.27966750379)) ;
#25354=CARTESIAN_POINT('Ctrl Pts',(16.3098420183649,-10.5522747158843,-321.281857556101)) ;
#25355=CARTESIAN_POINT('Ctrl Pts',(16.1436423911797,-10.8041362103686,-321.285595750241)) ;
#25356=CARTESIAN_POINT('Ctrl Pts',(16.0731153451493,-10.9087814194378,-321.287151133628)) ;
#25357=CARTESIAN_POINT('Ctrl Pts',(15.9246811865839,-11.1244572482492,-321.290361871379)) ;
#25358=CARTESIAN_POINT('Ctrl Pts',(15.8466207061054,-11.2353741468099,-321.292015909578)) ;
#25359=CARTESIAN_POINT('Ctrl Pts',(15.6329138780215,-11.5323740712162,-321.296454331035)) ;
#25360=CARTESIAN_POINT('Ctrl Pts',(15.4951097923419,-11.7168776052897,-321.299221569021)) ;
#25361=CARTESIAN_POINT('Ctrl Pts',(14.869419234496,-12.5242546755011,-321.311401143046)) ;
#25362=CARTESIAN_POINT('Ctrl Pts',(14.3470285630605,-13.1194264797603,-321.32053670096)) ;
#25363=CARTESIAN_POINT('Ctrl Pts',(13.6459709550603,-13.8260553766132,-321.332237181178)) ;
#25364=CARTESIAN_POINT('Ctrl Pts',(13.4998614933809,-13.9687533464353,-321.33465011243)) ;
#25365=CARTESIAN_POINT('Ctrl Pts',(13.2460566205082,-14.2089301301279,-321.338821093324)) ;
#25366=CARTESIAN_POINT('Ctrl Pts',(13.1394680563667,-14.3075536178086,-321.340566821618)) ;
#25367=CARTESIAN_POINT('Ctrl Pts',(12.9761047335796,-14.4553439387318,-321.343241487496)) ;
#25368=CARTESIAN_POINT('Ctrl Pts',(12.9201340552045,-14.5053920464456,-321.344157711655)) ;
#25369=CARTESIAN_POINT('Ctrl Pts',(12.8135854618768,-14.5995601662011,-321.345903041322)) ;
#25370=CARTESIAN_POINT('Ctrl Pts',(12.7630663755014,-14.6437449476966,-321.3467311779)) ;
#25371=CARTESIAN_POINT('Ctrl Pts',(12.6313396693781,-14.7577557001439,-321.348891029275)) ;
#25372=CARTESIAN_POINT('Ctrl Pts',(12.5497817585437,-14.8271734634048,-321.350228730606)) ;
#25373=CARTESIAN_POINT('Ctrl Pts',(11.9865722969862,-15.2985712667869,-321.359456899253)) ;
#25374=CARTESIAN_POINT('Ctrl Pts',(11.4862667574422,-15.6776871254774,-321.36759432973)) ;
#25375=CARTESIAN_POINT('Ctrl Pts',(10.58061777079,-16.2973011699244,-321.38173947329)) ;
#25376=CARTESIAN_POINT('Ctrl Pts',(10.1832354113472,-16.5485109988157,-321.387767673571)) ;
#25377=CARTESIAN_POINT('Ctrl Pts',(9.59434973451866,-16.8915311307317,-321.396369168149)) ;
#25378=CARTESIAN_POINT('Ctrl Pts',(9.40983873194986,-16.9950082679644,-321.399019596404)) ;
#25379=CARTESIAN_POINT('Ctrl Pts',(9.1072776613571,-17.1582519711745,-321.403291850379)) ;
#25380=CARTESIAN_POINT('Ctrl Pts',(8.99024255019759,-17.2198622541645,-321.404926846089)) ;
#25381=CARTESIAN_POINT('Ctrl Pts',(8.76006304022102,-17.3380483411624,-321.408108574698)) ;
#25382=CARTESIAN_POINT('Ctrl Pts',(8.64697706453917,-17.3947236955144,-321.409655973363)) ;
#25383=CARTESIAN_POINT('Ctrl Pts',(8.39370823198772,-17.5185743819712,-321.413087543211)) ;
#25384=CARTESIAN_POINT('Ctrl Pts',(8.25325625181947,-17.5851797712574,-321.414967597029)) ;
#25385=CARTESIAN_POINT('Ctrl Pts',(7.61711711514107,-17.8775506690007,-321.423386416683)) ;
#25386=CARTESIAN_POINT('Ctrl Pts',(7.11286595131701,-18.0840933047186,-321.429790962048)) ;
#25387=CARTESIAN_POINT('Ctrl Pts',(6.10313375195545,-18.4489068358048,-321.442342410594)) ;
#25388=CARTESIAN_POINT('Ctrl Pts',(5.59853202656793,-18.6082466071838,-321.448487168445)) ;
#25389=CARTESIAN_POINT('Ctrl Pts',(4.92326852600235,-18.7915195884469,-321.456808079855)) ;
#25390=CARTESIAN_POINT('Ctrl Pts',(4.75789531272295,-18.834070549204,-321.458854129379)) ;
#25391=CARTESIAN_POINT('Ctrl Pts',(4.51466224231644,-18.8932469997572,-321.461887872693)) ;
#25392=CARTESIAN_POINT('Ctrl Pts',(4.4372267699825,-18.9115831152886,-321.462857304731)) ;
#25393=CARTESIAN_POINT('Ctrl Pts',(4.29498374693055,-18.9443434132671,-321.464646358844)) ;
#25394=CARTESIAN_POINT('Ctrl Pts',(4.23021086537938,-18.9589121192833,-321.465464323057)) ;
#25395=CARTESIAN_POINT('Ctrl Pts',(4.06985379793206,-18.994116906332,-321.467496859649)) ;
#25396=CARTESIAN_POINT('Ctrl Pts',(3.9741861151502,-19.0143638250913,-321.468715899728)) ;
#25397=CARTESIAN_POINT('Ctrl Pts',(3.5781198566014,-19.0950668025527,-321.473783559325)) ;
#25398=CARTESIAN_POINT('Ctrl Pts',(3.27646481875271,-19.1491330235686,-321.477691933158)) ;
#25399=CARTESIAN_POINT('Ctrl Pts',(2.55571883252368,-19.2607837616109,-321.487056220905)) ;
#25400=CARTESIAN_POINT('Ctrl Pts',(2.13577667859977,-19.3118602947752,-321.492531580012)) ;
#25401=CARTESIAN_POINT('Ctrl Pts',(1.38812085748488,-19.3781089649739,-321.502189177703)) ;
#25402=CARTESIAN_POINT('Ctrl Pts',(1.06105900170137,-19.3987664805379,-321.506383987448)) ;
#25403=CARTESIAN_POINT('Ctrl Pts',(0.48925235475261,-19.4203775300337,-321.51363416366)) ;
#25404=CARTESIAN_POINT('Ctrl Pts',(0.244720710913186,-19.4249978991941,
-321.516708288758)) ;
#25405=CARTESIAN_POINT('Ctrl Pts',(0.000166810840218079,-19.4249999992838,
-321.519753599958)) ;
#25406=CARTESIAN_POINT('Origin',(0.,0.,-328.125)) ;
#25407=CARTESIAN_POINT('',(-2.2413097626006E-5,-19.4249999999871,-323.232124485186)) ;
#25408=CARTESIAN_POINT('',(0.00013264926062382,-19.425000134948,-323.017923319024)) ;
#25409=CARTESIAN_POINT('',(-2.37887640734373E-15,-19.425,-328.125)) ;
#25410=CARTESIAN_POINT('Ctrl Pts',(-2.2413097626006E-5,-19.4249999999871,
-323.232124485186)) ;
#25411=CARTESIAN_POINT('Ctrl Pts',(0.0869997778376345,-19.4250001003957,
-323.231049337307)) ;
#25412=CARTESIAN_POINT('Ctrl Pts',(0.174020913669814,-19.4244154237938,
-323.229967325262)) ;
#25413=CARTESIAN_POINT('Ctrl Pts',(0.482637683223412,-19.4202678263039,
-323.226109168543)) ;
#25414=CARTESIAN_POINT('Ctrl Pts',(0.704172780379017,-19.4134974171337,
-323.223301697483)) ;
#25415=CARTESIAN_POINT('Ctrl Pts',(1.32702784953033,-19.3837864970045,-323.215343540241)) ;
#25416=CARTESIAN_POINT('Ctrl Pts',(1.72782138467197,-19.3521785556824,-323.210148410201)) ;
#25417=CARTESIAN_POINT('Ctrl Pts',(2.30672350311634,-19.2883959679957,-323.202636239244)) ;
#25418=CARTESIAN_POINT('Ctrl Pts',(2.48581818589073,-19.2661335075859,-323.200310667552)) ;
#25419=CARTESIAN_POINT('Ctrl Pts',(3.09821215149749,-19.181328219945,-323.192368330831)) ;
#25420=CARTESIAN_POINT('Ctrl Pts',(3.52969452221682,-19.1066357356759,-323.18679188898)) ;
#25421=CARTESIAN_POINT('Ctrl Pts',(4.11855605978414,-18.9840701809965,-323.179253949649)) ;
#25422=CARTESIAN_POINT('Ctrl Pts',(4.27839924596018,-18.948686620764,-323.177214820923)) ;
#25423=CARTESIAN_POINT('Ctrl Pts',(4.55948297852701,-18.8827267148357,-323.17364176892)) ;
#25424=CARTESIAN_POINT('Ctrl Pts',(4.68091130540498,-18.852992404848,-323.17210241951)) ;
#25425=CARTESIAN_POINT('Ctrl Pts',(4.93709217864169,-18.7876334562154,-323.168863237503)) ;
#25426=CARTESIAN_POINT('Ctrl Pts',(5.07176550519992,-18.7517264482508,-323.167165384179)) ;
#25427=CARTESIAN_POINT('Ctrl Pts',(5.44836162425121,-18.6469634004204,-323.16242946667)) ;
#25428=CARTESIAN_POINT('Ctrl Pts',(5.68935053225407,-18.574853412416,-323.159413018638)) ;
#25429=CARTESIAN_POINT('Ctrl Pts',(6.25475661969532,-18.3936335649466,-323.152350630556)) ;
#25430=CARTESIAN_POINT('Ctrl Pts',(6.577825054827,-18.2805895444727,-323.148327468335)) ;
#25431=CARTESIAN_POINT('Ctrl Pts',(7.51962474731159,-17.9228461192883,-323.136537018371)) ;
#25432=CARTESIAN_POINT('Ctrl Pts',(8.12896320634184,-17.6548327693419,-323.128839886506)) ;
#25433=CARTESIAN_POINT('Ctrl Pts',(8.82770544112915,-17.3036378776863,-323.119457046502)) ;
#25434=CARTESIAN_POINT('Ctrl Pts',(8.93158973132352,-17.2502455625886,-323.118046626246)) ;
#25435=CARTESIAN_POINT('Ctrl Pts',(9.0905223962333,-17.1667400313011,-323.115860700008)) ;
#25436=CARTESIAN_POINT('Ctrl Pts',(9.14591704681406,-17.1372915625693,-323.115093507582)) ;
#25437=CARTESIAN_POINT('Ctrl Pts',(9.2628527935397,-17.0743986373128,-323.113461784867)) ;
#25438=CARTESIAN_POINT('Ctrl Pts',(9.32435759757997,-17.0408886525382,-323.112596294773)) ;
#25439=CARTESIAN_POINT('Ctrl Pts',(9.49010526874783,-16.9494174772654,-323.11024568341)) ;
#25440=CARTESIAN_POINT('Ctrl Pts',(9.5939977019496,-16.89082765475,-323.108752698418)) ;
#25441=CARTESIAN_POINT('Ctrl Pts',(10.0483999403069,-16.6290238304381,-323.102147074575)) ;
#25442=CARTESIAN_POINT('Ctrl Pts',(10.393041788145,-16.4158294452402,-323.096939538221)) ;
#25443=CARTESIAN_POINT('Ctrl Pts',(11.3482469054453,-15.782796411105,-323.082165609928)) ;
#25444=CARTESIAN_POINT('Ctrl Pts',(11.9418195589868,-15.3385893937751,-323.072594224182)) ;
#25445=CARTESIAN_POINT('Ctrl Pts',(12.6441997119397,-14.7474155432783,-323.061064896001)) ;
#25446=CARTESIAN_POINT('Ctrl Pts',(12.7782596458076,-14.6314090954591,-323.058852975362)) ;
#25447=CARTESIAN_POINT('Ctrl Pts',(13.0051845529903,-14.4295456279523,-323.055089810607)) ;
#25448=CARTESIAN_POINT('Ctrl Pts',(13.0988333805552,-14.3445870071012,-323.053531063806)) ;
#25449=CARTESIAN_POINT('Ctrl Pts',(13.2907686917593,-14.1670154795538,-323.050323970256)) ;
#25450=CARTESIAN_POINT('Ctrl Pts',(13.3889323875443,-14.0742797185615,-323.048676827952)) ;
#25451=CARTESIAN_POINT('Ctrl Pts',(13.6494765392487,-13.8229494368484,-323.044284645697)) ;
#25452=CARTESIAN_POINT('Ctrl Pts',(13.8100576455257,-13.6625198629165,-323.041556095821)) ;
#25453=CARTESIAN_POINT('Ctrl Pts',(14.0763835575138,-13.3869514261829,-323.036984625653)) ;
#25454=CARTESIAN_POINT('Ctrl Pts',(14.1836168091959,-13.2732835734265,-323.035130724143)) ;
#25455=CARTESIAN_POINT('Ctrl Pts',(14.6540316274703,-12.762430383637,-323.026926743015)) ;
#25456=CARTESIAN_POINT('Ctrl Pts',(15.0019856332515,-12.3515464247775,-323.020672813628)) ;
#25457=CARTESIAN_POINT('Ctrl Pts',(15.5510335136416,-11.6457179741454,-323.01020523527)) ;
#25458=CARTESIAN_POINT('Ctrl Pts',(15.7618710180762,-11.3587328275654,-323.00601743898)) ;
#25459=CARTESIAN_POINT('Ctrl Pts',(16.0310779815112,-10.9703573067439,-323.000347403103)) ;
#25460=CARTESIAN_POINT('Ctrl Pts',(16.0965916171744,-10.87400289397,-322.998940351682)) ;
#25461=CARTESIAN_POINT('Ctrl Pts',(16.196012502994,-10.724911817012,-322.996758427174)) ;
#25462=CARTESIAN_POINT('Ctrl Pts',(16.2305380165881,-10.672590602143,-322.995991819993)) ;
#25463=CARTESIAN_POINT('Ctrl Pts',(16.3031357035559,-10.5614064136519,-322.9943599156)) ;
#25464=CARTESIAN_POINT('Ctrl Pts',(16.3411437029352,-10.5025026378754,-322.993493646817)) ;
#25465=CARTESIAN_POINT('Ctrl Pts',(16.4431219479328,-10.3425656996578,-322.991138362917)) ;
#25466=CARTESIAN_POINT('Ctrl Pts',(16.5064794343286,-10.2411455056021,-322.989641432816)) ;
#25467=CARTESIAN_POINT('Ctrl Pts',(16.7818098915375,-9.79121398340524,-322.982996830855)) ;
#25468=CARTESIAN_POINT('Ctrl Pts',(16.9837109381512,-9.43666129196871,-322.97775306242)) ;
#25469=CARTESIAN_POINT('Ctrl Pts',(17.5177863120818,-8.42604498324527,-322.963015347482)) ;
#25470=CARTESIAN_POINT('Ctrl Pts',(17.824100386648,-7.75709514527957,-322.953517883187)) ;
#25471=CARTESIAN_POINT('Ctrl Pts',(18.1566679898363,-6.90636035587834,-322.942044761967)) ;
#25472=CARTESIAN_POINT('Ctrl Pts',(18.2192858205663,-6.7394384173965,-322.939820097018)) ;
#25473=CARTESIAN_POINT('Ctrl Pts',(18.3224238904226,-6.452552427232,-322.936042346173)) ;
#25474=CARTESIAN_POINT('Ctrl Pts',(18.3640851368324,-6.33301090976489,-322.934481604619)) ;
#25475=CARTESIAN_POINT('Ctrl Pts',(18.4476612368103,-6.08543886559645,-322.931276415262)) ;
#25476=CARTESIAN_POINT('Ctrl Pts',(18.4894187578426,-5.95736228129027,-322.929633108635)) ;
#25477=CARTESIAN_POINT('Ctrl Pts',(18.5973986736284,-5.61409617397655,-322.925266613537)) ;
#25478=CARTESIAN_POINT('Ctrl Pts',(18.6612178094072,-5.39817222670828,-322.922559555595)) ;
#25479=CARTESIAN_POINT('Ctrl Pts',(18.7984514335964,-4.90230374157214,-322.916420747491)) ;
#25480=CARTESIAN_POINT('Ctrl Pts',(18.8693924512028,-4.62172988671266,-322.913003583844)) ;
#25481=CARTESIAN_POINT('Ctrl Pts',(19.0283262012247,-3.92830072628598,-322.904650841262)) ;
#25482=CARTESIAN_POINT('Ctrl Pts',(19.1091814049624,-3.51396221886849,-322.899741097268)) ;
#25483=CARTESIAN_POINT('Ctrl Pts',(19.2362322672417,-2.72735058505679,-322.89040993936)) ;
#25484=CARTESIAN_POINT('Ctrl Pts',(19.2852691634251,-2.35573025466299,-322.885996787262)) ;
#25485=CARTESIAN_POINT('Ctrl Pts',(19.3337443494514,-1.88334166999296,-322.880277645816)) ;
#25486=CARTESIAN_POINT('Ctrl Pts',(19.3431934123166,-1.78368018165155,-322.879064817845)) ;
#25487=CARTESIAN_POINT('Ctrl Pts',(19.3576533883666,-1.61750686075319,-322.877029230405)) ;
#25488=CARTESIAN_POINT('Ctrl Pts',(19.3630928838455,-1.55103421284794,-322.876211348155)) ;
#25489=CARTESIAN_POINT('Ctrl Pts',(19.3741783345324,-1.40640633281511,-322.874423193859)) ;
#25490=CARTESIAN_POINT('Ctrl Pts',(19.3796939314511,-1.32824245298972,-322.873451505502)) ;
#25491=CARTESIAN_POINT('Ctrl Pts',(19.395259761519,-1.08685999870199,-322.870436753541)) ;
#25492=CARTESIAN_POINT('Ctrl Pts',(19.4037220083472,-0.923546399624622,
-322.868377309549)) ;
#25493=CARTESIAN_POINT('Ctrl Pts',(19.4151763502325,-0.631062792373783,
-322.864664816512)) ;
#25494=CARTESIAN_POINT('Ctrl Pts',(19.4189437520683,-0.501932728601272,
-322.863017335223)) ;
#25495=CARTESIAN_POINT('Ctrl Pts',(19.4319767935828,0.177083646483194,-322.854324418943)) ;
#25496=CARTESIAN_POINT('Ctrl Pts',(19.4191746899495,0.727142348784302,-322.847187379231)) ;
#25497=CARTESIAN_POINT('Ctrl Pts',(19.3550134811969,1.70184655988742,-322.834645257377)) ;
#25498=CARTESIAN_POINT('Ctrl Pts',(19.3129441715516,2.12673872818456,-322.829211689476)) ;
#25499=CARTESIAN_POINT('Ctrl Pts',(19.2356352008606,2.71057807836531,-322.821833289147)) ;
#25500=CARTESIAN_POINT('Ctrl Pts',(19.2123488441196,2.87098364563849,-322.819814949636)) ;
#25501=CARTESIAN_POINT('Ctrl Pts',(19.167580379941,3.15437285205711,-322.816265108653)) ;
#25502=CARTESIAN_POINT('Ctrl Pts',(19.1469150626167,3.27747606302304,-322.814728415509)) ;
#25503=CARTESIAN_POINT('Ctrl Pts',(19.100516605888,3.53843974095426,-322.811481671427)) ;
#25504=CARTESIAN_POINT('Ctrl Pts',(19.0744741479358,3.67623808495461,-322.809773743679)) ;
#25505=CARTESIAN_POINT('Ctrl Pts',(18.9965782629021,4.06527284869614,-322.804968073117)) ;
#25506=CARTESIAN_POINT('Ctrl Pts',(18.941237079387,4.31578118990166,-322.801893061239)) ;
#25507=CARTESIAN_POINT('Ctrl Pts',(18.7980024091233,4.9081876643326,-322.794647366709)) ;
#25508=CARTESIAN_POINT('Ctrl Pts',(18.7057190569609,5.24893091513465,-322.790501345458)) ;
#25509=CARTESIAN_POINT('Ctrl Pts',(18.5401987527362,5.8001014298908,-322.783769405367)) ;
#25510=CARTESIAN_POINT('Ctrl Pts',(18.4725363289533,6.01211676226762,-322.781173246079)) ;
#25511=CARTESIAN_POINT('Ctrl Pts',(18.350723583399,6.37231830452902,-322.776729223834)) ;
#25512=CARTESIAN_POINT('Ctrl Pts',(18.2983835519658,6.52109315654854,-322.774883799043)) ;
#25513=CARTESIAN_POINT('Ctrl Pts',(18.1397591947078,6.95502442022907,-322.769456480611)) ;
#25514=CARTESIAN_POINT('Ctrl Pts',(18.0285791309943,7.23833973377031,-322.765856298736)) ;
#25515=CARTESIAN_POINT('Ctrl Pts',(17.873042257305,7.60884324873802,-322.761013632062)) ;
#25516=CARTESIAN_POINT('Ctrl Pts',(17.8346182488141,7.69847562818859,-322.759831463014)) ;
#25517=CARTESIAN_POINT('Ctrl Pts',(17.7689167814171,7.84860655399534,-322.757830693935)) ;
#25518=CARTESIAN_POINT('Ctrl Pts',(17.7420013016323,7.90926154858949,-322.757016572187)) ;
#25519=CARTESIAN_POINT('Ctrl Pts',(17.6820657839034,8.04248286297659,-322.755214997895)) ;
#25520=CARTESIAN_POINT('Ctrl Pts',(17.6489088123999,8.11498605652443,-322.754225897238)) ;
#25521=CARTESIAN_POINT('Ctrl Pts',(17.5429593346683,8.34294110824593,-322.751091263241)) ;
#25522=CARTESIAN_POINT('Ctrl Pts',(17.4685522507388,8.497633238349,-322.74892751584)) ;
#25523=CARTESIAN_POINT('Ctrl Pts',(17.1558907389562,9.12618965355925,-322.740014412872)) ;
#25524=CARTESIAN_POINT('Ctrl Pts',(16.9003271319231,9.59118695496446,-322.733141999619)) ;
#25525=CARTESIAN_POINT('Ctrl Pts',(16.3585805094029,10.4878502518783,-322.719640244599)) ;
#25526=CARTESIAN_POINT('Ctrl Pts',(16.0735284448559,10.9196998698081,-322.713014586628)) ;
#25527=CARTESIAN_POINT('Ctrl Pts',(15.664660186896,11.4883677227629,-322.704210293706)) ;
#25528=CARTESIAN_POINT('Ctrl Pts',(15.5556409618938,11.6355578342765,-322.701923136603)) ;
#25529=CARTESIAN_POINT('Ctrl Pts',(15.3680848490691,11.8814347246312,-322.698089202648)) ;
#25530=CARTESIAN_POINT('Ctrl Pts',(15.2906389954855,11.9809382855656,-322.69653385234)) ;
#25531=CARTESIAN_POINT('Ctrl Pts',(15.1295726469833,12.1837729746726,-322.69335506498)) ;
#25532=CARTESIAN_POINT('Ctrl Pts',(15.0458492040519,12.2870140458884,-322.691732591438)) ;
#25533=CARTESIAN_POINT('Ctrl Pts',(14.8238137630592,12.55513773662,-322.687505534836)) ;
#25534=CARTESIAN_POINT('Ctrl Pts',(14.683809735164,12.7185954391102,-322.684915184268)) ;
#25535=CARTESIAN_POINT('Ctrl Pts',(14.4452889975934,12.9878843306704,-322.680617572545)) ;
#25536=CARTESIAN_POINT('Ctrl Pts',(14.3482549464116,13.0950026215281,-322.678899759297)) ;
#25537=CARTESIAN_POINT('Ctrl Pts',(13.9327305659614,13.5435462271936,-322.671662845646)) ;
#25538=CARTESIAN_POINT('Ctrl Pts',(13.6031803182369,13.8745130010345,-322.666217699342)) ;
#25539=CARTESIAN_POINT('Ctrl Pts',(13.2003545699369,14.2509083301663,-322.659777343217)) ;
#25540=CARTESIAN_POINT('Ctrl Pts',(13.1383082215875,14.3081307681494,-322.658790975433)) ;
#25541=CARTESIAN_POINT('Ctrl Pts',(13.0014293858998,14.4327266141721,-322.656625541003)) ;
#25542=CARTESIAN_POINT('Ctrl Pts',(12.9264419980141,14.4999262362785,-322.655446052979)) ;
#25543=CARTESIAN_POINT('Ctrl Pts',(12.6171521406402,14.7727888438875,-322.650603143933)) ;
#25544=CARTESIAN_POINT('Ctrl Pts',(12.3784377761401,14.9733795716315,-322.646917022754)) ;
#25545=CARTESIAN_POINT('Ctrl Pts',(12.0581948446088,15.2295842633598,-322.641975519103)) ;
#25546=CARTESIAN_POINT('Ctrl Pts',(11.9809240431651,15.290446650764,-322.640783389535)) ;
#25547=CARTESIAN_POINT('Ctrl Pts',(11.8506719919057,15.3914461831979,-322.638771371947)) ;
#25548=CARTESIAN_POINT('Ctrl Pts',(11.7979409598654,15.4319030383557,-322.637956091592)) ;
#25549=CARTESIAN_POINT('Ctrl Pts',(11.6818711338585,15.520012699695,-322.636159177546)) ;
#25550=CARTESIAN_POINT('Ctrl Pts',(11.6184463498184,15.5675499607975,-322.635175973614)) ;
#25551=CARTESIAN_POINT('Ctrl Pts',(11.4189926511198,15.7151438608799,-322.632082387631)) ;
#25552=CARTESIAN_POINT('Ctrl Pts',(11.281949002343,15.8138156776445,-322.629954429962)) ;
#25553=CARTESIAN_POINT('Ctrl Pts',(10.7118192459671,16.2131270586636,-322.621120132497)) ;
#25554=CARTESIAN_POINT('Ctrl Pts',(10.2678688598499,16.4978613562975,-322.614290258458)) ;
#25555=CARTESIAN_POINT('Ctrl Pts',(9.33536068872856,17.0437035113906,-322.600362669254)) ;
#25556=CARTESIAN_POINT('Ctrl Pts',(8.84610710733002,17.3026928852136,-322.593276145969)) ;
#25557=CARTESIAN_POINT('Ctrl Pts',(8.20749016137047,17.6065731344844,-322.584404332839)) ;
#25558=CARTESIAN_POINT('Ctrl Pts',(8.06773385525448,17.6710492845382,-322.582484584167)) ;
#25559=CARTESIAN_POINT('Ctrl Pts',(7.8120588445231,17.7853387757181,-322.579012390081)) ;
#25560=CARTESIAN_POINT('Ctrl Pts',(7.69639287358411,17.8356966654461,-322.57745621456)) ;
#25561=CARTESIAN_POINT('Ctrl Pts',(7.45796239913722,17.9367516803025,-322.574277865685)) ;
#25562=CARTESIAN_POINT('Ctrl Pts',(7.3351518966843,17.987323611267,-322.572656633783)) ;
#25563=CARTESIAN_POINT('Ctrl Pts',(7.01255981392454,18.1163099983745,-322.568437900182)) ;
#25564=CARTESIAN_POINT('Ctrl Pts',(6.81198033543965,18.1926800451154,-322.565854520478)) ;
#25565=CARTESIAN_POINT('Ctrl Pts',(6.47481819673122,18.3146956206919,-322.561570585785)) ;
#25566=CARTESIAN_POINT('Ctrl Pts',(6.33891956713202,18.3621743030175,-322.559859502709)) ;
#25567=CARTESIAN_POINT('Ctrl Pts',(5.76310794750276,18.5561903862949,-322.552667030541)) ;
#25568=CARTESIAN_POINT('Ctrl Pts',(5.31854983005023,18.6884628297979,-322.547258659107)) ;
#25569=CARTESIAN_POINT('Ctrl Pts',(4.71461716494869,18.8448578886458,-322.539971153993)) ;
#25570=CARTESIAN_POINT('Ctrl Pts',(4.55905775957654,18.8830949838841,-322.538098866466)) ;
#25571=CARTESIAN_POINT('Ctrl Pts',(4.17441555221242,18.972611351941,-322.533467813402)) ;
#25572=CARTESIAN_POINT('Ctrl Pts',(3.94484234042544,19.0216704146268,-322.53070254467)) ;
#25573=CARTESIAN_POINT('Ctrl Pts',(3.55850844385497,19.0969337617057,-322.526014091636)) ;
#25574=CARTESIAN_POINT('Ctrl Pts',(3.40221342063259,19.1253968625489,-322.524107755234)) ;
#25575=CARTESIAN_POINT('Ctrl Pts',(3.16912874001578,19.1648966028949,-322.521240436452)) ;
#25576=CARTESIAN_POINT('Ctrl Pts',(3.09259350308339,19.1773956567416,-322.520295025345)) ;
#25577=CARTESIAN_POINT('Ctrl Pts',(2.949860083551,19.1998289335079,-322.518523056933)) ;
#25578=CARTESIAN_POINT('Ctrl Pts',(2.88368155280495,19.2098799125099,-322.517697808486)) ;
#25579=CARTESIAN_POINT('Ctrl Pts',(2.71672680244498,19.2343542694947,-322.515607439356)) ;
#25580=CARTESIAN_POINT('Ctrl Pts',(2.61588671427294,19.2483278582912,-322.514337235252)) ;
#25581=CARTESIAN_POINT('Ctrl Pts',(2.10089796422886,19.3155690424,-322.507819484516)) ;
#25582=CARTESIAN_POINT('Ctrl Pts',(1.68521943037275,19.3562654979736,-322.502459398614)) ;
#25583=CARTESIAN_POINT('Ctrl Pts',(0.489751691572928,19.434502805936,-322.487019752218)) ;
#25584=CARTESIAN_POINT('Ctrl Pts',(-0.291419212319321,19.4384886585489,
-322.476926688712)) ;
#25585=CARTESIAN_POINT('Ctrl Pts',(-1.22337185668507,19.3870411261111,-322.465220392933)) ;
#25586=CARTESIAN_POINT('Ctrl Pts',(-1.37593116208305,19.3768112920489,-322.463313575677)) ;
#25587=CARTESIAN_POINT('Ctrl Pts',(-1.65389300600906,19.3548733181328,-322.459857110122)) ;
#25588=CARTESIAN_POINT('Ctrl Pts',(-1.77933287456766,19.3437446686656,-322.458303854341)) ;
#25589=CARTESIAN_POINT('Ctrl Pts',(-2.03721168180052,19.3183367610048,-322.455123859811)) ;
#25590=CARTESIAN_POINT('Ctrl Pts',(-2.169629875131,19.3039134091911,-322.453498141629)) ;
#25591=CARTESIAN_POINT('Ctrl Pts',(-2.51711581112937,19.2624436450665,-322.449249348791)) ;
#25592=CARTESIAN_POINT('Ctrl Pts',(-2.73189749187674,19.2331573980715,-322.446640796656)) ;
#25593=CARTESIAN_POINT('Ctrl Pts',(-3.09050272956732,19.1781320235074,-322.442307412956)) ;
#25594=CARTESIAN_POINT('Ctrl Pts',(-3.2346069067873,19.1543538979184,-322.440571967631)) ;
#25595=CARTESIAN_POINT('Ctrl Pts',(-3.84667863159392,19.0462538334518,-322.433217279741)) ;
#25596=CARTESIAN_POINT('Ctrl Pts',(-4.31173384204213,18.9463894494896,-322.427674506825)) ;
#25597=CARTESIAN_POINT('Ctrl Pts',(-4.87226877282771,18.8043128681415,-322.420918391098)) ;
#25598=CARTESIAN_POINT('Ctrl Pts',(-4.97168077436332,18.778274034338,-322.419717054076)) ;
#25599=CARTESIAN_POINT('Ctrl Pts',(-5.40511072537198,18.6610632491404,-322.414459404615)) ;
#25600=CARTESIAN_POINT('Ctrl Pts',(-5.73686314199073,18.5617591803445,-322.410384389416)) ;
#25601=CARTESIAN_POINT('Ctrl Pts',(-6.17581623915929,18.4174736120994,-322.404839499393)) ;
#25602=CARTESIAN_POINT('Ctrl Pts',(-6.28552371482691,18.3803218699986,-322.403440602502)) ;
#25603=CARTESIAN_POINT('Ctrl Pts',(-6.45396983264457,18.321594166538,-322.401268358509)) ;
#25604=CARTESIAN_POINT('Ctrl Pts',(-6.51294756114321,18.3007118292949,-322.40050316236)) ;
#25605=CARTESIAN_POINT('Ctrl Pts',(-6.63793235574191,18.2557775603373,-322.398870769856)) ;
#25606=CARTESIAN_POINT('Ctrl Pts',(-6.70391188855861,18.2316517534617,-322.398002573236)) ;
#25607=CARTESIAN_POINT('Ctrl Pts',(-6.88255835819828,18.1652277215225,-322.395635746618)) ;
#25608=CARTESIAN_POINT('Ctrl Pts',(-6.99496539828431,18.1222395619581,-322.394129074699)) ;
#25609=CARTESIAN_POINT('Ctrl Pts',(-7.49299741770808,17.9264515681888,-322.387387202085)) ;
#25610=CARTESIAN_POINT('Ctrl Pts',(-7.8740689591123,17.7623678941348,-322.382052883541)) ;
#25611=CARTESIAN_POINT('Ctrl Pts',(-8.90420875761483,17.2791350405659,-322.367380541591)) ;
#25612=CARTESIAN_POINT('Ctrl Pts',(-9.54117056944496,16.9357466142364,-322.358042458411)) ;
#25613=CARTESIAN_POINT('Ctrl Pts',(-10.3108819180533,16.4635572473466,-322.346697155179)) ;
#25614=CARTESIAN_POINT('Ctrl Pts',(-10.4629454964899,16.3673386609066,-322.344451163442)) ;
#25615=CARTESIAN_POINT('Ctrl Pts',(-10.7188359308319,16.2003998151189,-322.340664497575)) ;
#25616=CARTESIAN_POINT('Ctrl Pts',(-10.823353544009,16.1307599322396,-322.339115753194)) ;
#25617=CARTESIAN_POINT('Ctrl Pts',(-11.0378449485883,15.9848214658981,-322.335932657128)) ;
#25618=CARTESIAN_POINT('Ctrl Pts',(-11.1477203510333,15.9083899071589,-322.334299454614)) ;
#25619=CARTESIAN_POINT('Ctrl Pts',(-11.4363541859676,15.7031515991841,-322.3300005706)) ;
#25620=CARTESIAN_POINT('Ctrl Pts',(-11.6137261738016,15.5724285775482,-322.327350088126)) ;
#25621=CARTESIAN_POINT('Ctrl Pts',(-11.9077179901487,15.3479396202782,-322.322933961974)) ;
#25622=CARTESIAN_POINT('Ctrl Pts',(-12.0255473918856,15.2557926147761,-322.321157568217)) ;
#25623=CARTESIAN_POINT('Ctrl Pts',(-12.5295593962879,14.8521686361351,-322.313521385374)) ;
#25624=CARTESIAN_POINT('Ctrl Pts',(-12.9047947148662,14.5273206550763,-322.307744282539)) ;
#25625=CARTESIAN_POINT('Ctrl Pts',(-13.341653473265,14.1188279630559,-322.300753330409)) ;
#25626=CARTESIAN_POINT('Ctrl Pts',(-13.4155765591881,14.0486058392722,-322.299560518826)) ;
#25627=CARTESIAN_POINT('Ctrl Pts',(-13.7385750969175,13.7369038965997,-322.294298777419)) ;
#25628=CARTESIAN_POINT('Ctrl Pts',(-13.9817081523641,13.4893591561411,-322.290206945558)) ;
#25629=CARTESIAN_POINT('Ctrl Pts',(-14.2864287851527,13.1620150377113,-322.28482103629)) ;
#25630=CARTESIAN_POINT('Ctrl Pts',(-14.3542069338745,13.0880644308583,-322.283605792094)) ;
#25631=CARTESIAN_POINT('Ctrl Pts',(-14.4661094303812,12.9640562662635,-322.281567437303)) ;
#25632=CARTESIAN_POINT('Ctrl Pts',(-14.5105541479562,12.9142903504261,-322.280749235464)) ;
#25633=CARTESIAN_POINT('Ctrl Pts',(-14.606567617893,12.8056601376005,-322.278962027649)) ;
#25634=CARTESIAN_POINT('Ctrl Pts',(-14.6580387321836,12.7467113264984,-322.277991622682)) ;
#25635=CARTESIAN_POINT('Ctrl Pts',(-14.8155764736944,12.5640705249583,-322.27498555188)) ;
#25636=CARTESIAN_POINT('Ctrl Pts',(-14.9204440074153,12.4393538772248,-322.272933634802)) ;
#25637=CARTESIAN_POINT('Ctrl Pts',(-15.1051789891208,12.2139552390321,-322.269237627923)) ;
#25638=CARTESIAN_POINT('Ctrl Pts',(-15.1856400342428,12.1137719797313,-322.267599110672)) ;
#25639=CARTESIAN_POINT('Ctrl Pts',(-15.6014937969851,11.5853314127671,-322.258992659673)) ;
#25640=CARTESIAN_POINT('Ctrl Pts',(-15.9197826657461,11.1439236060407,-322.251934361317)) ;
#25641=CARTESIAN_POINT('Ctrl Pts',(-16.449567940532,10.34010110995,-322.239570016606)) ;
#25642=CARTESIAN_POINT('Ctrl Pts',(-16.668643711703,9.98310045591224,-322.234236073943)) ;
#25643=CARTESIAN_POINT('Ctrl Pts',(-16.9518879398559,9.48617933383256,-322.227061899713)) ;
#25644=CARTESIAN_POINT('Ctrl Pts',(-17.0261878783808,9.35216710152718,-322.225150869763)) ;
#25645=CARTESIAN_POINT('Ctrl Pts',(-17.1586827863538,9.10637722992468,-322.221689284653)) ;
#25646=CARTESIAN_POINT('Ctrl Pts',(-17.2173904885116,8.99488554854081,-322.220135082108)) ;
#25647=CARTESIAN_POINT('Ctrl Pts',(-17.3358608066736,8.76448873391843,-322.216955650361)) ;
#25648=CARTESIAN_POINT('Ctrl Pts',(-17.395494676012,8.64552472141425,-322.215331415742)) ;
#25649=CARTESIAN_POINT('Ctrl Pts',(-17.5487275487607,8.3318342604138,-322.211092559301)) ;
#25650=CARTESIAN_POINT('Ctrl Pts',(-17.6403085221292,8.13614258631874,-322.208492327156)) ;
#25651=CARTESIAN_POINT('Ctrl Pts',(-17.9560938653736,7.43095811739825,-322.199262648058)) ;
#25652=CARTESIAN_POINT('Ctrl Pts',(-18.1616415910947,6.91340879581943,-322.192754902568)) ;
#25653=CARTESIAN_POINT('Ctrl Pts',(-18.3948655766226,6.24362363387668,-322.184471623747)) ;
#25654=CARTESIAN_POINT('Ctrl Pts',(-18.4433507829266,6.09891199690866,-322.182689407968)) ;
#25655=CARTESIAN_POINT('Ctrl Pts',(-18.6006950984343,5.61025058015102,-322.176681020637)) ;
#25656=CARTESIAN_POINT('Ctrl Pts',(-18.7016767652763,5.26384410957424,-322.172439057617)) ;
#25657=CARTESIAN_POINT('Ctrl Pts',(-18.8225206854836,4.80177012775681,-322.166708719203)) ;
#25658=CARTESIAN_POINT('Ctrl Pts',(-18.851067287678,4.68844786379004,-322.165297582483)) ;
#25659=CARTESIAN_POINT('Ctrl Pts',(-18.8933671775832,4.5138939691891,-322.163110804998)) ;
#25660=CARTESIAN_POINT('Ctrl Pts',(-18.9078492453798,4.45284167415197,-322.162343487938)) ;
#25661=CARTESIAN_POINT('Ctrl Pts',(-18.9378675667605,4.32350562990393,-322.160711802385)) ;
#25662=CARTESIAN_POINT('Ctrl Pts',(-18.9533308846873,4.2552059008357,-322.159846476585)) ;
#25663=CARTESIAN_POINT('Ctrl Pts',(-18.9941181061296,4.07041922116845,-322.157496851858)) ;
#25664=CARTESIAN_POINT('Ctrl Pts',(-19.0187395997611,3.95378037315729,-322.156004700023)) ;
#25665=CARTESIAN_POINT('Ctrl Pts',(-19.0584857145935,3.75652413665362,-322.153470173061)) ;
#25666=CARTESIAN_POINT('Ctrl Pts',(-19.0741762133927,3.67602408678508,-322.152432740773)) ;
#25667=CARTESIAN_POINT('Ctrl Pts',(-19.1869287925475,3.07738195450072,-322.14470050552)) ;
#25668=CARTESIAN_POINT('Ctrl Pts',(-19.2633726920502,2.55557985530033,-322.137871018886)) ;
#25669=CARTESIAN_POINT('Ctrl Pts',(-19.3762796102483,1.48179737095789,-322.12395418446)) ;
#25670=CARTESIAN_POINT('Ctrl Pts',(-19.4105879310623,0.930061611787838,
-322.116877906103)) ;
#25671=CARTESIAN_POINT('Ctrl Pts',(-19.4243187996811,0.223860244337423,
-322.108017542089)) ;
#25672=CARTESIAN_POINT('Ctrl Pts',(-19.4254823281291,0.0700760075874453,
-322.106099376195)) ;
#25673=CARTESIAN_POINT('Ctrl Pts',(-19.4242761611515,-0.209827369957383,
-322.102629109354)) ;
#25674=CARTESIAN_POINT('Ctrl Pts',(-19.4225043666603,-0.335940598764716,
-322.10107329333)) ;
#25675=CARTESIAN_POINT('Ctrl Pts',(-19.4163444496347,-0.594848308822051,
-322.097894755938)) ;
#25676=CARTESIAN_POINT('Ctrl Pts',(-19.4118218219957,-0.727633083781163,
-322.096272985603)) ;
#25677=CARTESIAN_POINT('Ctrl Pts',(-19.3964204866916,-1.07501902176696,
-322.092050642375)) ;
#25678=CARTESIAN_POINT('Ctrl Pts',(-19.383342643812,-1.28950446306553,-322.08946423936)) ;
#25679=CARTESIAN_POINT('Ctrl Pts',(-19.3555463204165,-1.64749671126433,
-322.0851743744)) ;
#25680=CARTESIAN_POINT('Ctrl Pts',(-19.3427829286629,-1.79113578601075,
-322.083460373931)) ;
#25681=CARTESIAN_POINT('Ctrl Pts',(-19.2821030922746,-2.39737667679644,
-322.076248671407)) ;
#25682=CARTESIAN_POINT('Ctrl Pts',(-19.219180869292,-2.85832147729128,-322.070824391367)) ;
#25683=CARTESIAN_POINT('Ctrl Pts',(-19.1215975061618,-3.42147194416013,
-322.064147839149)) ;
#25684=CARTESIAN_POINT('Ctrl Pts',(-19.1025564455917,-3.52623009582374,
-322.062903520324)) ;
#25685=CARTESIAN_POINT('Ctrl Pts',(-19.01593727303,-3.98147736549663,-322.057479100484)) ;
#25686=CARTESIAN_POINT('Ctrl Pts',(-18.9395672420655,-4.33022216782846,
-322.053280957858)) ;
#25687=CARTESIAN_POINT('Ctrl Pts',(-18.8255646696006,-4.78981534358015,
-322.047599401192)) ;
#25688=CARTESIAN_POINT('Ctrl Pts',(-18.7964791567579,-4.90271224993069,
-322.046191565082)) ;
#25689=CARTESIAN_POINT('Ctrl Pts',(-18.7501913649732,-5.07591171248897,
-322.044008708593)) ;
#25690=CARTESIAN_POINT('Ctrl Pts',(-18.7337104324694,-5.13640432185019,
-322.043241965212)) ;
#25691=CARTESIAN_POINT('Ctrl Pts',(-18.6981863458054,-5.26434844868946,
-322.041610104164)) ;
#25692=CARTESIAN_POINT('Ctrl Pts',(-18.6790704253005,-5.33177880579128,
-322.040744017672)) ;
#25693=CARTESIAN_POINT('Ctrl Pts',(-18.6263729945161,-5.513903919051,-322.038389827069)) ;
#25694=CARTESIAN_POINT('Ctrl Pts',(-18.5920972888899,-5.62839459316946,
-322.036893819974)) ;
#25695=CARTESIAN_POINT('Ctrl Pts',(-18.4363693228443,-6.13162083053171,
-322.030258358534)) ;
#25696=CARTESIAN_POINT('Ctrl Pts',(-18.3037658065016,-6.51679708026814,
-322.025023089399)) ;
#25697=CARTESIAN_POINT('Ctrl Pts',(-17.8976377207438,-7.58601374652019,
-322.01027662991)) ;
#25698=CARTESIAN_POINT('Ctrl Pts',(-17.597176331973,-8.25908191593055,-322.000761582616)) ;
#25699=CARTESIAN_POINT('Ctrl Pts',(-17.1775331646046,-9.07164117981292,
-321.989275165638)) ;
#25700=CARTESIAN_POINT('Ctrl Pts',(-17.0936710434952,-9.22869057382707,
-321.987053607131)) ;
#25701=CARTESIAN_POINT('Ctrl Pts',(-16.9465216151526,-9.49536971034638,
-321.983279413837)) ;
#25702=CARTESIAN_POINT('Ctrl Pts',(-16.8842999371922,-9.60557423944086,
-321.981719160736)) ;
#25703=CARTESIAN_POINT('Ctrl Pts',(-16.7535935894244,-9.83188153246851,
-321.978513521547)) ;
#25704=CARTESIAN_POINT('Ctrl Pts',(-16.684968377873,-9.94789540133737,-321.976869291936)) ;
#25705=CARTESIAN_POINT('Ctrl Pts',(-16.4982782810744,-10.2561359936287,
-321.972496617361)) ;
#25706=CARTESIAN_POINT('Ctrl Pts',(-16.3780630092293,-10.4470361380337,
-321.969784389133)) ;
#25707=CARTESIAN_POINT('Ctrl Pts',(-16.0956551439354,-10.878636305276,-321.963630698536)) ;
#25708=CARTESIAN_POINT('Ctrl Pts',(-15.9313382249562,-11.1178822212779,
-321.96020393827)) ;
#25709=CARTESIAN_POINT('Ctrl Pts',(-15.5150628733721,-11.6957920631672,
-321.951842159534)) ;
#25710=CARTESIAN_POINT('Ctrl Pts',(-15.2573090139932,-12.030097648066,-321.946932734982)) ;
#25711=CARTESIAN_POINT('Ctrl Pts',(-14.751487024472,-12.6437152653019,-321.937619599178)) ;
#25712=CARTESIAN_POINT('Ctrl Pts',(-14.5058532489479,-12.9247872463635,
-321.933224410298)) ;
#25713=CARTESIAN_POINT('Ctrl Pts',(-14.1842744019425,-13.2720383144944,
-321.927524343496)) ;
#25714=CARTESIAN_POINT('Ctrl Pts',(-14.1157060249559,-13.3449422894551,
-321.926311816486)) ;
#25715=CARTESIAN_POINT('Ctrl Pts',(-14.0005123595303,-13.465538472383,-321.924276573522)) ;
#25716=CARTESIAN_POINT('Ctrl Pts',(-13.9541993190358,-13.5135263367605,
-321.923458730857)) ;
#25717=CARTESIAN_POINT('Ctrl Pts',(-13.8711575136069,-13.5986890923662,
-321.921992373221)) ;
#25718=CARTESIAN_POINT('Ctrl Pts',(-13.8345242301836,-13.6359559663533,
-321.921345616515)) ;
#25719=CARTESIAN_POINT('Ctrl Pts',(-13.7971649502257,-13.6736558756643,
-321.920686384005)) ;
#25720=CARTESIAN_POINT('Ctrl Pts',(-13.7965888289167,-13.6742371763707,
-321.920676217995)) ;
#25721=CARTESIAN_POINT('Ctrl Pts',(-13.795426520587,-13.6754097857558,-321.920655708525)) ;
#25722=CARTESIAN_POINT('Ctrl Pts',(-13.7948403323311,-13.6760010931102,
-321.920645365048)) ;
#25723=CARTESIAN_POINT('Ctrl Pts',(-13.7936573054439,-13.6771942977524,
-321.920624490337)) ;
#25724=CARTESIAN_POINT('Ctrl Pts',(-13.7930604654103,-13.6777961936868,
-321.920613959083)) ;
#25725=CARTESIAN_POINT('Ctrl Pts',(-13.7918555253142,-13.6790111818994,
-321.920592698075)) ;
#25726=CARTESIAN_POINT('Ctrl Pts',(-13.7912474237859,-13.679624272676,-321.920581968299)) ;
#25727=CARTESIAN_POINT('Ctrl Pts',(-13.7900193246764,-13.6808622827647,
-321.920560299035)) ;
#25728=CARTESIAN_POINT('Ctrl Pts',(-13.7893993254175,-13.6814872005603,
-321.920549359522)) ;
#25729=CARTESIAN_POINT('Ctrl Pts',(-13.7881467659951,-13.6827495250698,
-321.920527259068)) ;
#25730=CARTESIAN_POINT('Ctrl Pts',(-13.7875142041195,-13.6833869300559,
-321.920516098101)) ;
#25731=CARTESIAN_POINT('Ctrl Pts',(-13.7862358240191,-13.6846749192253,
-321.920493542483)) ;
#25732=CARTESIAN_POINT('Ctrl Pts',(-13.7855900039887,-13.6853255015095,
-321.920482147804)) ;
#25733=CARTESIAN_POINT('Ctrl Pts',(-13.7842843795546,-13.6866405673725,
-321.920459111935)) ;
#25734=CARTESIAN_POINT('Ctrl Pts',(-13.7836245731173,-13.6873050489948,
-321.920447470712)) ;
#25735=CARTESIAN_POINT('Ctrl Pts',(-13.7822902124971,-13.6886486701486,
-321.920423928303)) ;
#25736=CARTESIAN_POINT('Ctrl Pts',(-13.7816156561877,-13.6893278075067,
-321.920412027083)) ;
#25737=CARTESIAN_POINT('Ctrl Pts',(-13.7802509950926,-13.6907015331921,
-321.920387950571)) ;
#25738=CARTESIAN_POINT('Ctrl Pts',(-13.7795608879517,-13.6913961192396,
-321.920375775243)) ;
#25739=CARTESIAN_POINT('Ctrl Pts',(-13.7781642840296,-13.6928015747971,
-321.920351135693)) ;
#25740=CARTESIAN_POINT('Ctrl Pts',(-13.7774577847946,-13.6935124417614,
-321.920338671434)) ;
#25741=CARTESIAN_POINT('Ctrl Pts',(-13.7760275127563,-13.694951333307,-321.92031343845)) ;
#25742=CARTESIAN_POINT('Ctrl Pts',(-13.7753037372358,-13.6956793552114,
-321.920300669684)) ;
#25743=CARTESIAN_POINT('Ctrl Pts',(-13.7738379827284,-13.697153475549,-321.920274811305)) ;
#25744=CARTESIAN_POINT('Ctrl Pts',(-13.77309600078,-13.6978995711201,-321.920261721648)) ;
#25745=CARTESIAN_POINT('Ctrl Pts',(-13.7715928542687,-13.6994108056173,
-321.920235204237)) ;
#25746=CARTESIAN_POINT('Ctrl Pts',(-13.7708316865645,-13.7001759413929,
-321.920221776437)) ;
#25747=CARTESIAN_POINT('Ctrl Pts',(-13.7692891369936,-13.7017262740489,
-321.920194564574)) ;
#25748=CARTESIAN_POINT('Ctrl Pts',(-13.7685077517204,-13.7025114675343,
-321.920180780459)) ;
#25749=CARTESIAN_POINT('Ctrl Pts',(-13.7669236793154,-13.7041029878782,
-321.920152836808)) ;
#25750=CARTESIAN_POINT('Ctrl Pts',(-13.7661209885129,-13.7049093110496,
-321.920138677218)) ;
#25751=CARTESIAN_POINT('Ctrl Pts',(-13.7644931574563,-13.7065442211285,
-321.920109962406)) ;
#25752=CARTESIAN_POINT('Ctrl Pts',(-13.7636680132028,-13.7073728040697,
-321.920095407126)) ;
#25753=CARTESIAN_POINT('Ctrl Pts',(-13.7619940636091,-13.7090534260987,
-321.920065879599)) ;
#25754=CARTESIAN_POINT('Ctrl Pts',(-13.7611452539216,-13.7099054609035,
-321.920050907287)) ;
#25755=CARTESIAN_POINT('Ctrl Pts',(-13.7594226931801,-13.711634245506,-321.920020523155)) ;
#25756=CARTESIAN_POINT('Ctrl Pts',(-13.7585489375027,-13.712510990569,-321.920005111267)) ;
#25757=CARTESIAN_POINT('Ctrl Pts',(-13.7567751315302,-13.7142905250557,
-321.919973824156)) ;
#25758=CARTESIAN_POINT('Ctrl Pts',(-13.7558750761642,-13.7151933093954,
-321.919957948858)) ;
#25759=CARTESIAN_POINT('Ctrl Pts',(-13.7540472394486,-13.7170263272011,
-321.919925709733)) ;
#25760=CARTESIAN_POINT('Ctrl Pts',(-13.7531194525344,-13.7179565552028,
-321.919909345821)) ;
#25761=CARTESIAN_POINT('Ctrl Pts',(-13.7512346375733,-13.7198459458662,
-321.919876102798)) ;
#25762=CARTESIAN_POINT('Ctrl Pts',(-13.7502776035718,-13.7208051024933,
-321.919859223599)) ;
#25763=CARTESIAN_POINT('Ctrl Pts',(-13.7483326902503,-13.7227539216271,
-321.919824921764)) ;
#25764=CARTESIAN_POINT('Ctrl Pts',(-13.7473448043854,-13.7237435776349,
-321.919807499033)) ;
#25765=CARTESIAN_POINT('Ctrl Pts',(-13.7453364876211,-13.7257550585561,
-321.919772080225)) ;
#25766=CARTESIAN_POINT('Ctrl Pts',(-13.7443160496214,-13.7267768763656,
-321.919754084043)) ;
#25767=CARTESIAN_POINT('Ctrl Pts',(-13.7422408269565,-13.7288544416897,
-321.919717486633)) ;
#25768=CARTESIAN_POINT('Ctrl Pts',(-13.7411860345493,-13.7299101814644,
-321.91969888529)) ;
#25769=CARTESIAN_POINT('Ctrl Pts',(-13.7390401924381,-13.7320574559098,
-321.919661043943)) ;
#25770=CARTESIAN_POINT('Ctrl Pts',(-13.737949134304,-13.7331489821204,-321.919641803815)) ;
#25771=CARTESIAN_POINT('Ctrl Pts',(-13.7357287336744,-13.7353698059295,
-321.919602649239)) ;
#25772=CARTESIAN_POINT('Ctrl Pts',(-13.7345993819667,-13.7364990942964,
-321.919582734656)) ;
#25773=CARTESIAN_POINT('Ctrl Pts',(-13.7323002426266,-13.7387975376917,
-321.919542193329)) ;
#25774=CARTESIAN_POINT('Ctrl Pts',(-13.7311304449302,-13.7399666826247,
-321.919521566438)) ;
#25775=CARTESIAN_POINT('Ctrl Pts',(-13.7287481290465,-13.7423470610551,
-321.919479560317)) ;
#25776=CARTESIAN_POINT('Ctrl Pts',(-13.7275355998298,-13.7435582835266,
-321.919458180928)) ;
#25777=CARTESIAN_POINT('Ctrl Pts',(-13.7250653940659,-13.7460251741028,
-321.919414627141)) ;
#25778=CARTESIAN_POINT('Ctrl Pts',(-13.7238077054677,-13.7472808301059,
-321.919392452569)) ;
#25779=CARTESIAN_POINT('Ctrl Pts',(-13.7212446021085,-13.7498390888763,
-321.919347263082)) ;
#25780=CARTESIAN_POINT('Ctrl Pts',(-13.7199391741447,-13.7511416783716,
-321.919324247977)) ;
#25781=CARTESIAN_POINT('Ctrl Pts',(-13.717277850786,-13.7537964588403,-321.919277329243)) ;
#25782=CARTESIAN_POINT('Ctrl Pts',(-13.7159219408863,-13.7551486352706,
-321.919253425406)) ;
#25783=CARTESIAN_POINT('Ctrl Pts',(-13.7131567386621,-13.7579054081601,
-321.919204677983)) ;
#25784=CARTESIAN_POINT('Ctrl Pts',(-13.7117474304253,-13.7593099886303,
-321.91917983417)) ;
#25785=CARTESIAN_POINT('Ctrl Pts',(-13.7088723308401,-13.7621745627954,
-321.91912915232)) ;
#25786=CARTESIAN_POINT('Ctrl Pts',(-13.7074065220258,-13.7636345388873,
-321.919103314035)) ;
#25787=CARTESIAN_POINT('Ctrl Pts',(-13.70441512222,-13.76661308352,-321.919050585294)) ;
#25788=CARTESIAN_POINT('Ctrl Pts',(-13.7028895119838,-13.7681316327177,
-321.919023694564)) ;
#25789=CARTESIAN_POINT('Ctrl Pts',(-13.6997749979669,-13.771230701275,-321.918968799274)) ;
#25790=CARTESIAN_POINT('Ctrl Pts',(-13.6981860730402,-13.7728111992804,
-321.918940794414)) ;
#25791=CARTESIAN_POINT('Ctrl Pts',(-13.6949411915582,-13.7760377544292,
-321.918883605238)) ;
#25792=CARTESIAN_POINT('Ctrl Pts',(-13.6932852116582,-13.7776837880639,
-321.918854420593)) ;
#25793=CARTESIAN_POINT('Ctrl Pts',(-13.6899022395683,-13.7810452287258,
-321.918794801983)) ;
#25794=CARTESIAN_POINT('Ctrl Pts',(-13.6881752216315,-13.7827606097994,
-321.918764367658)) ;
#25795=CARTESIAN_POINT('Ctrl Pts',(-13.684645933437,-13.7862647995924,-321.918702175293)) ;
#25796=CARTESIAN_POINT('Ctrl Pts',(-13.6828436347763,-13.7880535796128,
-321.918670416859)) ;
#25797=CARTESIAN_POINT('Ctrl Pts',(-13.6804789199589,-13.7903996369732,
-321.91862874977)) ;
#25798=CARTESIAN_POINT('Ctrl Pts',(-13.6799168203588,-13.7909572334532,
-321.918618845509)) ;
#25799=CARTESIAN_POINT('Ctrl Pts',(-13.6787263080345,-13.7921380638829,
-321.918597868814)) ;
#25800=CARTESIAN_POINT('Ctrl Pts',(-13.6780978868282,-13.7927612892295,
-321.918586796262)) ;
#25801=CARTESIAN_POINT('Ctrl Pts',(-13.6767665319042,-13.7940814558863,
-321.918563338617)) ;
#25802=CARTESIAN_POINT('Ctrl Pts',(-13.6760635875719,-13.7947783863508,
-321.918550953377)) ;
#25803=CARTESIAN_POINT('Ctrl Pts',(-13.6745738944745,-13.7962551089636,
-321.91852470677)) ;
#25804=CARTESIAN_POINT('Ctrl Pts',(-13.6737871322104,-13.7970348876143,
-321.918510845216)) ;
#25805=CARTESIAN_POINT('Ctrl Pts',(-13.6721192576387,-13.7986876746815,
-321.918481460347)) ;
#25806=CARTESIAN_POINT('Ctrl Pts',(-13.6712381284496,-13.7995606659679,
-321.9184659368)) ;
#25807=CARTESIAN_POINT('Ctrl Pts',(-13.669369535232,-13.8014116466694,-321.918433017009)) ;
#25808=CARTESIAN_POINT('Ctrl Pts',(-13.6683820498343,-13.8023896145311,
-321.91841562047)) ;
#25809=CARTESIAN_POINT('Ctrl Pts',(-13.6662871039958,-13.8044639236585,
-321.918378714664)) ;
#25810=CARTESIAN_POINT('Ctrl Pts',(-13.6651796165536,-13.8055602376637,
-321.918359205026)) ;
#25811=CARTESIAN_POINT('Ctrl Pts',(-13.6628291206958,-13.8078864594264,
-321.918317799503)) ;
#25812=CARTESIAN_POINT('Ctrl Pts',(-13.6615860781113,-13.8091163326297,
-321.918295903151)) ;
#25813=CARTESIAN_POINT('Ctrl Pts',(-13.6589467303143,-13.8117270127501,
-321.918249412119)) ;
#25814=CARTESIAN_POINT('Ctrl Pts',(-13.6575503817547,-13.8131077758095,
-321.918224816848)) ;
#25815=CARTESIAN_POINT('Ctrl Pts',(-13.6545841492008,-13.8160400109437,
-321.918172571458)) ;
#25816=CARTESIAN_POINT('Ctrl Pts',(-13.6530142101109,-13.8175914272391,
-321.918144920593)) ;
#25817=CARTESIAN_POINT('Ctrl Pts',(-13.649677605723,-13.8208875411423,-321.918086156294)) ;
#25818=CARTESIAN_POINT('Ctrl Pts',(-13.6479108702678,-13.8226321676554,
-321.918055041915)) ;
#25819=CARTESIAN_POINT('Ctrl Pts',(-13.6441541200476,-13.8263404834621,
-321.917988883907)) ;
#25820=CARTESIAN_POINT('Ctrl Pts',(-13.6421640157737,-13.8283040819532,
-321.917953839078)) ;
#25821=CARTESIAN_POINT('Ctrl Pts',(-13.6379301046876,-13.8324797989296,
-321.917879285671)) ;
#25822=CARTESIAN_POINT('Ctrl Pts',(-13.635686183427,-13.8346918012378,-321.917839775566)) ;
#25823=CARTESIAN_POINT('Ctrl Pts',(-13.6309097684997,-13.83939798248,-321.917755679256)) ;
#25824=CARTESIAN_POINT('Ctrl Pts',(-13.6283771282392,-13.841892012472,-321.917711091107)) ;
#25825=CARTESIAN_POINT('Ctrl Pts',(-13.6229833098943,-13.8472006863084,
-321.917616137236)) ;
#25826=CARTESIAN_POINT('Ctrl Pts',(-13.620121943785,-13.8500151387998,-321.917565769039)) ;
#25827=CARTESIAN_POINT('Ctrl Pts',(-13.6140248907664,-13.8560085107072,
-321.917458451974)) ;
#25828=CARTESIAN_POINT('Ctrl Pts',(-13.6107889622523,-13.8591871839666,
-321.917401499953)) ;
#25829=CARTESIAN_POINT('Ctrl Pts',(-13.6038903909734,-13.8659589482889,
-321.917280096852)) ;
#25830=CARTESIAN_POINT('Ctrl Pts',(-13.6002274374487,-13.8695517222049,
-321.917215641754)) ;
#25831=CARTESIAN_POINT('Ctrl Pts',(-13.5924149577786,-13.8772084494627,
-321.917078184163)) ;
#25832=CARTESIAN_POINT('Ctrl Pts',(-13.5882650315659,-13.8812719938123,
-321.917005176554)) ;
#25833=CARTESIAN_POINT('Ctrl Pts',(-13.5794103844198,-13.8899345533679,
-321.916849420367)) ;
#25834=CARTESIAN_POINT('Ctrl Pts',(-13.5747051482798,-13.8945330408254,
-321.916766665283)) ;
#25835=CARTESIAN_POINT('Ctrl Pts',(-13.4660251496906,-14.0006394956279,
-321.914855492211)) ;
#25836=CARTESIAN_POINT('Ctrl Pts',(-13.360917067357,-14.1009799181697,-321.913013011225)) ;
#25837=CARTESIAN_POINT('Ctrl Pts',(-12.9934555293007,-14.4439760356215,
-321.906606112049)) ;
#25838=CARTESIAN_POINT('Ctrl Pts',(-12.7255388078101,-14.6805651119825,
-321.901995665326)) ;
#25839=CARTESIAN_POINT('Ctrl Pts',(-11.9679977559987,-15.3131987308327,
-321.889261891804)) ;
#25840=CARTESIAN_POINT('Ctrl Pts',(-11.465409817794,-15.6930369365424,-321.881155919804)) ;
#25841=CARTESIAN_POINT('Ctrl Pts',(-10.7901467633406,-16.1535944146192,
-321.870873886645)) ;
#25842=CARTESIAN_POINT('Ctrl Pts',(-10.6335025923433,-16.257136970012,-321.868527818771)) ;
#25843=CARTESIAN_POINT('Ctrl Pts',(-10.3696157153385,-16.426121533064,-321.864641237735)) ;
#25844=CARTESIAN_POINT('Ctrl Pts',(-10.2631951885802,-16.4928233869235,
-321.863091264631)) ;
#25845=CARTESIAN_POINT('Ctrl Pts',(-10.0642590600527,-16.6148406963404,
-321.860225666613)) ;
#25846=CARTESIAN_POINT('Ctrl Pts',(-9.97191543731357,-16.67042723909,-321.858908027175)) ;
#25847=CARTESIAN_POINT('Ctrl Pts',(-9.73799206223305,-16.8085989687794,
-321.855600934164)) ;
#25848=CARTESIAN_POINT('Ctrl Pts',(-9.59582074590066,-16.8901661628774,
-321.85361907834)) ;
#25849=CARTESIAN_POINT('Ctrl Pts',(-9.27499232951797,-17.0688748920229,
-321.849205477607)) ;
#25850=CARTESIAN_POINT('Ctrl Pts',(-9.09580766392284,-17.1650300288908,
-321.846780560478)) ;
#25851=CARTESIAN_POINT('Ctrl Pts',(-8.71562730490277,-17.3614197574898,
-321.841708755823)) ;
#25852=CARTESIAN_POINT('Ctrl Pts',(-8.51433595414785,-17.4610176884455,
-321.839065541142)) ;
#25853=CARTESIAN_POINT('Ctrl Pts',(-7.92989044423887,-17.7376885444461,
-321.831484049055)) ;
#25854=CARTESIAN_POINT('Ctrl Pts',(-7.54263405977385,-17.9057931541581,
-321.82657566955)) ;
#25855=CARTESIAN_POINT('Ctrl Pts',(-6.83548122026538,-18.1857471782768,
-321.817656725286)) ;
#25856=CARTESIAN_POINT('Ctrl Pts',(-6.51754975639907,-18.302096823207,-321.813661608518)) ;
#25857=CARTESIAN_POINT('Ctrl Pts',(-6.10252592606983,-18.4417917957282,
-321.808386735216)) ;
#25858=CARTESIAN_POINT('Ctrl Pts',(-6.00806810705088,-18.4727806487798,
-321.807182168297)) ;
#25859=CARTESIAN_POINT('Ctrl Pts',(-5.84993811696017,-18.523317319709,-321.805156017952)) ;
#25860=CARTESIAN_POINT('Ctrl Pts',(-5.78639575683629,-18.5432652101179,
-321.804339204036)) ;
#25861=CARTESIAN_POINT('Ctrl Pts',(-5.66352047137734,-18.5811464308203,
-321.802753922913)) ;
#25862=CARTESIAN_POINT('Ctrl Pts',(-5.60420196725724,-18.5991232888309,
-321.801986167679)) ;
#25863=CARTESIAN_POINT('Ctrl Pts',(-5.44976255011084,-18.6451212430377,
-321.79998185025)) ;
#25864=CARTESIAN_POINT('Ctrl Pts',(-5.35451135023511,-18.6726984173206,
-321.798740356006)) ;
#25865=CARTESIAN_POINT('Ctrl Pts',(-5.23329529387914,-18.7067891771549,
-321.797155511464)) ;
#25866=CARTESIAN_POINT('Ctrl Pts',(-5.20752237901617,-18.7139801117475,
-321.796818259972)) ;
#25867=CARTESIAN_POINT('Ctrl Pts',(-4.88067279530254,-18.8044473503303,
-321.792538034086)) ;
#25868=CARTESIAN_POINT('Ctrl Pts',(-4.5776449616963,-18.8805024603371,-321.788535774688)) ;
#25869=CARTESIAN_POINT('Ctrl Pts',(-3.82995213981358,-19.0491019582444,
-321.778670535125)) ;
#25870=CARTESIAN_POINT('Ctrl Pts',(-3.38362170254857,-19.1334242537664,
-321.772792219302)) ;
#25871=CARTESIAN_POINT('Ctrl Pts',(-2.54134139382648,-19.2621544093536,
-321.761866201931)) ;
#25872=CARTESIAN_POINT('Ctrl Pts',(-2.14617973628184,-19.3101766546514,
-321.756807599584)) ;
#25873=CARTESIAN_POINT('Ctrl Pts',(-1.59033795421999,-19.3604517857785,
-321.749818056103)) ;
#25874=CARTESIAN_POINT('Ctrl Pts',(-1.43068176917797,-19.3729042203815,
-321.74782460285)) ;
#25875=CARTESIAN_POINT('Ctrl Pts',(-1.15143259223858,-19.3912134571859,
-321.744362943065)) ;
#25876=CARTESIAN_POINT('Ctrl Pts',(-1.03190551029623,-19.397941319024,-321.742889227387)) ;
#25877=CARTESIAN_POINT('Ctrl Pts',(-0.796102252058334,-19.4090284021025,
-321.739997183021)) ;
#25878=CARTESIAN_POINT('Ctrl Pts',(-0.679833882419814,-19.4134486436397,
-321.738578519148)) ;
#25879=CARTESIAN_POINT('Ctrl Pts',(-0.375642228969848,-19.4222771708154,
-321.73488496426)) ;
#25880=CARTESIAN_POINT('Ctrl Pts',(-0.187682302120229,-19.4250027819016,
-321.732620827941)) ;
#25881=CARTESIAN_POINT('Ctrl Pts',(0.000287704542308483,-19.4249999978694,
-321.730371769961)) ;
#25882=CARTESIAN_POINT('Ctrl Pts',(0.000166810840220334,-19.4249999992838,
-321.519753599958)) ;
#25883=CARTESIAN_POINT('Ctrl Pts',(-0.137993919525454,-19.4250011857295,
-321.521474048577)) ;
#25884=CARTESIAN_POINT('Ctrl Pts',(-0.276150831818518,-19.4235283656108,
-321.523185239571)) ;
#25885=CARTESIAN_POINT('Ctrl Pts',(-0.53957842532853,-19.4179089211439,
-321.526430631963)) ;
#25886=CARTESIAN_POINT('Ctrl Pts',(-0.664847763116804,-19.4140235202933,
-321.527966437048)) ;
#25887=CARTESIAN_POINT('Ctrl Pts',(-0.959143785326477,-19.4020437386808,
-321.531557767981)) ;
#25888=CARTESIAN_POINT('Ctrl Pts',(-1.12811975032796,-19.3929524306718,
-321.533606773427)) ;
#25889=CARTESIAN_POINT('Ctrl Pts',(-1.82385781940178,-19.346395966334,-321.541996772373)) ;
#25890=CARTESIAN_POINT('Ctrl Pts',(-2.34910384164736,-19.2896658081241,
-321.548214171527)) ;
#25891=CARTESIAN_POINT('Ctrl Pts',(-3.4541968831645,-19.1244975507954,-321.561283593549)) ;
#25892=CARTESIAN_POINT('Ctrl Pts',(-4.03274157583352,-19.0109146101146,
-321.568117561937)) ;
#25893=CARTESIAN_POINT('Ctrl Pts',(-4.74844141749848,-18.8362592300831,
-321.5769081418)) ;
#25894=CARTESIAN_POINT('Ctrl Pts',(-4.89125599936391,-18.7996801120878,
-321.578679877863)) ;
#25895=CARTESIAN_POINT('Ctrl Pts',(-5.10655323721792,-18.7419166053703,
-321.581385834935)) ;
#25896=CARTESIAN_POINT('Ctrl Pts',(-5.1793516369488,-18.7219294040292,-321.582306896747)) ;
#25897=CARTESIAN_POINT('Ctrl Pts',(-5.31724060076121,-18.6832054254666,
-321.584064563423)) ;
#25898=CARTESIAN_POINT('Ctrl Pts',(-5.38235319448009,-18.6645516053336,
-321.584900229818)) ;
#25899=CARTESIAN_POINT('Ctrl Pts',(-5.54987476571115,-18.6156095752097,
-321.587063843937)) ;
#25900=CARTESIAN_POINT('Ctrl Pts',(-5.65213392953952,-18.5848166998563,
-321.588397649147)) ;
#25901=CARTESIAN_POINT('Ctrl Pts',(-5.88117861791001,-18.5137801639357,
-321.591410553692)) ;
#25902=CARTESIAN_POINT('Ctrl Pts',(-6.00781521955603,-18.4730743005298,
-321.593093934034)) ;
#25903=CARTESIAN_POINT('Ctrl Pts',(-6.42275009447146,-18.3349803013719,
-321.59865700866)) ;
#25904=CARTESIAN_POINT('Ctrl Pts',(-6.70917858998817,-18.2321184654356,
-321.602572211709)) ;
#25905=CARTESIAN_POINT('Ctrl Pts',(-7.67103749769757,-17.8609598394091,
-321.615865964881)) ;
#25906=CARTESIAN_POINT('Ctrl Pts',(-8.33379196344689,-17.5615096785485,
-321.625252196394)) ;
#25907=CARTESIAN_POINT('Ctrl Pts',(-9.13759232078629,-17.1425592042303,
-321.636640143357)) ;
#25908=CARTESIAN_POINT('Ctrl Pts',(-9.29581612929397,-17.0572779809668,
-321.638883515212)) ;
#25909=CARTESIAN_POINT('Ctrl Pts',(-9.56252306762809,-16.9087120347454,
-321.642667179836)) ;
#25910=CARTESIAN_POINT('Ctrl Pts',(-9.67161745506976,-16.8465487843646,
-321.644215511052)) ;
#25911=CARTESIAN_POINT('Ctrl Pts',(-9.89579471499568,-16.7159146321512,
-321.647398929157)) ;
#25912=CARTESIAN_POINT('Ctrl Pts',(-10.0107877640252,-16.6473025872586,
-321.649032854664)) ;
#25913=CARTESIAN_POINT('Ctrl Pts',(-10.3133823722953,-16.462486543861,-321.653336574777)) ;
#25914=CARTESIAN_POINT('Ctrl Pts',(-10.4997290232265,-16.3442653500482,
-321.655991104438)) ;
#25915=CARTESIAN_POINT('Ctrl Pts',(-11.0107845513228,-16.0076960674286,
-321.663296403465)) ;
#25916=CARTESIAN_POINT('Ctrl Pts',(-11.330971816777,-15.7826736711742,-321.667900800916)) ;
#25917=CARTESIAN_POINT('Ctrl Pts',(-12.1840755435748,-15.1437762679862,
-321.680375958236)) ;
#25918=CARTESIAN_POINT('Ctrl Pts',(-12.702574619797,-14.7115684999939,-321.688178121742)) ;
#25919=CARTESIAN_POINT('Ctrl Pts',(-13.2815616675023,-14.1754667738344,
-321.697649881584)) ;
#25920=CARTESIAN_POINT('Ctrl Pts',(-13.3648980395466,-14.0969230302277,
-321.699033277616)) ;
#25921=CARTESIAN_POINT('Ctrl Pts',(-13.4925199781998,-13.9744916075537,
-321.701187145043)) ;
#25922=CARTESIAN_POINT('Ctrl Pts',(-13.5372970155398,-13.9311198600096,
-321.70194968251)) ;
#25923=CARTESIAN_POINT('Ctrl Pts',(-13.6323036452477,-13.8382043555132,
-321.703583200554)) ;
#25924=CARTESIAN_POINT('Ctrl Pts',(-13.6824736613103,-13.7886009786697,
-321.704455236815)) ;
#25925=CARTESIAN_POINT('Ctrl Pts',(-13.8185575841274,-13.6525799847649,
-321.706844956081)) ;
#25926=CARTESIAN_POINT('Ctrl Pts',(-13.9039302876838,-13.565625545279,-321.708370934074)) ;
#25927=CARTESIAN_POINT('Ctrl Pts',(-14.2859818476908,-13.169100072345,-321.715310012587)) ;
#25928=CARTESIAN_POINT('Ctrl Pts',(-14.5731792235212,-12.8505610933593,
-321.72082848209)) ;
#25929=CARTESIAN_POINT('Ctrl Pts',(-15.3020610583068,-11.9862480059601,
-321.73541065802)) ;
#25930=CARTESIAN_POINT('Ctrl Pts',(-15.7251142087192,-11.4255855040086,
-321.74446844012)) ;
#25931=CARTESIAN_POINT('Ctrl Pts',(-16.2184492557989,-10.6923162048437,
-321.755575729801)) ;
#25932=CARTESIAN_POINT('Ctrl Pts',(-16.3178770547089,-10.5399530671514,
-321.757847133281)) ;
#25933=CARTESIAN_POINT('Ctrl Pts',(-16.4824639559744,-10.2798276497053,
-321.761662955554)) ;
#25934=CARTESIAN_POINT('Ctrl Pts',(-16.5487420876878,-10.172787716823,-321.763215754428)) ;
#25935=CARTESIAN_POINT('Ctrl Pts',(-16.6830241611637,-9.95113501770478,
-321.766396031634)) ;
#25936=CARTESIAN_POINT('Ctrl Pts',(-16.7508986650605,-9.83645145731254,
-321.768022476734)) ;
#25937=CARTESIAN_POINT('Ctrl Pts',(-16.9262338974671,-9.53311930498286,
-321.772276136057)) ;
#25938=CARTESIAN_POINT('Ctrl Pts',(-17.031721455623,-9.34335176009869,-321.774888762541)) ;
#25939=CARTESIAN_POINT('Ctrl Pts',(-17.2029754883793,-9.02273179961395,
-321.779230165537)) ;
#25940=CARTESIAN_POINT('Ctrl Pts',(-17.2704831731612,-8.89283227116158,
-321.780969569412)) ;
#25941=CARTESIAN_POINT('Ctrl Pts',(-17.5518823967115,-8.33606659766567,
-321.788350972823)) ;
#25942=CARTESIAN_POINT('Ctrl Pts',(-17.7514653072975,-7.9021555119831,-321.793915925178)) ;
#25943=CARTESIAN_POINT('Ctrl Pts',(-18.0129624793137,-7.27359294896615,
-321.801870197743)) ;
#25944=CARTESIAN_POINT('Ctrl Pts',(-18.0881141909734,-7.08463807105786,
-321.804248659626)) ;
#25945=CARTESIAN_POINT('Ctrl Pts',(-18.2612309716059,-6.62864667907774,
-321.809985652093)) ;
#25946=CARTESIAN_POINT('Ctrl Pts',(-18.3563246673777,-6.36057053072341,
-321.81335592492)) ;
#25947=CARTESIAN_POINT('Ctrl Pts',(-18.4753554835077,-6.00007776171063,
-321.817933958195)) ;
#25948=CARTESIAN_POINT('Ctrl Pts',(-18.5045478651989,-5.90943327729716,
-321.819088963623)) ;
#25949=CARTESIAN_POINT('Ctrl Pts',(-18.5528726745015,-5.7555112692649,-321.821059410071)) ;
#25950=CARTESIAN_POINT('Ctrl Pts',(-18.5723507722436,-5.69234409038847,
-321.821870724917)) ;
#25951=CARTESIAN_POINT('Ctrl Pts',(-18.6150049985991,-5.5514673381143,-321.82368666578)) ;
#25952=CARTESIAN_POINT('Ctrl Pts',(-18.6380176541675,-5.4737097661826,-321.824693166421)) ;
#25953=CARTESIAN_POINT('Ctrl Pts',(-18.7105700238134,-5.22279906336804,
-321.82795180155)) ;
#25954=CARTESIAN_POINT('Ctrl Pts',(-18.7581887316726,-5.04910051344394,
-321.830224146284)) ;
#25955=CARTESIAN_POINT('Ctrl Pts',(-18.8743149182203,-4.60116809336992,
-321.836105119959)) ;
#25956=CARTESIAN_POINT('Ctrl Pts',(-18.9392648631523,-4.32605566155452,
-321.839736903673)) ;
#25957=CARTESIAN_POINT('Ctrl Pts',(-19.1617721700492,-3.28219698126016,
-321.853490887193)) ;
#25958=CARTESIAN_POINT('Ctrl Pts',(-19.2787063760172,-2.50555798944725,
-321.863640031432)) ;
#25959=CARTESIAN_POINT('Ctrl Pts',(-19.3619035059237,-1.57183035006413,
-321.875396848927)) ;
#25960=CARTESIAN_POINT('Ctrl Pts',(-19.3736651547587,-1.41952688539306,
-321.877301810919)) ;
#25961=CARTESIAN_POINT('Ctrl Pts',(-19.3918416028456,-1.14147036985379,
-321.88075602338)) ;
#25962=CARTESIAN_POINT('Ctrl Pts',(-19.3988324445314,-1.01576335473321,
-321.88230886377)) ;
#25963=CARTESIAN_POINT('Ctrl Pts',(-19.4107060822563,-0.756882535287205,
-321.885489115068)) ;
#25964=CARTESIAN_POINT('Ctrl Pts',(-19.4154415234315,-0.623708498257451,
-321.887115493897)) ;
#25965=CARTESIAN_POINT('Ctrl Pts',(-19.4242874661633,-0.273496505423218,
-321.891368709497)) ;
#25966=CARTESIAN_POINT('Ctrl Pts',(-19.426130878585,-0.0564199848549467,
-321.893980964478)) ;
#25967=CARTESIAN_POINT('Ctrl Pts',(-19.4231253852299,0.306995018624896,
-321.898321636079)) ;
#25968=CARTESIAN_POINT('Ctrl Pts',(-19.4202610138816,0.453329770050739,
-321.900060678823)) ;
#25969=CARTESIAN_POINT('Ctrl Pts',(-19.4010106240392,1.07666074869678,-321.907439640759)) ;
#25970=CARTESIAN_POINT('Ctrl Pts',(-19.368701749369,1.55299853504544,-321.913002565655)) ;
#25971=CARTESIAN_POINT('Ctrl Pts',(-19.3064972400198,2.14566234795309,-321.91996522085)) ;
#25972=CARTESIAN_POINT('Ctrl Pts',(-19.2930312948164,2.26354722416188,-321.921352459695)) ;
#25973=CARTESIAN_POINT('Ctrl Pts',(-19.2345354755949,2.73711638167395,-321.926943506424)) ;
#25974=CARTESIAN_POINT('Ctrl Pts',(-19.18074258187,3.09164582336676,-321.931169354635)) ;
#25975=CARTESIAN_POINT('Ctrl Pts',(-19.0993957261344,3.54312782823735,-321.936694207466)) ;
#25976=CARTESIAN_POINT('Ctrl Pts',(-19.0808587260183,3.6416345435994,-321.93790854326)) ;
#25977=CARTESIAN_POINT('Ctrl Pts',(-19.0487157364733,3.8054571728456,-321.939945857371)) ;
#25978=CARTESIAN_POINT('Ctrl Pts',(-19.0355341776143,3.87085443867606,-321.940763938792)) ;
#25979=CARTESIAN_POINT('Ctrl Pts',(-19.0061507414482,4.01285298058675,-321.942551501063)) ;
#25980=CARTESIAN_POINT('Ctrl Pts',(-18.9898221312005,4.089426665838,-321.943522387402)) ;
#25981=CARTESIAN_POINT('Ctrl Pts',(-18.9380397034528,4.32526279607029,-321.946531711417)) ;
#25982=CARTESIAN_POINT('Ctrl Pts',(-18.9010419519967,4.48417874869191,-321.948586448672)) ;
#25983=CARTESIAN_POINT('Ctrl Pts',(-18.831275264322,4.76762764335202,-321.952288629498)) ;
#25984=CARTESIAN_POINT('Ctrl Pts',(-18.7992617566922,4.89233674040736,-321.953930502264)) ;
#25985=CARTESIAN_POINT('Ctrl Pts',(-18.6249503843949,5.54438235124987,-321.962569197615)) ;
#25986=CARTESIAN_POINT('Ctrl Pts',(-18.4616973416045,6.06586223043786,-321.969656847603)) ;
#25987=CARTESIAN_POINT('Ctrl Pts',(-18.1386381233472,6.96322698490873,-321.98190487759)) ;
#25988=CARTESIAN_POINT('Ctrl Pts',(-17.9885556775987,7.3422468648902,-321.987096612051)) ;
#25989=CARTESIAN_POINT('Ctrl Pts',(-17.7645531369485,7.85975337840269,-321.994173851226)) ;
#25990=CARTESIAN_POINT('Ctrl Pts',(-17.7007141651313,8.0024864548459,-321.996124914457)) ;
#25991=CARTESIAN_POINT('Ctrl Pts',(-17.5820381049605,8.25945598079471,-321.999635349625)) ;
#25992=CARTESIAN_POINT('Ctrl Pts',(-17.5277931988091,8.37395621271068,-322.001198750424)) ;
#25993=CARTESIAN_POINT('Ctrl Pts',(-17.414777989142,8.60659873425551,-322.004374064247)) ;
#25994=CARTESIAN_POINT('Ctrl Pts',(-17.3559162529916,8.72468940752645,-322.005985219887)) ;
#25995=CARTESIAN_POINT('Ctrl Pts',(-17.2003629633093,9.02896164959694,-322.010136253277)) ;
#25996=CARTESIAN_POINT('Ctrl Pts',(-17.1018502710109,9.21419296780131,-322.012662896466)) ;
#25997=CARTESIAN_POINT('Ctrl Pts',(-16.9329772955244,9.51967968871202,-322.016835976153)) ;
#25998=CARTESIAN_POINT('Ctrl Pts',(-16.8642891225149,9.64083885914976,-322.018492737576)) ;
#25999=CARTESIAN_POINT('Ctrl Pts',(-16.5740093021148,10.1402675240861,-322.025336187019)) ;
#26000=CARTESIAN_POINT('Ctrl Pts',(-16.3409469725165,10.5117202349637,-322.030456974303)) ;
#26001=CARTESIAN_POINT('Ctrl Pts',(-16.0100360596828,11.0014855310064,-322.037360339665)) ;
#26002=CARTESIAN_POINT('Ctrl Pts',(-15.9230660812538,11.1269899378105,-322.03914365802)) ;
#26003=CARTESIAN_POINT('Ctrl Pts',(-15.6303717899033,11.5389103634005,-322.045059472361)) ;
#26004=CARTESIAN_POINT('Ctrl Pts',(-15.4183288133193,11.8207491411684,-322.049208084551)) ;
#26005=CARTESIAN_POINT('Ctrl Pts',(-15.1263313986596,12.1876265316248,-322.054834489446)) ;
#26006=CARTESIAN_POINT('Ctrl Pts',(-15.0531150864741,12.2779423435435,-322.056238562421)) ;
#26007=CARTESIAN_POINT('Ctrl Pts',(-14.9392095913001,12.415899715649,-322.058416950197)) ;
#26008=CARTESIAN_POINT('Ctrl Pts',(-14.8990933033547,12.4640108989375,-322.059183041143)) ;
#26009=CARTESIAN_POINT('Ctrl Pts',(-14.8135567080289,12.5655912905736,-322.060815116098)) ;
#26010=CARTESIAN_POINT('Ctrl Pts',(-14.7680780506843,12.6190101627988,-322.061682082124)) ;
#26011=CARTESIAN_POINT('Ctrl Pts',(-14.6441203401758,12.76302198776,-322.064041544328)) ;
#26012=CARTESIAN_POINT('Ctrl Pts',(-14.565090606265,12.853136829778,-322.065542001388)) ;
#26013=CARTESIAN_POINT('Ctrl Pts',(-14.2117989258282,13.2485400587148,-322.072221649667)) ;
#26014=CARTESIAN_POINT('Ctrl Pts',(-13.9287368160246,13.5458234214669,-322.077498021253)) ;
#26015=CARTESIAN_POINT('Ctrl Pts',(-13.1165490400812,14.3464192405241,-322.092202639988)) ;
#26016=CARTESIAN_POINT('Ctrl Pts',(-12.5681446078452,14.8292060812908,-322.101633139377)) ;
#26017=CARTESIAN_POINT('Ctrl Pts',(-11.8529139010312,15.3906194530765,-322.113055541061)) ;
#26018=CARTESIAN_POINT('Ctrl Pts',(-11.7104338918001,15.4993055746845,-322.115291985747)) ;
#26019=CARTESIAN_POINT('Ctrl Pts',(-11.4656620440075,15.680719482441,-322.11906771863)) ;
#26020=CARTESIAN_POINT('Ctrl Pts',(-11.3641320675004,15.75445562357,-322.120614961322)) ;
#26021=CARTESIAN_POINT('Ctrl Pts',(-11.1526571158441,15.9049312733297,-322.123799258323)) ;
#26022=CARTESIAN_POINT('Ctrl Pts',(-11.0426176480786,15.9815266820436,-322.125435118724)) ;
#26023=CARTESIAN_POINT('Ctrl Pts',(-10.7486246860528,16.1816808284978,-322.129751783756)) ;
#26024=CARTESIAN_POINT('Ctrl Pts',(-10.5633347891934,16.3032415623709,-322.132417146455)) ;
#26025=CARTESIAN_POINT('Ctrl Pts',(-10.1370283418555,16.5726036544938,-322.13843654961)) ;
#26026=CARTESIAN_POINT('Ctrl Pts',(-9.89478328088476,16.7183671346557,-322.14177691235)) ;
#26027=CARTESIAN_POINT('Ctrl Pts',(-9.32727839399568,17.0431891181357,-322.149458386695)) ;
#26028=CARTESIAN_POINT('Ctrl Pts',(-8.99989390334472,17.2183137186226,-322.153783072134)) ;
#26029=CARTESIAN_POINT('Ctrl Pts',(-8.30784773249189,17.563370164023,-322.162823789283)) ;
#26030=CARTESIAN_POINT('Ctrl Pts',(-7.94251862548703,17.7315735880065,-322.167540085576)) ;
#26031=CARTESIAN_POINT('Ctrl Pts',(-7.46279669768633,17.9346428207089,-322.173787619969)) ;
#26032=CARTESIAN_POINT('Ctrl Pts',(-7.35293636587208,17.9799631366386,-322.175222148817)) ;
#26033=CARTESIAN_POINT('Ctrl Pts',(-7.18412166801338,18.0477977016755,-322.177436751616)) ;
#26034=CARTESIAN_POINT('Ctrl Pts',(-7.12546187302847,18.0710375769158,-322.178208168271)) ;
#26035=CARTESIAN_POINT('Ctrl Pts',(-7.00183167015459,18.1193219106397,-322.17983891258)) ;
#26036=CARTESIAN_POINT('Ctrl Pts',(-6.93683777270874,18.1443036494965,-322.180699117302)) ;
#26037=CARTESIAN_POINT('Ctrl Pts',(-6.76212671099227,18.2103814857112,-322.18301783578)) ;
#26038=CARTESIAN_POINT('Ctrl Pts',(-6.65216974764954,18.250835298664,-322.184483865171)) ;
#26039=CARTESIAN_POINT('Ctrl Pts',(-6.46647331192613,18.317252987594,-322.186966981986)) ;
#26040=CARTESIAN_POINT('Ctrl Pts',(-6.39092702273029,18.3437478689615,-322.187979194431)) ;
#26041=CARTESIAN_POINT('Ctrl Pts',(-6.19050273883427,18.4126503612684,-322.190668040386)) ;
#26042=CARTESIAN_POINT('Ctrl Pts',(-6.06535299929608,18.4542545346315,-322.192350529913)) ;
#26043=CARTESIAN_POINT('Ctrl Pts',(-5.39307697334305,18.6701652400179,-322.201391544757)) ;
#26044=CARTESIAN_POINT('Ctrl Pts',(-4.83884768270826,18.8214214061858,-322.20884663313)) ;
#26045=CARTESIAN_POINT('Ctrl Pts',(-4.00110471714039,19.0105968930812,-322.219861174234)) ;
#26046=CARTESIAN_POINT('Ctrl Pts',(-3.72213119814023,19.0671805195667,-322.223489568204)) ;
#26047=CARTESIAN_POINT('Ctrl Pts',(-3.23009299049653,19.1557691316164,-322.229802649641)) ;
#26048=CARTESIAN_POINT('Ctrl Pts',(-3.01755101323832,19.1903980642888,-322.232501748979)) ;
#26049=CARTESIAN_POINT('Ctrl Pts',(-2.67292870491131,19.24067957461,-322.236830843358)) ;
#26050=CARTESIAN_POINT('Ctrl Pts',(-2.54118668679324,19.2585219742975,-322.238474694233)) ;
#26051=CARTESIAN_POINT('Ctrl Pts',(-2.2827284418658,19.2908278533652,-322.241678298675)) ;
#26052=CARTESIAN_POINT('Ctrl Pts',(-2.15603229868407,19.3053985502647,-322.24323867526)) ;
#26053=CARTESIAN_POINT('Ctrl Pts',(-1.84594096685738,19.3379699557666,-322.247034308825)) ;
#26054=CARTESIAN_POINT('Ctrl Pts',(-1.66241537467799,19.3546106994087,-322.249260695636)) ;
#26055=CARTESIAN_POINT('Ctrl Pts',(-1.26196896667993,19.3851824084985,-322.254080335228)) ;
#26056=CARTESIAN_POINT('Ctrl Pts',(-1.04499468819214,19.3980887969072,-322.256667314832)) ;
#26057=CARTESIAN_POINT('Ctrl Pts',(-0.341764790536675,19.4280861127892,
-322.264993508244)) ;
#26058=CARTESIAN_POINT('Ctrl Pts',(0.144927519837056,19.4305514446397,-322.270661568477)) ;
#26059=CARTESIAN_POINT('Ctrl Pts',(0.753617700200657,19.4107621670884,-322.277778530952)) ;
#26060=CARTESIAN_POINT('Ctrl Pts',(0.875997487490465,19.405624337621,-322.279211151562)) ;
#26061=CARTESIAN_POINT('Ctrl Pts',(1.33998658650594,19.3817467183513,-322.284658631148)) ;
#26062=CARTESIAN_POINT('Ctrl Pts',(1.6811279580789,19.35514085907,-322.288695501083)) ;
#26063=CARTESIAN_POINT('Ctrl Pts',(2.12046180633606,19.3091737247416,-322.294016213876)) ;
#26064=CARTESIAN_POINT('Ctrl Pts',(2.21945497267446,19.2980456987227,-322.295223215219)) ;
#26065=CARTESIAN_POINT('Ctrl Pts',(2.38450901996773,19.2782048157456,-322.297252142653)) ;
#26066=CARTESIAN_POINT('Ctrl Pts',(2.45061858922249,19.2699126288385,-322.298069267512)) ;
#26067=CARTESIAN_POINT('Ctrl Pts',(2.59462631556501,19.2510965389534,-322.299859768106)) ;
#26068=CARTESIAN_POINT('Ctrl Pts',(2.67250573269195,19.2404396196522,-322.300834602459)) ;
#26069=CARTESIAN_POINT('Ctrl Pts',(2.91362721410149,19.205952641226,-322.30387072156)) ;
#26070=CARTESIAN_POINT('Ctrl Pts',(3.07663180624033,19.1805155556675,-322.305948706644)) ;
#26071=CARTESIAN_POINT('Ctrl Pts',(3.36835222313166,19.1311777265822,-322.309701919699)) ;
#26072=CARTESIAN_POINT('Ctrl Pts',(3.49718814234211,19.108046288207,-322.31137159351)) ;
#26073=CARTESIAN_POINT('Ctrl Pts',(4.18102974980211,18.9781201975067,-322.320283188385)) ;
#26074=CARTESIAN_POINT('Ctrl Pts',(4.73141064502779,18.8484431840874,-322.327619836129)) ;
#26075=CARTESIAN_POINT('Ctrl Pts',(5.59989972668357,18.6033724321149,-322.339198251705)) ;
#26076=CARTESIAN_POINT('Ctrl Pts',(5.92200733024302,18.5033557152875,-322.343494847032)) ;
#26077=CARTESIAN_POINT('Ctrl Pts',(6.42546501764056,18.3325346259777,-322.350189287347)) ;
#26078=CARTESIAN_POINT('Ctrl Pts',(6.60863371843887,18.2673037707899,-322.352620635035)) ;
#26079=CARTESIAN_POINT('Ctrl Pts',(6.89979450310611,18.1586617486847,-322.35647739956)) ;
#26080=CARTESIAN_POINT('Ctrl Pts',(7.00842901518905,18.1170108866149,-322.357914608821)) ;
#26081=CARTESIAN_POINT('Ctrl Pts',(7.23591754646221,18.0274386223259,-322.360920717728)) ;
#26082=CARTESIAN_POINT('Ctrl Pts',(7.3546848296242,17.9793119203311,-322.362488109231)) ;
#26083=CARTESIAN_POINT('Ctrl Pts',(7.646525336519,17.8576770672284,-322.366335649204)) ;
#26084=CARTESIAN_POINT('Ctrl Pts',(7.81902408683818,17.7828243661498,-322.368606316912)) ;
#26085=CARTESIAN_POINT('Ctrl Pts',(8.45803550430294,17.4944411709327,-322.377014616087)) ;
#26086=CARTESIAN_POINT('Ctrl Pts',(8.91711818994298,17.2649599188393,-322.383043225155)) ;
#26087=CARTESIAN_POINT('Ctrl Pts',(9.91905429851975,16.7134881588428,-322.39641287395)) ;
#26088=CARTESIAN_POINT('Ctrl Pts',(10.4563932133784,16.3826786531704,-322.403726392021)) ;
#26089=CARTESIAN_POINT('Ctrl Pts',(11.065599604178,15.9654234142734,-322.412603058772)) ;
#26090=CARTESIAN_POINT('Ctrl Pts',(11.154005389719,15.9037858107882,-322.413906645861)) ;
#26091=CARTESIAN_POINT('Ctrl Pts',(11.2967194220409,15.8025085018902,-322.416039819654)) ;
#26092=CARTESIAN_POINT('Ctrl Pts',(11.3513429377013,15.7633168518619,-322.416863249034)) ;
#26093=CARTESIAN_POINT('Ctrl Pts',(11.466345344481,15.6798963976054,-322.418612675989)) ;
#26094=CARTESIAN_POINT('Ctrl Pts',(11.5266742085929,15.6356006686421,-322.419539568829)) ;
#26095=CARTESIAN_POINT('Ctrl Pts',(11.7022667328295,15.5051054183458,-322.422262384819)) ;
#26096=CARTESIAN_POINT('Ctrl Pts',(11.8168300768498,15.4179722256755,-322.424070610583)) ;
#26097=CARTESIAN_POINT('Ctrl Pts',(12.0149512620729,15.2637821733769,-322.427246038466)) ;
#26098=CARTESIAN_POINT('Ctrl Pts',(12.0989425021021,15.1972922050473,-322.428607722149)) ;
#26099=CARTESIAN_POINT('Ctrl Pts',(12.4858361754489,14.8857752884396,-322.434944918395)) ;
#26100=CARTESIAN_POINT('Ctrl Pts',(12.7818733456633,14.6323656460322,-322.439978125299)) ;
#26101=CARTESIAN_POINT('Ctrl Pts',(13.2283466654119,14.226286705167,-322.447763732511)) ;
#26102=CARTESIAN_POINT('Ctrl Pts',(13.3842156105213,14.0797429482958,-322.450521116386)) ;
#26103=CARTESIAN_POINT('Ctrl Pts',(13.8405425313196,13.6362902740204,-322.458690877162)) ;
#26104=CARTESIAN_POINT('Ctrl Pts',(14.1337717066096,13.3321239459225,-322.464067745774)) ;
#26105=CARTESIAN_POINT('Ctrl Pts',(14.5263715320709,12.89735859959,-322.471408681557)) ;
#26106=CARTESIAN_POINT('Ctrl Pts',(14.6343561248546,12.7746995913693,-322.473444060024)) ;
#26107=CARTESIAN_POINT('Ctrl Pts',(14.8221730074186,12.5558524902735,-322.477012914539)) ;
#26108=CARTESIAN_POINT('Ctrl Pts',(14.9026486345367,12.4602290565838,-322.478551774362)) ;
#26109=CARTESIAN_POINT('Ctrl Pts',(15.0710021850157,12.2562223100951,-322.481792261368)) ;
#26110=CARTESIAN_POINT('Ctrl Pts',(15.1586465097661,12.1476552565352,-322.483491883823)) ;
#26111=CARTESIAN_POINT('Ctrl Pts',(15.4015300358421,11.8400676341461,-322.488240004634)) ;
#26112=CARTESIAN_POINT('Ctrl Pts',(15.5540710314681,11.6389520019424,-322.49126669368)) ;
#26113=CARTESIAN_POINT('Ctrl Pts',(15.9051959723939,11.1567805860924,-322.498360920711)) ;
#26114=CARTESIAN_POINT('Ctrl Pts',(16.1003165449625,10.873307664811,-322.502405360083)) ;
#26115=CARTESIAN_POINT('Ctrl Pts',(16.607514919402,10.0928350404621,-322.513297769457)) ;
#26116=CARTESIAN_POINT('Ctrl Pts',(16.9047702995967,9.58663698366048,-322.520099352405)) ;
#26117=CARTESIAN_POINT('Ctrl Pts',(17.2543284449089,8.92440767078751,-322.529015093809)) ;
#26118=CARTESIAN_POINT('Ctrl Pts',(17.328202007139,8.78010919164021,-322.530959551231)) ;
#26119=CARTESIAN_POINT('Ctrl Pts',(17.4349837030527,8.56493256596178,-322.533872388238)) ;
#26120=CARTESIAN_POINT('Ctrl Pts',(17.4692843499664,8.4947531373728,-322.534824481347)) ;
#26121=CARTESIAN_POINT('Ctrl Pts',(17.5321155740631,8.36420982414766,-322.536600941388)) ;
#26122=CARTESIAN_POINT('Ctrl Pts',(17.5607599820299,8.30390217316753,-322.537423900966)) ;
#26123=CARTESIAN_POINT('Ctrl Pts',(17.6317875276063,8.1523502884539,-322.539496931454)) ;
#26124=CARTESIAN_POINT('Ctrl Pts',(17.6737737663007,8.06092224635881,-322.540751901965)) ;
#26125=CARTESIAN_POINT('Ctrl Pts',(17.8737773937493,7.6163247774033,-322.54686824153)) ;
#26126=CARTESIAN_POINT('Ctrl Pts',(18.0219293393609,7.25881418096625,-322.55182632041)) ;
#26127=CARTESIAN_POINT('Ctrl Pts',(18.4495936129414,6.13282434307509,-322.567337205528)) ;
#26128=CARTESIAN_POINT('Ctrl Pts',(18.691342319068,5.35096005747389,-322.577926246698)) ;
#26129=CARTESIAN_POINT('Ctrl Pts',(18.9186342108558,4.40895083119452,-322.590076449937)) ;
#26130=CARTESIAN_POINT('Ctrl Pts',(18.9524383080937,4.26129676235897,-322.591964995753)) ;
#26131=CARTESIAN_POINT('Ctrl Pts',(19.0111131611252,3.99048654752953,-322.595399308466)) ;
#26132=CARTESIAN_POINT('Ctrl Pts',(19.0365226431029,3.86745552245288,-322.596948510254)) ;
#26133=CARTESIAN_POINT('Ctrl Pts',(19.0865217833814,3.6129221452482,-322.60013125896)) ;
#26134=CARTESIAN_POINT('Ctrl Pts',(19.1109500252098,3.48139475013887,-322.601763670123)) ;
#26135=CARTESIAN_POINT('Ctrl Pts',(19.1719449121388,3.1329745247032,-322.606057258534)) ;
#26136=CARTESIAN_POINT('Ctrl Pts',(19.2061897498079,2.91569487581688,-322.608703308823)) ;
#26137=CARTESIAN_POINT('Ctrl Pts',(19.2755731146343,2.42096961665071,-322.614667768628)) ;
#26138=CARTESIAN_POINT('Ctrl Pts',(19.3084251679495,2.14325235131007,-322.617972907592)) ;
#26139=CARTESIAN_POINT('Ctrl Pts',(19.3712810694384,1.49157069937497,-322.625665929551)) ;
#26140=CARTESIAN_POINT('Ctrl Pts',(19.3964702207311,1.11725397078053,-322.630035863361)) ;
#26141=CARTESIAN_POINT('Ctrl Pts',(19.4238456911595,0.401536211112973,-322.638409144621)) ;
#26142=CARTESIAN_POINT('Ctrl Pts',(19.4279018549825,0.0603451208772657,
-322.642408773378)) ;
#26143=CARTESIAN_POINT('Ctrl Pts',(19.4207056058857,-0.437465243863178,
-322.648341074187)) ;
#26144=CARTESIAN_POINT('Ctrl Pts',(19.4165445020235,-0.594122496938241,
-322.650222095652)) ;
#26145=CARTESIAN_POINT('Ctrl Pts',(19.4075059715968,-0.827823698301524,
-322.653059142511)) ;
#26146=CARTESIAN_POINT('Ctrl Pts',(19.4040641485014,-0.904916910112894,
-322.654000063747)) ;
#26147=CARTESIAN_POINT('Ctrl Pts',(19.3967727894313,-1.0489651345334,-322.65576914048)) ;
#26148=CARTESIAN_POINT('Ctrl Pts',(19.393035730014,-1.11592456502311,-322.656596053999)) ;
#26149=CARTESIAN_POINT('Ctrl Pts',(19.3827016065989,-1.28531678165452,-322.658698684292)) ;
#26150=CARTESIAN_POINT('Ctrl Pts',(19.3756392530886,-1.38771909676743,-322.659979614227)) ;
#26151=CARTESIAN_POINT('Ctrl Pts',(19.3334879781438,-1.93560021469249,-322.66687697107)) ;
#26152=CARTESIAN_POINT('Ctrl Pts',(19.2838466744928,-2.37982390098811,-322.67262216572)) ;
#26153=CARTESIAN_POINT('Ctrl Pts',(19.1135824941099,-3.53941527140412,-322.687734748529)) ;
#26154=CARTESIAN_POINT('Ctrl Pts',(18.9681395997243,-4.25043342405456,-322.697100920326)) ;
#26155=CARTESIAN_POINT('Ctrl Pts',(18.7374211684101,-5.12562614107244,-322.708472414391)) ;
#26156=CARTESIAN_POINT('Ctrl Pts',(18.6891432179249,-5.29895473644626,-322.710718129449)) ;
#26157=CARTESIAN_POINT('Ctrl Pts',(18.6030893080468,-5.59208952525797,-322.714504478491)) ;
#26158=CARTESIAN_POINT('Ctrl Pts',(18.5665465005512,-5.71224545628891,-322.716053179363)) ;
#26159=CARTESIAN_POINT('Ctrl Pts',(18.4886555040694,-5.95971121910292,-322.719236309663)) ;
#26160=CARTESIAN_POINT('Ctrl Pts',(18.4471514274265,-6.08696512510024,-322.720869588631)) ;
#26161=CARTESIAN_POINT('Ctrl Pts',(18.3338456394452,-6.42256080602345,-322.72516898316)) ;
#26162=CARTESIAN_POINT('Ctrl Pts',(18.2598082240209,-6.63012723024059,-322.727819892744)) ;
#26163=CARTESIAN_POINT('Ctrl Pts',(18.1296007348864,-6.97643077307825,-322.732236864083)) ;
#26164=CARTESIAN_POINT('Ctrl Pts',(18.075329986854,-7.11585940440395,-322.734013677263)) ;
#26165=CARTESIAN_POINT('Ctrl Pts',(17.8340828202528,-7.71508112543066,-322.74165280418)) ;
#26166=CARTESIAN_POINT('Ctrl Pts',(17.631132195215,-8.16824121288439,-322.747432365097)) ;
#26167=CARTESIAN_POINT('Ctrl Pts',(17.3686908151508,-8.69875452392265,-322.75435074638)) ;
#26168=CARTESIAN_POINT('Ctrl Pts',(17.3257015301958,-8.78406610742526,-322.755468300551)) ;
#26169=CARTESIAN_POINT('Ctrl Pts',(17.1200548013404,-9.18478561513482,-322.760746816746)) ;
#26170=CARTESIAN_POINT('Ctrl Pts',(16.9494035152645,-9.49601403439818,-322.764931174595)) ;
#26171=CARTESIAN_POINT('Ctrl Pts',(16.7201446782959,-9.88823920657591,-322.770403673749)) ;
#26172=CARTESIAN_POINT('Ctrl Pts',(16.6693077448104,-9.97370001252993,-322.771608559738)) ;
#26173=CARTESIAN_POINT('Ctrl Pts',(16.5833280863899,-10.1157446863749,-322.773635073962)) ;
#26174=CARTESIAN_POINT('Ctrl Pts',(16.5485464651738,-10.1725449558792,-322.774451928531)) ;
#26175=CARTESIAN_POINT('Ctrl Pts',(16.4720324121002,-10.2960655693814,-322.77624330347)) ;
#26176=CARTESIAN_POINT('Ctrl Pts',(16.4301853513035,-10.3627133172376,-322.777219298011)) ;
#26177=CARTESIAN_POINT('Ctrl Pts',(16.2990757509775,-10.5687344061151,-322.780263328802)) ;
#26178=CARTESIAN_POINT('Ctrl Pts',(16.2084362314163,-10.7072224253812,-322.782348184611)) ;
#26179=CARTESIAN_POINT('Ctrl Pts',(16.0426081037255,-10.9536592200321,-322.78611652708)) ;
#26180=CARTESIAN_POINT('Ctrl Pts',(15.9680716300936,-11.0620347786483,-322.787794465269)) ;
#26181=CARTESIAN_POINT('Ctrl Pts',(15.5641149076755,-11.6367941532706,-322.796789246488)) ;
#26182=CARTESIAN_POINT('Ctrl Pts',(15.2153517394306,-12.089239997936,-322.80420199761)) ;
#26183=CARTESIAN_POINT('Ctrl Pts',(14.6516767220508,-12.7573862988255,-322.815414800771)) ;
#26184=CARTESIAN_POINT('Ctrl Pts',(14.4507890553021,-12.9844996882753,-322.819278912699)) ;
#26185=CARTESIAN_POINT('Ctrl Pts',(14.103420788886,-13.3591656750899,-322.825724215304)) ;
#26186=CARTESIAN_POINT('Ctrl Pts',(13.9597383439891,-13.5092372493731,-322.828326197325)) ;
#26187=CARTESIAN_POINT('Ctrl Pts',(13.7211677593507,-13.7505452056138,-322.832541873817)) ;
#26188=CARTESIAN_POINT('Ctrl Pts',(13.6277109279214,-13.8431727957304,-322.83416806751)) ;
#26189=CARTESIAN_POINT('Ctrl Pts',(13.4411783322032,-14.0243305738142,-322.837364752507)) ;
#26190=CARTESIAN_POINT('Ctrl Pts',(13.3481511496616,-14.1129013295838,-322.838935570202)) ;
#26191=CARTESIAN_POINT('Ctrl Pts',(13.1261199870023,-14.3201368594211,-322.842630921113)) ;
#26192=CARTESIAN_POINT('Ctrl Pts',(12.9963747851105,-14.4379911397491,-322.844748326307)) ;
#26193=CARTESIAN_POINT('Ctrl Pts',(12.2370340099874,-15.1092093244002,-322.856913022308)) ;
#26194=CARTESIAN_POINT('Ctrl Pts',(11.5737450844556,-15.6231120215995,-322.866606528407)) ;
#26195=CARTESIAN_POINT('Ctrl Pts',(10.6026776546373,-16.2796000475014,-322.880355191387)) ;
#26196=CARTESIAN_POINT('Ctrl Pts',(10.3212369001265,-16.4594720161391,-322.884297958115)) ;
#26197=CARTESIAN_POINT('Ctrl Pts',(9.95197561359519,-16.6822743362106,-322.889493266984)) ;
#26198=CARTESIAN_POINT('Ctrl Pts',(9.86827447074587,-16.731923218094,-322.890672413436)) ;
#26199=CARTESIAN_POINT('Ctrl Pts',(9.74073238547206,-16.8062872103374,-322.892473935217)) ;
#26200=CARTESIAN_POINT('Ctrl Pts',(9.69716259894677,-16.8314644260805,-322.893090191981)) ;
#26201=CARTESIAN_POINT('Ctrl Pts',(9.61185976675107,-16.8803163153879,-322.894298813693)) ;
#26202=CARTESIAN_POINT('Ctrl Pts',(9.57013585944713,-16.9040062325456,-322.894890949063)) ;
#26203=CARTESIAN_POINT('Ctrl Pts',(9.46867694390825,-16.9611163270856,-322.896332749112)) ;
#26204=CARTESIAN_POINT('Ctrl Pts',(9.40885224689384,-16.9943758200189,-322.897184504911)) ;
#26205=CARTESIAN_POINT('Ctrl Pts',(9.26175212567027,-17.0751411752099,-322.899281585752)) ;
#26206=CARTESIAN_POINT('Ctrl Pts',(9.17428560077857,-17.1222948891907,-322.900530864548)) ;
#26207=CARTESIAN_POINT('Ctrl Pts',(8.92179119011246,-17.2559258920544,-322.904139893733)) ;
#26208=CARTESIAN_POINT('Ctrl Pts',(8.75587601677594,-17.340702738409,-322.906514579502)) ;
#26209=CARTESIAN_POINT('Ctrl Pts',(8.04393633664461,-17.6916558625468,-322.916682092757)) ;
#26210=CARTESIAN_POINT('Ctrl Pts',(7.4868072470979,-17.9345286581561,-322.924572516332)) ;
#26211=CARTESIAN_POINT('Ctrl Pts',(6.57490146321972,-18.2821518305876,-322.937066907569)) ;
#26212=CARTESIAN_POINT('Ctrl Pts',(6.22692190783548,-18.4035825160469,-322.941742950214)) ;
#26213=CARTESIAN_POINT('Ctrl Pts',(5.72417099986703,-18.5631291656674,-322.948344820402)) ;
#26214=CARTESIAN_POINT('Ctrl Pts',(5.57205838008161,-18.6093541952061,-322.95032272096)) ;
#26215=CARTESIAN_POINT('Ctrl Pts',(5.30006249758082,-18.6883761953486,-322.953824508075)) ;
#26216=CARTESIAN_POINT('Ctrl Pts',(5.18039961511664,-18.7218996678123,-322.955353172802)) ;
#26217=CARTESIAN_POINT('Ctrl Pts',(4.94753469589348,-18.7847330854415,-322.958305386963)) ;
#26218=CARTESIAN_POINT('Ctrl Pts',(4.83437337503027,-18.8141736668697,-322.959729753044)) ;
#26219=CARTESIAN_POINT('Ctrl Pts',(4.58250643362185,-18.8772781531852,-322.962878235672)) ;
#26220=CARTESIAN_POINT('Ctrl Pts',(4.44368160306907,-18.9104386401209,-322.964599035349)) ;
#26221=CARTESIAN_POINT('Ctrl Pts',(3.70405155802869,-19.0785164167593,-322.97369633314)) ;
#26222=CARTESIAN_POINT('Ctrl Pts',(3.09745009698045,-19.1863386514346,-322.980897528552)) ;
#26223=CARTESIAN_POINT('Ctrl Pts',(2.20442059347208,-19.3016112149995,-322.991413987379)) ;
#26224=CARTESIAN_POINT('Ctrl Pts',(1.92131974369172,-19.3318440886322,-322.994737745289)) ;
#26225=CARTESIAN_POINT('Ctrl Pts',(1.36637633688919,-19.3787966821376,-323.001293732493)) ;
#26226=CARTESIAN_POINT('Ctrl Pts',(1.09464332293375,-19.3960434259652,-323.004522971869)) ;
#26227=CARTESIAN_POINT('Ctrl Pts',(0.737648523269101,-19.4111755419578,
-323.008833033094)) ;
#26228=CARTESIAN_POINT('Ctrl Pts',(0.652635922886302,-19.4142197265943,
-323.009864465169)) ;
#26229=CARTESIAN_POINT('Ctrl Pts',(0.501713535925727,-19.4186316221097,
-323.011706476176)) ;
#26230=CARTESIAN_POINT('Ctrl Pts',(0.435811563933142,-19.4202224198884,
-323.012514542114)) ;
#26231=CARTESIAN_POINT('Ctrl Pts',(0.312331841668734,-19.4225742223848,
-323.014036349015)) ;
#26232=CARTESIAN_POINT('Ctrl Pts',(0.254756450495114,-19.4234147292876,
-323.014748980697)) ;
#26233=CARTESIAN_POINT('Ctrl Pts',(0.131498421320462,-19.4246659545244,
-323.016280492723)) ;
#26234=CARTESIAN_POINT('Ctrl Pts',(0.0658157106903807,-19.4249995511085,
-323.017100204061)) ;
#26235=CARTESIAN_POINT('Ctrl Pts',(0.000132620481587507,-19.4249999995473,
-323.017923084864)) ;
#26236=CARTESIAN_POINT('Origin',(0.,0.,-328.125)) ;
#26237=CARTESIAN_POINT('',(-0.000256514499293202,-19.4249998742613,-324.730315018138)) ;
#26238=CARTESIAN_POINT('',(-0.000363249087843348,-19.4249999966036,-324.51951242736)) ;
#26239=CARTESIAN_POINT('',(-2.37887640734373E-15,-19.425,-328.125)) ;
#26240=CARTESIAN_POINT('Ctrl Pts',(-0.000256517197342009,-19.4249999983063,
-324.730314803303)) ;
#26241=CARTESIAN_POINT('Ctrl Pts',(0.125871645587764,-19.4250016638941,
-324.728731715617)) ;
#26242=CARTESIAN_POINT('Ctrl Pts',(0.25199692284909,-19.4237748883942,-324.727155907634)) ;
#26243=CARTESIAN_POINT('Ctrl Pts',(0.492716637007198,-19.4190884685471,
-324.724162542893)) ;
#26244=CARTESIAN_POINT('Ctrl Pts',(0.607309956047675,-19.4158425335503,
-324.722743703952)) ;
#26245=CARTESIAN_POINT('Ctrl Pts',(0.841981751499335,-19.4071156800803,
-324.719850540467)) ;
#26246=CARTESIAN_POINT('Ctrl Pts',(0.962051638294548,-19.4015341913279,
-324.71837692661)) ;
#26247=CARTESIAN_POINT('Ctrl Pts',(1.24291559657716,-19.3858644433473,-324.71494477395)) ;
#26248=CARTESIAN_POINT('Ctrl Pts',(1.40365138829175,-19.3748894776853,-324.712992043177)) ;
#26249=CARTESIAN_POINT('Ctrl Pts',(1.97416110602041,-19.3287984997702,-324.706096689383)) ;
#26250=CARTESIAN_POINT('Ctrl Pts',(2.38293536698671,-19.2826705519056,-324.701223762598)) ;
#26251=CARTESIAN_POINT('Ctrl Pts',(3.24382563400641,-19.1577288385263,-324.691005652723)) ;
#26252=CARTESIAN_POINT('Ctrl Pts',(3.69523829679299,-19.0758012305962,-324.685674552727)) ;
#26253=CARTESIAN_POINT('Ctrl Pts',(4.15399625952156,-18.9756438451624,-324.680170582219)) ;
#26254=CARTESIAN_POINT('Ctrl Pts',(4.16466371469226,-18.9733054686336,-324.680042548669)) ;
#26255=CARTESIAN_POINT('Ctrl Pts',(4.18908042593862,-18.9679315804666,-324.679749373779)) ;
#26256=CARTESIAN_POINT('Ctrl Pts',(4.20282836465936,-18.964890112875,-324.679584213758)) ;
#26257=CARTESIAN_POINT('Ctrl Pts',(4.23441152255483,-18.9578669160457,-324.679204583377)) ;
#26258=CARTESIAN_POINT('Ctrl Pts',(4.25224445378373,-18.9538749614433,-324.67899007854)) ;
#26259=CARTESIAN_POINT('Ctrl Pts',(4.34722066756254,-18.9324734687161,-324.677846790306)) ;
#26260=CARTESIAN_POINT('Ctrl Pts',(4.42426270576187,-18.9146181214092,-324.67691636852)) ;
#26261=CARTESIAN_POINT('Ctrl Pts',(4.74203652589619,-18.8389227732947,-324.673063179854)) ;
#26262=CARTESIAN_POINT('Ctrl Pts',(4.9817603298835,-18.7769535668658,-324.670119833988)) ;
#26263=CARTESIAN_POINT('Ctrl Pts',(5.28873764727473,-18.69130646114,-324.66627164003)) ;
#26264=CARTESIAN_POINT('Ctrl Pts',(5.35713633672492,-18.6718176239355,-324.665409090905)) ;
#26265=CARTESIAN_POINT('Ctrl Pts',(5.49060971635529,-18.6329932727356,-324.663714641459)) ;
#26266=CARTESIAN_POINT('Ctrl Pts',(5.55569319506363,-18.6136913719743,-324.662883119783)) ;
#26267=CARTESIAN_POINT('Ctrl Pts',(5.6926242952028,-18.5722993589952,-324.661121449546)) ;
#26268=CARTESIAN_POINT('Ctrl Pts',(5.76444747070642,-18.5501326190803,-324.660190453576)) ;
#26269=CARTESIAN_POINT('Ctrl Pts',(5.97506666101891,-18.4837880062138,-324.657441766396)) ;
#26270=CARTESIAN_POINT('Ctrl Pts',(6.11349644899662,-18.4384652757121,-324.655611433014)) ;
#26271=CARTESIAN_POINT('Ctrl Pts',(6.81086585539274,-18.2014255570839,-324.646292685717)) ;
#26272=CARTESIAN_POINT('Ctrl Pts',(7.3613598910765,-17.9858323805382,-324.638626154682)) ;
#26273=CARTESIAN_POINT('Ctrl Pts',(8.22659800554869,-17.6005855038616,-324.626424379731)) ;
#26274=CARTESIAN_POINT('Ctrl Pts',(8.54798077629938,-17.4467633158693,-324.621854655847)) ;
#26275=CARTESIAN_POINT('Ctrl Pts',(9.02988234878637,-17.1995990524533,-324.614982922847)) ;
#26276=CARTESIAN_POINT('Ctrl Pts',(9.19359363643251,-17.1126508462491,-324.612644624789)) ;
#26277=CARTESIAN_POINT('Ctrl Pts',(9.49452168690257,-16.9472609693741,-324.60834219153)) ;
#26278=CARTESIAN_POINT('Ctrl Pts',(9.63207400723271,-16.869461960622,-324.606373869676)) ;
#26279=CARTESIAN_POINT('Ctrl Pts',(9.85656108998313,-16.738852116167,-324.603159025708)) ;
#26280=CARTESIAN_POINT('Ctrl Pts',(9.94405743788405,-16.6870215552464,-324.601905350647)) ;
#26281=CARTESIAN_POINT('Ctrl Pts',(10.1306587110563,-16.5744949803651,-324.599230028075)) ;
#26282=CARTESIAN_POINT('Ctrl Pts',(10.2296341597051,-16.5135918191769,-324.597810005638)) ;
#26283=CARTESIAN_POINT('Ctrl Pts',(10.4864027606522,-16.3523985072033,-324.594122521985)) ;
#26284=CARTESIAN_POINT('Ctrl Pts',(10.6433050625315,-16.2507119009682,-324.591865741618)) ;
#26285=CARTESIAN_POINT('Ctrl Pts',(11.2854290470963,-15.8212692710672,-324.582604346409)) ;
#26286=CARTESIAN_POINT('Ctrl Pts',(11.7571769603466,-15.4739219791359,-324.57574898153)) ;
#26287=CARTESIAN_POINT('Ctrl Pts',(12.511190882758,-14.8643278951423,-324.564424003201)) ;
#26288=CARTESIAN_POINT('Ctrl Pts',(12.8026405330555,-14.614052679681,-324.55994474344)) ;
#26289=CARTESIAN_POINT('Ctrl Pts',(13.1980202915024,-14.2536194184083,-324.553615417755)) ;
#26290=CARTESIAN_POINT('Ctrl Pts',(13.3083734269114,-14.1506396596358,-324.551819844298)) ;
#26291=CARTESIAN_POINT('Ctrl Pts',(13.4204144461015,-14.0436148185614,-324.549960967423)) ;
#26292=CARTESIAN_POINT('Ctrl Pts',(13.4233129959695,-14.0408443225285,-324.549912852529)) ;
#26293=CARTESIAN_POINT('Ctrl Pts',(13.4282718711619,-14.0361015844445,-324.549830494091)) ;
#26294=CARTESIAN_POINT('Ctrl Pts',(13.4303326202965,-14.034129785736,-324.549796255889)) ;
#26295=CARTESIAN_POINT('Ctrl Pts',(13.4338560439608,-14.0307569607785,-324.549737694403)) ;
#26296=CARTESIAN_POINT('Ctrl Pts',(13.4353189337409,-14.0293561595305,-324.54971337385)) ;
#26297=CARTESIAN_POINT('Ctrl Pts',(13.437819155381,-14.0269613035568,-324.54967179665)) ;
#26298=CARTESIAN_POINT('Ctrl Pts',(13.4388565949491,-14.0259673635935,-324.549654541409)) ;
#26299=CARTESIAN_POINT('Ctrl Pts',(13.4446378196615,-14.0204273140564,-324.549558366964)) ;
#26300=CARTESIAN_POINT('Ctrl Pts',(13.4493794080407,-14.0158789131888,-324.549479419718)) ;
#26301=CARTESIAN_POINT('Ctrl Pts',(13.4583102900934,-14.007303198867,-324.549330592116)) ;
#26302=CARTESIAN_POINT('Ctrl Pts',(13.4625000861162,-14.0032764094957,-324.549260718279)) ;
#26303=CARTESIAN_POINT('Ctrl Pts',(13.4703934737861,-13.9956833022396,-324.549128977615)) ;
#26304=CARTESIAN_POINT('Ctrl Pts',(13.4740974577576,-13.9921173928056,-324.54906711594)) ;
#26305=CARTESIAN_POINT('Ctrl Pts',(13.481077610462,-13.9853920994617,-324.548950457728)) ;
#26306=CARTESIAN_POINT('Ctrl Pts',(13.4843540854478,-13.9822330338629,-324.548895665254)) ;
#26307=CARTESIAN_POINT('Ctrl Pts',(13.4905306476756,-13.9762736126845,-324.548792311602)) ;
#26308=CARTESIAN_POINT('Ctrl Pts',(13.4934309740496,-13.9734735052188,-324.548743753624)) ;
#26309=CARTESIAN_POINT('Ctrl Pts',(13.498900431314,-13.9681897508018,-324.548652132908)) ;
#26310=CARTESIAN_POINT('Ctrl Pts',(13.5014697490095,-13.9657062974099,-324.548609072691)) ;
#26311=CARTESIAN_POINT('Ctrl Pts',(13.5063168374287,-13.9610186066021,-324.548527799163)) ;
#26312=CARTESIAN_POINT('Ctrl Pts',(13.5085947541932,-13.9588145203626,-324.548489587838)) ;
#26313=CARTESIAN_POINT('Ctrl Pts',(13.5128937890432,-13.9546527854814,-324.548417441894)) ;
#26314=CARTESIAN_POINT('Ctrl Pts',(13.5149150214764,-13.9526952550243,-324.548383508838)) ;
#26315=CARTESIAN_POINT('Ctrl Pts',(13.5187311246206,-13.9489978145049,-324.548319418425)) ;
#26316=CARTESIAN_POINT('Ctrl Pts',(13.5205260849428,-13.9472579970125,-324.548289262301)) ;
#26317=CARTESIAN_POINT('Ctrl Pts',(13.5239163009915,-13.9439706620255,-324.548232285751)) ;
#26318=CARTESIAN_POINT('Ctrl Pts',(13.5255116270924,-13.9424232171111,-324.548205466298)) ;
#26319=CARTESIAN_POINT('Ctrl Pts',(13.5285259267417,-13.9394983826594,-324.548154776697)) ;
#26320=CARTESIAN_POINT('Ctrl Pts',(13.5299449555774,-13.9381210501894,-324.548130907318)) ;
#26321=CARTESIAN_POINT('Ctrl Pts',(13.5326271279239,-13.9355168945112,-324.548085778468)) ;
#26322=CARTESIAN_POINT('Ctrl Pts',(13.5338903150372,-13.9342901161548,-324.548064519603)) ;
#26323=CARTESIAN_POINT('Ctrl Pts',(13.5362787561782,-13.9319698857294,-324.548024313505)) ;
#26324=CARTESIAN_POINT('Ctrl Pts',(13.5374040445636,-13.9308764690549,-324.548005366752)) ;
#26325=CARTESIAN_POINT('Ctrl Pts',(13.5395324490336,-13.9288078462888,-324.547969522558)) ;
#26326=CARTESIAN_POINT('Ctrl Pts',(13.5405355922734,-13.9278326681378,-324.547952625497)) ;
#26327=CARTESIAN_POINT('Ctrl Pts',(13.5424335578306,-13.9259872141917,-324.547920649783)) ;
#26328=CARTESIAN_POINT('Ctrl Pts',(13.5433284016245,-13.9251169605083,-324.547905571433)) ;
#26329=CARTESIAN_POINT('Ctrl Pts',(13.5450219554417,-13.9234696275172,-324.547877029699)) ;
#26330=CARTESIAN_POINT('Ctrl Pts',(13.5458206825035,-13.922692565709,-324.547863566554)) ;
#26331=CARTESIAN_POINT('Ctrl Pts',(13.5473327385723,-13.9212212704635,-324.547838075791)) ;
#26332=CARTESIAN_POINT('Ctrl Pts',(13.5480460810647,-13.9205270509469,-324.547826048364)) ;
#26333=CARTESIAN_POINT('Ctrl Pts',(13.549396836602,-13.9192123037056,-324.547803270597)) ;
#26334=CARTESIAN_POINT('Ctrl Pts',(13.5500342603979,-13.9185917870089,-324.547792520409)) ;
#26335=CARTESIAN_POINT('Ctrl Pts',(13.5512415398332,-13.917416368053,-324.547772157067)) ;
#26336=CARTESIAN_POINT('Ctrl Pts',(13.5518114039996,-13.9168614745954,-324.547762544035)) ;
#26337=CARTESIAN_POINT('Ctrl Pts',(13.5541461590969,-13.9145877756753,-324.547723154738)) ;
#26338=CARTESIAN_POINT('Ctrl Pts',(13.5559107570913,-13.9128686695055,-324.547693374316)) ;
#26339=CARTESIAN_POINT('Ctrl Pts',(13.5593667439018,-13.909500497307,-324.547635029041)) ;
#26340=CARTESIAN_POINT('Ctrl Pts',(13.5610581590446,-13.907851458339,-324.547606464563)) ;
#26341=CARTESIAN_POINT('Ctrl Pts',(13.6113030912996,-13.8588474662358,-324.546757653284)) ;
#26342=CARTESIAN_POINT('Ctrl Pts',(13.6596085349735,-13.8112388870189,-324.545933864278)) ;
#26343=CARTESIAN_POINT('Ctrl Pts',(13.7417232814844,-13.729456544378,-324.544519251147)) ;
#26344=CARTESIAN_POINT('Ctrl Pts',(13.7756568982474,-13.6954084556214,-324.543930456384)) ;
#26345=CARTESIAN_POINT('Ctrl Pts',(13.8531958091174,-13.6170282215136,-324.542574888772)) ;
#26346=CARTESIAN_POINT('Ctrl Pts',(13.8967153045163,-13.5726119610664,-324.541806627025)) ;
#26347=CARTESIAN_POINT('Ctrl Pts',(14.0191406703622,-13.44645778366,-324.539625352577)) ;
#26348=CARTESIAN_POINT('Ctrl Pts',(14.0975437442527,-13.3642355706125,-324.53820463081)) ;
#26349=CARTESIAN_POINT('Ctrl Pts',(14.5608120248477,-12.8697873477605,-324.529679537809)) ;
#26350=CARTESIAN_POINT('Ctrl Pts',(14.9282977049269,-12.441647794467,-324.522381766745)) ;
#26351=CARTESIAN_POINT('Ctrl Pts',(15.5267684436833,-11.6796441076633,-324.509883731573)) ;
#26352=CARTESIAN_POINT('Ctrl Pts',(15.7668828777971,-11.3534149082756,-324.50467318165)) ;
#26353=CARTESIAN_POINT('Ctrl Pts',(16.1549650848596,-10.7900708977611,-324.495976068044)) ;
#26354=CARTESIAN_POINT('Ctrl Pts',(16.3083332618964,-10.5568363432292,-324.492457391103)) ;
#26355=CARTESIAN_POINT('Ctrl Pts',(16.5331213324466,-10.1983947721088,-324.487180013928)) ;
#26356=CARTESIAN_POINT('Ctrl Pts',(16.6082614965002,-10.0755648505417,-324.485394011543)) ;
#26357=CARTESIAN_POINT('Ctrl Pts',(16.7456823833816,-9.84521117381113,-324.482085994218)) ;
#26358=CARTESIAN_POINT('Ctrl Pts',(16.8083105032362,-9.73790324533171,-324.480561428218)) ;
#26359=CARTESIAN_POINT('Ctrl Pts',(16.9485635630967,-9.49220694874396,-324.477107203508)) ;
#26360=CARTESIAN_POINT('Ctrl Pts',(17.0255310828992,-9.35345342896753,-324.475182485457)) ;
#26361=CARTESIAN_POINT('Ctrl Pts',(17.2751091842933,-8.8902357013305,-324.468838184852)) ;
#26362=CARTESIAN_POINT('Ctrl Pts',(17.4402116662648,-8.5618167475796,-324.464472037462)) ;
#26363=CARTESIAN_POINT('Ctrl Pts',(17.6094478464844,-8.19993869350873,-324.459768034931)) ;
#26364=CARTESIAN_POINT('Ctrl Pts',(17.6229258741506,-8.17093211757172,-324.459391704819)) ;
#26365=CARTESIAN_POINT('Ctrl Pts',(17.8806613827085,-7.61264556268122,-324.452161847256)) ;
#26366=CARTESIAN_POINT('Ctrl Pts',(18.101043099233,-7.07267000009167,-324.445409332011)) ;
#26367=CARTESIAN_POINT('Ctrl Pts',(18.3414122534194,-6.39850458998067,-324.436978036906)) ;
#26368=CARTESIAN_POINT('Ctrl Pts',(18.3847315455827,-6.27295069197035,-324.435407301272)) ;
#26369=CARTESIAN_POINT('Ctrl Pts',(18.4794735006115,-5.98894257655249,-324.43184483854)) ;
#26370=CARTESIAN_POINT('Ctrl Pts',(18.5301522950866,-5.83025126503291,-324.429847776945)) ;
#26371=CARTESIAN_POINT('Ctrl Pts',(18.6018111209536,-5.59548654778721,-324.426872262453)) ;
#26372=CARTESIAN_POINT('Ctrl Pts',(18.6243788989533,-5.51990555113917,-324.425911106243)) ;
#26373=CARTESIAN_POINT('Ctrl Pts',(18.6651392612199,-5.38030028139642,-324.424128222736)) ;
#26374=CARTESIAN_POINT('Ctrl Pts',(18.6834642997845,-5.31631606303256,-324.42330803459)) ;
#26375=CARTESIAN_POINT('Ctrl Pts',(18.7282510747588,-5.15684538950689,-324.421256930535)) ;
#26376=CARTESIAN_POINT('Ctrl Pts',(18.7543117240835,-5.06124830529967,-324.420021348324)) ;
#26377=CARTESIAN_POINT('Ctrl Pts',(18.8622572587937,-4.65299210361357,-324.414725295977)) ;
#26378=CARTESIAN_POINT('Ctrl Pts',(18.9370633718439,-4.33851524724382,-324.410598301299)) ;
#26379=CARTESIAN_POINT('Ctrl Pts',(19.0415365913418,-3.8449175000952,-324.404115201769)) ;
#26380=CARTESIAN_POINT('Ctrl Pts',(19.0765989743507,-3.66699848317527,-324.401777065726)) ;
#26381=CARTESIAN_POINT('Ctrl Pts',(19.1919333517009,-3.03524524941692,-324.393492217077)) ;
#26382=CARTESIAN_POINT('Ctrl Pts',(19.258541045613,-2.57907301058873,-324.387545118158)) ;
#26383=CARTESIAN_POINT('Ctrl Pts',(19.3245237143148,-1.97837914170319,-324.37984798158)) ;
#26384=CARTESIAN_POINT('Ctrl Pts',(19.3386060076449,-1.83562484007966,-324.378028262132)) ;
#26385=CARTESIAN_POINT('Ctrl Pts',(19.3697622472116,-1.47944957823182,-324.373514213664)) ;
#26386=CARTESIAN_POINT('Ctrl Pts',(19.3848914093966,-1.26587749898368,-324.370830969847)) ;
#26387=CARTESIAN_POINT('Ctrl Pts',(19.4036754400626,-0.919575220124958,
-324.366520391534)) ;
#26388=CARTESIAN_POINT('Ctrl Pts',(19.4095053918465,-0.786981365495109,
-324.364879425956)) ;
#26389=CARTESIAN_POINT('Ctrl Pts',(19.4182273292702,-0.528204614963243,
-324.361695059482)) ;
#26390=CARTESIAN_POINT('Ctrl Pts',(19.4212492529852,-0.402032621095737,
-324.360150896082)) ;
#26391=CARTESIAN_POINT('Ctrl Pts',(19.425230488021,-0.121697365432233,-324.35673779676)) ;
#26392=CARTESIAN_POINT('Ctrl Pts',(19.4255845678111,0.0324660379283422,
-324.354872818804)) ;
#26393=CARTESIAN_POINT('Ctrl Pts',(19.418832499331,0.735256114931439,-324.346419201716)) ;
#26394=CARTESIAN_POINT('Ctrl Pts',(19.3903191585564,1.28342579855236,-324.339967550575)) ;
#26395=CARTESIAN_POINT('Ctrl Pts',(19.2888463679684,2.35594981702353,-324.327372985851)) ;
#26396=CARTESIAN_POINT('Ctrl Pts',(19.2175889248286,2.87999431961308,-324.321231531113)) ;
#26397=CARTESIAN_POINT('Ctrl Pts',(19.0951867294415,3.56841175327356,-324.312916103241)) ;
#26398=CARTESIAN_POINT('Ctrl Pts',(19.0631169427811,3.73594578876227,-324.310872211801)) ;
#26399=CARTESIAN_POINT('Ctrl Pts',(19.0128619591295,3.98095875729358,-324.307841030905)) ;
#26400=CARTESIAN_POINT('Ctrl Pts',(18.99640049962,4.05878313548917,-324.306871960192)) ;
#26401=CARTESIAN_POINT('Ctrl Pts',(18.9653222899369,4.20137883114159,-324.305083181363)) ;
#26402=CARTESIAN_POINT('Ctrl Pts',(18.9508506017545,4.26618038530291,-324.304265125958)) ;
#26403=CARTESIAN_POINT('Ctrl Pts',(18.9142329262094,4.42628405720179,-324.302231806478)) ;
#26404=CARTESIAN_POINT('Ctrl Pts',(18.8916986239486,4.52149541707464,-324.301012066303)) ;
#26405=CARTESIAN_POINT('Ctrl Pts',(18.7955134697668,4.91461827353979,-324.295937893922)) ;
#26406=CARTESIAN_POINT('Ctrl Pts',(18.7155274983197,5.21093361934284,-324.292023534478)) ;
#26407=CARTESIAN_POINT('Ctrl Pts',(18.6013865024622,5.59716314591487,-324.286852454013)) ;
#26408=CARTESIAN_POINT('Ctrl Pts',(18.5735372737967,5.68889516736497,-324.285619062832)) ;
#26409=CARTESIAN_POINT('Ctrl Pts',(18.3868376954508,6.28787365493976,-324.277537520985)) ;
#26410=CARTESIAN_POINT('Ctrl Pts',(18.2079028459711,6.7886251379805,-324.270656866799)) ;
#26411=CARTESIAN_POINT('Ctrl Pts',(17.9504630604211,7.42533520745249,-324.261893320593)) ;
#26412=CARTESIAN_POINT('Ctrl Pts',(17.8905452777847,7.56856107608931,-324.259920427049)) ;
#26413=CARTESIAN_POINT('Ctrl Pts',(17.7392134782481,7.91845906840116,-324.255100309245)) ;
#26414=CARTESIAN_POINT('Ctrl Pts',(17.6458975447267,8.12428390398573,-324.252264717981)) ;
#26415=CARTESIAN_POINT('Ctrl Pts',(17.4911916777543,8.45026776639919,-324.247776341995)) ;
#26416=CARTESIAN_POINT('Ctrl Pts',(17.4321044106705,8.57149622335695,-324.246107712866)) ;
#26417=CARTESIAN_POINT('Ctrl Pts',(17.3151450670212,8.80524752328319,-324.242891072728)) ;
#26418=CARTESIAN_POINT('Ctrl Pts',(17.257426476415,8.91783965421954,-324.241342055688)) ;
#26419=CARTESIAN_POINT('Ctrl Pts',(17.1159536176771,9.18729419968506,-324.237634838935)) ;
#26420=CARTESIAN_POINT('Ctrl Pts',(17.0311373660391,9.34358620124853,-324.235484484652)) ;
#26421=CARTESIAN_POINT('Ctrl Pts',(16.5834638954172,10.1421659680954,-324.224485926699)) ;
#26422=CARTESIAN_POINT('Ctrl Pts',(16.1863780064869,10.7645702498429,-324.215901696527)) ;
#26423=CARTESIAN_POINT('Ctrl Pts',(15.516966172878,11.6927232401586,-324.202524228862)) ;
#26424=CARTESIAN_POINT('Ctrl Pts',(15.2687729781095,12.0150150328863,-324.197755617331)) ;
#26425=CARTESIAN_POINT('Ctrl Pts',(14.9348352809406,12.4215774745786,-324.191446573768)) ;
#26426=CARTESIAN_POINT('Ctrl Pts',(14.8581732385816,12.5131762464725,-324.190004892964)) ;
#26427=CARTESIAN_POINT('Ctrl Pts',(14.7352030803571,12.6573822567672,-324.187698134258)) ;
#26428=CARTESIAN_POINT('Ctrl Pts',(14.6894466234363,12.7104560620122,-324.186841037902)) ;
#26429=CARTESIAN_POINT('Ctrl Pts',(14.6022016638557,12.8105528302915,-324.185207934169)) ;
#26430=CARTESIAN_POINT('Ctrl Pts',(14.5607706929394,12.8576247443385,-324.184432915606)) ;
#26431=CARTESIAN_POINT('Ctrl Pts',(14.4416251738034,12.9916778148437,-324.182206699129)) ;
#26432=CARTESIAN_POINT('Ctrl Pts',(14.3633541926598,13.0781606650973,-324.180747296458)) ;
#26433=CARTESIAN_POINT('Ctrl Pts',(14.0418659142358,13.4270106545796,-324.174774885447)) ;
#26434=CARTESIAN_POINT('Ctrl Pts',(13.7922015111667,13.683339876464,-324.170188161503)) ;
#26435=CARTESIAN_POINT('Ctrl Pts',(13.4309912329852,14.0342570680523,-324.163702478683)) ;
#26436=CARTESIAN_POINT('Ctrl Pts',(13.3252393669374,14.1347052588773,-324.161820737723)) ;
#26437=CARTESIAN_POINT('Ctrl Pts',(12.8966576208982,14.5327078769028,-324.154274561331)) ;
#26438=CARTESIAN_POINT('Ctrl Pts',(12.5649123835614,14.8204707748305,-324.148615306103)) ;
#26439=CARTESIAN_POINT('Ctrl Pts',(12.063003476793,15.2268620032086,-324.140395103994)) ;
#26440=CARTESIAN_POINT('Ctrl Pts',(11.9002372904511,15.354404318099,-324.137778867419)) ;
#26441=CARTESIAN_POINT('Ctrl Pts',(11.5937868949547,15.5867360511484,-324.1329489242)) ;
#26442=CARTESIAN_POINT('Ctrl Pts',(11.4506398493319,15.6921981401101,-324.130730385727)) ;
#26443=CARTESIAN_POINT('Ctrl Pts',(11.2031853435626,15.8693185102424,-324.126959649701)) ;
#26444=CARTESIAN_POINT('Ctrl Pts',(11.0995885623812,15.9419498687279,-324.125399870103)) ;
#26445=CARTESIAN_POINT('Ctrl Pts',(10.8841097264858,16.0899027035284,-324.122193784817)) ;
#26446=CARTESIAN_POINT('Ctrl Pts',(10.7721378284229,16.1650815095757,-324.120548650556)) ;
#26447=CARTESIAN_POINT('Ctrl Pts',(10.4704479396077,16.3631117657161,-324.116169918292)) ;
#26448=CARTESIAN_POINT('Ctrl Pts',(10.2793534988691,16.4838283964614,-324.113452621711)) ;
#26449=CARTESIAN_POINT('Ctrl Pts',(9.86464297391063,16.7357894524273,-324.107663512867)) ;
#26450=CARTESIAN_POINT('Ctrl Pts',(9.64041745778643,16.8659473822315,-324.104598986468)) ;
#26451=CARTESIAN_POINT('Ctrl Pts',(8.90740023340052,17.2720527066333,-324.094748363309)) ;
#26452=CARTESIAN_POINT('Ctrl Pts',(8.38886557993144,17.5297608709405,-324.088043465915)) ;
#26453=CARTESIAN_POINT('Ctrl Pts',(7.73855120047659,17.8174906185905,-324.079665980757)) ;
#26454=CARTESIAN_POINT('Ctrl Pts',(7.61695685527719,17.8698101512118,-324.078100401765)) ;
#26455=CARTESIAN_POINT('Ctrl Pts',(7.42078717273703,17.9518518614838,-324.0755701538)) ;
#26456=CARTESIAN_POINT('Ctrl Pts',(7.34654577283159,17.9823617111985,-324.074611542018)) ;
#26457=CARTESIAN_POINT('Ctrl Pts',(7.16327429091798,18.0563535704242,-324.072240492881)) ;
#26458=CARTESIAN_POINT('Ctrl Pts',(7.05403516699561,18.0993091202385,-324.070823222436)) ;
#26459=CARTESIAN_POINT('Ctrl Pts',(6.87934636894805,18.1661793633048,-324.06854594957)) ;
#26460=CARTESIAN_POINT('Ctrl Pts',(6.81414564487461,18.1907366055378,-324.067693583296)) ;
#26461=CARTESIAN_POINT('Ctrl Pts',(6.68968579680111,18.2368501955939,-324.066060807299)) ;
#26462=CARTESIAN_POINT('Ctrl Pts',(6.63045108654184,18.2584698015542,-324.065281306199)) ;
#26463=CARTESIAN_POINT('Ctrl Pts',(6.45948572471922,18.3199273962544,-324.063025681475)) ;
#26464=CARTESIAN_POINT('Ctrl Pts',(6.3474941456886,18.3590308469753,-324.061541024162)) ;
#26465=CARTESIAN_POINT('Ctrl Pts',(5.81915797722385,18.538094667918,-324.054515197923)) ;
#26466=CARTESIAN_POINT('Ctrl Pts',(5.39850248749337,18.6649329852563,-324.048861014837)) ;
#26467=CARTESIAN_POINT('Ctrl Pts',(4.5113039961088,18.8999413257944,-324.037023178291)) ;
#26468=CARTESIAN_POINT('Ctrl Pts',(4.04432598583278,19.0053433169365,-324.030842521955)) ;
#26469=CARTESIAN_POINT('Ctrl Pts',(3.42985226523001,19.1203615292352,-324.022875955431)) ;
#26470=CARTESIAN_POINT('Ctrl Pts',(3.28547088461554,19.1456990652919,-324.021015511383)) ;
#26471=CARTESIAN_POINT('Ctrl Pts',(2.92637835450433,19.2045346957661,-324.016419498541)) ;
#26472=CARTESIAN_POINT('Ctrl Pts',(2.71136555680763,19.2360687306529,-324.013695170536)) ;
#26473=CARTESIAN_POINT('Ctrl Pts',(2.36367789851189,19.2811156199011,-324.009336618072)) ;
#26474=CARTESIAN_POINT('Ctrl Pts',(2.23131414254014,19.2968813545335,-324.007688177499)) ;
#26475=CARTESIAN_POINT('Ctrl Pts',(1.97365977504464,19.3248838745931,-324.004500181916)) ;
#26476=CARTESIAN_POINT('Ctrl Pts',(1.84839171316729,19.3372675887003,-324.002959746504)) ;
#26477=CARTESIAN_POINT('Ctrl Pts',(1.54192781274599,19.3645587392681,-323.999213364857)) ;
#26478=CARTESIAN_POINT('Ctrl Pts',(1.36062595790063,19.3781416468176,-323.997016048999)) ;
#26479=CARTESIAN_POINT('Ctrl Pts',(0.481697117337168,19.4315940296009,-323.986444469316)) ;
#26480=CARTESIAN_POINT('Ctrl Pts',(-0.217547312467332,19.4363461749917,
-323.978300685476)) ;
#26481=CARTESIAN_POINT('Ctrl Pts',(-1.34665732998864,19.3830707002484,-323.965093091122)) ;
#26482=CARTESIAN_POINT('Ctrl Pts',(-1.77699310810494,19.3483645174177,-323.960040303611)) ;
#26483=CARTESIAN_POINT('Ctrl Pts',(-2.32718005746257,19.2854810742828,-323.953403329958)) ;
#26484=CARTESIAN_POINT('Ctrl Pts',(-2.44841304287205,19.270464986377,-323.951929586599)) ;
#26485=CARTESIAN_POINT('Ctrl Pts',(-2.63948654898389,19.2449661380225,-323.949583993282)) ;
#26486=CARTESIAN_POINT('Ctrl Pts',(-2.70942545630609,19.2352443337843,-323.948720584755)) ;
#26487=CARTESIAN_POINT('Ctrl Pts',(-2.84096362654731,19.2162283322199,-323.94708638334)) ;
#26488=CARTESIAN_POINT('Ctrl Pts',(-2.90257422886891,19.2070187295803,-323.946316678993)) ;
#26489=CARTESIAN_POINT('Ctrl Pts',(-3.07706368467753,19.1800771629516,-323.944125735647)) ;
#26490=CARTESIAN_POINT('Ctrl Pts',(-3.18983180186316,19.1616453864455,-323.942696681624)) ;
#26491=CARTESIAN_POINT('Ctrl Pts',(-3.96824790430937,19.0273524374654,-323.932756716078)) ;
#26492=CARTESIAN_POINT('Ctrl Pts',(-4.62761855989996,18.8778250618139,-323.923971883679)) ;
#26493=CARTESIAN_POINT('Ctrl Pts',(-5.60415085812844,18.6021255205123,-323.910908739748)) ;
#26494=CARTESIAN_POINT('Ctrl Pts',(-5.92797981419138,18.5014766084425,-323.90656452254)) ;
#26495=CARTESIAN_POINT('Ctrl Pts',(-6.48574386535623,18.3119705275486,-323.899096358991)) ;
#26496=CARTESIAN_POINT('Ctrl Pts',(-6.72090440067535,18.2269740352565,-323.895951905491)) ;
#26497=CARTESIAN_POINT('Ctrl Pts',(-7.08425283639934,18.0876571089554,-323.891104698753)) ;
#26498=CARTESIAN_POINT('Ctrl Pts',(-7.21360812391362,18.0364585171606,-323.889381236262)) ;
#26499=CARTESIAN_POINT('Ctrl Pts',(-7.45819832737231,17.9365979636946,-323.88612644729)) ;
#26500=CARTESIAN_POINT('Ctrl Pts',(-7.57353504542024,17.8882038160591,-323.884593354671)) ;
#26501=CARTESIAN_POINT('Ctrl Pts',(-7.83920315812354,17.7737020941868,-323.881065128646)) ;
#26502=CARTESIAN_POINT('Ctrl Pts',(-7.98917974606112,17.7067952880801,-323.879075716891)) ;
#26503=CARTESIAN_POINT('Ctrl Pts',(-8.54045436631188,17.4524334512764,-323.871766159098)) ;
#26504=CARTESIAN_POINT('Ctrl Pts',(-8.93615502989921,17.2531715535896,-323.866528474948)) ;
#26505=CARTESIAN_POINT('Ctrl Pts',(-9.4963717609437,16.9466175085144,-323.859038723582)) ;
#26506=CARTESIAN_POINT('Ctrl Pts',(-9.66661576643364,16.8500878710835,-323.856751827851)) ;
#26507=CARTESIAN_POINT('Ctrl Pts',(-10.2965813990487,16.4802027576613,-323.84821915828)) ;
#26508=CARTESIAN_POINT('Ctrl Pts',(-10.7464086564466,16.1904715545451,-323.841990346003)) ;
#26509=CARTESIAN_POINT('Ctrl Pts',(-11.2811101066073,15.8139613020223,-323.834147853795)) ;
#26510=CARTESIAN_POINT('Ctrl Pts',(-11.3778829491473,15.7444782966092,-323.832709865522)) ;
#26511=CARTESIAN_POINT('Ctrl Pts',(-11.5305041852741,15.6327540779715,-323.830407571966)) ;
#26512=CARTESIAN_POINT('Ctrl Pts',(-11.5867739897787,15.5910934617566,-323.829551195723)) ;
#26513=CARTESIAN_POINT('Ctrl Pts',(-11.693053531867,15.5115138757633,-323.827918171387)) ;
#26514=CARTESIAN_POINT('Ctrl Pts',(-11.7431071278147,15.4736549848682,-323.827142500227)) ;
#26515=CARTESIAN_POINT('Ctrl Pts',(-11.8858919402527,15.3645654186613,-323.824911984799)) ;
#26516=CARTESIAN_POINT('Ctrl Pts',(-11.9781645725456,15.2927391638277,-323.823448887924)) ;
#26517=CARTESIAN_POINT('Ctrl Pts',(-12.3532041578665,14.9953264616059,-323.817422531285)) ;
#26518=CARTESIAN_POINT('Ctrl Pts',(-12.6302917279212,14.7626961879381,-323.812783894701)) ;
#26519=CARTESIAN_POINT('Ctrl Pts',(-13.2996874857151,14.1680528040269,-323.801251471557)) ;
#26520=CARTESIAN_POINT('Ctrl Pts',(-13.6838801597236,13.7973487684485,-323.794342853331)) ;
#26521=CARTESIAN_POINT('Ctrl Pts',(-14.1597301004758,13.2987544949148,-323.785547788573)) ;
#26522=CARTESIAN_POINT('Ctrl Pts',(-14.2657833881751,13.1849251810078,-323.78357069257)) ;
#26523=CARTESIAN_POINT('Ctrl Pts',(-14.5227155517269,12.9024248212297,-323.778742262111)) ;
#26524=CARTESIAN_POINT('Ctrl Pts',(-14.6720363590043,12.732367517934,-323.775902574225)) ;
#26525=CARTESIAN_POINT('Ctrl Pts',(-14.9055849419306,12.4568200054184,-323.77140942221)) ;
#26526=CARTESIAN_POINT('Ctrl Pts',(-14.9917433325266,12.3529939294072,-323.769740052485)) ;
#26527=CARTESIAN_POINT('Ctrl Pts',(-15.1565737827816,12.1500986511782,-323.766522973728)) ;
#26528=CARTESIAN_POINT('Ctrl Pts',(-15.2353735282519,12.0511418367658,-323.764974247692)) ;
#26529=CARTESIAN_POINT('Ctrl Pts',(-15.4224964045813,11.8113837425712,-323.761269393801)) ;
#26530=CARTESIAN_POINT('Ctrl Pts',(-15.5298656485882,11.6698523695491,-323.759121084207)) ;
#26531=CARTESIAN_POINT('Ctrl Pts',(-16.0736049585664,10.9323132982139,-323.748112522918)) ;
#26532=CARTESIAN_POINT('Ctrl Pts',(-16.4776618053925,10.3132396543224,-323.739517163243)) ;
#26533=CARTESIAN_POINT('Ctrl Pts',(-17.0477482798001,9.32040262183154,-323.726133710761)) ;
#26534=CARTESIAN_POINT('Ctrl Pts',(-17.2389175073694,8.96188306883237,-323.721370567336)) ;
#26535=CARTESIAN_POINT('Ctrl Pts',(-17.4715480200683,8.49057646834734,-323.71506784694)) ;
#26536=CARTESIAN_POINT('Ctrl Pts',(-17.523402668829,8.38303273438424,-323.713626801781)) ;
#26537=CARTESIAN_POINT('Ctrl Pts',(-17.6041095747364,8.21162955901805,-323.711320811837)) ;
#26538=CARTESIAN_POINT('Ctrl Pts',(-17.6336134515915,8.14808017680627,-323.710463839554)) ;
#26539=CARTESIAN_POINT('Ctrl Pts',(-17.6888743853544,8.02734584519176,-323.708830750218)) ;
#26540=CARTESIAN_POINT('Ctrl Pts',(-17.7146995681574,7.97019306780394,-323.70805561994)) ;
#26541=CARTESIAN_POINT('Ctrl Pts',(-17.7877822310987,7.80634645500603,-323.705828667086)) ;
#26542=CARTESIAN_POINT('Ctrl Pts',(-17.8343556715796,7.69935058278744,-323.704368631563)) ;
#26543=CARTESIAN_POINT('Ctrl Pts',(-18.0200488044502,7.26202027723913,-323.698387031033)) ;
#26544=CARTESIAN_POINT('Ctrl Pts',(-18.1509768795058,6.92828513897287,-323.693791468658)) ;
#26545=CARTESIAN_POINT('Ctrl Pts',(-18.3217870991037,6.45474707416447,-323.687308233108)) ;
#26546=CARTESIAN_POINT('Ctrl Pts',(-18.3694499854059,6.31782791147704,-323.685437792121)) ;
#26547=CARTESIAN_POINT('Ctrl Pts',(-18.5552836343323,5.76410319740506,-323.677902025856)) ;
#26548=CARTESIAN_POINT('Ctrl Pts',(-18.6808364219737,5.34320018011998,-323.672241864091)) ;
#26549=CARTESIAN_POINT('Ctrl Pts',(-18.8273153261259,4.78354020869679,-323.664878221018)) ;
#26550=CARTESIAN_POINT('Ctrl Pts',(-18.8611603269011,4.64829974240889,-323.663110816821)) ;
#26551=CARTESIAN_POINT('Ctrl Pts',(-18.9423153746605,4.30852434499854,-323.65870269278)) ;
#26552=CARTESIAN_POINT('Ctrl Pts',(-18.9877710768902,4.10356473473042,-323.656072847981)) ;
#26553=CARTESIAN_POINT('Ctrl Pts',(-19.0563773488577,3.76862351583381,-323.651824633378)) ;
#26554=CARTESIAN_POINT('Ctrl Pts',(-19.0815407143368,3.63907198188087,-323.650193380017)) ;
#26555=CARTESIAN_POINT('Ctrl Pts',(-19.1282676049678,3.38467888108712,-323.647013177503)) ;
#26556=CARTESIAN_POINT('Ctrl Pts',(-19.1499338733852,3.2598627868882,-323.645463624505)) ;
#26557=CARTESIAN_POINT('Ctrl Pts',(-19.2005335405463,2.95043276379485,-323.641647721112)) ;
#26558=CARTESIAN_POINT('Ctrl Pts',(-19.228026923018,2.76559623389185,-323.639390818261)) ;
#26559=CARTESIAN_POINT('Ctrl Pts',(-19.3003523500571,2.22596088937323,-323.632859614584)) ;
#26560=CARTESIAN_POINT('Ctrl Pts',(-19.3380592406342,1.87028559468797,-323.628628607325)) ;
#26561=CARTESIAN_POINT('Ctrl Pts',(-19.409703432285,0.953730138556838,-323.61783122505)) ;
#26562=CARTESIAN_POINT('Ctrl Pts',(-19.4291657242124,0.392053781323674,
-323.61132066603)) ;
#26563=CARTESIAN_POINT('Ctrl Pts',(-19.4231189534842,-0.300180780468465,
-323.603163308272)) ;
#26564=CARTESIAN_POINT('Ctrl Pts',(-19.4206637161338,-0.430672913210518,
-323.601619289569)) ;
#26565=CARTESIAN_POINT('Ctrl Pts',(-19.4121373626804,-0.72571188962875,
-323.598106246829)) ;
#26566=CARTESIAN_POINT('Ctrl Pts',(-19.4052887613691,-0.890226192792095,
-323.596131857322)) ;
#26567=CARTESIAN_POINT('Ctrl Pts',(-19.392084821417,-1.13306723477477,-323.593183337395)) ;
#26568=CARTESIAN_POINT('Ctrl Pts',(-19.3873444389983,-1.21147458190062,
-323.592226064955)) ;
#26569=CARTESIAN_POINT('Ctrl Pts',(-19.3777034784967,-1.35634584573807,
-323.590445978822)) ;
#26570=CARTESIAN_POINT('Ctrl Pts',(-19.3729362000099,-1.42281731370898,
-323.589624648043)) ;
#26571=CARTESIAN_POINT('Ctrl Pts',(-19.3601814528439,-1.5886924852847,-323.58756436198)) ;
#26572=CARTESIAN_POINT('Ctrl Pts',(-19.3517703978409,-1.68806164873633,
-323.586320642559)) ;
#26573=CARTESIAN_POINT('Ctrl Pts',(-19.3109055945624,-2.13029524959461,
-323.580749921347)) ;
#26574=CARTESIAN_POINT('Ctrl Pts',(-19.2701022439277,-2.472325105742,-323.576346942396)) ;
#26575=CARTESIAN_POINT('Ctrl Pts',(-19.137644587618,-3.37733276370464,-323.564584168215)) ;
#26576=CARTESIAN_POINT('Ctrl Pts',(-19.0302544704618,-3.93766857669095,
-323.557191003107)) ;
#26577=CARTESIAN_POINT('Ctrl Pts',(-18.8611536591895,-4.64902164722299,
-323.547853577139)) ;
#26578=CARTESIAN_POINT('Ctrl Pts',(-18.8219937848632,-4.80510870572095,
-323.545807051461)) ;
#26579=CARTESIAN_POINT('Ctrl Pts',(-18.7217748465601,-5.18453198790289,
-323.540841931866)) ;
#26580=CARTESIAN_POINT('Ctrl Pts',(-18.658653576193,-5.40729806358084,-323.537935197315)) ;
#26581=CARTESIAN_POINT('Ctrl Pts',(-18.5521989494274,-5.75890569536453,
-323.533363931289)) ;
#26582=CARTESIAN_POINT('Ctrl Pts',(-18.5114695706259,-5.88851212651266,
-323.531682480159)) ;
#26583=CARTESIAN_POINT('Ctrl Pts',(-18.4303192367839,-6.13757762864983,
-323.528457903134)) ;
#26584=CARTESIAN_POINT('Ctrl Pts',(-18.3900879269123,-6.25709136951226,
-323.526913584495)) ;
#26585=CARTESIAN_POINT('Ctrl Pts',(-18.2912709921966,-6.5414551680368,-323.52324533772)) ;
#26586=CARTESIAN_POINT('Ctrl Pts',(-18.2316164370514,-6.70592219155419,
-323.521128808011)) ;
#26587=CARTESIAN_POINT('Ctrl Pts',(-17.8615467149122,-7.68474363911383,
-323.508550855591)) ;
#26588=CARTESIAN_POINT('Ctrl Pts',(-17.4988365365402,-8.47825756652103,
-323.498482177846)) ;
#26589=CARTESIAN_POINT('Ctrl Pts',(-16.9783588271972,-9.44008994187764,
-323.485646558628)) ;
#26590=CARTESIAN_POINT('Ctrl Pts',(-16.8692999707021,-9.63362262312248,
-323.483026867081)) ;
#26591=CARTESIAN_POINT('Ctrl Pts',(-16.6791509620289,-9.9579216801876,-323.478545482386)) ;
#26592=CARTESIAN_POINT('Ctrl Pts',(-16.5997827615458,-10.0896725987044,
-323.476698594713)) ;
#26593=CARTESIAN_POINT('Ctrl Pts',(-16.4785276852816,-10.2856514586877,
-323.473902421987)) ;
#26594=CARTESIAN_POINT('Ctrl Pts',(-16.4378115151813,-10.3505967545955,
-323.472967621136)) ;
#26595=CARTESIAN_POINT('Ctrl Pts',(-16.3610693846082,-10.4714112008615,
-323.471211808896)) ;
#26596=CARTESIAN_POINT('Ctrl Pts',(-16.3251390349912,-10.5273396162912,
-323.470392048358)) ;
#26597=CARTESIAN_POINT('Ctrl Pts',(-16.2327475477995,-10.6695437209957,
-323.468290817608)) ;
#26598=CARTESIAN_POINT('Ctrl Pts',(-16.1758852825917,-10.7555563057642,
-323.467003982076)) ;
#26599=CARTESIAN_POINT('Ctrl Pts',(-15.9800496913339,-11.0467206105465,
-323.462599038316)) ;
#26600=CARTESIAN_POINT('Ctrl Pts',(-15.8378370685598,-11.2496640395573,
-323.459445708451)) ;
#26601=CARTESIAN_POINT('Ctrl Pts',(-15.1492639469477,-12.1933407660628,
-323.444481118247)) ;
#26602=CARTESIAN_POINT('Ctrl Pts',(-14.554583351921,-12.8973593787649,-323.432482732829)) ;
#26603=CARTESIAN_POINT('Ctrl Pts',(-13.7857370178849,-13.6863777352626,
-323.418638470101)) ;
#26604=CARTESIAN_POINT('Ctrl Pts',(-13.6574251855423,-13.81442065674,-323.416375570281)) ;
#26605=CARTESIAN_POINT('Ctrl Pts',(-13.4361608112116,-14.02912503643,-323.412553926382)) ;
#26606=CARTESIAN_POINT('Ctrl Pts',(-13.3441157417402,-14.1167043517115,
-323.410987064035)) ;
#26607=CARTESIAN_POINT('Ctrl Pts',(-13.1533962175897,-14.2946385471667,
-323.407786699666)) ;
#26608=CARTESIAN_POINT('Ctrl Pts',(-13.0546340901228,-14.3848897139084,
-323.406154156418)) ;
#26609=CARTESIAN_POINT('Ctrl Pts',(-12.7910127909742,-14.6208419937983,
-323.401859683262)) ;
#26610=CARTESIAN_POINT('Ctrl Pts',(-12.6245970202311,-14.7647749434726,
-323.399212892351)) ;
#26611=CARTESIAN_POINT('Ctrl Pts',(-12.2459747382249,-15.0811629940521,
-323.39332195572)) ;
#26612=CARTESIAN_POINT('Ctrl Pts',(-12.0324993525569,-15.2520272154325,
-323.390089569789)) ;
#26613=CARTESIAN_POINT('Ctrl Pts',(-11.3581347485751,-15.7688113265417,
-323.380103799924)) ;
#26614=CARTESIAN_POINT('Ctrl Pts',(-10.8854138524811,-16.0987701141266,
-323.37342807247)) ;
#26615=CARTESIAN_POINT('Ctrl Pts',(-10.2871542479516,-16.4779407566661,
-323.365083574892)) ;
#26616=CARTESIAN_POINT('Ctrl Pts',(-10.1748625083327,-16.5475148281444,
-323.363521179059)) ;
#26617=CARTESIAN_POINT('Ctrl Pts',(-9.99331188975665,-16.6574537742026,
-323.360995506104)) ;
#26618=CARTESIAN_POINT('Ctrl Pts',(-9.9244975549191,-16.6985447579445,-323.360038262407)) ;
#26619=CARTESIAN_POINT('Ctrl Pts',(-9.75438705056792,-16.7986995717895,
-323.357670028279)) ;
#26620=CARTESIAN_POINT('Ctrl Pts',(-9.65280668031727,-16.8572743101659,
-323.356254208695)) ;
#26621=CARTESIAN_POINT('Ctrl Pts',(-9.4900543498643,-16.949169426556,-323.353978685847)) ;
#26622=CARTESIAN_POINT('Ctrl Pts',(-9.4292226447491,-16.9830867667616,-323.353126598324)) ;
#26623=CARTESIAN_POINT('Ctrl Pts',(-9.31295212156922,-17.0470973083787,
-323.351493826643)) ;
#26624=CARTESIAN_POINT('Ctrl Pts',(-9.25754657869402,-17.0772490522363,
-323.350714046218)) ;
#26625=CARTESIAN_POINT('Ctrl Pts',(-9.09742170144324,-17.1633808768052,
-323.348456597574)) ;
#26626=CARTESIAN_POINT('Ctrl Pts',(-8.99233473141471,-17.2186712830012,
-323.346970375143)) ;
#26627=CARTESIAN_POINT('Ctrl Pts',(-8.49628707071214,-17.4738818263802,
-323.339944465932)) ;
#26628=CARTESIAN_POINT('Ctrl Pts',(-8.09912762548097,-17.6614713642143,
-323.334291916759)) ;
#26629=CARTESIAN_POINT('Ctrl Pts',(-7.25661199318999,-18.0250150484085,
-323.322456552779)) ;
#26630=CARTESIAN_POINT('Ctrl Pts',(-6.81041448258537,-18.1982922578074,
-323.316276734357)) ;
#26631=CARTESIAN_POINT('Ctrl Pts',(-6.21977718436647,-18.4028932538056,
-323.308311131244)) ;
#26632=CARTESIAN_POINT('Ctrl Pts',(-6.08074092390645,-18.4493007513255,
-323.306450830368)) ;
#26633=CARTESIAN_POINT('Ctrl Pts',(-5.7343191259791,-18.5605878798342,-323.301855104929)) ;
#26634=CARTESIAN_POINT('Ctrl Pts',(-5.52634483295248,-18.623569778894,-323.299130920621)) ;
#26635=CARTESIAN_POINT('Ctrl Pts',(-5.18915502957829,-18.7195369145831,
-323.294772535929)) ;
#26636=CARTESIAN_POINT('Ctrl Pts',(-5.06058028526859,-18.7547039286553,
-323.293124121493)) ;
#26637=CARTESIAN_POINT('Ctrl Pts',(-4.80990127159673,-18.8205026423085,
-323.289936139191)) ;
#26638=CARTESIAN_POINT('Ctrl Pts',(-4.68784101703242,-18.8512762591514,
-323.288395691329)) ;
#26639=CARTESIAN_POINT('Ctrl Pts',(-4.41711430663743,-18.9167393818612,
-323.28500422521)) ;
#26640=CARTESIAN_POINT('Ctrl Pts',(-4.26832054143699,-18.950867195877,-323.283156978403)) ;
#26641=CARTESIAN_POINT('Ctrl Pts',(-3.64749333363458,-19.0855794166643,
-323.275513482985)) ;
#26642=CARTESIAN_POINT('Ctrl Pts',(-3.17219600264366,-19.1703083756524,
-323.26981953233)) ;
#26643=CARTESIAN_POINT('Ctrl Pts',(-2.5943557281925,-19.2512367216642,-323.262986970316)) ;
#26644=CARTESIAN_POINT('Ctrl Pts',(-2.49436698198753,-19.2644473142325,
-323.261807687158)) ;
#26645=CARTESIAN_POINT('Ctrl Pts',(-1.97755099516221,-19.3286383146348,
-323.255722233387)) ;
#26646=CARTESIAN_POINT('Ctrl Pts',(-1.55925382385643,-19.3668710345487,
-323.250832730254)) ;
#26647=CARTESIAN_POINT('Ctrl Pts',(-0.913545351985959,-19.4048329170795,
-323.243188570478)) ;
#26648=CARTESIAN_POINT('Ctrl Pts',(-0.68682738132068,-19.4141797007271,
-323.240485793241)) ;
#26649=CARTESIAN_POINT('Ctrl Pts',(-0.372335173539643,-19.4216291966745,
-323.236683945311)) ;
#26650=CARTESIAN_POINT('Ctrl Pts',(-0.284659071174872,-19.4231120915325,
-323.235618343446)) ;
#26651=CARTESIAN_POINT('Ctrl Pts',(-0.131326814215122,-19.4246670120776,
-323.233742695222)) ;
#26652=CARTESIAN_POINT('Ctrl Pts',(-0.0656749078580174,-19.4249999242354,
-323.232935613241)) ;
#26653=CARTESIAN_POINT('Ctrl Pts',(-2.2413097626006E-5,-19.4249999999871,
-323.232124485186)) ;
#26654=CARTESIAN_POINT('Ctrl Pts',(0.000132646322085553,-19.4249999995471,
-323.01792308454)) ;
#26655=CARTESIAN_POINT('Ctrl Pts',(-0.143386424633033,-19.4250009795871,
-323.019721098121)) ;
#26656=CARTESIAN_POINT('Ctrl Pts',(-0.286900965316344,-19.4234114015544,
-323.021534137457)) ;
#26657=CARTESIAN_POINT('Ctrl Pts',(-0.892780897527133,-19.4099840984498,
-323.029234622781)) ;
#26658=CARTESIAN_POINT('Ctrl Pts',(-1.35466350679508,-19.383225395553,-323.035215324363)) ;
#26659=CARTESIAN_POINT('Ctrl Pts',(-2.21603517801831,-19.3023816737848,
-323.046374478159)) ;
#26660=CARTESIAN_POINT('Ctrl Pts',(-2.61565493465555,-19.2523011719939,
-323.051554477303)) ;
#26661=CARTESIAN_POINT('Ctrl Pts',(-3.20887809445812,-19.1591458208909,
-323.059188247264)) ;
#26662=CARTESIAN_POINT('Ctrl Pts',(-3.403846742271,-19.1254697911577,-323.061688538205)) ;
#26663=CARTESIAN_POINT('Ctrl Pts',(-3.72974769344513,-19.0640370476888,
-323.065849842204)) ;
#26664=CARTESIAN_POINT('Ctrl Pts',(-3.86096882826084,-19.0378950038165,
-323.067520446422)) ;
#26665=CARTESIAN_POINT('Ctrl Pts',(-4.1055476061043,-18.9865369903663,-323.070624669101)) ;
#26666=CARTESIAN_POINT('Ctrl Pts',(-4.21896954152059,-18.9616561533648,
-323.072060375519)) ;
#26667=CARTESIAN_POINT('Ctrl Pts',(-4.45544312413976,-18.9075552462617,
-323.075045806443)) ;
#26668=CARTESIAN_POINT('Ctrl Pts',(-4.57844631081098,-18.8781473733737,
-323.076594211844)) ;
#26669=CARTESIAN_POINT('Ctrl Pts',(-4.873327380895,-18.8045950062122,-323.080296453797)) ;
#26670=CARTESIAN_POINT('Ctrl Pts',(-5.0449047280323,-18.7592923512697,-323.082442502117)) ;
#26671=CARTESIAN_POINT('Ctrl Pts',(-5.92843454562076,-18.5130100050128,
-323.093462328778)) ;
#26672=CARTESIAN_POINT('Ctrl Pts',(-6.62910384577733,-18.273829870117,-323.102070183016)) ;
#26673=CARTESIAN_POINT('Ctrl Pts',(-7.59162490930686,-17.8826003263373,
-323.114216110483)) ;
#26674=CARTESIAN_POINT('Ctrl Pts',(-7.8661894456942,-17.7635364260414,-323.117722856702)) ;
#26675=CARTESIAN_POINT('Ctrl Pts',(-8.25753035144572,-17.5829797630774,
-323.122837994371)) ;
#26676=CARTESIAN_POINT('Ctrl Pts',(-8.37660260771509,-17.5265659368768,
-323.124410372325)) ;
#26677=CARTESIAN_POINT('Ctrl Pts',(-8.56740842014738,-17.4337776870325,
-323.126961997382)) ;
#26678=CARTESIAN_POINT('Ctrl Pts',(-8.63950615788171,-17.3981615352633,
-323.127933593836)) ;
#26679=CARTESIAN_POINT('Ctrl Pts',(-8.72039468690472,-17.3575759601992,
-323.129033079265)) ;
#26680=CARTESIAN_POINT('Ctrl Pts',(-8.72940525285799,-17.3530461487548,
-323.129155688443)) ;
#26681=CARTESIAN_POINT('Ctrl Pts',(-8.74650660093109,-17.3444322311362,
-323.129388645558)) ;
#26682=CARTESIAN_POINT('Ctrl Pts',(-8.75459806064397,-17.3403494756347,
-323.129498976926)) ;
#26683=CARTESIAN_POINT('Ctrl Pts',(-8.7706232512677,-17.3322494750861,-323.129717706229)) ;
#26684=CARTESIAN_POINT('Ctrl Pts',(-8.77855708681536,-17.3282324417637,
-323.129826101507)) ;
#26685=CARTESIAN_POINT('Ctrl Pts',(-8.79537798527605,-17.3197012229957,
-323.130056142232)) ;
#26686=CARTESIAN_POINT('Ctrl Pts',(-8.80426433755254,-17.3151856424404,
-323.130177805386)) ;
#26687=CARTESIAN_POINT('Ctrl Pts',(-8.86959167477885,-17.2819264060786,
-323.13107320469)) ;
#26688=CARTESIAN_POINT('Ctrl Pts',(-8.92589517362289,-17.2529137288977,
-323.131850483198)) ;
#26689=CARTESIAN_POINT('Ctrl Pts',(-9.05279843305058,-17.1867341591782,
-323.133615584406)) ;
#26690=CARTESIAN_POINT('Ctrl Pts',(-9.12331297511337,-17.1494067204736,
-323.134605446849)) ;
#26691=CARTESIAN_POINT('Ctrl Pts',(-9.33344809044489,-17.036507163536,-323.137580153682)) ;
#26692=CARTESIAN_POINT('Ctrl Pts',(-9.47237412502849,-16.9596567740692,
-323.139579849131)) ;
#26693=CARTESIAN_POINT('Ctrl Pts',(-10.1570596056975,-16.569868368094,-323.149572018442)) ;
#26694=CARTESIAN_POINT('Ctrl Pts',(-10.6883341102687,-16.232249143419,-323.157748498575)) ;
#26695=CARTESIAN_POINT('Ctrl Pts',(-11.4636366688155,-15.6849608839045,
-323.169954118049)) ;
#26696=CARTESIAN_POINT('Ctrl Pts',(-11.7203885274914,-15.4940458542533,
-323.174047239196)) ;
#26697=CARTESIAN_POINT('Ctrl Pts',(-12.1098852388484,-15.1892009672042,
-323.18031153823)) ;
#26698=CARTESIAN_POINT('Ctrl Pts',(-12.2460031514858,-15.0796735194339,
-323.182511743866)) ;
#26699=CARTESIAN_POINT('Ctrl Pts',(-12.4775701246374,-14.8881394669293,
-323.186271927244)) ;
#26700=CARTESIAN_POINT('Ctrl Pts',(-12.5737338567238,-14.8070142145534,
-323.1878386812)) ;
#26701=CARTESIAN_POINT('Ctrl Pts',(-12.713759455592,-14.6865385970889,-323.190127695147)) ;
#26702=CARTESIAN_POINT('Ctrl Pts',(-12.7582411459618,-14.6479137874618,
-323.190855996472)) ;
#26703=CARTESIAN_POINT('Ctrl Pts',(-12.8959578814861,-14.5272269246428,
-323.193114482445)) ;
#26704=CARTESIAN_POINT('Ctrl Pts',(-12.988582089848,-14.444472546375,-323.194638684284)) ;
#26705=CARTESIAN_POINT('Ctrl Pts',(-13.1973025715893,-14.2543618308937,
-323.198086021243)) ;
#26706=CARTESIAN_POINT('Ctrl Pts',(-13.3128945278941,-14.146464779333,-323.200004296898)) ;
#26707=CARTESIAN_POINT('Ctrl Pts',(-13.6826711172453,-13.7927575400755,
-323.206174862732)) ;
#26708=CARTESIAN_POINT('Ctrl Pts',(-13.9314651080532,-13.5414153676737,
-323.210378580259)) ;
#26709=CARTESIAN_POINT('Ctrl Pts',(-14.3477302531199,-13.0972652068633,
-323.217551605327)) ;
#26710=CARTESIAN_POINT('Ctrl Pts',(-14.518515690468,-12.9076884681071,-323.220538395394)) ;
#26711=CARTESIAN_POINT('Ctrl Pts',(-15.0718096362092,-12.2686374358373,
-323.230416289805)) ;
#26712=CARTESIAN_POINT('Ctrl Pts',(-15.4375674512257,-11.8051013117611,
-323.237270876837)) ;
#26713=CARTESIAN_POINT('Ctrl Pts',(-15.8496772546526,-11.2308489446518,
-323.245751564206)) ;
#26714=CARTESIAN_POINT('Ctrl Pts',(-15.9168461291785,-11.1354499835129,
-323.247160461846)) ;
#26715=CARTESIAN_POINT('Ctrl Pts',(-16.0226687870724,-10.9822377054587,
-323.24942763978)) ;
#26716=CARTESIAN_POINT('Ctrl Pts',(-16.0618786815928,-10.9248118197246,
-323.250278401492)) ;
#26717=CARTESIAN_POINT('Ctrl Pts',(-16.1361270207473,-10.8148056821631,
-323.251911177553)) ;
#26718=CARTESIAN_POINT('Ctrl Pts',(-16.171218900861,-10.7622626069916,-323.252692311706)) ;
#26719=CARTESIAN_POINT('Ctrl Pts',(-16.271846793337,-10.6099890620111,-323.254958586621)) ;
#26720=CARTESIAN_POINT('Ctrl Pts',(-16.3367208932937,-10.5098247536915,
-323.256452381128)) ;
#26721=CARTESIAN_POINT('Ctrl Pts',(-16.6354949905299,-10.0390723121715,
-323.263475450053)) ;
#26722=CARTESIAN_POINT('Ctrl Pts',(-16.8577340450092,-9.66123534115661,
-323.269116717026)) ;
#26723=CARTESIAN_POINT('Ctrl Pts',(-17.29544083861,-8.85591229306789,-323.280938996491)) ;
#26724=CARTESIAN_POINT('Ctrl Pts',(-17.5082752987824,-8.42732186496238,
-323.287117038402)) ;
#26725=CARTESIAN_POINT('Ctrl Pts',(-17.7653603303499,-7.85773973904837,
-323.2950805989)) ;
#26726=CARTESIAN_POINT('Ctrl Pts',(-17.8241359323304,-7.72348883613966,
-323.296940596201)) ;
#26727=CARTESIAN_POINT('Ctrl Pts',(-17.9662626870975,-7.3885880259425,-323.30153571232)) ;
#26728=CARTESIAN_POINT('Ctrl Pts',(-18.0477773443667,-7.18718033204947,
-323.304259592017)) ;
#26729=CARTESIAN_POINT('Ctrl Pts',(-18.1738218749033,-6.86007212346064,
-323.308617621235)) ;
#26730=CARTESIAN_POINT('Ctrl Pts',(-18.2204660110835,-6.73520671371519,
-323.310265980438)) ;
#26731=CARTESIAN_POINT('Ctrl Pts',(-18.3086550532496,-6.49150373083635,
-323.313453935068)) ;
#26732=CARTESIAN_POINT('Ctrl Pts',(-18.3503371909897,-6.37272277535232,
-323.314994409628)) ;
#26733=CARTESIAN_POINT('Ctrl Pts',(-18.44939668465,-6.08140169775523,-323.318741096068)) ;
#26734=CARTESIAN_POINT('Ctrl Pts',(-18.5055117099719,-5.90844489898369,
-323.32093867402)) ;
#26735=CARTESIAN_POINT('Ctrl Pts',(-18.7660168079652,-5.06537689677788,
-323.331532370737)) ;
#26736=CARTESIAN_POINT('Ctrl Pts',(-18.9364813393758,-4.38532840550178,
-323.339696610419)) ;
#26737=CARTESIAN_POINT('Ctrl Pts',(-19.1516948471729,-3.27538460645364,
-323.352907442427)) ;
#26738=CARTESIAN_POINT('Ctrl Pts',(-19.2195110323268,-2.85060586610566,
-323.357942311224)) ;
#26739=CARTESIAN_POINT('Ctrl Pts',(-19.2883953883009,-2.3028916600985,-323.364558645826)) ;
#26740=CARTESIAN_POINT('Ctrl Pts',(-19.3024772982789,-2.1817141738926,-323.366030422663)) ;
#26741=CARTESIAN_POINT('Ctrl Pts',(-19.32290299794,-1.99023263802887,-323.368373631185)) ;
#26742=CARTESIAN_POINT('Ctrl Pts',(-19.3300066506805,-1.92001278487359,
-323.369236649854)) ;
#26743=CARTESIAN_POINT('Ctrl Pts',(-19.3426617857914,-1.78772024384861,
-323.37087076424)) ;
#26744=CARTESIAN_POINT('Ctrl Pts',(-19.3482975541984,-1.7256565049681,-323.371640777361)) ;
#26745=CARTESIAN_POINT('Ctrl Pts',(-19.3634319781995,-1.54958535661214,
-323.373833784115)) ;
#26746=CARTESIAN_POINT('Ctrl Pts',(-19.3722222731532,-1.43551972988006,
-323.375264615431)) ;
#26747=CARTESIAN_POINT('Ctrl Pts',(-19.4236591336926,-0.681123474079131,
-323.384779930384)) ;
#26748=CARTESIAN_POINT('Ctrl Pts',(-19.4355585149201,-0.0390939553886075,
-323.393112368081)) ;
#26749=CARTESIAN_POINT('Ctrl Pts',(-19.4045562047933,0.960219865977938,
-323.40599348878)) ;
#26750=CARTESIAN_POINT('Ctrl Pts',(-19.3835609533153,1.31772121561742,-323.410587095107)) ;
#26751=CARTESIAN_POINT('Ctrl Pts',(-19.3303837156406,1.93232920996966,-323.418415075141)) ;
#26752=CARTESIAN_POINT('Ctrl Pts',(-19.3029176722244,2.18974895868517,-323.421673040308)) ;
#26753=CARTESIAN_POINT('Ctrl Pts',(-19.2526030924553,2.58605417937906,-323.426651323357)) ;
#26754=CARTESIAN_POINT('Ctrl Pts',(-19.2333763714757,2.72536886953968,-323.428394268476)) ;
#26755=CARTESIAN_POINT('Ctrl Pts',(-19.1942435908834,2.98784182698217,-323.431664770204)) ;
#26756=CARTESIAN_POINT('Ctrl Pts',(-19.1746606018074,3.11104108970512,-323.433194344231)) ;
#26757=CARTESIAN_POINT('Ctrl Pts',(-19.1270270339797,3.39315488800447,-323.436685015405)) ;
#26758=CARTESIAN_POINT('Ctrl Pts',(-19.0981802034418,3.55192571237075,-323.438640809748)) ;
#26759=CARTESIAN_POINT('Ctrl Pts',(-18.9853611507544,4.13170374116557,-323.445756059982)) ;
#26760=CARTESIAN_POINT('Ctrl Pts',(-18.8894174812303,4.55025518098348,-323.450838260009)) ;
#26761=CARTESIAN_POINT('Ctrl Pts',(-18.6392171875696,5.49656215316194,-323.462327161267)) ;
#26762=CARTESIAN_POINT('Ctrl Pts',(-18.4762677729012,6.0216393554429,-323.468698120952)) ;
#26763=CARTESIAN_POINT('Ctrl Pts',(-18.247806316017,6.66069553474473,-323.476696830969)) ;
#26764=CARTESIAN_POINT('Ctrl Pts',(-18.2031244281092,6.78185530371852,-323.47822483961)) ;
#26765=CARTESIAN_POINT('Ctrl Pts',(-18.0991443561076,7.05537567603066,-323.481708164781)) ;
#26766=CARTESIAN_POINT('Ctrl Pts',(-18.0391241018999,7.20745127241923,-323.48366886308)) ;
#26767=CARTESIAN_POINT('Ctrl Pts',(-17.9475099913573,7.4312615961913,-323.486601067615)) ;
#26768=CARTESIAN_POINT('Ctrl Pts',(-17.9173901477882,7.50359207795672,-323.487555978367)) ;
#26769=CARTESIAN_POINT('Ctrl Pts',(-17.8608219159182,7.63715352240042,-323.489334396038)) ;
#26770=CARTESIAN_POINT('Ctrl Pts',(-17.8344942318668,7.69843418456466,-323.490156454413)) ;
#26771=CARTESIAN_POINT('Ctrl Pts',(-17.7678566609664,7.85136414646085,-323.492222479649)) ;
#26772=CARTESIAN_POINT('Ctrl Pts',(-17.7271528389148,7.94283963524125,-323.493471271692)) ;
#26773=CARTESIAN_POINT('Ctrl Pts',(-17.5304216763139,8.37591637697794,-323.499438296061)) ;
#26774=CARTESIAN_POINT('Ctrl Pts',(-17.3652169912488,8.71325984865016,-323.504247640434)) ;
#26775=CARTESIAN_POINT('Ctrl Pts',(-16.9938018453592,9.41910038404857,-323.514515425724)) ;
#26776=CARTESIAN_POINT('Ctrl Pts',(-16.7851448551763,9.78609553769101,-323.519977023167)) ;
#26777=CARTESIAN_POINT('Ctrl Pts',(-16.4137775995368,10.3924020520023,-323.529103359175)) ;
#26778=CARTESIAN_POINT('Ctrl Pts',(-16.2573764524252,10.6354044033376,-323.532791125172)) ;
#26779=CARTESIAN_POINT('Ctrl Pts',(-15.9696948736269,11.0611961013223,-323.539287580104)) ;
#26780=CARTESIAN_POINT('Ctrl Pts',(-15.8405494446539,11.2453638048455,-323.542109648654)) ;
#26781=CARTESIAN_POINT('Ctrl Pts',(-15.6290127539202,11.5361484432598,-323.546582257078)) ;
#26782=CARTESIAN_POINT('Ctrl Pts',(-15.5486602988448,11.6442227536989,-323.548248440002)) ;
#26783=CARTESIAN_POINT('Ctrl Pts',(-15.3905966080659,11.8522652181337,-323.551463650068)) ;
#26784=CARTESIAN_POINT('Ctrl Pts',(-15.3130189126214,11.9523264088609,-323.553013646823)) ;
#26785=CARTESIAN_POINT('Ctrl Pts',(-15.1237890434908,12.1915320905379,-323.556728773702)) ;
#26786=CARTESIAN_POINT('Ctrl Pts',(-15.0111874100405,12.3299108843271,-323.55888596738)) ;
#26787=CARTESIAN_POINT('Ctrl Pts',(-14.4253167372631,13.0299777560931,-323.569851873545)) ;
#26788=CARTESIAN_POINT('Ctrl Pts',(-13.9223705892237,13.566048829545,-323.578399615859)) ;
#26789=CARTESIAN_POINT('Ctrl Pts',(-13.0945376844315,14.3537578057832,-323.591757265473)) ;
#26790=CARTESIAN_POINT('Ctrl Pts',(-12.7899972030179,14.625773496284,-323.596543579263)) ;
#26791=CARTESIAN_POINT('Ctrl Pts',(-12.3854347032698,14.9648234389019,-323.602873089819)) ;
#26792=CARTESIAN_POINT('Ctrl Pts',(-12.2930480739379,15.0408079016813,-323.60431682358)) ;
#26793=CARTESIAN_POINT('Ctrl Pts',(-12.1454093999765,15.1599660522091,-323.606626065588)) ;
#26794=CARTESIAN_POINT('Ctrl Pts',(-12.090615197618,15.2037023232426,-323.607483563056)) ;
#26795=CARTESIAN_POINT('Ctrl Pts',(-11.9863866292015,15.2859768849173,-323.609116715607)) ;
#26796=CARTESIAN_POINT('Ctrl Pts',(-11.9370001648602,15.3245744085783,-323.609891375306)) ;
#26797=CARTESIAN_POINT('Ctrl Pts',(-11.7953043855647,15.4342148290028,-323.612115224577)) ;
#26798=CARTESIAN_POINT('Ctrl Pts',(-11.7025417703818,15.5046673292005,-323.613572592589)) ;
#26799=CARTESIAN_POINT('Ctrl Pts',(-11.3240513924708,15.7867960512071,-323.61951556186)) ;
#26800=CARTESIAN_POINT('Ctrl Pts',(-11.033170284997,15.9914421550908,-323.624073979175)) ;
#26801=CARTESIAN_POINT('Ctrl Pts',(-10.2880324070921,16.485661935317,-323.63558847017)) ;
#26802=CARTESIAN_POINT('Ctrl Pts',(-9.82704166035124,16.7645433664448,-323.642561898039)) ;
#26803=CARTESIAN_POINT('Ctrl Pts',(-9.21806634349993,17.0991904042027,-323.651429917981)) ;
#26804=CARTESIAN_POINT('Ctrl Pts',(-9.08016877566304,17.1728155720452,-323.653416670403)) ;
#26805=CARTESIAN_POINT('Ctrl Pts',(-8.73985357585639,17.3492687095376,-323.658264184836)) ;
#26806=CARTESIAN_POINT('Ctrl Pts',(-8.53649293002245,17.4502279070833,-323.66111326938)) ;
#26807=CARTESIAN_POINT('Ctrl Pts',(-8.20941454368964,17.605521164429,-323.665617375329)) ;
#26808=CARTESIAN_POINT('Ctrl Pts',(-8.08681909811009,17.6621691633769,-323.667288443016)) ;
#26809=CARTESIAN_POINT('Ctrl Pts',(-7.84832005389831,17.7693692500818,-323.6705065373)) ;
#26810=CARTESIAN_POINT('Ctrl Pts',(-7.73249386650602,17.820077156609,-323.672054605962)) ;
#26811=CARTESIAN_POINT('Ctrl Pts',(-7.45312609622506,17.9391458215196,-323.675754098106)) ;
#26812=CARTESIAN_POINT('Ctrl Pts',(-7.2891277173627,18.0064060450117,-323.677897764949)) ;
#26813=CARTESIAN_POINT('Ctrl Pts',(-6.43491789120533,18.343158289268,-323.688929736911)) ;
#26814=CARTESIAN_POINT('Ctrl Pts',(-5.73061961604093,18.5752422166151,-323.697551008809)) ;
#26815=CARTESIAN_POINT('Ctrl Pts',(-4.62345263128522,18.8710993944514,-323.710948207612)) ;
#26816=CARTESIAN_POINT('Ctrl Pts',(-4.22893946590713,18.9634062371226,-323.715698412016)) ;
#26817=CARTESIAN_POINT('Ctrl Pts',(-3.7149116230149,19.0668371837529,-323.721986168133)) ;
#26818=CARTESIAN_POINT('Ctrl Pts',(-3.59777842990869,19.0892859705462,-323.723425706394)) ;
#26819=CARTESIAN_POINT('Ctrl Pts',(-3.41154072054601,19.1232037154467,-323.725729874141)) ;
#26820=CARTESIAN_POINT('Ctrl Pts',(-3.3425679997651,19.135380048266,-323.726586552559)) ;
#26821=CARTESIAN_POINT('Ctrl Pts',(-3.21169119646415,19.1577556251621,-323.728219609246)) ;
#26822=CARTESIAN_POINT('Ctrl Pts',(-3.14980061866052,19.1680285106877,-323.728995005584)) ;
#26823=CARTESIAN_POINT('Ctrl Pts',(-2.97253816018169,19.1965696445581,-323.731223710988)) ;
#26824=CARTESIAN_POINT('Ctrl Pts',(-2.85704988817862,19.214097301432,-323.732685252504)) ;
#26825=CARTESIAN_POINT('Ctrl Pts',(-2.08286541049713,19.3244609707748,-323.742530722904)) ;
#26826=CARTESIAN_POINT('Ctrl Pts',(-1.41993272885781,19.38445024856,-323.75117690688)) ;
#26827=CARTESIAN_POINT('Ctrl Pts',(-0.41326624759806,19.4236184554067,-323.764148208138)) ;
#26828=CARTESIAN_POINT('Ctrl Pts',(-0.0710077632526839,19.4278846366049,
-323.768534071267)) ;
#26829=CARTESIAN_POINT('Ctrl Pts',(0.522687238255438,19.419595486858,-323.776062670934)) ;
#26830=CARTESIAN_POINT('Ctrl Pts',(0.774098068005405,19.4111994314001,-323.779226415267)) ;
#26831=CARTESIAN_POINT('Ctrl Pts',(1.16445555781883,19.3905671281626,-323.784095932084)) ;
#26832=CARTESIAN_POINT('Ctrl Pts',(1.30355284956452,19.3817130391547,-323.78582273479)) ;
#26833=CARTESIAN_POINT('Ctrl Pts',(1.56721041596976,19.362079038365,-323.789080152039)) ;
#26834=CARTESIAN_POINT('Ctrl Pts',(1.69178548551039,19.3515920558029,-323.79061257634)) ;
#26835=CARTESIAN_POINT('Ctrl Pts',(1.97923801521736,19.3245967881544,-323.794134017637)) ;
#26836=CARTESIAN_POINT('Ctrl Pts',(2.14202542972823,19.3072305446627,-323.796117388452)) ;
#26837=CARTESIAN_POINT('Ctrl Pts',(2.73838514779966,19.2359754257731,-323.803349105952)) ;
#26838=CARTESIAN_POINT('Ctrl Pts',(3.17032460713276,19.1695213001071,-323.808517517856)) ;
#26839=CARTESIAN_POINT('Ctrl Pts',(4.12898455655346,18.9887404643677,-323.819962149067)) ;
#26840=CARTESIAN_POINT('Ctrl Pts',(4.65393141807666,18.8669472566369,-323.82620882754)) ;
#26841=CARTESIAN_POINT('Ctrl Pts',(5.29639084717439,18.6894414181096,-323.834065921175)) ;
#26842=CARTESIAN_POINT('Ctrl Pts',(5.41930664523481,18.6541708999714,-323.835579298324)) ;
#26843=CARTESIAN_POINT('Ctrl Pts',(5.69752939147568,18.5713532688025,-323.839035396755)) ;
#26844=CARTESIAN_POINT('Ctrl Pts',(5.85260623832162,18.5230667946202,-323.840983513214)) ;
#26845=CARTESIAN_POINT('Ctrl Pts',(6.0813938881543,18.4486688776541,-323.84390071498)) ;
#26846=CARTESIAN_POINT('Ctrl Pts',(6.15558211518285,18.4240479749458,-323.844853444417)) ;
#26847=CARTESIAN_POINT('Ctrl Pts',(6.29284282748865,18.3775735491629,-323.846630343352)) ;
#26848=CARTESIAN_POINT('Ctrl Pts',(6.35595505133229,18.3558414613773,-323.847453096178)) ;
#26849=CARTESIAN_POINT('Ctrl Pts',(6.51380439161475,18.3005758589561,-323.849524529215)) ;
#26850=CARTESIAN_POINT('Ctrl Pts',(6.60839560648056,18.2666316514541,-323.850778092066)) ;
#26851=CARTESIAN_POINT('Ctrl Pts',(7.04447919596128,18.1063117196939,-323.85660706349)) ;
#26852=CARTESIAN_POINT('Ctrl Pts',(7.38263851109961,17.9710839668721,-323.861267609204)) ;
#26853=CARTESIAN_POINT('Ctrl Pts',(8.22600338520252,17.6060039231026,-323.873094471585)) ;
#26854=CARTESIAN_POINT('Ctrl Pts',(8.72553351070651,17.3638582330167,-323.880283893682)) ;
#26855=CARTESIAN_POINT('Ctrl Pts',(9.35374781505606,17.0253699520917,-323.889394129695)) ;
#26856=CARTESIAN_POINT('Ctrl Pts',(9.49255657955187,16.9483683537343,-323.891412233581)) ;
#26857=CARTESIAN_POINT('Ctrl Pts',(9.8296202460706,16.7559485142312,-323.896321544975)) ;
#26858=CARTESIAN_POINT('Ctrl Pts',(10.0268045249737,16.6387029569601,-323.899200977598)) ;
#26859=CARTESIAN_POINT('Ctrl Pts',(10.3370635211211,16.4467046892308,-323.90374044758)) ;
#26860=CARTESIAN_POINT('Ctrl Pts',(10.451512022963,16.3742136870409,-323.905416988784)) ;
#26861=CARTESIAN_POINT('Ctrl Pts',(10.6711397595513,16.2318619219588,-323.908638443262)) ;
#26862=CARTESIAN_POINT('Ctrl Pts',(10.7764146434824,16.1621611395826,-323.910184478566)) ;
#26863=CARTESIAN_POINT('Ctrl Pts',(11.0268075031128,15.992845930002,-323.913867177838)) ;
#26864=CARTESIAN_POINT('Ctrl Pts',(11.1712657574136,15.8922756756911,-323.915996277857)) ;
#26865=CARTESIAN_POINT('Ctrl Pts',(11.9232446476411,15.3534362615982,-323.927113703577)) ;
#26866=CARTESIAN_POINT('Ctrl Pts',(12.5064039418228,14.8822588539162,-323.935827359411)) ;
#26867=CARTESIAN_POINT('Ctrl Pts',(13.2795314224237,14.179982956458,-323.948038726717)) ;
#26868=CARTESIAN_POINT('Ctrl Pts',(13.4936125245616,13.9764191427277,-323.951501221385)) ;
#26869=CARTESIAN_POINT('Ctrl Pts',(13.7956691979493,13.6757903738945,-323.956560046464)) ;
#26870=CARTESIAN_POINT('Ctrl Pts',(13.8874361360587,13.5825935841234,-323.958121153379)) ;
#26871=CARTESIAN_POINT('Ctrl Pts',(14.0514941146829,13.4125785278567,-323.96096289631)) ;
#26872=CARTESIAN_POINT('Ctrl Pts',(14.1241140162456,13.3360846140068,-323.962239289385)) ;
#26873=CARTESIAN_POINT('Ctrl Pts',(14.2421887244028,13.2096647617785,-323.964348603576)) ;
#26874=CARTESIAN_POINT('Ctrl Pts',(14.2880126852939,13.1600864851035,-323.965175811265)) ;
#26875=CARTESIAN_POINT('Ctrl Pts',(14.3848666498527,13.0541951678067,-323.966943576037)) ;
#26876=CARTESIAN_POINT('Ctrl Pts',(14.4358264469138,12.9978196167208,-323.967885132581)) ;
#26877=CARTESIAN_POINT('Ctrl Pts',(14.5864912996801,12.8291638130494,-323.970701156253)) ;
#26878=CARTESIAN_POINT('Ctrl Pts',(14.6852265873954,12.7160250290335,-323.972589169031)) ;
#26879=CARTESIAN_POINT('Ctrl Pts',(15.1732287810414,12.1435681074222,-323.982112541924)) ;
#26880=CARTESIAN_POINT('Ctrl Pts',(15.5423042402199,11.6674717484546,-323.989928289688)) ;
#26881=CARTESIAN_POINT('Ctrl Pts',(16.1220994874027,10.8431163544081,-324.002906787567)) ;
#26882=CARTESIAN_POINT('Ctrl Pts',(16.3450717740052,10.5039941954433,-324.008103154881)) ;
#26883=CARTESIAN_POINT('Ctrl Pts',(16.6718083210111,9.97142986490923,-324.015996500905)) ;
#26884=CARTESIAN_POINT('Ctrl Pts',(16.783190469953,9.78279735743369,-324.018743251148)) ;
#26885=CARTESIAN_POINT('Ctrl Pts',(16.9573374918235,9.47613750782843,-324.023127980214)) ;
#26886=CARTESIAN_POINT('Ctrl Pts',(17.0221158998602,9.35927599917526,-324.024780498107)) ;
#26887=CARTESIAN_POINT('Ctrl Pts',(17.145491023379,9.13118639641089,-324.027970614032)) ;
#26888=CARTESIAN_POINT('Ctrl Pts',(17.2042238226143,9.02003936511063,-324.029509155398)) ;
#26889=CARTESIAN_POINT('Ctrl Pts',(17.3315178345717,8.77337886275919,-324.032889319376)) ;
#26890=CARTESIAN_POINT('Ctrl Pts',(17.399577133164,8.6376155729785,-324.034727267962)) ;
#26891=CARTESIAN_POINT('Ctrl Pts',(17.819715586545,7.77441180646962,-324.046279914371)) ;
#26892=CARTESIAN_POINT('Ctrl Pts',(18.127700411271,7.02639447393589,-324.055659154228)) ;
#26893=CARTESIAN_POINT('Ctrl Pts',(18.4750496852388,6.00631038139689,-324.068270333796)) ;
#26894=CARTESIAN_POINT('Ctrl Pts',(18.556584792282,5.74946830278234,-324.071434887027)) ;
#26895=CARTESIAN_POINT('Ctrl Pts',(18.6821350400666,5.32343651612519,-324.076714048854)) ;
#26896=CARTESIAN_POINT('Ctrl Pts',(18.7292565434663,5.15520078681904,-324.078806455304)) ;
#26897=CARTESIAN_POINT('Ctrl Pts',(18.794695643267,4.90881621843598,-324.081895175818)) ;
#26898=CARTESIAN_POINT('Ctrl Pts',(18.8148085691335,4.83115301708702,-324.0828722933)) ;
#26899=CARTESIAN_POINT('Ctrl Pts',(18.8506528809163,4.68912580615298,-324.084667315452)) ;
#26900=CARTESIAN_POINT('Ctrl Pts',(18.8665371296415,4.62480178668731,-324.085483453268)) ;
#26901=CARTESIAN_POINT('Ctrl Pts',(18.9047823430172,4.46644945151271,-324.087499872155)) ;
#26902=CARTESIAN_POINT('Ctrl Pts',(18.9267712161514,4.37233317980457,-324.088704447505)) ;
#26903=CARTESIAN_POINT('Ctrl Pts',(19.0129342588639,3.99070612638146,-324.093608070745)) ;
#26904=CARTESIAN_POINT('Ctrl Pts',(19.0712666876844,3.70191718677557,-324.09736235941)) ;
#26905=CARTESIAN_POINT('Ctrl Pts',(19.1571413140811,3.22060930498687,-324.103635621354)) ;
#26906=CARTESIAN_POINT('Ctrl Pts',(19.1884011865441,3.0288029762415,-324.106139960428)) ;
#26907=CARTESIAN_POINT('Ctrl Pts',(19.2860810594539,2.3670534054374,-324.114768260717)) ;
#26908=CARTESIAN_POINT('Ctrl Pts',(19.3381545187024,1.89516375334783,-324.120896549801)) ;
#26909=CARTESIAN_POINT('Ctrl Pts',(19.3835718623038,1.27634272530671,-324.128802861905)) ;
#26910=CARTESIAN_POINT('Ctrl Pts',(19.3926110283401,1.13072828685348,-324.13065431783)) ;
#26911=CARTESIAN_POINT('Ctrl Pts',(19.4109922510037,0.768711476549691,-324.135232277737)) ;
#26912=CARTESIAN_POINT('Ctrl Pts',(19.4183568186144,0.552228398323954,-324.137947574658)) ;
#26913=CARTESIAN_POINT('Ctrl Pts',(19.4244007697893,0.20251831684377,-324.142295582733)) ;
#26914=CARTESIAN_POINT('Ctrl Pts',(19.4253326789454,0.0693491450277581,
-324.143942380656)) ;
#26915=CARTESIAN_POINT('Ctrl Pts',(19.4244813800595,-0.189764089123379,
-324.147129549792)) ;
#26916=CARTESIAN_POINT('Ctrl Pts',(19.4228427253298,-0.31570208922855,-324.148670775783)) ;
#26917=CARTESIAN_POINT('Ctrl Pts',(19.4158360611705,-0.623819279378259,
-324.15242332307)) ;
#26918=CARTESIAN_POINT('Ctrl Pts',(19.4091286623342,-0.805956048857765,
-324.154625942019)) ;
#26919=CARTESIAN_POINT('Ctrl Pts',(19.3810162464742,-1.35797283713606,-324.161261337898)) ;
#26920=CARTESIAN_POINT('Ctrl Pts',(19.3515919324436,-1.72735966439392,-324.165645236293)) ;
#26921=CARTESIAN_POINT('Ctrl Pts',(19.2512512259567,-2.65199640169618,-324.176567253709)) ;
#26922=CARTESIAN_POINT('Ctrl Pts',(19.1668694517215,-3.20544419908358,-324.183053050338)) ;
#26923=CARTESIAN_POINT('Ctrl Pts',(19.0335344359576,-3.88228826772713,-324.191182299165)) ;
#26924=CARTESIAN_POINT('Ctrl Pts',(19.0070706603997,-4.00984540605621,-324.192723510309)) ;
#26925=CARTESIAN_POINT('Ctrl Pts',(18.9443021007148,-4.29780008340211,-324.196231347359)) ;
#26926=CARTESIAN_POINT('Ctrl Pts',(18.9072395071955,-4.45802217470933,-324.198203341717)) ;
#26927=CARTESIAN_POINT('Ctrl Pts',(18.849482261209,-4.69401833178835,-324.201149008251)) ;
#26928=CARTESIAN_POINT('Ctrl Pts',(18.8303552874522,-4.77016869120389,-324.202105868501)) ;
#26929=CARTESIAN_POINT('Ctrl Pts',(18.7941388073036,-4.91074473973838,-324.203885661795)) ;
#26930=CARTESIAN_POINT('Ctrl Pts',(18.7771784120087,-4.9752023330357,-324.204707117914)) ;
#26931=CARTESIAN_POINT('Ctrl Pts',(18.7339968130889,-5.1359465412719,-324.206768397711)) ;
#26932=CARTESIAN_POINT('Ctrl Pts',(18.7073647501064,-5.23212074926365,-324.208012996101)) ;
#26933=CARTESIAN_POINT('Ctrl Pts',(18.5851013659566,-5.66076987653046,-324.213604220541)) ;
#26934=CARTESIAN_POINT('Ctrl Pts',(18.4813394813232,-5.99085958224712,-324.21802752766)) ;
#26935=CARTESIAN_POINT('Ctrl Pts',(18.1530169867385,-6.94541723367151,-324.231010153445)) ;
#26936=CARTESIAN_POINT('Ctrl Pts',(17.9052108432216,-7.56136729532687,-324.239617472846)) ;
#26937=CARTESIAN_POINT('Ctrl Pts',(17.5125146059858,-8.40927233045729,-324.251488432656)) ;
#26938=CARTESIAN_POINT('Ctrl Pts',(17.3935235064486,-8.65270879152121,-324.254901801307)) ;
#26939=CARTESIAN_POINT('Ctrl Pts',(17.2041666955727,-9.02040039306527,-324.260058709053)) ;
#26940=CARTESIAN_POINT('Ctrl Pts',(17.1374589745752,-9.14650069182183,-324.261827616468)) ;
#26941=CARTESIAN_POINT('Ctrl Pts',(17.0099864066733,-9.38117608735243,-324.265120334795)) ;
#26942=CARTESIAN_POINT('Ctrl Pts',(16.9495556620643,-9.48992440657347,-324.266646487876)) ;
#26943=CARTESIAN_POINT('Ctrl Pts',(16.8100068467778,-9.73546424320192,-324.270093818968)) ;
#26944=CARTESIAN_POINT('Ctrl Pts',(16.730255858124,-9.87188600178964,-324.272010182737)) ;
#26945=CARTESIAN_POINT('Ctrl Pts',(16.4578490221333,-10.3250803138368,-324.278384292262)) ;
#26946=CARTESIAN_POINT('Ctrl Pts',(16.2577906060784,-10.6373080887085,-324.282787409926)) ;
#26947=CARTESIAN_POINT('Ctrl Pts',(15.9478116237152,-11.0918951451245,-324.289264240264)) ;
#26948=CARTESIAN_POINT('Ctrl Pts',(15.8446536467219,-11.2387625815284,-324.291367731757)) ;
#26949=CARTESIAN_POINT('Ctrl Pts',(15.468094697273,-11.7593833529207,-324.298883542137)) ;
#26950=CARTESIAN_POINT('Ctrl Pts',(15.1833848718419,-12.124762808691,-324.304266229413)) ;
#26951=CARTESIAN_POINT('Ctrl Pts',(14.7794880161957,-12.6065375627144,-324.311688107612)) ;
#26952=CARTESIAN_POINT('Ctrl Pts',(14.6714657692087,-12.7320912425245,-324.31365422033)) ;
#26953=CARTESIAN_POINT('Ctrl Pts',(14.4789375459549,-12.9501616596825,-324.317138572761)) ;
#26954=CARTESIAN_POINT('Ctrl Pts',(14.3951173055137,-13.0432709532823,-324.318649183161)) ;
#26955=CARTESIAN_POINT('Ctrl Pts',(14.2622324450179,-13.1880409837315,-324.321039527313)) ;
#26956=CARTESIAN_POINT('Ctrl Pts',(14.2137742598569,-13.2402537958351,-324.321910281528)) ;
#26957=CARTESIAN_POINT('Ctrl Pts',(14.1226895817937,-13.337319542058,-324.32354652899)) ;
#26958=CARTESIAN_POINT('Ctrl Pts',(14.0801338407855,-13.3822376530489,-324.324310825099)) ;
#26959=CARTESIAN_POINT('Ctrl Pts',(13.9600900650932,-13.5077388280364,-324.326465270509)) ;
#26960=CARTESIAN_POINT('Ctrl Pts',(13.8821199813453,-13.587857360246,-324.327862836662)) ;
#26961=CARTESIAN_POINT('Ctrl Pts',(13.3198593051154,-14.1557197237068,-324.337913664347)) ;
#26962=CARTESIAN_POINT('Ctrl Pts',(12.81067339067,-14.618129177171,-324.346853736898)) ;
#26963=CARTESIAN_POINT('Ctrl Pts',(12.0183225785821,-15.2644322009246,-324.360015005856)) ;
#26964=CARTESIAN_POINT('Ctrl Pts',(11.7531520033427,-15.4695309119914,-324.364308383037)) ;
#26965=CARTESIAN_POINT('Ctrl Pts',(11.3881690686964,-15.7370263250289,-324.370044077578)) ;
#26966=CARTESIAN_POINT('Ctrl Pts',(11.2929040829425,-15.8055278209848,-324.371525822738)) ;
#26967=CARTESIAN_POINT('Ctrl Pts',(11.0448875511486,-15.9804801788329,-324.375342920027)) ;
#26968=CARTESIAN_POINT('Ctrl Pts',(10.8912156756376,-16.0856056467634,-324.377668735046)) ;
#26969=CARTESIAN_POINT('Ctrl Pts',(10.6295171300252,-16.2591615213897,-324.381562964749)) ;
#26970=CARTESIAN_POINT('Ctrl Pts',(10.5222830843481,-16.3287637786815,-324.383140271606)) ;
#26971=CARTESIAN_POINT('Ctrl Pts',(10.3158913591436,-16.4598487383366,-324.386141494111)) ;
#26972=CARTESIAN_POINT('Ctrl Pts',(10.2168514799252,-16.5215066170698,-324.387566706128)) ;
#26973=CARTESIAN_POINT('Ctrl Pts',(9.94955033317331,-16.6845938176103,-324.391374301421)) ;
#26974=CARTESIAN_POINT('Ctrl Pts',(9.78029569111016,-16.7843688905172,-324.393744250283)) ;
#26975=CARTESIAN_POINT('Ctrl Pts',(9.26246603281474,-17.0791351057108,-324.400881323137)) ;
#26976=CARTESIAN_POINT('Ctrl Pts',(8.90936440882511,-17.2659595630313,-324.405592601799)) ;
#26977=CARTESIAN_POINT('Ctrl Pts',(8.09026389142239,-17.6675202552011,-324.416282278911)) ;
#26978=CARTESIAN_POINT('Ctrl Pts',(7.62101385343965,-17.8749486244568,-324.422234049938)) ;
#26979=CARTESIAN_POINT('Ctrl Pts',(6.98270746560611,-18.1273976659743,-324.430329249737)) ;
#26980=CARTESIAN_POINT('Ctrl Pts',(6.82045926039131,-18.1890649852683,-324.432387472011)) ;
#26981=CARTESIAN_POINT('Ctrl Pts',(6.53570661518215,-18.2929479900004,-324.436015219369)) ;
#26982=CARTESIAN_POINT('Ctrl Pts',(6.41356558710243,-18.3361278220489,-324.437576227114)) ;
#26983=CARTESIAN_POINT('Ctrl Pts',(6.22280664554407,-18.4014265205564,-324.440027704807)) ;
#26984=CARTESIAN_POINT('Ctrl Pts',(6.15448198543807,-18.4243906822909,-324.440908439457)) ;
#26985=CARTESIAN_POINT('Ctrl Pts',(6.02773974167217,-18.4662055210767,-324.44254842077)) ;
#26986=CARTESIAN_POINT('Ctrl Pts',(5.96935757792709,-18.4851606113572,-324.44330632624)) ;
#26987=CARTESIAN_POINT('Ctrl Pts',(5.807253738359,-18.5369432406899,-324.445416578835)) ;
#26988=CARTESIAN_POINT('Ctrl Pts',(5.70334466969332,-18.5691766166284,-324.446775865346)) ;
#26989=CARTESIAN_POINT('Ctrl Pts',(5.37440883403443,-18.6681935412559,-324.451093619567)) ;
#26990=CARTESIAN_POINT('Ctrl Pts',(5.14843963413857,-18.7317721913582,-324.454081327165)) ;
#26991=CARTESIAN_POINT('Ctrl Pts',(4.30396942894941,-18.9529366247887,-324.465262939739)) ;
#26992=CARTESIAN_POINT('Ctrl Pts',(3.67897035963435,-19.0841069828959,-324.473557659298)) ;
#26993=CARTESIAN_POINT('Ctrl Pts',(2.70140624977385,-19.2394556179909,-324.48621266116)) ;
#26994=CARTESIAN_POINT('Ctrl Pts',(2.35272785827551,-19.2851995261928,-324.490667728301)) ;
#26995=CARTESIAN_POINT('Ctrl Pts',(1.84945245054677,-19.3373726449075,-324.496994520506)) ;
#26996=CARTESIAN_POINT('Ctrl Pts',(1.69572065494551,-19.3514595502254,-324.498913515799)) ;
#26997=CARTESIAN_POINT('Ctrl Pts',(1.43018252699412,-19.3726030450014,-324.502204605072)) ;
#26998=CARTESIAN_POINT('Ctrl Pts',(1.31845301135227,-19.380527662859,-324.503582218661)) ;
#26999=CARTESIAN_POINT('Ctrl Pts',(1.06468201517957,-19.3963221607867,-324.506695370624)) ;
#27000=CARTESIAN_POINT('Ctrl Pts',(0.922610002033545,-19.403598944801,-324.508426999435)) ;
#27001=CARTESIAN_POINT('Ctrl Pts',(0.520324503775809,-19.419775305685,-324.513300715947)) ;
#27002=CARTESIAN_POINT('Ctrl Pts',(0.259993944107991,-19.4250048653043,
-324.516419438809)) ;
#27003=CARTESIAN_POINT('Ctrl Pts',(-0.000363249083133038,-19.4249999966036,
-324.51951242736)) ;
#27004=CARTESIAN_POINT('Origin',(0.,0.,-328.125)) ;
#27005=CARTESIAN_POINT('',(0.000472547777405694,-19.4249999942522,-326.231461493639)) ;
#27006=CARTESIAN_POINT('',(0.000483615249731608,-19.4249999937201,-326.018849107561)) ;
#27007=CARTESIAN_POINT('',(-2.37887640734373E-15,-19.425,-328.125)) ;
#27008=CARTESIAN_POINT('Ctrl Pts',(0.000472547765765496,-19.4249999942522,
-326.231461493639)) ;
#27009=CARTESIAN_POINT('Ctrl Pts',(0.396084841908866,-19.4249903702777,
-326.226835776913)) ;
#27010=CARTESIAN_POINT('Ctrl Pts',(0.791603743676953,-19.4128951015776,
-326.222193988934)) ;
#27011=CARTESIAN_POINT('Ctrl Pts',(1.30529304516484,-19.3814603553559,-326.216022043007)) ;
#27012=CARTESIAN_POINT('Ctrl Pts',(1.42404097536059,-19.3730973950539,-326.214585139653)) ;
#27013=CARTESIAN_POINT('Ctrl Pts',(1.60563597321444,-19.3586296944345,-326.212367709118)) ;
#27014=CARTESIAN_POINT('Ctrl Pts',(1.66854271952288,-19.3533091668245,-326.211595873353)) ;
#27015=CARTESIAN_POINT('Ctrl Pts',(1.80073618527897,-19.3414791852382,-326.209965196664)) ;
#27016=CARTESIAN_POINT('Ctrl Pts',(1.87001606900058,-19.3349038723957,-326.209105486689)) ;
#27017=CARTESIAN_POINT('Ctrl Pts',(2.05563583516961,-19.3162798234963,-326.206789770731)) ;
#27018=CARTESIAN_POINT('Ctrl Pts',(2.17190470149032,-19.303552388465,-326.205326281727)) ;
#27019=CARTESIAN_POINT('Ctrl Pts',(2.36736283260079,-19.2803681766676,-326.202848152535)) ;
#27020=CARTESIAN_POINT('Ctrl Pts',(2.44661547478579,-19.270471621426,-326.201838380587)) ;
#27021=CARTESIAN_POINT('Ctrl Pts',(2.65612601446928,-19.2429960065884,-326.199157691651)) ;
#27022=CARTESIAN_POINT('Ctrl Pts',(2.7862703524327,-19.2245831732981,-326.197480955458)) ;
#27023=CARTESIAN_POINT('Ctrl Pts',(3.47989406675427,-19.1192578192112,-326.188498333768)) ;
#27024=CARTESIAN_POINT('Ctrl Pts',(4.03952898542165,-19.0088897385276,-326.18109671263)) ;
#27025=CARTESIAN_POINT('Ctrl Pts',(4.89285894758898,-18.8012095801006,-326.169831073617)) ;
#27026=CARTESIAN_POINT('Ctrl Pts',(5.19044480333996,-18.7212401741557,-326.165904310168)) ;
#27027=CARTESIAN_POINT('Ctrl Pts',(5.68339826004158,-18.5761123874569,-326.159423465814)) ;
#27028=CARTESIAN_POINT('Ctrl Pts',(5.87985801859845,-18.5148653005826,-326.156846833119)) ;
#27029=CARTESIAN_POINT('Ctrl Pts',(6.19995025965793,-18.4094666395598,-326.152660754872)) ;
#27030=CARTESIAN_POINT('Ctrl Pts',(6.32417374400339,-18.3671628643641,-326.151039156393)) ;
#27031=CARTESIAN_POINT('Ctrl Pts',(6.56937795113919,-18.2808770692902,-326.147843866928)) ;
#27032=CARTESIAN_POINT('Ctrl Pts',(6.69036918367765,-18.2369447365749,-326.14626993091)) ;
#27033=CARTESIAN_POINT('Ctrl Pts',(6.99019521860138,-18.1246915156906,-326.142375203866)) ;
#27034=CARTESIAN_POINT('Ctrl Pts',(7.16847366040169,-18.0549233526264,-326.140064455599)) ;
#27035=CARTESIAN_POINT('Ctrl Pts',(7.55793724072128,-17.8958312096743,-326.13502141511)) ;
#27036=CARTESIAN_POINT('Ctrl Pts',(7.76863118091874,-17.8053800803884,-326.132296549346)) ;
#27037=CARTESIAN_POINT('Ctrl Pts',(8.47703854575547,-17.4862917638369,-326.123119856379)) ;
#27038=CARTESIAN_POINT('Ctrl Pts',(8.96666650135865,-17.2403443607228,-326.116758422149)) ;
#27039=CARTESIAN_POINT('Ctrl Pts',(9.77294345290514,-16.7916895589981,-326.105953059719)) ;
#27040=CARTESIAN_POINT('Ctrl Pts',(10.0952915702622,-16.5998900229452,-326.101537009417)) ;
#27041=CARTESIAN_POINT('Ctrl Pts',(10.4963999569461,-16.3452205632584,-326.095814785557)) ;
#27042=CARTESIAN_POINT('Ctrl Pts',(10.5804994655467,-16.2909078426628,-326.094601904215)) ;
#27043=CARTESIAN_POINT('Ctrl Pts',(10.7199208244748,-16.199332416763,-326.092566255682)) ;
#27044=CARTESIAN_POINT('Ctrl Pts',(10.775477402656,-16.1624305098516,-326.091748366406)) ;
#27045=CARTESIAN_POINT('Ctrl Pts',(10.895887921769,-16.0815543700598,-326.089960233181)) ;
#27046=CARTESIAN_POINT('Ctrl Pts',(10.9606679288801,-16.0374724658583,-326.088988573305)) ;
#27047=CARTESIAN_POINT('Ctrl Pts',(11.1598032586344,-15.9001934843546,-326.085974014216)) ;
#27048=CARTESIAN_POINT('Ctrl Pts',(11.2932497849952,-15.8056910877373,-326.083914737489)) ;
#27049=CARTESIAN_POINT('Ctrl Pts',(11.5299474163125,-15.6335415553318,-326.080202611092)) ;
#27050=CARTESIAN_POINT('Ctrl Pts',(11.6336473610395,-15.5565278264689,-326.078555329287)) ;
#27051=CARTESIAN_POINT('Ctrl Pts',(12.1746904051219,-15.1462816011811,-326.069864348592)) ;
#27052=CARTESIAN_POINT('Ctrl Pts',(12.5985073981272,-14.7956258755794,-326.062729072707)) ;
#27053=CARTESIAN_POINT('Ctrl Pts',(13.3244840162353,-14.1411318903667,-326.050178730053)) ;
#27054=CARTESIAN_POINT('Ctrl Pts',(13.6325491130252,-13.844388457096,-326.044735417857)) ;
#27055=CARTESIAN_POINT('Ctrl Pts',(14.0433691453359,-13.4216468675579,-326.03735055532)) ;
#27056=CARTESIAN_POINT('Ctrl Pts',(14.1547135357055,-13.3041687607106,-326.03533511821)) ;
#27057=CARTESIAN_POINT('Ctrl Pts',(14.349286739696,-13.093669057971,-326.031788505995)) ;
#27058=CARTESIAN_POINT('Ctrl Pts',(14.4331115795398,-13.0012110788826,-326.030252171891)) ;
#27059=CARTESIAN_POINT('Ctrl Pts',(14.6093078536236,-12.8030640630554,-326.027004305764)) ;
#27060=CARTESIAN_POINT('Ctrl Pts',(14.7014365272681,-12.697168560939,-326.025294917591)) ;
#27061=CARTESIAN_POINT('Ctrl Pts',(14.9591472116259,-12.3943825371397,-326.020479082189)) ;
#27062=CARTESIAN_POINT('Ctrl Pts',(15.1219770626562,-12.1951881428237,-326.017395530525)) ;
#27063=CARTESIAN_POINT('Ctrl Pts',(15.4996929057522,-11.7139166756847,-326.010122851828)) ;
#27064=CARTESIAN_POINT('Ctrl Pts',(15.710906538774,-11.4290743394916,-326.005958671032)) ;
#27065=CARTESIAN_POINT('Ctrl Pts',(16.2506144402162,-10.6579707793137,-325.994949217009)) ;
#27066=CARTESIAN_POINT('Ctrl Pts',(16.565074473972,-10.1623380600414,-325.988145466328)) ;
#27067=CARTESIAN_POINT('Ctrl Pts',(16.9312463594053,-9.52292352911861,-325.97935700466)) ;
#27068=CARTESIAN_POINT('Ctrl Pts',(17.0043591495648,-9.39174880526528,-325.977552902012)) ;
#27069=CARTESIAN_POINT('Ctrl Pts',(17.1121698836036,-9.19293436211056,-325.974808053192)) ;
#27070=CARTESIAN_POINT('Ctrl Pts',(17.1480039276312,-9.12591702736912,-325.973881030145)) ;
#27071=CARTESIAN_POINT('Ctrl Pts',(17.2149267948511,-8.99897094887938,-325.972120194062)) ;
#27072=CARTESIAN_POINT('Ctrl Pts',(17.2460982151123,-8.93908714618695,-325.971287412036)) ;
#27073=CARTESIAN_POINT('Ctrl Pts',(17.3251656313346,-8.78523672972515,-325.969143362188)) ;
#27074=CARTESIAN_POINT('Ctrl Pts',(17.3726096636444,-8.6910403278129,-325.967826443599)) ;
#27075=CARTESIAN_POINT('Ctrl Pts',(17.6397247722339,-8.14977651512699,-325.960245303503)) ;
#27076=CARTESIAN_POINT('Ctrl Pts',(17.8429019095926,-7.6947772836951,-325.953823127078)) ;
#27077=CARTESIAN_POINT('Ctrl Pts',(18.271838173851,-6.62556919956201,-325.938960369494)) ;
#27078=CARTESIAN_POINT('Ctrl Pts',(18.4845107431424,-6.00675500020633,-325.930534180472)) ;
#27079=CARTESIAN_POINT('Ctrl Pts',(18.7171504889706,-5.19938532732032,-325.91996710361)) ;
#27080=CARTESIAN_POINT('Ctrl Pts',(18.7661536168004,-5.01964229726913,-325.917639830639)) ;
#27081=CARTESIAN_POINT('Ctrl Pts',(18.844099693531,-4.7166255067859,-325.913759664277)) ;
#27082=CARTESIAN_POINT('Ctrl Pts',(18.8744365109715,-4.59372353040788,-325.912197700383)) ;
#27083=CARTESIAN_POINT('Ctrl Pts',(18.9339734996157,-4.34197246584523,-325.909021890631)) ;
#27084=CARTESIAN_POINT('Ctrl Pts',(18.9630648768828,-4.21310430783586,-325.907408837553)) ;
#27085=CARTESIAN_POINT('Ctrl Pts',(19.0351365151872,-3.87796280650687,-325.903245028846)) ;
#27086=CARTESIAN_POINT('Ctrl Pts',(19.0760793072788,-3.67126901026545,-325.900707673654)) ;
#27087=CARTESIAN_POINT('Ctrl Pts',(19.1386435201803,-3.32604734238882,-325.896513726673)) ;
#27088=CARTESIAN_POINT('Ctrl Pts',(19.1621423368513,-3.1878782644296,-325.894846770509)) ;
#27089=CARTESIAN_POINT('Ctrl Pts',(19.2536930146786,-2.61193452786711,-325.887939074793)) ;
#27090=CARTESIAN_POINT('Ctrl Pts',(19.3082536480854,-2.17215058894986,-325.882765514894)) ;
#27091=CARTESIAN_POINT('Ctrl Pts',(19.3533723314318,-1.66781714160012,-325.876851656223)) ;
#27092=CARTESIAN_POINT('Ctrl Pts',(19.3587062438886,-1.60472028063411,-325.87611204624)) ;
#27093=CARTESIAN_POINT('Ctrl Pts',(19.3723718487853,-1.43306916054423,-325.874099860656)) ;
#27094=CARTESIAN_POINT('Ctrl Pts',(19.3800995802141,-1.32446914582103,-325.872826668675)) ;
#27095=CARTESIAN_POINT('Ctrl Pts',(19.4092960029773,-0.85891238884552,-325.8673607595)) ;
#27096=CARTESIAN_POINT('Ctrl Pts',(19.4218184782115,-0.501465522976049,
-325.863145504404)) ;
#27097=CARTESIAN_POINT('Ctrl Pts',(19.425209268976,-0.0436874878296498,
-325.857632172223)) ;
#27098=CARTESIAN_POINT('Ctrl Pts',(19.4251762054148,0.0565074280901048,
-325.856418319449)) ;
#27099=CARTESIAN_POINT('Ctrl Pts',(19.4238298594906,0.223401737647895,-325.854381558668)) ;
#27100=CARTESIAN_POINT('Ctrl Pts',(19.4229481584071,0.290102726359439,-325.853563541254)) ;
#27101=CARTESIAN_POINT('Ctrl Pts',(19.4202844115637,0.435099498364049,-325.851775790253)) ;
#27102=CARTESIAN_POINT('Ctrl Pts',(19.4183724160824,0.513391555499843,-325.850804647716)) ;
#27103=CARTESIAN_POINT('Ctrl Pts',(19.4110137382568,0.754870814786239,-325.847793590315)) ;
#27104=CARTESIAN_POINT('Ctrl Pts',(19.4039829861281,0.918002409764678,-325.845737350085)) ;
#27105=CARTESIAN_POINT('Ctrl Pts',(19.3648500244098,1.62009465194668,-325.836818990162)) ;
#27106=CARTESIAN_POINT('Ctrl Pts',(19.312342056374,2.1576763271493,-325.829822673471)) ;
#27107=CARTESIAN_POINT('Ctrl Pts',(19.1617932126091,3.23337699561174,-325.815823072259)) ;
#27108=CARTESIAN_POINT('Ctrl Pts',(19.0632889334125,3.77095004986145,-325.808827641273)) ;
#27109=CARTESIAN_POINT('Ctrl Pts',(18.907937506103,4.45471909157949,-325.800029815056)) ;
#27110=CARTESIAN_POINT('Ctrl Pts',(18.8718103689917,4.60536604461547,-325.798097191525)) ;
#27111=CARTESIAN_POINT('Ctrl Pts',(18.8029470312267,4.87809162635995,-325.794609299792)) ;
#27112=CARTESIAN_POINT('Ctrl Pts',(18.7708140035024,5.00031365710854,-325.793050178972)) ;
#27113=CARTESIAN_POINT('Ctrl Pts',(18.7025662023517,5.24996989065656,-325.789873234782)) ;
#27114=CARTESIAN_POINT('Ctrl Pts',(18.6663360928169,5.37736583577967,-325.788256275946)) ;
#27115=CARTESIAN_POINT('Ctrl Pts',(18.5685715019384,5.70823636677896,-325.784066213437)) ;
#27116=CARTESIAN_POINT('Ctrl Pts',(18.5049948939301,5.91108908958802,-325.781506853459)) ;
#27117=CARTESIAN_POINT('Ctrl Pts',(18.3543613027813,6.36544245985224,-325.775786320851)) ;
#27118=CARTESIAN_POINT('Ctrl Pts',(18.2654393628329,6.61628005150345,-325.772636693414)) ;
#27119=CARTESIAN_POINT('Ctrl Pts',(18.0175211818165,7.27248974960846,-325.764384178665)) ;
#27120=CARTESIAN_POINT('Ctrl Pts',(17.8500010577672,7.67447971423041,-325.759317554533)) ;
#27121=CARTESIAN_POINT('Ctrl Pts',(17.6271365894711,8.16240710837583,-325.753041881376)) ;
#27122=CARTESIAN_POINT('Ctrl Pts',(17.5844409502142,8.25398513474412,-325.75185826426)) ;
#27123=CARTESIAN_POINT('Ctrl Pts',(17.4074493418963,8.62600809272875,-325.747020643377)) ;
#27124=CARTESIAN_POINT('Ctrl Pts',(17.2671436068629,8.9035419401335,-325.743343976852)) ;
#27125=CARTESIAN_POINT('Ctrl Pts',(17.0738027308345,9.26420771263443,-325.738413194164)) ;
#27126=CARTESIAN_POINT('Ctrl Pts',(17.0267117592125,9.35047436581089,-325.737221999383)) ;
#27127=CARTESIAN_POINT('Ctrl Pts',(16.946686515366,9.49446455000255,-325.735211040179)) ;
#27128=CARTESIAN_POINT('Ctrl Pts',(16.914107029944,9.55238317534052,-325.734395871269)) ;
#27129=CARTESIAN_POINT('Ctrl Pts',(16.8419967647843,9.67905259429694,-325.732598532699)) ;
#27130=CARTESIAN_POINT('Ctrl Pts',(16.8023409570405,9.74773063283268,-325.731614785599)) ;
#27131=CARTESIAN_POINT('Ctrl Pts',(16.6768041268439,9.96209968189783,-325.728517438262)) ;
#27132=CARTESIAN_POINT('Ctrl Pts',(16.5894404450087,10.1069130560024,-325.726386204364)) ;
#27133=CARTESIAN_POINT('Ctrl Pts',(16.2221460244764,10.6981418528673,-325.717551998203)) ;
#27134=CARTESIAN_POINT('Ctrl Pts',(15.9259992493394,11.1342179038783,-325.710725819506)) ;
#27135=CARTESIAN_POINT('Ctrl Pts',(15.2832966131833,12.0023991109174,-325.696802487383)) ;
#27136=CARTESIAN_POINT('Ctrl Pts',(14.9352524282809,12.4328185922866,-325.689716562144)) ;
#27137=CARTESIAN_POINT('Ctrl Pts',(14.4675281589715,12.9632147058041,-325.680845568925)) ;
#27138=CARTESIAN_POINT('Ctrl Pts',(14.3643777437455,13.0774217130603,-325.678926059348)) ;
#27139=CARTESIAN_POINT('Ctrl Pts',(14.1742228968212,13.2829945039999,-325.675454156428)) ;
#27140=CARTESIAN_POINT('Ctrl Pts',(14.0876646352958,13.3747614144889,-325.67389803525)) ;
#27141=CARTESIAN_POINT('Ctrl Pts',(13.9081467453182,13.5614055301608,-325.670719658124)) ;
#27142=CARTESIAN_POINT('Ctrl Pts',(13.8150954490209,13.6561855447752,-325.669098345074)) ;
#27143=CARTESIAN_POINT('Ctrl Pts',(13.5691389656526,13.9016246344569,-325.664879067421)) ;
#27144=CARTESIAN_POINT('Ctrl Pts',(13.4146956986639,14.0507166817985,-325.662295232026)) ;
#27145=CARTESIAN_POINT('Ctrl Pts',(13.1525768129787,14.2954916124292,-325.658010403642)) ;
#27146=CARTESIAN_POINT('Ctrl Pts',(13.0462510346838,14.3925915406517,-325.656298880989)) ;
#27147=CARTESIAN_POINT('Ctrl Pts',(12.5928614539457,14.7974879823851,-325.64910351462)) ;
#27148=CARTESIAN_POINT('Ctrl Pts',(12.2359100273527,15.093982786436,-325.643692749335)) ;
#27149=CARTESIAN_POINT('Ctrl Pts',(11.7488876920241,15.4698792771196,-325.636506148707)) ;
#27150=CARTESIAN_POINT('Ctrl Pts',(11.6280110639731,15.5609410229762,-325.634737342497)) ;
#27151=CARTESIAN_POINT('Ctrl Pts',(11.2273698264863,15.8554867178555,-325.628908145165)) ;
#27152=CARTESIAN_POINT('Ctrl Pts',(10.9432335434142,16.0529103544129,-325.62482770151)) ;
#27153=CARTESIAN_POINT('Ctrl Pts',(10.5700809031297,16.297671054631,-325.619453391335)) ;
#27154=CARTESIAN_POINT('Ctrl Pts',(10.4857585903689,16.3520506007277,-325.618237862659)) ;
#27155=CARTESIAN_POINT('Ctrl Pts',(10.3446639730459,16.4415025061108,-325.61619918184)) ;
#27156=CARTESIAN_POINT('Ctrl Pts',(10.2881254175035,16.4769400307424,-325.615380942167)) ;
#27157=CARTESIAN_POINT('Ctrl Pts',(10.1648936269429,16.553298307062,-325.61359384479)) ;
#27158=CARTESIAN_POINT('Ctrl Pts',(10.0981336076106,16.5941087411156,-325.612623590125)) ;
#27159=CARTESIAN_POINT('Ctrl Pts',(9.89165476917093,16.7186218925867,-325.609618534667)) ;
#27160=CARTESIAN_POINT('Ctrl Pts',(9.75112850969913,16.8009715404932,-325.607567497704)) ;
#27161=CARTESIAN_POINT('Ctrl Pts',(9.497987099999,16.9450687574504,-325.603873416864)) ;
#27162=CARTESIAN_POINT('Ctrl Pts',(9.38576360586516,17.0074852824696,-325.602235946072)) ;
#27163=CARTESIAN_POINT('Ctrl Pts',(8.79556612168375,17.3281208697744,-325.593639521415)) ;
#27164=CARTESIAN_POINT('Ctrl Pts',(8.30753342520917,17.5673175379234,-325.586590346927)) ;
#27165=CARTESIAN_POINT('Ctrl Pts',(7.42357290732393,17.9554843794327,-325.574190601969)) ;
#27166=CARTESIAN_POINT('Ctrl Pts',(7.03159627399173,18.1125787616569,-325.568813203361)) ;
#27167=CARTESIAN_POINT('Ctrl Pts',(6.4916775198293,18.3087940989341,-325.561609130395)) ;
#27168=CARTESIAN_POINT('Ctrl Pts',(6.34793587494923,18.3591265748238,-325.55971002771)) ;
#27169=CARTESIAN_POINT('Ctrl Pts',(6.08440513016666,18.4479393103549,-325.556262926084)) ;
#27170=CARTESIAN_POINT('Ctrl Pts',(5.96480560268138,18.4869560706288,-325.554711392624)) ;
#27171=CARTESIAN_POINT('Ctrl Pts',(5.71758288809553,18.5649582856223,-325.551530298572)) ;
#27172=CARTESIAN_POINT('Ctrl Pts',(5.58991992884497,18.6037959963842,-325.549901806679)) ;
#27173=CARTESIAN_POINT('Ctrl Pts',(5.25258801267257,18.7026335507579,-325.545634444311)) ;
#27174=CARTESIAN_POINT('Ctrl Pts',(5.04229121569352,18.7604232916986,-325.543010345816)) ;
#27175=CARTESIAN_POINT('Ctrl Pts',(4.68834397027207,18.8513068070034,-325.538646339078)) ;
#27176=CARTESIAN_POINT('Ctrl Pts',(4.54520968921524,18.8863285593903,-325.536895765584)) ;
#27177=CARTESIAN_POINT('Ctrl Pts',(3.93124955800609,19.0291669760619,-325.529438420388)) ;
#27178=CARTESIAN_POINT('Ctrl Pts',(3.45688959178512,19.1210311832898,-325.523810351705)) ;
#27179=CARTESIAN_POINT('Ctrl Pts',(2.84212074088501,19.2164598907093,-325.516540622699)) ;
#27180=CARTESIAN_POINT('Ctrl Pts',(2.70441595484694,19.2363228128021,-325.514913420452)) ;
#27181=CARTESIAN_POINT('Ctrl Pts',(2.23751401919986,19.2985573881291,-325.509387988822)) ;
#27182=CARTESIAN_POINT('Ctrl Pts',(1.90744899709749,19.3339707156132,-325.50546887953)) ;
#27183=CARTESIAN_POINT('Ctrl Pts',(1.4778991003224,19.368950763298,-325.500277049071)) ;
#27184=CARTESIAN_POINT('Ctrl Pts',(1.37909821824477,19.3762361538079,-325.499076535612)) ;
#27185=CARTESIAN_POINT('Ctrl Pts',(1.21383665341167,19.3871518028391,-325.497055001474)) ;
#27186=CARTESIAN_POINT('Ctrl Pts',(1.14740522044847,19.391196861357,-325.49623869752)) ;
#27187=CARTESIAN_POINT('Ctrl Pts',(1.00219016441312,19.3992902683791,-325.494445476449)) ;
#27188=CARTESIAN_POINT('Ctrl Pts',(0.923400190141356,19.4032002543485,-325.49346705268)) ;
#27189=CARTESIAN_POINT('Ctrl Pts',(0.678114941577363,19.4138752214988,-325.490406399665)) ;
#27190=CARTESIAN_POINT('Ctrl Pts',(0.511555090690949,19.4189778883406,-325.488307099043)) ;
#27191=CARTESIAN_POINT('Ctrl Pts',(0.212096983529731,19.4242965252181,-325.484506877959)) ;
#27192=CARTESIAN_POINT('Ctrl Pts',(0.0792228208986704,19.4252929018594,
-325.482811492848)) ;
#27193=CARTESIAN_POINT('Ctrl Pts',(-0.637144776103283,19.4233143195477,
-325.473637808661)) ;
#27194=CARTESIAN_POINT('Ctrl Pts',(-1.22026982434284,19.3954127480834,-325.466061074104)) ;
#27195=CARTESIAN_POINT('Ctrl Pts',(-1.8645501317094,19.3354110137535,-325.457766339239)) ;
#27196=CARTESIAN_POINT('Ctrl Pts',(-1.92781786674355,19.3292054813668,-325.456952503665)) ;
#27197=CARTESIAN_POINT('Ctrl Pts',(-2.32890427390012,19.287876622844,-325.451798510013)) ;
#27198=CARTESIAN_POINT('Ctrl Pts',(-2.66578387154997,19.2442089192046,-325.447494783036)) ;
#27199=CARTESIAN_POINT('Ctrl Pts',(-3.15653004257167,19.1674623850162,-325.441280217299)) ;
#27200=CARTESIAN_POINT('Ctrl Pts',(-3.31141454551974,19.1413121282674,-325.43932667505)) ;
#27201=CARTESIAN_POINT('Ctrl Pts',(-3.58810845795464,19.0911370094629,-325.435850996478)) ;
#27202=CARTESIAN_POINT('Ctrl Pts',(-3.71003689988122,19.0678174122861,-325.43432436018)) ;
#27203=CARTESIAN_POINT('Ctrl Pts',(-3.97399378550779,19.0147063014837,-325.431029628515)) ;
#27204=CARTESIAN_POINT('Ctrl Pts',(-4.11592894129979,18.9844887042316,-325.429264437186)) ;
#27205=CARTESIAN_POINT('Ctrl Pts',(-4.53672429806264,18.8899616471011,-325.424047724228)) ;
#27206=CARTESIAN_POINT('Ctrl Pts',(-4.81451647953566,18.8210772781552,-325.420626047351)) ;
#27207=CARTESIAN_POINT('Ctrl Pts',(-5.30638877774985,18.687504440139,-325.414584514576)) ;
#27208=CARTESIAN_POINT('Ctrl Pts',(-5.52106502101552,18.6252094011296,-325.411953423699)) ;
#27209=CARTESIAN_POINT('Ctrl Pts',(-6.13783686938827,18.4346329357197,-325.404383996537)) ;
#27210=CARTESIAN_POINT('Ctrl Pts',(-6.53688761140747,18.2969350700254,-325.39947589223)) ;
#27211=CARTESIAN_POINT('Ctrl Pts',(-7.24928254297333,18.0248304259889,-325.390533864692)) ;
#27212=CARTESIAN_POINT('Ctrl Pts',(-7.5641781448081,17.8949662547641,-325.386514902835)) ;
#27213=CARTESIAN_POINT('Ctrl Pts',(-7.96648494652901,17.716536066583,-325.381213741478)) ;
#27214=CARTESIAN_POINT('Ctrl Pts',(-8.05716260927202,17.6754819807262,-325.380007668473)) ;
#27215=CARTESIAN_POINT('Ctrl Pts',(-8.20799421657633,17.6057914821919,-325.377979800514)) ;
#27216=CARTESIAN_POINT('Ctrl Pts',(-8.26832362945437,17.5775392800325,-325.377162794693)) ;
#27217=CARTESIAN_POINT('Ctrl Pts',(-8.3995556877948,17.5152583247555,-325.375371912301)) ;
#27218=CARTESIAN_POINT('Ctrl Pts',(-8.4703992682553,17.4811082643757,-325.3743965703)) ;
#27219=CARTESIAN_POINT('Ctrl Pts',(-8.68941199258846,17.3738895157889,-325.371356990998)) ;
#27220=CARTESIAN_POINT('Ctrl Pts',(-8.83685765693119,17.2993602276784,-325.369276001264)) ;
#27221=CARTESIAN_POINT('Ctrl Pts',(-9.09963580621888,17.1622976041766,-325.365516174525)) ;
#27222=CARTESIAN_POINT('Ctrl Pts',(-9.21531970046943,17.1004594566374,-325.363842889233)) ;
#27223=CARTESIAN_POINT('Ctrl Pts',(-9.82830009622013,16.7647677095671,-325.354895062352)) ;
#27224=CARTESIAN_POINT('Ctrl Pts',(-10.3140384817978,16.470383436115,-325.347525279057)) ;
#27225=CARTESIAN_POINT('Ctrl Pts',(-11.0542380440815,15.9761800330096,-325.336107181016)) ;
#27226=CARTESIAN_POINT('Ctrl Pts',(-11.3177954555445,15.7905672429973,-325.331999949366)) ;
#27227=CARTESIAN_POINT('Ctrl Pts',(-11.7373448421941,15.4791933200159,-325.325415713842)) ;
#27228=CARTESIAN_POINT('Ctrl Pts',(-11.896223738703,15.3574265659992,-325.322910934181)) ;
#27229=CARTESIAN_POINT('Ctrl Pts',(-12.1451388796296,15.1604740551693,-325.318969897457)) ;
#27230=CARTESIAN_POINT('Ctrl Pts',(-12.236424730392,15.0868910594503,-325.31752086666)) ;
#27231=CARTESIAN_POINT('Ctrl Pts',(-12.4254476052965,14.9316807689751,-325.314512367915)) ;
#27232=CARTESIAN_POINT('Ctrl Pts',(-12.5230595077615,14.8499097436134,-325.312954199042)) ;
#27233=CARTESIAN_POINT('Ctrl Pts',(-12.7590220875803,14.6482589309166,-325.309175259915)) ;
#27234=CARTESIAN_POINT('Ctrl Pts',(-12.8964958303719,14.5273717434908,-325.306963164984)) ;
#27235=CARTESIAN_POINT('Ctrl Pts',(-13.4421571901979,14.0336954113039,-325.298130765579)) ;
#27236=CARTESIAN_POINT('Ctrl Pts',(-13.8360567781492,13.6455022312483,-325.291642829936)) ;
#27237=CARTESIAN_POINT('Ctrl Pts',(-14.6185895700435,12.8055355763361,-325.278228551828)) ;
#27238=CARTESIAN_POINT('Ctrl Pts',(-15.0040829844115,12.3516149349621,-325.271314446436)) ;
#27239=CARTESIAN_POINT('Ctrl Pts',(-15.4360989494827,11.7927870380293,-325.262829499861)) ;
#27240=CARTESIAN_POINT('Ctrl Pts',(-15.5033179036917,11.7042774585965,-325.261486037796)) ;
#27241=CARTESIAN_POINT('Ctrl Pts',(-15.6067066728022,11.5656883451552,-325.259379337861)) ;
#27242=CARTESIAN_POINT('Ctrl Pts',(-15.6434034935567,11.5160048280485,-325.258623482972)) ;
#27243=CARTESIAN_POINT('Ctrl Pts',(-15.7220145385164,11.4085048652786,-325.256985800007)) ;
#27244=CARTESIAN_POINT('Ctrl Pts',(-15.7638481627917,11.3506306210139,-325.256102767062)) ;
#27245=CARTESIAN_POINT('Ctrl Pts',(-15.8787043670023,11.1898744114611,-325.253647794848)) ;
#27246=CARTESIAN_POINT('Ctrl Pts',(-15.9510451857132,11.0865097812202,-325.25206682712)) ;
#27247=CARTESIAN_POINT('Ctrl Pts',(-16.1169345638572,10.8444925506724,-325.248366336661)) ;
#27248=CARTESIAN_POINT('Ctrl Pts',(-16.2097095479583,10.7053217920047,-325.246239300687)) ;
#27249=CARTESIAN_POINT('Ctrl Pts',(-16.5578352597424,10.168199205621,-325.238057219706)) ;
#27250=CARTESIAN_POINT('Ctrl Pts',(-16.8004225966218,9.76217108044045,-325.231932129668)) ;
#27251=CARTESIAN_POINT('Ctrl Pts',(-17.05376759195,9.30067275081635,-325.225152231068)) ;
#27252=CARTESIAN_POINT('Ctrl Pts',(-17.0793873382062,9.25354153018789,-325.224461827909)) ;
#27253=CARTESIAN_POINT('Ctrl Pts',(-17.3158714098972,8.81416703960838,-325.218045252925)) ;
#27254=CARTESIAN_POINT('Ctrl Pts',(-17.5133843011955,8.41488653451556,-325.212362892978)) ;
#27255=CARTESIAN_POINT('Ctrl Pts',(-17.7691101723148,7.84983667910317,-325.204576985564)) ;
#27256=CARTESIAN_POINT('Ctrl Pts',(-17.8390652671148,7.68953592407484,-325.202395545304)) ;
#27257=CARTESIAN_POINT('Ctrl Pts',(-17.9557145367167,7.41207392937469,-325.198667163691)) ;
#27258=CARTESIAN_POINT('Ctrl Pts',(-18.0034499688762,7.29536248076059,-325.197113083154)) ;
#27259=CARTESIAN_POINT('Ctrl Pts',(-18.1002543879553,7.05194135329516,-325.193900773564)) ;
#27260=CARTESIAN_POINT('Ctrl Pts',(-18.1491371029069,6.92516485281814,-325.19224390582)) ;
#27261=CARTESIAN_POINT('Ctrl Pts',(-18.2777432755427,6.58090986513966,-325.187786481361)) ;
#27262=CARTESIAN_POINT('Ctrl Pts',(-18.354913570991,6.36250123483369,-325.185003342196)) ;
#27263=CARTESIAN_POINT('Ctrl Pts',(-18.4790809710085,5.99000174850145,-325.18032220449)) ;
#27264=CARTESIAN_POINT('Ctrl Pts',(-18.5281008393189,5.83661150313104,-325.178413081954)) ;
#27265=CARTESIAN_POINT('Ctrl Pts',(-18.742259423375,5.13657637620256,-325.169770903708)) ;
#27266=CARTESIAN_POINT('Ctrl Pts',(-18.8851511305252,4.58342352960965,-325.163145314514)) ;
#27267=CARTESIAN_POINT('Ctrl Pts',(-19.0746222314727,3.68881403487805,-325.152423939428)) ;
#27268=CARTESIAN_POINT('Ctrl Pts',(-19.1368553128876,3.35101924194614,-325.148372066186)) ;
#27269=CARTESIAN_POINT('Ctrl Pts',(-19.2055552960972,2.91328104766467,-325.143035004805)) ;
#27270=CARTESIAN_POINT('Ctrl Pts',(-19.2202516871079,2.81469105580526,-325.141827260868)) ;
#27271=CARTESIAN_POINT('Ctrl Pts',(-19.2435055375327,2.65001130961778,-325.139797485778)) ;
#27272=CARTESIAN_POINT('Ctrl Pts',(-19.2524829186465,2.58398273798356,-325.138980265536)) ;
#27273=CARTESIAN_POINT('Ctrl Pts',(-19.27130514207,2.43999934238564,-325.137190069394)) ;
#27274=CARTESIAN_POINT('Ctrl Pts',(-19.2810170891532,2.36202850462239,-325.136215640312)) ;
#27275=CARTESIAN_POINT('Ctrl Pts',(-19.3096311085158,2.12035971438911,-325.13318228033)) ;
#27276=CARTESIAN_POINT('Ctrl Pts',(-19.3269234399747,1.95647874094133,-325.131106690573)) ;
#27277=CARTESIAN_POINT('Ctrl Pts',(-19.3541858703878,1.66228433565311,-325.127358746894)) ;
#27278=CARTESIAN_POINT('Ctrl Pts',(-19.3649300274119,1.53205251272656,-325.125691949031)) ;
#27279=CARTESIAN_POINT('Ctrl Pts',(-19.4149988140806,0.84001055586709,-325.116809074575)) ;
#27280=CARTESIAN_POINT('Ctrl Pts',(-19.4311909363592,0.276797040068225,
-325.109498680027)) ;
#27281=CARTESIAN_POINT('Ctrl Pts',(-19.417744045745,-0.63538152314059,-325.097792450297)) ;
#27282=CARTESIAN_POINT('Ctrl Pts',(-19.4031896511467,-0.9842386427811,-325.093345099064)) ;
#27283=CARTESIAN_POINT('Ctrl Pts',(-19.3662102197858,-1.52204406103101,
-325.086561579064)) ;
#27284=CARTESIAN_POINT('Ctrl Pts',(-19.3503984453435,-1.71137271484999,
-325.084187167638)) ;
#27285=CARTESIAN_POINT('Ctrl Pts',(-19.3204967723043,-2.01554111185302,
-325.080395597961)) ;
#27286=CARTESIAN_POINT('Ctrl Pts',(-19.30815376008,-2.13053981822835,-325.078967390448)) ;
#27287=CARTESIAN_POINT('Ctrl Pts',(-19.2798857624754,-2.37344517915201,
-325.075961609207)) ;
#27288=CARTESIAN_POINT('Ctrl Pts',(-19.263713242992,-2.50131748802154,-325.074385718642)) ;
#27289=CARTESIAN_POINT('Ctrl Pts',(-19.2202248084203,-2.81968337948499,
-325.070477084289)) ;
#27290=CARTESIAN_POINT('Ctrl Pts',(-19.1913485108284,-3.0099499233247,-325.068154550253)) ;
#27291=CARTESIAN_POINT('Ctrl Pts',(-19.1216056445185,-3.42755952841807,
-325.06308005832)) ;
#27292=CARTESIAN_POINT('Ctrl Pts',(-19.0795015650774,-3.65466646762184,
-325.060335697121)) ;
#27293=CARTESIAN_POINT('Ctrl Pts',(-18.9220424391497,-4.42689012892456,
-325.051029120634)) ;
#27294=CARTESIAN_POINT('Ctrl Pts',(-18.7872913964923,-4.96776889548514,
-325.044560511481)) ;
#27295=CARTESIAN_POINT('Ctrl Pts',(-18.5271474023991,-5.84858564806015,
-325.033800285075)) ;
#27296=CARTESIAN_POINT('Ctrl Pts',(-18.4151707174467,-6.19214269991828,
-325.029542713167)) ;
#27297=CARTESIAN_POINT('Ctrl Pts',(-18.2599377107106,-6.62686704863102,
-325.023983596761)) ;
#27298=CARTESIAN_POINT('Ctrl Pts',(-18.2254648371978,-6.72109540982123,
-325.022768069526)) ;
#27299=CARTESIAN_POINT('Ctrl Pts',(-18.1668533760571,-6.87753704346685,
-325.020729390357)) ;
#27300=CARTESIAN_POINT('Ctrl Pts',(-18.1431214584966,-6.93990065656124,
-325.019911150876)) ;
#27301=CARTESIAN_POINT('Ctrl Pts',(-18.0908635771359,-7.0751256054184,-325.01812405294)) ;
#27302=CARTESIAN_POINT('Ctrl Pts',(-18.0622178125445,-7.14793921145577,
-325.017153797515)) ;
#27303=CARTESIAN_POINT('Ctrl Pts',(-17.9725909710944,-7.3717790226332,-325.014148736918)) ;
#27304=CARTESIAN_POINT('Ctrl Pts',(-17.9101498348287,-7.52221276780784,
-325.012097695501)) ;
#27305=CARTESIAN_POINT('Ctrl Pts',(-17.795109040592,-7.78981440631045,-325.008403604915)) ;
#27306=CARTESIAN_POINT('Ctrl Pts',(-17.743225215228,-7.90727975761271,-325.006766128828)) ;
#27307=CARTESIAN_POINT('Ctrl Pts',(-17.4657653127215,-8.51896719920325,
-324.998169653473)) ;
#27308=CARTESIAN_POINT('Ctrl Pts',(-17.2206938810605,-9.00408036202466,
-324.991120432854)) ;
#27309=CARTESIAN_POINT('Ctrl Pts',(-16.7496251075442,-9.84677095407904,
-324.978720865924)) ;
#27310=CARTESIAN_POINT('Ctrl Pts',(-16.5316800765929,-10.2084472304841,
-324.973343686081)) ;
#27311=CARTESIAN_POINT('Ctrl Pts',(-16.2193087154888,-10.6905493119142,
-324.966139763965)) ;
#27312=CARTESIAN_POINT('Ctrl Pts',(-16.1349930409324,-10.8173850561086,
-324.964240601602)) ;
#27313=CARTESIAN_POINT('Ctrl Pts',(-15.9783236758234,-11.0471545362745,
-324.960793427597)) ;
#27314=CARTESIAN_POINT('Ctrl Pts',(-15.9064448121643,-11.1504019803719,
-324.959241880871)) ;
#27315=CARTESIAN_POINT('Ctrl Pts',(-15.7562692224957,-11.3617080546284,
-324.956060795673)) ;
#27316=CARTESIAN_POINT('Ctrl Pts',(-15.6778517224656,-11.469672844314,-324.954432325524)) ;
#27317=CARTESIAN_POINT('Ctrl Pts',(-15.4683656838477,-11.7519292506606,
-324.950165108696)) ;
#27318=CARTESIAN_POINT('Ctrl Pts',(-15.335463792758,-11.9248366246883,-324.947541132036)) ;
#27319=CARTESIAN_POINT('Ctrl Pts',(-15.1079328779118,-12.2107615919193,
-324.943177365538)) ;
#27320=CARTESIAN_POINT('Ctrl Pts',(-15.0148781504649,-12.3250058288699,
-324.941426910848)) ;
#27321=CARTESIAN_POINT('Ctrl Pts',(-14.611293800828,-12.8091356031988,-324.9339703778)) ;
#27322=CARTESIAN_POINT('Ctrl Pts',(-14.2883282720562,-13.1684295531974,
-324.928342984642)) ;
#27323=CARTESIAN_POINT('Ctrl Pts',(-13.8527552853799,-13.6180861125026,
-324.921027695776)) ;
#27324=CARTESIAN_POINT('Ctrl Pts',(-13.7520685835165,-13.7197561208005,
-324.919354151233)) ;
#27325=CARTESIAN_POINT('Ctrl Pts',(-13.4169969565866,-14.050705232608,-324.913828681741)) ;
#27326=CARTESIAN_POINT('Ctrl Pts',(-13.1779305257114,-14.2751627317519,
-324.909956315435)) ;
#27327=CARTESIAN_POINT('Ctrl Pts',(-12.8593247697737,-14.5594718658922,
-324.904812259717)) ;
#27328=CARTESIAN_POINT('Ctrl Pts',(-12.7848467594902,-14.6249153107428,
-324.90361084194)) ;
#27329=CARTESIAN_POINT('Ctrl Pts',(-12.6595332055423,-14.7333388885969,
-324.901588278773)) ;
#27330=CARTESIAN_POINT('Ctrl Pts',(-12.608971834638,-14.7766330762512,-324.900771861881)) ;
#27331=CARTESIAN_POINT('Ctrl Pts',(-12.5088695028484,-14.8614598149172,
-324.899154115393)) ;
#27332=CARTESIAN_POINT('Ctrl Pts',(-12.4593418784281,-14.9030065427896,
-324.898353179809)) ;
#27333=CARTESIAN_POINT('Ctrl Pts',(-12.3470059019273,-14.9962892609332,
-324.896536301882)) ;
#27334=CARTESIAN_POINT('Ctrl Pts',(-12.2840780040508,-15.0478793824886,
-324.895518366136)) ;
#27335=CARTESIAN_POINT('Ctrl Pts',(-12.1163758174103,-15.1836135178141,
-324.892807247386)) ;
#27336=CARTESIAN_POINT('Ctrl Pts',(-12.0110494255584,-15.2670682854659,
-324.89110623763)) ;
#27337=CARTESIAN_POINT('Ctrl Pts',(-11.6600185560434,-15.5393244653469,
-324.885453775664)) ;
#27338=CARTESIAN_POINT('Ctrl Pts',(-11.4106628089186,-15.7233397051941,
-324.881465738513)) ;
#27339=CARTESIAN_POINT('Ctrl Pts',(-10.5698958691711,-16.3132563050286,
-324.868220810446)) ;
#27340=CARTESIAN_POINT('Ctrl Pts',(-9.96041182877992,-16.6923705271283,
-324.858960304287)) ;
#27341=CARTESIAN_POINT('Ctrl Pts',(-9.17625143333914,-17.1218664623924,
-324.847726790361)) ;
#27342=CARTESIAN_POINT('Ctrl Pts',(-9.019988594336,-17.2047001547047,-324.845519004315)) ;
#27343=CARTESIAN_POINT('Ctrl Pts',(-8.75156815941257,-17.3423254858162,
-324.8417794228)) ;
#27344=CARTESIAN_POINT('Ctrl Pts',(-8.63997384254361,-17.3981910137934,
-324.840240006221)) ;
#27345=CARTESIAN_POINT('Ctrl Pts',(-8.42416522002516,-17.5036391147451,
-324.837291916696)) ;
#27346=CARTESIAN_POINT('Ctrl Pts',(-8.32003210973969,-17.553375961431,-324.835882181701)) ;
#27347=CARTESIAN_POINT('Ctrl Pts',(-8.07790275567883,-17.6663849333925,
-324.832632938715)) ;
#27348=CARTESIAN_POINT('Ctrl Pts',(-7.93959560311288,-17.7289732156982,
-324.830798283569)) ;
#27349=CARTESIAN_POINT('Ctrl Pts',(-7.24756956185587,-18.0324142997913,
-324.821717435721)) ;
#27350=CARTESIAN_POINT('Ctrl Pts',(-6.68356404261919,-18.2489781452747,
-324.814640938176)) ;
#27351=CARTESIAN_POINT('Ctrl Pts',(-5.58364637795645,-18.6134748534662,
-324.80110584276)) ;
#27352=CARTESIAN_POINT('Ctrl Pts',(-5.04966680747359,-18.7653780770332,
-324.794647447349)) ;
#27353=CARTESIAN_POINT('Ctrl Pts',(-4.39902852307145,-18.9206810315247,
-324.786617109329)) ;
#27354=CARTESIAN_POINT('Ctrl Pts',(-4.2879057954522,-18.9461733993227,-324.785239714493)) ;
#27355=CARTESIAN_POINT('Ctrl Pts',(-4.1157701721843,-18.9840705876446,-324.783092952287)) ;
#27356=CARTESIAN_POINT('Ctrl Pts',(-4.0549111575994,-18.997162832384,-324.782331435344)) ;
#27357=CARTESIAN_POINT('Ctrl Pts',(-3.93487736158078,-19.022381915437,-324.780823641292)) ;
#27358=CARTESIAN_POINT('Ctrl Pts',(-3.87570685362606,-19.0345257351029,
-324.780077582616)) ;
#27359=CARTESIAN_POINT('Ctrl Pts',(-3.74585696339403,-19.0605448135223,
-324.778434988017)) ;
#27360=CARTESIAN_POINT('Ctrl Pts',(-3.67515509241211,-19.074303342726,-324.777537136675)) ;
#27361=CARTESIAN_POINT('Ctrl Pts',(-3.49718704242215,-19.1079095529508,
-324.775269776329)) ;
#27362=CARTESIAN_POINT('Ctrl Pts',(-3.38982717854915,-19.1272474849493,
-324.77389531636)) ;
#27363=CARTESIAN_POINT('Ctrl Pts',(-3.06832164573027,-19.1823659712464,
-324.769764870065)) ;
#27364=CARTESIAN_POINT('Ctrl Pts',(-2.85373323831447,-19.2154617008725,
-324.766989080645)) ;
#27365=CARTESIAN_POINT('Ctrl Pts',(-1.76429229245401,-19.3648326843405,
-324.752866134105)) ;
#27366=CARTESIAN_POINT('Ctrl Pts',(-0.882788452479083,-19.4249883427977,
-324.741391833281)) ;
#27367=CARTESIAN_POINT('Ctrl Pts',(-0.000256543979532398,-19.4249999983059,
-324.730314803639)) ;
#27368=CARTESIAN_POINT('Ctrl Pts',(-0.000363249083131095,-19.4249999966036,
-324.51951242736)) ;
#27369=CARTESIAN_POINT('Ctrl Pts',(-0.368607332582545,-19.4249931104092,
-324.523887089415)) ;
#27370=CARTESIAN_POINT('Ctrl Pts',(-0.73677704384083,-19.4145148993854,
-324.528207924419)) ;
#27371=CARTESIAN_POINT('Ctrl Pts',(-1.74422720388531,-19.3571425948576,
-324.540005485921)) ;
#27372=CARTESIAN_POINT('Ctrl Pts',(-2.38183084770121,-19.2890687619575,
-324.547434282136)) ;
#27373=CARTESIAN_POINT('Ctrl Pts',(-3.1193991887729,-19.1731886686412,-324.556413841303)) ;
#27374=CARTESIAN_POINT('Ctrl Pts',(-3.2237642527278,-19.155917075924,-324.557693900277)) ;
#27375=CARTESIAN_POINT('Ctrl Pts',(-3.39389086251675,-19.126332764801,-324.559799404865)) ;
#27376=CARTESIAN_POINT('Ctrl Pts',(-3.45973917404293,-19.1145312543628,
-324.560619007596)) ;
#27377=CARTESIAN_POINT('Ctrl Pts',(-3.59984144819257,-19.0886740650673,
-324.56237375461)) ;
#27378=CARTESIAN_POINT('Ctrl Pts',(-3.67407688585795,-19.0745247655761,
-324.563309926414)) ;
#27379=CARTESIAN_POINT('Ctrl Pts',(-3.89330097014754,-19.0314133133711,
-324.566091477331)) ;
#27380=CARTESIAN_POINT('Ctrl Pts',(-4.03804352861184,-19.0012286312902,
-324.567949935994)) ;
#27381=CARTESIAN_POINT('Ctrl Pts',(-4.38714467628392,-18.9242577974208,
-324.572474247856)) ;
#27382=CARTESIAN_POINT('Ctrl Pts',(-4.59111793609637,-18.8758101150869,
-324.575152592198)) ;
#27383=CARTESIAN_POINT('Ctrl Pts',(-5.63482349233041,-18.6099907333345,
-324.58897734174)) ;
#27384=CARTESIAN_POINT('Ctrl Pts',(-6.46010429753605,-18.3398489056761,
-324.600261335798)) ;
#27385=CARTESIAN_POINT('Ctrl Pts',(-7.43744471109511,-17.9457457261627,
-324.613514878287)) ;
#27386=CARTESIAN_POINT('Ctrl Pts',(-7.60931543644837,-17.8735472763722,
-324.615843637309)) ;
#27387=CARTESIAN_POINT('Ctrl Pts',(-7.89612842799482,-17.7481776540722,
-324.61972551927)) ;
#27388=CARTESIAN_POINT('Ctrl Pts',(-8.01163789221662,-17.6963361328111,
-324.621287731253)) ;
#27389=CARTESIAN_POINT('Ctrl Pts',(-8.24659723913017,-17.5881125713985,
-324.62446345231)) ;
#27390=CARTESIAN_POINT('Ctrl Pts',(-8.3659955044135,-17.5316339547681,-324.626076174751)) ;
#27391=CARTESIAN_POINT('Ctrl Pts',(-8.67419904665552,-17.3819797981122,
-324.630237757478)) ;
#27392=CARTESIAN_POINT('Ctrl Pts',(-8.86208210442236,-17.286944547256,-324.632773246298)) ;
#27393=CARTESIAN_POINT('Ctrl Pts',(-9.17226337590775,-17.1236622363684,
-324.636963555373)) ;
#27394=CARTESIAN_POINT('Ctrl Pts',(-9.29543490974306,-17.0571132877477,
-324.638628733178)) ;
#27395=CARTESIAN_POINT('Ctrl Pts',(-9.80463915371254,-16.7748391550134,
-324.645525181517)) ;
#27396=CARTESIAN_POINT('Ctrl Pts',(-10.1839681700064,-16.5472949560962,
-324.650689497295)) ;
#27397=CARTESIAN_POINT('Ctrl Pts',(-10.625255237654,-16.2616585880031,-324.656828940282)) ;
#27398=CARTESIAN_POINT('Ctrl Pts',(-10.6950173349779,-16.2158623915263,
-324.657803659373)) ;
#27399=CARTESIAN_POINT('Ctrl Pts',(-10.8248997979754,-16.129396684843,-324.659627526123)) ;
#27400=CARTESIAN_POINT('Ctrl Pts',(-10.8850915333987,-16.0888369797221,
-324.660476480876)) ;
#27401=CARTESIAN_POINT('Ctrl Pts',(-11.2550270070968,-15.8365327147582,
-324.665720257567)) ;
#27402=CARTESIAN_POINT('Ctrl Pts',(-11.5588086445539,-15.6161884836158,
-324.670138444608)) ;
#27403=CARTESIAN_POINT('Ctrl Pts',(-11.935321334371,-15.3260807985454,-324.675862941955)) ;
#27404=CARTESIAN_POINT('Ctrl Pts',(-12.0141520293376,-15.2643636937481,
-324.677075863568)) ;
#27405=CARTESIAN_POINT('Ctrl Pts',(-12.1446980500494,-15.1605205243333,
-324.679111558303)) ;
#27406=CARTESIAN_POINT('Ctrl Pts',(-12.1966798830382,-15.118732524105,-324.679929452985)) ;
#27407=CARTESIAN_POINT('Ctrl Pts',(-12.3092596274258,-15.0272715994966,
-324.681717570718)) ;
#27408=CARTESIAN_POINT('Ctrl Pts',(-12.3697741618878,-14.9774981710467,
-324.682689209409)) ;
#27409=CARTESIAN_POINT('Ctrl Pts',(-12.5556320198291,-14.8227346670844,
-324.685703624531)) ;
#27410=CARTESIAN_POINT('Ctrl Pts',(-12.6799520714954,-14.7165272312688,
-324.687762776328)) ;
#27411=CARTESIAN_POINT('Ctrl Pts',(-12.9000485408463,-14.5236377557519,
-324.691474628817)) ;
#27412=CARTESIAN_POINT('Ctrl Pts',(-12.9963293755352,-14.4375458001215,
-324.693121761559)) ;
#27413=CARTESIAN_POINT('Ctrl Pts',(-13.4978614919641,-13.9800056309785,
-324.701811295967)) ;
#27414=CARTESIAN_POINT('Ctrl Pts',(-13.8880682228419,-13.59243849508,-324.708945253904)) ;
#27415=CARTESIAN_POINT('Ctrl Pts',(-14.5520398094792,-12.8744752783496,
-324.721501728454)) ;
#27416=CARTESIAN_POINT('Ctrl Pts',(-14.8322947178448,-12.5505781281214,
-324.726952310985)) ;
#27417=CARTESIAN_POINT('Ctrl Pts',(-15.2033110505697,-12.0919849506846,
-324.734342000055)) ;
#27418=CARTESIAN_POINT('Ctrl Pts',(-15.303432133127,-11.9650211866163,-324.736355277088)) ;
#27419=CARTESIAN_POINT('Ctrl Pts',(-15.4779915321134,-11.7378862140117,
-324.739899488485)) ;
#27420=CARTESIAN_POINT('Ctrl Pts',(-15.5530715046046,-11.6382198579215,
-324.741435557541)) ;
#27421=CARTESIAN_POINT('Ctrl Pts',(-15.7106097808053,-11.4248453790538,
-324.744684270358)) ;
#27422=CARTESIAN_POINT('Ctrl Pts',(-15.7928056676612,-11.3109522512111,
-324.746394754798)) ;
#27423=CARTESIAN_POINT('Ctrl Pts',(-16.0223502412724,-10.9855076750169,
-324.751218228642)) ;
#27424=CARTESIAN_POINT('Ctrl Pts',(-16.1667328223465,-10.7719003119683,
-324.754308198409)) ;
#27425=CARTESIAN_POINT('Ctrl Pts',(-16.5001278919634,-10.2568491186854,
-324.761601200645)) ;
#27426=CARTESIAN_POINT('Ctrl Pts',(-16.6851947927748,-9.95296184527758,
-324.765779071058)) ;
#27427=CARTESIAN_POINT('Ctrl Pts',(-17.1546116698316,-9.13223553285217,
-324.776837972113)) ;
#27428=CARTESIAN_POINT('Ctrl Pts',(-17.4239446690138,-8.60723973028282,
-324.783677291709)) ;
#27429=CARTESIAN_POINT('Ctrl Pts',(-17.7300154118263,-7.9371759473243,-324.792468037807)) ;
#27430=CARTESIAN_POINT('Ctrl Pts',(-17.7895377357261,-7.80285560307284,
-324.794233806537)) ;
#27431=CARTESIAN_POINT('Ctrl Pts',(-17.8772934261257,-7.59859787440915,
-324.796932587157)) ;
#27432=CARTESIAN_POINT('Ctrl Pts',(-17.9066527183147,-7.52914990606029,
-324.797852542709)) ;
#27433=CARTESIAN_POINT('Ctrl Pts',(-17.9616335713812,-7.39695463453026,
-324.799609647532)) ;
#27434=CARTESIAN_POINT('Ctrl Pts',(-17.9873324856987,-7.33424082155586,
-324.800445875654)) ;
#27435=CARTESIAN_POINT('Ctrl Pts',(-18.0527738100199,-7.17212952202171,
-324.802613251178)) ;
#27436=CARTESIAN_POINT('Ctrl Pts',(-18.0920237353459,-7.07253570007065,
-324.803950295831)) ;
#27437=CARTESIAN_POINT('Ctrl Pts',(-18.3095247827385,-6.50698214795709,
-324.811563596741)) ;
#27438=CARTESIAN_POINT('Ctrl Pts',(-18.4705961028508,-6.03461620884636,
-324.817996869729)) ;
#27439=CARTESIAN_POINT('Ctrl Pts',(-18.7988848052937,-4.93492142458627,
-324.832803259053)) ;
#27440=CARTESIAN_POINT('Ctrl Pts',(-18.9532062671738,-4.30435790939297,
-324.841161715128)) ;
#27441=CARTESIAN_POINT('Ctrl Pts',(-19.110964143209,-3.48376084504112,-324.851671915868)) ;
#27442=CARTESIAN_POINT('Ctrl Pts',(-19.1435912961154,-3.29976552958719,
-324.854006385731)) ;
#27443=CARTESIAN_POINT('Ctrl Pts',(-19.1938751866936,-2.9902889221362,-324.85789486167)) ;
#27444=CARTESIAN_POINT('Ctrl Pts',(-19.2129679622242,-2.8650540400479,-324.859458028139)) ;
#27445=CARTESIAN_POINT('Ctrl Pts',(-19.2494470467824,-2.60899013884006,
-324.862633419556)) ;
#27446=CARTESIAN_POINT('Ctrl Pts',(-19.2667278168091,-2.47815262636089,
-324.864244881386)) ;
#27447=CARTESIAN_POINT('Ctrl Pts',(-19.3080403099529,-2.13875563626868,
-324.868397977124)) ;
#27448=CARTESIAN_POINT('Ctrl Pts',(-19.3300267363531,-1.9299644699258,-324.870926349816)) ;
#27449=CARTESIAN_POINT('Ctrl Pts',(-19.3609751410651,-1.58199320377107,
-324.875102796553)) ;
#27450=CARTESIAN_POINT('Ctrl Pts',(-19.3718304014805,-1.44299960345173,
-324.876761201998)) ;
#27451=CARTESIAN_POINT('Ctrl Pts',(-19.4106652614121,-0.86575818283232,
-324.883614974356)) ;
#27452=CARTESIAN_POINT('Ctrl Pts',(-19.4252761978651,-0.426741381569603,
-324.888744235974)) ;
#27453=CARTESIAN_POINT('Ctrl Pts',(-19.4249037842933,0.157013435474684,
-324.895562093413)) ;
#27454=CARTESIAN_POINT('Ctrl Pts',(-19.4231964476866,0.301628892196292,
-324.897251231417)) ;
#27455=CARTESIAN_POINT('Ctrl Pts',(-19.4116346715268,0.804816558384056,
-324.903142417549)) ;
#27456=CARTESIAN_POINT('Ctrl Pts',(-19.3934636536477,1.16312371228953,-324.907360757565)) ;
#27457=CARTESIAN_POINT('Ctrl Pts',(-19.356245472028,1.6370728455232,-324.913064801735)) ;
#27458=CARTESIAN_POINT('Ctrl Pts',(-19.3460601909795,1.75334004201231,-324.914474164533)) ;
#27459=CARTESIAN_POINT('Ctrl Pts',(-19.3287914436211,1.93193687836117,-324.916658834579)) ;
#27460=CARTESIAN_POINT('Ctrl Pts',(-19.3224528243252,1.99433588287526,-324.917425843237)) ;
#27461=CARTESIAN_POINT('Ctrl Pts',(-19.3083942515218,2.12636892063776,-324.919057622037)) ;
#27462=CARTESIAN_POINT('Ctrl Pts',(-19.3005995602904,2.19599406817172,-324.919923355672)) ;
#27463=CARTESIAN_POINT('Ctrl Pts',(-19.2785061742896,2.38412952436164,-324.922275428641)) ;
#27464=CARTESIAN_POINT('Ctrl Pts',(-19.2634914820184,2.50255264880877,-324.923769647723)) ;
#27465=CARTESIAN_POINT('Ctrl Pts',(-19.1926066687591,3.02313106842967,-324.930387438392)) ;
#27466=CARTESIAN_POINT('Ctrl Pts',(-19.1252275133483,3.4236156079509,-324.935606281046)) ;
#27467=CARTESIAN_POINT('Ctrl Pts',(-18.8999474976657,4.54629511324837,-324.950369269271)) ;
#27468=CARTESIAN_POINT('Ctrl Pts',(-18.7133120267843,5.26201255935657,-324.959917939432)) ;
#27469=CARTESIAN_POINT('Ctrl Pts',(-18.4318193692617,6.13434528246556,-324.971429891259)) ;
#27470=CARTESIAN_POINT('Ctrl Pts',(-18.3749724260403,6.30258246921978,-324.973645623024)) ;
#27471=CARTESIAN_POINT('Ctrl Pts',(-18.27369742355,6.58927962630996,-324.977413147375)) ;
#27472=CARTESIAN_POINT('Ctrl Pts',(-18.2304042300151,6.70812829191659,-324.978972488328)) ;
#27473=CARTESIAN_POINT('Ctrl Pts',(-18.1385320812043,6.95287617442221,-324.982178996623)) ;
#27474=CARTESIAN_POINT('Ctrl Pts',(-18.0897957378861,7.07870916042882,-324.983824978575)) ;
#27475=CARTESIAN_POINT('Ctrl Pts',(-17.9557823515233,7.41429496806485,-324.988209387055)) ;
#27476=CARTESIAN_POINT('Ctrl Pts',(-17.8681424591935,7.62308172809699,-324.990931432654)) ;
#27477=CARTESIAN_POINT('Ctrl Pts',(-17.7141100294958,7.97277698637304,-324.995489894093)) ;
#27478=CARTESIAN_POINT('Ctrl Pts',(-17.6496364976262,8.11450544260688,-324.997337273074)) ;
#27479=CARTESIAN_POINT('Ctrl Pts',(-17.3563169390301,8.73925376450783,-325.005491493212)) ;
#27480=CARTESIAN_POINT('Ctrl Pts',(-17.1092963951651,9.21348309503388,-325.011703415862)) ;
#27481=CARTESIAN_POINT('Ctrl Pts',(-16.6633549071506,9.9896606498155,-325.022180284475)) ;
#27482=CARTESIAN_POINT('Ctrl Pts',(-16.4749992001847,10.2973354291511,-325.026421402697)) ;
#27483=CARTESIAN_POINT('Ctrl Pts',(-16.2144236414078,10.6975112079814,-325.032150801032)) ;
#27484=CARTESIAN_POINT('Ctrl Pts',(-16.1497774817049,10.7948583733239,-325.033561874647)) ;
#27485=CARTESIAN_POINT('Ctrl Pts',(-16.0490756956369,10.9435703164506,-325.03574857723)) ;
#27486=CARTESIAN_POINT('Ctrl Pts',(-16.013642925308,10.9953536643952,-325.03651588339)) ;
#27487=CARTESIAN_POINT('Ctrl Pts',(-15.9381345061251,11.1045665171004,-325.038147572487)) ;
#27488=CARTESIAN_POINT('Ctrl Pts',(-15.8979979536569,11.1619527910017,-325.039012912954)) ;
#27489=CARTESIAN_POINT('Ctrl Pts',(-15.7886994689323,11.3164396223703,-325.041362625346)) ;
#27490=CARTESIAN_POINT('Ctrl Pts',(-15.7189525725689,11.4131225615677,-325.042854851139)) ;
#27491=CARTESIAN_POINT('Ctrl Pts',(-15.4197721690338,11.8199004576638,-325.049215118221)) ;
#27492=CARTESIAN_POINT('Ctrl Pts',(-15.1820190343417,12.123766648707,-325.05416858626)) ;
#27493=CARTESIAN_POINT('Ctrl Pts',(-14.4451991957954,13.0097868472777,-325.069020313278)) ;
#27494=CARTESIAN_POINT('Ctrl Pts',(-13.9205544390007,13.569690764296,-325.078934043954)) ;
#27495=CARTESIAN_POINT('Ctrl Pts',(-13.2374997315169,14.2172326559511,-325.090748781695)) ;
#27496=CARTESIAN_POINT('Ctrl Pts',(-13.1091891076168,14.3356292015037,-325.092926245476)) ;
#27497=CARTESIAN_POINT('Ctrl Pts',(-12.8855190659725,14.5365027320809,-325.096650100929)) ;
#27498=CARTESIAN_POINT('Ctrl Pts',(-12.7909206778261,14.6198105850174,-325.098203584598)) ;
#27499=CARTESIAN_POINT('Ctrl Pts',(-12.5925957493675,14.7910665270515,-325.101416648189)) ;
#27500=CARTESIAN_POINT('Ctrl Pts',(-12.4887429276944,14.878858049614,-325.103074845725)) ;
#27501=CARTESIAN_POINT('Ctrl Pts',(-12.2050376314705,15.1136238515859,-325.107541206289)) ;
#27502=CARTESIAN_POINT('Ctrl Pts',(-12.0234570239237,15.2584747262203,-325.110331823123)) ;
#27503=CARTESIAN_POINT('Ctrl Pts',(-11.7111393562844,15.4985800011832,-325.115028052145)) ;
#27504=CARTESIAN_POINT('Ctrl Pts',(-11.5817308258968,15.5955210949443,-325.116944806609)) ;
#27505=CARTESIAN_POINT('Ctrl Pts',(-10.9860200675328,16.0302691146094,-325.125650132465)) ;
#27506=CARTESIAN_POINT('Ctrl Pts',(-10.5060515857835,16.3488545200602,-325.132329538069)) ;
#27507=CARTESIAN_POINT('Ctrl Pts',(-9.88787461375091,16.720698555901,-325.140789654089)) ;
#27508=CARTESIAN_POINT('Ctrl Pts',(-9.7622667993393,16.7943434364832,-325.142502173436)) ;
#27509=CARTESIAN_POINT('Ctrl Pts',(-9.44690652593406,16.9745082384834,-325.146797016947)) ;
#27510=CARTESIAN_POINT('Ctrl Pts',(-9.25616996445633,17.0792649177425,-325.149390325727)) ;
#27511=CARTESIAN_POINT('Ctrl Pts',(-8.98662443584238,17.2214634400773,-325.153072967232)) ;
#27512=CARTESIAN_POINT('Ctrl Pts',(-8.90926189738624,17.2616127342032,-325.154131972869)) ;
#27513=CARTESIAN_POINT('Ctrl Pts',(-8.77314327357809,17.3310961686683,-325.156000933056)) ;
#27514=CARTESIAN_POINT('Ctrl Pts',(-8.71450391206616,17.3606554848438,-325.15680801149)) ;
#27515=CARTESIAN_POINT('Ctrl Pts',(-8.57869231175896,17.4282548065239,-325.158681898262)) ;
#27516=CARTESIAN_POINT('Ctrl Pts',(-8.50141520428343,17.4660804669774,-325.159751370941)) ;
#27517=CARTESIAN_POINT('Ctrl Pts',(-8.23098669893119,17.5962300917132,-325.16350179842)) ;
#27518=CARTESIAN_POINT('Ctrl Pts',(-8.03656266261235,17.685873339037,-325.166211900098)) ;
#27519=CARTESIAN_POINT('Ctrl Pts',(-7.49531398524474,17.924659014154,-325.173756756317)) ;
#27520=CARTESIAN_POINT('Ctrl Pts',(-7.14556263465918,18.0669329663617,-325.178631325225)) ;
#27521=CARTESIAN_POINT('Ctrl Pts',(-6.65250779134534,18.2509423844661,-325.185420995463)) ;
#27522=CARTESIAN_POINT('Ctrl Pts',(-6.51253389172983,18.3013567847367,-325.187339703212)) ;
#27523=CARTESIAN_POINT('Ctrl Pts',(-5.9095715038718,18.510732261236,-325.195555919158)) ;
#27524=CARTESIAN_POINT('Ctrl Pts',(-5.44124290075414,18.653769653589,-325.201809566647)) ;
#27525=CARTESIAN_POINT('Ctrl Pts',(-4.8188103906079,18.8184353860043,-325.209886926799)) ;
#27526=CARTESIAN_POINT('Ctrl Pts',(-4.66914407922479,18.8561273227786,-325.211812143026)) ;
#27527=CARTESIAN_POINT('Ctrl Pts',(-4.39626426216751,18.9214011917838,-325.215290999131)) ;
#27528=CARTESIAN_POINT('Ctrl Pts',(-4.27320066601249,18.949573046387,-325.216848421088)) ;
#27529=CARTESIAN_POINT('Ctrl Pts',(-4.02027991853283,19.0048828300569,-325.220026146259)) ;
#27530=CARTESIAN_POINT('Ctrl Pts',(-3.8904017388695,19.0318941877486,-325.221645540904)) ;
#27531=CARTESIAN_POINT('Ctrl Pts',(-3.55056662750564,19.0989471826183,-325.225851951702)) ;
#27532=CARTESIAN_POINT('Ctrl Pts',(-3.34020749841544,19.1368576558235,-325.2284250089)) ;
#27533=CARTESIAN_POINT('Ctrl Pts',(-2.98804172153173,19.1943404986764,-325.232688713624)) ;
#27534=CARTESIAN_POINT('Ctrl Pts',(-2.84656752583494,19.2158308142655,-325.234389853303)) ;
#27535=CARTESIAN_POINT('Ctrl Pts',(-2.2504064075521,19.2996610295794,-325.241517168713)) ;
#27536=CARTESIAN_POINT('Ctrl Pts',(-1.79382180773071,19.3474403621072,-325.246871687205)) ;
#27537=CARTESIAN_POINT('Ctrl Pts',(-0.868674254276153,19.4112193736203,
-325.25770378038)) ;
#27538=CARTESIAN_POINT('Ctrl Pts',(-0.400362562262684,19.4265215652412,
-325.263178244891)) ;
#27539=CARTESIAN_POINT('Ctrl Pts',(0.187025652032619,19.4244640529543,-325.270222623098)) ;
#27540=CARTESIAN_POINT('Ctrl Pts',(0.306003078054853,19.4229540593874,-325.271658875818)) ;
#27541=CARTESIAN_POINT('Ctrl Pts',(0.48806508791664,19.4189701519047,-325.273875531531)) ;
#27542=CARTESIAN_POINT('Ctrl Pts',(0.551164070730255,19.4172816698578,-325.274647252462)) ;
#27543=CARTESIAN_POINT('Ctrl Pts',(0.683820183459702,19.4130847446476,-325.276277947389)) ;
#27544=CARTESIAN_POINT('Ctrl Pts',(0.753374275789827,19.4105099499722,-325.277137792633)) ;
#27545=CARTESIAN_POINT('Ctrl Pts',(0.939823431378142,19.4026041952801,-325.279454329519)) ;
#27546=CARTESIAN_POINT('Ctrl Pts',(1.0566866429843,19.3965907035092,-325.280918513096)) ;
#27547=CARTESIAN_POINT('Ctrl Pts',(1.76202815745998,19.3539021846119,-325.28981532353)) ;
#27548=CARTESIAN_POINT('Ctrl Pts',(2.34864076285009,19.2915048356768,-325.297455202503)) ;
#27549=CARTESIAN_POINT('Ctrl Pts',(3.18749649349097,19.163443076039,-325.308396900876)) ;
#27550=CARTESIAN_POINT('Ctrl Pts',(3.44268206259244,19.1192474967462,-325.311729299308)) ;
#27551=CARTESIAN_POINT('Ctrl Pts',(4.04014302449614,19.0034235689134,-325.319513271679)) ;
#27552=CARTESIAN_POINT('Ctrl Pts',(4.38151981789101,18.9276292228183,-325.323946111349)) ;
#27553=CARTESIAN_POINT('Ctrl Pts',(4.87405700639025,18.8042335430064,-325.330300306474)) ;
#27554=CARTESIAN_POINT('Ctrl Pts',(5.02697389711931,18.7639325402317,-325.332267429082)) ;
#27555=CARTESIAN_POINT('Ctrl Pts',(5.2990908966547,18.6886513080914,-325.335757626753)) ;
#27556=CARTESIAN_POINT('Ctrl Pts',(5.41847970892812,18.654386340405,-325.33728535688)) ;
#27557=CARTESIAN_POINT('Ctrl Pts',(5.67589511557756,18.5778275766727,-325.340572153735)) ;
#27558=CARTESIAN_POINT('Ctrl Pts',(5.81379556488206,18.5351353928778,-325.342328434714)) ;
#27559=CARTESIAN_POINT('Ctrl Pts',(6.21907285743305,18.4046989119538,-325.347479281235)) ;
#27560=CARTESIAN_POINT('Ctrl Pts',(6.48503361034648,18.3126772689196,-325.350845206379)) ;
#27561=CARTESIAN_POINT('Ctrl Pts',(7.13392445866303,18.0722533307277,-325.359051446528)) ;
#27562=CARTESIAN_POINT('Ctrl Pts',(7.51432768800239,17.917424438839,-325.363855706064)) ;
#27563=CARTESIAN_POINT('Ctrl Pts',(8.39559008253239,17.5257345362505,-325.375120538798)) ;
#27564=CARTESIAN_POINT('Ctrl Pts',(8.89179086982165,17.2792753108281,-325.381566145849)) ;
#27565=CARTESIAN_POINT('Ctrl Pts',(9.47673183865562,16.9568630366151,-325.389584211315)) ;
#27566=CARTESIAN_POINT('Ctrl Pts',(9.57619557678084,16.9008913553037,-325.39096304451)) ;
#27567=CARTESIAN_POINT('Ctrl Pts',(9.72915810139678,16.8130302272867,-325.393111509246)) ;
#27568=CARTESIAN_POINT('Ctrl Pts',(9.78300656109073,16.781754538799,-325.393873270373)) ;
#27569=CARTESIAN_POINT('Ctrl Pts',(9.89761917857128,16.7144473439642,-325.395507171316)) ;
#27570=CARTESIAN_POINT('Ctrl Pts',(9.95833904811313,16.6783422078526,-325.396380383355)) ;
#27571=CARTESIAN_POINT('Ctrl Pts',(10.1236531178821,16.5788188393363,-325.398777090183)) ;
#27572=CARTESIAN_POINT('Ctrl Pts',(10.2278473510381,16.514742657855,-325.400308957564)) ;
#27573=CARTESIAN_POINT('Ctrl Pts',(10.4670981303155,16.3644782456107,-325.403869645579)) ;
#27574=CARTESIAN_POINT('Ctrl Pts',(10.6017075145806,16.2775946991318,-325.405905253548)) ;
#27575=CARTESIAN_POINT('Ctrl Pts',(11.0954299089653,15.950199345179,-325.413471488027)) ;
#27576=CARTESIAN_POINT('Ctrl Pts',(11.4475610480983,15.6993875639636,-325.419063631053)) ;
#27577=CARTESIAN_POINT('Ctrl Pts',(11.864998600235,15.3805427780386,-325.42583542734)) ;
#27578=CARTESIAN_POINT('Ctrl Pts',(11.9385581588302,15.3235151654231,-325.427034444693)) ;
#27579=CARTESIAN_POINT('Ctrl Pts',(12.3822719068559,14.9743882006204,-325.434298155488)) ;
#27580=CARTESIAN_POINT('Ctrl Pts',(12.7421001938579,14.6694186779427,-325.440316871328)) ;
#27581=CARTESIAN_POINT('Ctrl Pts',(13.2038260649252,14.2482679740031,-325.448155735435)) ;
#27582=CARTESIAN_POINT('Ctrl Pts',(13.3159484470554,14.1435384558895,-325.450069266996)) ;
#27583=CARTESIAN_POINT('Ctrl Pts',(13.5179038621064,13.9503687091569,-325.45353389443)) ;
#27584=CARTESIAN_POINT('Ctrl Pts',(13.6081391772843,13.8623612753066,-325.455088661402)) ;
#27585=CARTESIAN_POINT('Ctrl Pts',(13.7918132126998,13.6797003278597,-325.458267771821)) ;
#27586=CARTESIAN_POINT('Ctrl Pts',(13.8851492632979,13.5849528061858,-325.459891136017)) ;
#27587=CARTESIAN_POINT('Ctrl Pts',(14.1272444060979,13.3340948991893,-325.464124160004)) ;
#27588=CARTESIAN_POINT('Ctrl Pts',(14.2743900060806,13.1764529164931,-325.466719507893)) ;
#27589=CARTESIAN_POINT('Ctrl Pts',(14.5160062522204,12.908803066421,-325.471026932218)) ;
#27590=CARTESIAN_POINT('Ctrl Pts',(14.6119246120961,12.8001286441634,-325.472749577824)) ;
#27591=CARTESIAN_POINT('Ctrl Pts',(15.0131750363146,12.3351282602621,-325.480018573662)) ;
#27592=CARTESIAN_POINT('Ctrl Pts',(15.3067589266248,11.9688740228255,-325.485490289447)) ;
#27593=CARTESIAN_POINT('Ctrl Pts',(15.6612775639348,11.4921968623271,-325.492430264243)) ;
#27594=CARTESIAN_POINT('Ctrl Pts',(15.7347966678068,11.3913290474519,-325.493889231992)) ;
#27595=CARTESIAN_POINT('Ctrl Pts',(16.0188763503328,10.9935753474814,-325.499615163043)) ;
#27596=CARTESIAN_POINT('Ctrl Pts',(16.222047524525,10.6915046346124,-325.503903694146)) ;
#27597=CARTESIAN_POINT('Ctrl Pts',(16.4703263920015,10.2989839564173,-325.50949683315)) ;
#27598=CARTESIAN_POINT('Ctrl Pts',(16.523381616473,10.2136468467653,-325.510714125339)) ;
#27599=CARTESIAN_POINT('Ctrl Pts',(16.6105731091213,10.0709453947153,-325.512754828303)) ;
#27600=CARTESIAN_POINT('Ctrl Pts',(16.645080146972,10.0138098177995,-325.513573303581)) ;
#27601=CARTESIAN_POINT('Ctrl Pts',(16.7193601196066,9.8893747573778,-325.5153597214)) ;
#27602=CARTESIAN_POINT('Ctrl Pts',(16.7590225866423,9.82201088478792,-325.516329048357)) ;
#27603=CARTESIAN_POINT('Ctrl Pts',(16.8798520113859,9.61392794712047,-325.519327842514)) ;
#27604=CARTESIAN_POINT('Ctrl Pts',(16.9596611716917,9.47242879616766,-325.521373453081)) ;
#27605=CARTESIAN_POINT('Ctrl Pts',(17.0991234205372,9.21775271055658,-325.525055666434)) ;
#27606=CARTESIAN_POINT('Ctrl Pts',(17.1594511820689,9.10495589591066,-325.526686692969)) ;
#27607=CARTESIAN_POINT('Ctrl Pts',(17.4681559887362,8.51379302888635,-325.535221679839)) ;
#27608=CARTESIAN_POINT('Ctrl Pts',(17.6976576210753,8.02583708176584,-325.542214977713)) ;
#27609=CARTESIAN_POINT('Ctrl Pts',(18.0757390442214,7.12662492662806,-325.554745917007)) ;
#27610=CARTESIAN_POINT('Ctrl Pts',(18.2313002038026,6.71869179542986,-325.560305374599)) ;
#27611=CARTESIAN_POINT('Ctrl Pts',(18.4261308783734,6.15102633449882,-325.567826863017)) ;
#27612=CARTESIAN_POINT('Ctrl Pts',(18.4773141747127,5.99552208808988,-325.569865970646)) ;
#27613=CARTESIAN_POINT('Ctrl Pts',(18.5641060972116,5.72015891252125,-325.573438999226)) ;
#27614=CARTESIAN_POINT('Ctrl Pts',(18.6005345804788,5.60056841232328,-325.574978346069)) ;
#27615=CARTESIAN_POINT('Ctrl Pts',(18.6751297821451,5.34692228588037,-325.57821753599)) ;
#27616=CARTESIAN_POINT('Ctrl Pts',(18.7130132387495,5.2127906059857,-325.57991539965)) ;
#27617=CARTESIAN_POINT('Ctrl Pts',(18.8152065044151,4.83548292998529,-325.584651387391)) ;
#27618=CARTESIAN_POINT('Ctrl Pts',(18.876241449477,4.59144857723551,-325.587667894214)) ;
#27619=CARTESIAN_POINT('Ctrl Pts',(19.0090923937612,4.01274840202132,-325.594730464643)) ;
#27620=CARTESIAN_POINT('Ctrl Pts',(19.0768366527529,3.6772336271874,-325.598753748592)) ;
#27621=CARTESIAN_POINT('Ctrl Pts',(19.2500629795013,2.68480841869195,-325.61054389156)) ;
#27622=CARTESIAN_POINT('Ctrl Pts',(19.3307073497453,2.0240721052377,-325.618240613138)) ;
#27623=CARTESIAN_POINT('Ctrl Pts',(19.3854783679516,1.24398464233931,-325.62762311095)) ;
#27624=CARTESIAN_POINT('Ctrl Pts',(19.3926083448609,1.12739117805713,-325.629033641919)) ;
#27625=CARTESIAN_POINT('Ctrl Pts',(19.401950651708,0.948088526546092,-325.631219699773)) ;
#27626=CARTESIAN_POINT('Ctrl Pts',(19.4049115071287,0.885420993089332,-325.631986911533)) ;
#27627=CARTESIAN_POINT('Ctrl Pts',(19.4105351865448,0.752764370559301,-325.633618628765)) ;
#27628=CARTESIAN_POINT('Ctrl Pts',(19.4131231744416,0.68277303308811,-325.634484093655)) ;
#27629=CARTESIAN_POINT('Ctrl Pts',(19.419094737144,0.493566636258129,-325.636834553257)) ;
#27630=CARTESIAN_POINT('Ctrl Pts',(19.4217590336872,0.374331950196478,-325.638327410027)) ;
#27631=CARTESIAN_POINT('Ctrl Pts',(19.428644258307,-0.149949519781678,-325.644931770118)) ;
#27632=CARTESIAN_POINT('Ctrl Pts',(19.4212930891236,-0.555046297710654,
-325.650138132174)) ;
#27633=CARTESIAN_POINT('Ctrl Pts',(19.3646787539922,-1.69966175390807,-325.664913171771)) ;
#27634=CARTESIAN_POINT('Ctrl Pts',(19.2857620517131,-2.43701128522958,-325.674486892313)) ;
#27635=CARTESIAN_POINT('Ctrl Pts',(19.1360113345374,-3.34291954851933,-325.686018013787)) ;
#27636=CARTESIAN_POINT('Ctrl Pts',(19.1047120465276,-3.51738804445568,-325.688229549931)) ;
#27637=CARTESIAN_POINT('Ctrl Pts',(19.0470022281513,-3.81553630322163,-325.691992275192)) ;
#27638=CARTESIAN_POINT('Ctrl Pts',(19.0217636568214,-3.93943125257594,-325.693550962383)) ;
#27639=CARTESIAN_POINT('Ctrl Pts',(18.9670698464512,-4.19513100999603,-325.696758116407)) ;
#27640=CARTESIAN_POINT('Ctrl Pts',(18.9374459906652,-4.32689289913894,-325.698405376862)) ;
#27641=CARTESIAN_POINT('Ctrl Pts',(18.8543442335556,-4.67930230128461,-325.702798349683)) ;
#27642=CARTESIAN_POINT('Ctrl Pts',(18.7983680964116,-4.89933910485499,-325.705527560862)) ;
#27643=CARTESIAN_POINT('Ctrl Pts',(18.6973591209794,-5.26913867199483,-325.710100354237)) ;
#27644=CARTESIAN_POINT('Ctrl Pts',(18.654351624084,-5.41943041233557,-325.711954919475)) ;
#27645=CARTESIAN_POINT('Ctrl Pts',(18.45512619462,-6.08514566439696,-325.720163986161)) ;
#27646=CARTESIAN_POINT('Ctrl Pts',(18.2793264852936,-6.59446007216371,-325.726422210917)) ;
#27647=CARTESIAN_POINT('Ctrl Pts',(17.9527051869881,-7.42680484279685,-325.736888857779)) ;
#27648=CARTESIAN_POINT('Ctrl Pts',(17.8137553333078,-7.75417136742226,-325.741071215078)) ;
#27649=CARTESIAN_POINT('Ctrl Pts',(17.6174632413621,-8.18347001519694,-325.746735194471)) ;
#27650=CARTESIAN_POINT('Ctrl Pts',(17.5680754081074,-8.28896368351932,-325.748141832945)) ;
#27651=CARTESIAN_POINT('Ctrl Pts',(17.4906565081747,-8.45053185472246,-325.750323267103)) ;
#27652=CARTESIAN_POINT('Ctrl Pts',(17.4632978043589,-8.50692561974942,-325.751089802715)) ;
#27653=CARTESIAN_POINT('Ctrl Pts',(17.4047603248558,-8.62611490128409,-325.752721730465)) ;
#27654=CARTESIAN_POINT('Ctrl Pts',(17.3735135753857,-8.68887600771602,-325.753588095619)) ;
#27655=CARTESIAN_POINT('Ctrl Pts',(17.2880361791306,-8.85825822880064,-325.755943956954)) ;
#27656=CARTESIAN_POINT('Ctrl Pts',(17.2331593446905,-8.96454977765163,-325.757441374456)) ;
#27657=CARTESIAN_POINT('Ctrl Pts',(16.9866755808574,-9.43133850274607,-325.764090807529)) ;
#27658=CARTESIAN_POINT('Ctrl Pts',(16.7847135299939,-9.7862497425443,-325.769339068751)) ;
#27659=CARTESIAN_POINT('Ctrl Pts',(16.1885418630482,-10.7610938883815,-325.784072138248)) ;
#27660=CARTESIAN_POINT('Ctrl Pts',(15.7701363047459,-11.3654229387726,-325.793560286702)) ;
#27661=CARTESIAN_POINT('Ctrl Pts',(15.2088176358446,-12.0852934644555,-325.80502637145)) ;
#27662=CARTESIAN_POINT('Ctrl Pts',(15.0971840980272,-12.2244625422872,-325.807252691013)) ;
#27663=CARTESIAN_POINT('Ctrl Pts',(14.9030748808706,-12.4597357151092,-325.811032337506)) ;
#27664=CARTESIAN_POINT('Ctrl Pts',(14.8215475466529,-12.5566071598604,-325.812593339994)) ;
#27665=CARTESIAN_POINT('Ctrl Pts',(14.651362637607,-12.7548552668303,-325.815798294029)) ;
#27666=CARTESIAN_POINT('Ctrl Pts',(14.562586080773,-12.8561209824293,-325.817441112519)) ;
#27667=CARTESIAN_POINT('Ctrl Pts',(14.4698035249581,-12.9597619825596,-325.819129065824)) ;
#27668=CARTESIAN_POINT('Ctrl Pts',(14.4668422771126,-12.9630675082959,-325.819182908441)) ;
#27669=CARTESIAN_POINT('Ctrl Pts',(14.4608152749881,-12.9697905789233,-325.819292432702)) ;
#27670=CARTESIAN_POINT('Ctrl Pts',(14.4577494413635,-12.9732080523367,-325.819348113678)) ;
#27671=CARTESIAN_POINT('Ctrl Pts',(14.4514825751406,-12.9801887244908,-325.819461865476)) ;
#27672=CARTESIAN_POINT('Ctrl Pts',(14.448281435609,-12.9837518268191,-325.8195199354)) ;
#27673=CARTESIAN_POINT('Ctrl Pts',(14.4417095754615,-12.9910613475353,-325.819639079928)) ;
#27674=CARTESIAN_POINT('Ctrl Pts',(14.4383387141463,-12.9948076389376,-325.819700153353)) ;
#27675=CARTESIAN_POINT('Ctrl Pts',(14.4313880826089,-13.0025263546757,-325.819826005797)) ;
#27676=CARTESIAN_POINT('Ctrl Pts',(14.4278081291634,-13.0064986134991,-325.819890783282)) ;
#27677=CARTESIAN_POINT('Ctrl Pts',(14.4203935131201,-13.0147189242541,-325.820024857457)) ;
#27678=CARTESIAN_POINT('Ctrl Pts',(14.4165586125585,-13.0189667608933,-325.82009415216)) ;
#27679=CARTESIAN_POINT('Ctrl Pts',(14.4085799305906,-13.027796726638,-325.820238220004)) ;
#27680=CARTESIAN_POINT('Ctrl Pts',(14.4044358392714,-13.0323785748856,-325.820312990563)) ;
#27681=CARTESIAN_POINT('Ctrl Pts',(14.3957738308613,-13.0419464069701,-325.820469156361)) ;
#27682=CARTESIAN_POINT('Ctrl Pts',(14.3912555075687,-13.0469320220301,-325.820550548223)) ;
#27683=CARTESIAN_POINT('Ctrl Pts',(14.3817662435857,-13.0573917529893,-325.820721342493)) ;
#27684=CARTESIAN_POINT('Ctrl Pts',(14.3767947657148,-13.0628653801797,-325.820810740447)) ;
#27685=CARTESIAN_POINT('Ctrl Pts',(14.2640103450764,-13.1868993344541,-325.822836992038)) ;
#27686=CARTESIAN_POINT('Ctrl Pts',(14.1547374110561,-13.3041239505955,-325.82476165103)) ;
#27687=CARTESIAN_POINT('Ctrl Pts',(13.8544910749184,-13.6183320566801,-325.829952337115)) ;
#27688=CARTESIAN_POINT('Ctrl Pts',(13.6607748072115,-13.8126435895157,-325.833196813771)) ;
#27689=CARTESIAN_POINT('Ctrl Pts',(13.1895220767711,-14.2657304810727,-325.840881878341)) ;
#27690=CARTESIAN_POINT('Ctrl Pts',(12.9083916190039,-14.5206055189928,-325.845302310798)) ;
#27691=CARTESIAN_POINT('Ctrl Pts',(12.5720206005074,-14.8080688385666,-325.850474450753)) ;
#27692=CARTESIAN_POINT('Ctrl Pts',(12.5238634319281,-14.8488197997022,-325.851212278184)) ;
#27693=CARTESIAN_POINT('Ctrl Pts',(12.2054641656248,-15.1156008662701,-325.856075350132)) ;
#27694=CARTESIAN_POINT('Ctrl Pts',(11.9293145861188,-15.3344774134465,-325.860220217427)) ;
#27695=CARTESIAN_POINT('Ctrl Pts',(11.5543412503041,-15.6154197745484,-325.865842453247)) ;
#27696=CARTESIAN_POINT('Ctrl Pts',(11.4606923136646,-15.6842809238087,-325.867246241772)) ;
#27697=CARTESIAN_POINT('Ctrl Pts',(11.3156366418857,-15.7889491678306,-325.869424291835)) ;
#27698=CARTESIAN_POINT('Ctrl Pts',(11.2646652580572,-15.8253551318289,-325.870190333527)) ;
#27699=CARTESIAN_POINT('Ctrl Pts',(11.1748671158137,-15.8888391823217,-325.87154189618)) ;
#27700=CARTESIAN_POINT('Ctrl Pts',(11.1361158001846,-15.9160230740663,-325.872125810804)) ;
#27701=CARTESIAN_POINT('Ctrl Pts',(11.0242953808099,-15.9938563442287,-325.873812183941)) ;
#27702=CARTESIAN_POINT('Ctrl Pts',(10.9509774343343,-16.0441460541718,-325.874919645981)) ;
#27703=CARTESIAN_POINT('Ctrl Pts',(10.6701742449084,-16.2339309708988,-325.879163759012)) ;
#27704=CARTESIAN_POINT('Ctrl Pts',(10.4603482909359,-16.3699189494769,-325.882340204739)) ;
#27705=CARTESIAN_POINT('Ctrl Pts',(9.79546693794153,-16.7828234519928,-325.892355523447)) ;
#27706=CARTESIAN_POINT('Ctrl Pts',(9.33161089234153,-17.0450982505494,-325.899265475006)) ;
#27707=CARTESIAN_POINT('Ctrl Pts',(8.46310830199521,-17.4900789825837,-325.911804980233)) ;
#27708=CARTESIAN_POINT('Ctrl Pts',(8.06185063370071,-17.6786207355001,-325.917452404765)) ;
#27709=CARTESIAN_POINT('Ctrl Pts',(7.50356713705214,-17.9179817995941,-325.925065656562)) ;
#27710=CARTESIAN_POINT('Ctrl Pts',(7.35182462698565,-17.9807749085239,-325.927111294524)) ;
#27711=CARTESIAN_POINT('Ctrl Pts',(7.0831364085428,-18.0879917999438,-325.930691643099)) ;
#27712=CARTESIAN_POINT('Ctrl Pts',(6.96652369054359,-18.1332241053185,-325.932231853424)) ;
#27713=CARTESIAN_POINT('Ctrl Pts',(6.73160129575199,-18.2217462930249,-325.935307787692)) ;
#27714=CARTESIAN_POINT('Ctrl Pts',(6.61329102871445,-18.2650178151972,-325.93684332686)) ;
#27715=CARTESIAN_POINT('Ctrl Pts',(6.41931972932114,-18.3338303186149,-325.939339680997)) ;
#27716=CARTESIAN_POINT('Ctrl Pts',(6.34390740606857,-18.3600609686849,-325.940305031052)) ;
#27717=CARTESIAN_POINT('Ctrl Pts',(5.92267179432441,-18.5036741050653,-325.945669505806)) ;
#27718=CARTESIAN_POINT('Ctrl Pts',(5.57375305682515,-18.6117509719516,-325.950007494172)) ;
#27719=CARTESIAN_POINT('Ctrl Pts',(4.49543333633788,-18.9127131301077,-325.963188830535)) ;
#27720=CARTESIAN_POINT('Ctrl Pts',(3.75767969512353,-19.073003814011,-325.971875202038)) ;
#27721=CARTESIAN_POINT('Ctrl Pts',(2.85505859821545,-19.214699006034,-325.982755057587)) ;
#27722=CARTESIAN_POINT('Ctrl Pts',(2.69733833914895,-19.2374734110603,-325.984666544533)) ;
#27723=CARTESIAN_POINT('Ctrl Pts',(2.46144089807498,-19.2685783081648,-325.98755124297)) ;
#27724=CARTESIAN_POINT('Ctrl Pts',(2.38346422449059,-19.2783790704129,-325.988508985337)) ;
#27725=CARTESIAN_POINT('Ctrl Pts',(2.24174403935766,-19.2953186692742,-325.990258857179)) ;
#27726=CARTESIAN_POINT('Ctrl Pts',(2.17802067853291,-19.302615490631,-325.991049179009)) ;
#27727=CARTESIAN_POINT('Ctrl Pts',(2.0468631093184,-19.3169763041413,-325.992682559518)) ;
#27728=CARTESIAN_POINT('Ctrl Pts',(1.97942570103222,-19.3240031050592,-325.993525983449)) ;
#27729=CARTESIAN_POINT('Ctrl Pts',(1.81484186417456,-19.3402817152584,-325.995591989879)) ;
#27730=CARTESIAN_POINT('Ctrl Pts',(1.71765986544026,-19.3491548231964,-325.996818349495)) ;
#27731=CARTESIAN_POINT('Ctrl Pts',(1.08162212538613,-19.4023980696581,-326.004878017996)) ;
#27732=CARTESIAN_POINT('Ctrl Pts',(0.541181276773599,-19.4249859516044,
-326.011875812873)) ;
#27733=CARTESIAN_POINT('Ctrl Pts',(0.000504484077160222,-19.4249999934491,
-326.018849108403)) ;
#27734=CARTESIAN_POINT('Origin',(0.,0.,-328.125)) ;
#27735=CARTESIAN_POINT('',(-0.000502513484877063,-19.4249999935001,-327.731156847152)) ;
#27736=CARTESIAN_POINT('',(-0.000462715177408183,-19.4249999944889,-327.51849135163)) ;
#27737=CARTESIAN_POINT('',(-2.37887640734373E-15,-19.425,-328.125)) ;
#27738=CARTESIAN_POINT('Ctrl Pts',(-0.000501968905967098,-19.4249999935142,
-327.73119906165)) ;
#27739=CARTESIAN_POINT('Ctrl Pts',(0.566668136750594,-19.4250146499753,
-327.723882407847)) ;
#27740=CARTESIAN_POINT('Ctrl Pts',(1.13356879912891,-19.4001890010975,-327.716592548354)) ;
#27741=CARTESIAN_POINT('Ctrl Pts',(1.84523395830898,-19.3377199424505,-327.707595627717)) ;
#27742=CARTESIAN_POINT('Ctrl Pts',(1.99174650924835,-19.3231790047744,-327.705751083962)) ;
#27743=CARTESIAN_POINT('Ctrl Pts',(2.25516570455525,-19.2940076164169,-327.70244934237)) ;
#27744=CARTESIAN_POINT('Ctrl Pts',(2.37213141584046,-19.2799765259975,-327.700988468624)) ;
#27745=CARTESIAN_POINT('Ctrl Pts',(2.6003936402977,-19.2504857630597,-327.698147630888)) ;
#27746=CARTESIAN_POINT('Ctrl Pts',(2.71169801284079,-19.2351226437466,-327.696767100085)) ;
#27747=CARTESIAN_POINT('Ctrl Pts',(2.9687411230739,-19.1973680670589,-327.693589343242)) ;
#27748=CARTESIAN_POINT('Ctrl Pts',(3.11437077429207,-19.1742811941801,-327.691796736925)) ;
#27749=CARTESIAN_POINT('Ctrl Pts',(3.55675817356864,-19.0989759523275,-327.686371990605)) ;
#27750=CARTESIAN_POINT('Ctrl Pts',(3.85257645060155,-19.0415090353982,-327.682773666884)) ;
#27751=CARTESIAN_POINT('Ctrl Pts',(4.82290285328572,-18.8294710535858,-327.671016525914)) ;
#27752=CARTESIAN_POINT('Ctrl Pts',(5.49049028565787,-18.6457471262594,-327.663017810499)) ;
#27753=CARTESIAN_POINT('Ctrl Pts',(6.41461400812271,-18.3374760815901,-327.651556986669)) ;
#27754=CARTESIAN_POINT('Ctrl Pts',(6.68040060684859,-18.2423284981641,-327.648211192618)) ;
#27755=CARTESIAN_POINT('Ctrl Pts',(7.01872674118403,-18.1128269188619,-327.643841877151)) ;
#27756=CARTESIAN_POINT('Ctrl Pts',(7.093257555339,-18.0837695543178,-327.642872347894)) ;
#27757=CARTESIAN_POINT('Ctrl Pts',(7.2242356374264,-18.0317707596647,-327.64115457026)) ;
#27758=CARTESIAN_POINT('Ctrl Pts',(7.28075849345368,-18.0090225451982,-327.640408661855)) ;
#27759=CARTESIAN_POINT('Ctrl Pts',(7.3955320375174,-17.9622020747321,-327.638883819505)) ;
#27760=CARTESIAN_POINT('Ctrl Pts',(7.45377443851947,-17.9381114975901,-327.63810468766)) ;
#27761=CARTESIAN_POINT('Ctrl Pts',(7.6211400281547,-17.867928862847,-327.635851475496)) ;
#27762=CARTESIAN_POINT('Ctrl Pts',(7.7299601166779,-17.8211215614828,-327.634368888616)) ;
#27763=CARTESIAN_POINT('Ctrl Pts',(8.18918203480905,-17.6185966819481,-327.628048015504)) ;
#27764=CARTESIAN_POINT('Ctrl Pts',(8.53536031698953,-17.453517549193,-327.62312499457)) ;
#27765=CARTESIAN_POINT('Ctrl Pts',(9.33590965349982,-17.0422493520048,-327.611526415786)) ;
#27766=CARTESIAN_POINT('Ctrl Pts',(9.78579654832614,-16.7879617468808,-327.60484362662)) ;
#27767=CARTESIAN_POINT('Ctrl Pts',(10.4149830250614,-16.3984351314029,-327.595404233212)) ;
#27768=CARTESIAN_POINT('Ctrl Pts',(10.602910950418,-16.2775558907902,-327.592571372946)) ;
#27769=CARTESIAN_POINT('Ctrl Pts',(10.9350401002305,-16.055730636703,-327.587547080553)) ;
#27770=CARTESIAN_POINT('Ctrl Pts',(11.0800337011288,-15.9560158430098,-327.585347413003)) ;
#27771=CARTESIAN_POINT('Ctrl Pts',(11.3161706080924,-15.7888491355471,-327.581755525946)) ;
#27772=CARTESIAN_POINT('Ctrl Pts',(11.4081136007697,-15.722544907361,-327.580354533691)) ;
#27773=CARTESIAN_POINT('Ctrl Pts',(11.6006406115458,-15.5811270469345,-327.577415492209)) ;
#27774=CARTESIAN_POINT('Ctrl Pts',(11.7010875480931,-15.5058354463931,-327.575878957593)) ;
#27775=CARTESIAN_POINT('Ctrl Pts',(11.9434078426385,-15.3205048272493,-327.572163486772)) ;
#27776=CARTESIAN_POINT('Ctrl Pts',(12.0844991050308,-15.2094622051041,-327.569992821382)) ;
#27777=CARTESIAN_POINT('Ctrl Pts',(12.8551378581171,-14.5854550079223,-327.558083539922)) ;
#27778=CARTESIAN_POINT('Ctrl Pts',(13.4535768455231,-14.0353601777939,-327.54867443968)) ;
#27779=CARTESIAN_POINT('Ctrl Pts',(14.1895957964404,-13.2683451562877,-327.536222005879)) ;
#27780=CARTESIAN_POINT('Ctrl Pts',(14.3598373262853,-13.0839093436941,-327.533269964119)) ;
#27781=CARTESIAN_POINT('Ctrl Pts',(14.5799589030939,-12.8359618934182,-327.52932490935)) ;
#27782=CARTESIAN_POINT('Ctrl Pts',(14.6330852422614,-12.7753644027369,-327.528362527469)) ;
#27783=CARTESIAN_POINT('Ctrl Pts',(14.7628832766829,-12.6254409669097,-327.525983724717)) ;
#27784=CARTESIAN_POINT('Ctrl Pts',(14.8391229738793,-12.5357453530125,-327.524562459972)) ;
#27785=CARTESIAN_POINT('Ctrl Pts',(14.9592222454539,-12.391818190619,-327.522280367687)) ;
#27786=CARTESIAN_POINT('Ctrl Pts',(15.003613266523,-12.338033765723,-327.521427232539)) ;
#27787=CARTESIAN_POINT('Ctrl Pts',(15.0875519420893,-12.235210257274,-327.519794435575)) ;
#27788=CARTESIAN_POINT('Ctrl Pts',(15.1271525341827,-12.1862155668352,-327.519015695774)) ;
#27789=CARTESIAN_POINT('Ctrl Pts',(15.2404203624299,-12.0446753192894,-327.516765046904)) ;
#27790=CARTESIAN_POINT('Ctrl Pts',(15.3134814938793,-11.9516484572463,-327.515284660065)) ;
#27791=CARTESIAN_POINT('Ctrl Pts',(15.6181868016405,-11.5562937080068,-327.508998597108)) ;
#27792=CARTESIAN_POINT('Ctrl Pts',(15.8417625852091,-11.2478549323534,-327.504109321328)) ;
#27793=CARTESIAN_POINT('Ctrl Pts',(16.3738776064693,-10.4663977676742,-327.49192626063)) ;
#27794=CARTESIAN_POINT('Ctrl Pts',(16.6711357885627,-9.9861195722908,-327.484621259946)) ;
#27795=CARTESIAN_POINT('Ctrl Pts',(17.0142455631378,-9.3736318898535,-327.475688157411)) ;
#27796=CARTESIAN_POINT('Ctrl Pts',(17.0801629081835,-9.25297584412378,-327.473945670853)) ;
#27797=CARTESIAN_POINT('Ctrl Pts',(17.2425369969996,-8.94811567775496,-327.469588249399)) ;
#27798=CARTESIAN_POINT('Ctrl Pts',(17.3373274873748,-8.76304353983245,-327.466984085452)) ;
#27799=CARTESIAN_POINT('Ctrl Pts',(17.4872367995477,-8.45839791387403,-327.462765861239)) ;
#27800=CARTESIAN_POINT('Ctrl Pts',(17.5441433330496,-8.33972307201492,-327.461139271792)) ;
#27801=CARTESIAN_POINT('Ctrl Pts',(17.6535542601527,-8.10547701976162,-327.457960821823)) ;
#27802=CARTESIAN_POINT('Ctrl Pts',(17.706140601229,-7.98995123845244,-327.456408436128)) ;
#27803=CARTESIAN_POINT('Ctrl Pts',(17.8339515520026,-7.70170661881636,-327.452571530115)) ;
#27804=CARTESIAN_POINT('Ctrl Pts',(17.9078030513009,-7.5283931105201,-327.450296706834)) ;
#27805=CARTESIAN_POINT('Ctrl Pts',(18.1654080331232,-6.89860105018048,-327.442136301733)) ;
#27806=CARTESIAN_POINT('Ctrl Pts',(18.3343220985767,-6.43625511553254,-327.436349081787)) ;
#27807=CARTESIAN_POINT('Ctrl Pts',(18.6253515271782,-5.53480932736616,-327.425271254274)) ;
#27808=CARTESIAN_POINT('Ctrl Pts',(18.7499342377481,-5.09684204644661,-327.419978412791)) ;
#27809=CARTESIAN_POINT('Ctrl Pts',(18.8983832634481,-4.49541130894042,-327.412663834606)) ;
#27810=CARTESIAN_POINT('Ctrl Pts',(18.9357254740428,-4.33542540780872,-327.41071328482)) ;
#27811=CARTESIAN_POINT('Ctrl Pts',(18.9978026811942,-4.05334805885832,-327.407253258793)) ;
#27812=CARTESIAN_POINT('Ctrl Pts',(19.0234010809841,-3.93145627492153,-327.405751266031)) ;
#27813=CARTESIAN_POINT('Ctrl Pts',(19.0617662007668,-3.73961868242635,-327.403371383068)) ;
#27814=CARTESIAN_POINT('Ctrl Pts',(19.0753241990219,-3.66983450157261,-327.402502345583)) ;
#27815=CARTESIAN_POINT('Ctrl Pts',(19.0999833063529,-3.53908220189843,-327.400866636083)) ;
#27816=CARTESIAN_POINT('Ctrl Pts',(19.1111763305201,-3.47813231291543,-327.400101136104)) ;
#27817=CARTESIAN_POINT('Ctrl Pts',(19.1418411427795,-3.30653365463806,-327.397938504287)) ;
#27818=CARTESIAN_POINT('Ctrl Pts',(19.1606449130957,-3.19576807749216,-327.39653386666)) ;
#27819=CARTESIAN_POINT('Ctrl Pts',(19.286925947311,-2.41067886167694,-327.386531538265)) ;
#27820=CARTESIAN_POINT('Ctrl Pts',(19.3597420745788,-1.73126322544248,-327.377651447447)) ;
#27821=CARTESIAN_POINT('Ctrl Pts',(19.4148425161922,-0.712838622452622,
-327.364522424441)) ;
#27822=CARTESIAN_POINT('Ctrl Pts',(19.42428891004,-0.375832155735956,-327.360204052552)) ;
#27823=CARTESIAN_POINT('Ctrl Pts',(19.4251963094077,0.07903115954985,-327.354437981209)) ;
#27824=CARTESIAN_POINT('Ctrl Pts',(19.4243600257351,0.196812623540111,-327.352950449001)) ;
#27825=CARTESIAN_POINT('Ctrl Pts',(19.4194294443807,0.501231877525742,-327.349121166749)) ;
#27826=CARTESIAN_POINT('Ctrl Pts',(19.4137158078641,0.687831393476101,-327.346788983854)) ;
#27827=CARTESIAN_POINT('Ctrl Pts',(19.3995557331429,1.0021108076904,-327.342887386928)) ;
#27828=CARTESIAN_POINT('Ctrl Pts',(19.3925358278598,1.12984199358938,-327.341309001475)) ;
#27829=CARTESIAN_POINT('Ctrl Pts',(19.3767082182586,1.37382428624687,-327.338307730169)) ;
#27830=CARTESIAN_POINT('Ctrl Pts',(19.368114647542,1.49008375024846,-327.336883527271)) ;
#27831=CARTESIAN_POINT('Ctrl Pts',(19.3422757059462,1.80149214885456,-327.333083614171)) ;
#27832=CARTESIAN_POINT('Ctrl Pts',(19.3231238091603,1.99646935095384,-327.330720241292)) ;
#27833=CARTESIAN_POINT('Ctrl Pts',(19.2443915751077,2.69000067636812,-327.322359060484)) ;
#27834=CARTESIAN_POINT('Ctrl Pts',(19.1684366109644,3.18649491617604,-327.316462024864)) ;
#27835=CARTESIAN_POINT('Ctrl Pts',(18.9907444286586,4.10759646295215,-327.305496826173)) ;
#27836=CARTESIAN_POINT('Ctrl Pts',(18.8937667770527,4.53280251966119,-327.300423520097)) ;
#27837=CARTESIAN_POINT('Ctrl Pts',(18.7415271704949,5.10995809640824,-327.29337233588)) ;
#27838=CARTESIAN_POINT('Ctrl Pts',(18.698559115876,5.26501655375615,-327.291461057915)) ;
#27839=CARTESIAN_POINT('Ctrl Pts',(18.6194378857411,5.53734702931232,-327.288062545053)) ;
#27840=CARTESIAN_POINT('Ctrl Pts',(18.5840905040147,5.65484388600805,-327.286582431093)) ;
#27841=CARTESIAN_POINT('Ctrl Pts',(18.526618928557,5.83952199731724,-327.284229109465)) ;
#27842=CARTESIAN_POINT('Ctrl Pts',(18.5052369211638,5.90693089168744,-327.283364435468)) ;
#27843=CARTESIAN_POINT('Ctrl Pts',(18.4643518369039,6.03342418287602,-327.281729934414)) ;
#27844=CARTESIAN_POINT('Ctrl Pts',(18.4449320547868,6.09253458020453,-327.280961215013)) ;
#27845=CARTESIAN_POINT('Ctrl Pts',(18.389184867434,6.25950950045119,-327.278776868335)) ;
#27846=CARTESIAN_POINT('Ctrl Pts',(18.3521929909856,6.36714941247892,-327.277353498364)) ;
#27847=CARTESIAN_POINT('Ctrl Pts',(18.0883996877346,7.1133398326548,-327.267395163338)) ;
#27848=CARTESIAN_POINT('Ctrl Pts',(17.8292663515923,7.73996567300107,-327.258584083656)) ;
#27849=CARTESIAN_POINT('Ctrl Pts',(17.3704649851364,8.70340522876972,-327.24484673261)) ;
#27850=CARTESIAN_POINT('Ctrl Pts',(17.1924720892921,9.0499293308566,-327.239860933761)) ;
#27851=CARTESIAN_POINT('Ctrl Pts',(16.8974944480936,9.58404965050726,-327.232151044033)) ;
#27852=CARTESIAN_POINT('Ctrl Pts',(16.7875221512588,9.77539905052449,-327.229383295466)) ;
#27853=CARTESIAN_POINT('Ctrl Pts',(16.6056208213326,10.0797774255433,-327.224974057793)) ;
#27854=CARTESIAN_POINT('Ctrl Pts',(16.5357416159832,10.1940082930281,-327.223317724807)) ;
#27855=CARTESIAN_POINT('Ctrl Pts',(16.3980620560127,10.4139305993688,-327.220125541971)) ;
#27856=CARTESIAN_POINT('Ctrl Pts',(16.3304069663555,10.519705227921,-327.218588690707)) ;
#27857=CARTESIAN_POINT('Ctrl Pts',(16.1634276993092,10.775274057909,-327.214870678222)) ;
#27858=CARTESIAN_POINT('Ctrl Pts',(16.0630408596398,10.9243601408166,-327.212697817307)) ;
#27859=CARTESIAN_POINT('Ctrl Pts',(15.5488179095441,11.6656248629819,-327.201863019034)) ;
#27860=CARTESIAN_POINT('Ctrl Pts',(15.1042417609244,12.2357845352804,-327.19345142729)) ;
#27861=CARTESIAN_POINT('Ctrl Pts',(14.3554395815758,13.0929294497839,-327.180149104946)) ;
#27862=CARTESIAN_POINT('Ctrl Pts',(14.0719557399637,13.3971454884869,-327.17527742804)) ;
#27863=CARTESIAN_POINT('Ctrl Pts',(13.6940323823287,13.7774674517206,-327.168849297126)) ;
#27864=CARTESIAN_POINT('Ctrl Pts',(13.6083412286594,13.8621131582323,-327.167395769415)) ;
#27865=CARTESIAN_POINT('Ctrl Pts',(13.4714177347975,13.9948728942528,-327.165074674288)) ;
#27866=CARTESIAN_POINT('Ctrl Pts',(13.4207019244223,14.0435153348156,-327.164215257509)) ;
#27867=CARTESIAN_POINT('Ctrl Pts',(13.3178041141762,14.1411400028828,-327.162470919151)) ;
#27868=CARTESIAN_POINT('Ctrl Pts',(13.265613128547,14.190111180402,-327.161585864764)) ;
#27869=CARTESIAN_POINT('Ctrl Pts',(13.1200916214667,14.3251505712105,-327.159118846724)) ;
#27870=CARTESIAN_POINT('Ctrl Pts',(13.0261862103204,14.4105938733694,-327.15752771661)) ;
#27871=CARTESIAN_POINT('Ctrl Pts',(12.3337919302591,15.0282961089767,-327.145823757275)) ;
#27872=CARTESIAN_POINT('Ctrl Pts',(11.7037292927899,15.5240082809409,-327.135359251772)) ;
#27873=CARTESIAN_POINT('Ctrl Pts',(10.8293324702579,16.1283859429093,-327.121745459268)) ;
#27874=CARTESIAN_POINT('Ctrl Pts',(10.6108042556443,16.2729870727067,-327.118409705786)) ;
#27875=CARTESIAN_POINT('Ctrl Pts',(10.211730515983,16.5255985746628,-327.112449543477)) ;
#27876=CARTESIAN_POINT('Ctrl Pts',(10.0322283665869,16.6351808706627,-327.109814984559)) ;
#27877=CARTESIAN_POINT('Ctrl Pts',(9.73718496395107,16.8087860144633,-327.105561264456)) ;
#27878=CARTESIAN_POINT('Ctrl Pts',(9.62270792342425,16.8745829749602,-327.103929154302)) ;
#27879=CARTESIAN_POINT('Ctrl Pts',(9.39713888430339,17.0011894379518,-327.100748611605)) ;
#27880=CARTESIAN_POINT('Ctrl Pts',(9.28610534312561,17.062089822802,-327.099199560947)) ;
#27881=CARTESIAN_POINT('Ctrl Pts',(9.01001857262122,17.2100263064322,-327.0953874077)) ;
#27882=CARTESIAN_POINT('Ctrl Pts',(8.84429162752622,17.2957782681095,-327.093133708241)) ;
#27883=CARTESIAN_POINT('Ctrl Pts',(8.07672098442936,17.6790243274644,-327.082841772652)) ;
#27884=CARTESIAN_POINT('Ctrl Pts',(7.46094337387107,17.9475805610331,-327.075011020913)) ;
#27885=CARTESIAN_POINT('Ctrl Pts',(6.40336234459716,18.3449649055034,-327.061812816211)) ;
#27886=CARTESIAN_POINT('Ctrl Pts',(5.9686501663427,18.4909707634193,-327.05645088225)) ;
#27887=CARTESIAN_POINT('Ctrl Pts',(5.41733637926735,18.6546697616887,-327.049550617234)) ;
#27888=CARTESIAN_POINT('Ctrl Pts',(5.30519381248115,18.6868712179656,-327.048141705936)) ;
#27889=CARTESIAN_POINT('Ctrl Pts',(5.12576375440439,18.736648740995,-327.04587451163)) ;
#27890=CARTESIAN_POINT('Ctrl Pts',(5.05866008843115,18.754877184836,-327.045023747396)) ;
#27891=CARTESIAN_POINT('Ctrl Pts',(4.93039816095674,18.7889805768839,-327.043390971663)) ;
#27892=CARTESIAN_POINT('Ctrl Pts',(4.8692575155475,18.8049181965821,-327.042609840406)) ;
#27893=CARTESIAN_POINT('Ctrl Pts',(4.69241927466212,18.8500946156265,-327.040343583932)) ;
#27894=CARTESIAN_POINT('Ctrl Pts',(4.57652868663224,18.8785659091093,-327.038849805177)) ;
#27895=CARTESIAN_POINT('Ctrl Pts',(4.03386528017089,19.0065935692324,-327.031826728494)) ;
#27896=CARTESIAN_POINT('Ctrl Pts',(3.6040647352598,19.092757385174,-327.026185436129)) ;
#27897=CARTESIAN_POINT('Ctrl Pts',(2.69977606802398,19.2424183953177,-327.014363128814)) ;
#27898=CARTESIAN_POINT('Ctrl Pts',(2.22510743500877,19.3030659437785,-327.00818508451)) ;
#27899=CARTESIAN_POINT('Ctrl Pts',(1.60273133153192,19.3593221410527,-327.000221521302)) ;
#27900=CARTESIAN_POINT('Ctrl Pts',(1.45663307614301,19.3708626969991,-326.998361523632)) ;
#27901=CARTESIAN_POINT('Ctrl Pts',(1.09365063585451,19.3954055449964,-326.993766406868)) ;
#27902=CARTESIAN_POINT('Ctrl Pts',(0.876652267063747,19.4064244261836,-326.991042526894)) ;
#27903=CARTESIAN_POINT('Ctrl Pts',(0.526301933439306,19.4183263272582,-326.986684497529)) ;
#27904=CARTESIAN_POINT('Ctrl Pts',(0.393046185891204,19.4214805262244,-326.985036138449)) ;
#27905=CARTESIAN_POINT('Ctrl Pts',(0.133900628525554,19.4249463618657,-326.981848184261)) ;
#27906=CARTESIAN_POINT('Ctrl Pts',(0.00801934370696578,19.4254062062541,
-326.980307710019)) ;
#27907=CARTESIAN_POINT('Ctrl Pts',(-0.29967727195655,19.4235392795287,-326.976561024763)) ;
#27908=CARTESIAN_POINT('Ctrl Pts',(-0.481472646147607,19.4198833373667,
-326.974363447667)) ;
#27909=CARTESIAN_POINT('Ctrl Pts',(-1.36054938609427,19.3898532211094,-326.963803470521)) ;
#27910=CARTESIAN_POINT('Ctrl Pts',(-2.05611948930114,19.3284731949937,-326.955670778402)) ;
#27911=CARTESIAN_POINT('Ctrl Pts',(-3.17492987809722,19.1686571106704,-326.942465666141)) ;
#27912=CARTESIAN_POINT('Ctrl Pts',(-3.60082334543987,19.0932360969512,-326.9374039252)) ;
#27913=CARTESIAN_POINT('Ctrl Pts',(-4.14343126675036,18.9783441030285,-326.930756640686)) ;
#27914=CARTESIAN_POINT('Ctrl Pts',(-4.2627777868619,18.9518941804842,-326.929281917382)) ;
#27915=CARTESIAN_POINT('Ctrl Pts',(-4.45067349253324,18.908387522229,-326.926935135514)) ;
#27916=CARTESIAN_POINT('Ctrl Pts',(-4.51939301248104,18.892080351677,-326.926071532549)) ;
#27917=CARTESIAN_POINT('Ctrl Pts',(-4.64854275545965,18.8606880684438,-326.924437286712)) ;
#27918=CARTESIAN_POINT('Ctrl Pts',(-4.70899235067138,18.8456863816356,-326.923667735333)) ;
#27919=CARTESIAN_POINT('Ctrl Pts',(-4.88006651847555,18.802356657807,-326.921477815159)) ;
#27920=CARTESIAN_POINT('Ctrl Pts',(-4.99051483571171,18.7733435149545,-326.920049642568)) ;
#27921=CARTESIAN_POINT('Ctrl Pts',(-5.7529370018419,18.5658626955099,-326.910106871463)) ;
#27922=CARTESIAN_POINT('Ctrl Pts',(-6.39546372125375,18.3544432212098,-326.901318015372)) ;
#27923=CARTESIAN_POINT('Ctrl Pts',(-7.34166763172784,17.9873686779461,-326.888252264395)) ;
#27924=CARTESIAN_POINT('Ctrl Pts',(-7.65441356199913,17.8565245566211,-326.883909308)) ;
#27925=CARTESIAN_POINT('Ctrl Pts',(-8.1915833385204,17.6150809732716,-326.876442976331)) ;
#27926=CARTESIAN_POINT('Ctrl Pts',(-8.41759162717479,17.5082057002107,-326.873299108966)) ;
#27927=CARTESIAN_POINT('Ctrl Pts',(-8.76605840465014,17.3351145305557,-326.868452580306)) ;
#27928=CARTESIAN_POINT('Ctrl Pts',(-8.88997410658565,17.2718944007576,-326.866729219479)) ;
#27929=CARTESIAN_POINT('Ctrl Pts',(-9.12399785893963,17.1493128829453,-326.86347451004)) ;
#27930=CARTESIAN_POINT('Ctrl Pts',(-9.23423253101261,17.0902082754343,-326.861941396621)) ;
#27931=CARTESIAN_POINT('Ctrl Pts',(-9.48787302276198,16.951043123397,-326.858412961664)) ;
#27932=CARTESIAN_POINT('Ctrl Pts',(-9.63084973462912,16.8702202403512,-326.856423364099)) ;
#27933=CARTESIAN_POINT('Ctrl Pts',(-10.162122188545,16.5609435688433,-326.849022203673)) ;
#27934=CARTESIAN_POINT('Ctrl Pts',(-10.5434578538209,16.320817290034,-326.843696532373)) ;
#27935=CARTESIAN_POINT('Ctrl Pts',(-11.3519267139935,15.7715567210137,-326.832236401009)) ;
#27936=CARTESIAN_POINT('Ctrl Pts',(-11.775525302441,15.4578537960369,-326.82612416709)) ;
#27937=CARTESIAN_POINT('Ctrl Pts',(-12.2843381111514,15.0479785374472,-326.818420678904)) ;
#27938=CARTESIAN_POINT('Ctrl Pts',(-12.382053782604,14.9676773405857,-326.816923540845)) ;
#27939=CARTESIAN_POINT('Ctrl Pts',(-12.6025293359435,14.7828573367772,-326.813497737258)) ;
#27940=CARTESIAN_POINT('Ctrl Pts',(-12.7247861741752,14.6777530087043,-326.811563663347)) ;
#27941=CARTESIAN_POINT('Ctrl Pts',(-12.904199675055,14.5195844800975,-326.808663216711)) ;
#27942=CARTESIAN_POINT('Ctrl Pts',(-12.9623681656831,14.4676782603659,-326.80771293425)) ;
#27943=CARTESIAN_POINT('Ctrl Pts',(-13.0698023372714,14.37064213509,-326.805937712827)) ;
#27944=CARTESIAN_POINT('Ctrl Pts',(-13.1191506046413,14.3256056027662,-326.805114154647)) ;
#27945=CARTESIAN_POINT('Ctrl Pts',(-13.2424598566688,14.2118988028023,-326.803036529357)) ;
#27946=CARTESIAN_POINT('Ctrl Pts',(-13.3161198213233,14.1429050587323,-326.801777513884)) ;
#27947=CARTESIAN_POINT('Ctrl Pts',(-13.6549543331401,13.8205412138688,-326.795909510694)) ;
#27948=CARTESIAN_POINT('Ctrl Pts',(-13.9134567498053,13.560267609566,-326.791214313394)) ;
#27949=CARTESIAN_POINT('Ctrl Pts',(-14.5424124808288,12.8900716781056,-326.779384787836)) ;
#27950=CARTESIAN_POINT('Ctrl Pts',(-14.9030403284675,12.4713711967374,-326.772228808609)) ;
#27951=CARTESIAN_POINT('Ctrl Pts',(-15.3434734675197,11.9135857595116,-326.763155982997)) ;
#27952=CARTESIAN_POINT('Ctrl Pts',(-15.4400888892474,11.788102428551,-326.761142650473)) ;
#27953=CARTESIAN_POINT('Ctrl Pts',(-15.6726540307524,11.4782836689256,-326.756242728018)) ;
#27954=CARTESIAN_POINT('Ctrl Pts',(-15.8068988190968,11.2926980988616,-326.753367898429)) ;
#27955=CARTESIAN_POINT('Ctrl Pts',(-16.015239153861,10.9936834047738,-326.748833791124)) ;
#27956=CARTESIAN_POINT('Ctrl Pts',(-16.0914839950993,10.8817784785254,-326.747158079275)) ;
#27957=CARTESIAN_POINT('Ctrl Pts',(-16.2365621773585,10.6639870902589,-326.743937142684)) ;
#27958=CARTESIAN_POINT('Ctrl Pts',(-16.3055452492576,10.5582084736741,-326.742390807946)) ;
#27959=CARTESIAN_POINT('Ctrl Pts',(-16.4682946799596,10.3032489915601,-326.738705613038)) ;
#27960=CARTESIAN_POINT('Ctrl Pts',(-16.5610723739536,10.1534502213144,-326.736574345426)) ;
#27961=CARTESIAN_POINT('Ctrl Pts',(-16.8572969802614,9.6603017929765,-326.729661186565)) ;
#27962=CARTESIAN_POINT('Ctrl Pts',(-17.052203211794,9.31194172876649,-326.724940363902)) ;
#27963=CARTESIAN_POINT('Ctrl Pts',(-17.2905594545227,8.85330747705538,-326.71887407053)) ;
#27964=CARTESIAN_POINT('Ctrl Pts',(-17.3439265464113,8.7482976343601,-326.717494783342)) ;
#27965=CARTESIAN_POINT('Ctrl Pts',(-17.5996876258909,8.23349908479791,-326.710772015474)) ;
#27966=CARTESIAN_POINT('Ctrl Pts',(-17.7885307113949,7.81714051266059,-326.705458145723)) ;
#27967=CARTESIAN_POINT('Ctrl Pts',(-18.025168735461,7.24230687357798,-326.698118428772)) ;
#27968=CARTESIAN_POINT('Ctrl Pts',(-18.0858882867292,7.08931319371667,-326.69616421045)) ;
#27969=CARTESIAN_POINT('Ctrl Pts',(-18.1891865200064,6.81906693505941,-326.692698447572)) ;
#27970=CARTESIAN_POINT('Ctrl Pts',(-18.2325939537131,6.70214128267492,-326.691194420762)) ;
#27971=CARTESIAN_POINT('Ctrl Pts',(-18.298981964423,6.51789402633894,-326.688812068452)) ;
#27972=CARTESIAN_POINT('Ctrl Pts',(-18.322723968599,6.4508503181709,-326.68794262554)) ;
#27973=CARTESIAN_POINT('Ctrl Pts',(-18.366454838942,6.32517185745441,-326.686306792006)) ;
#27974=CARTESIAN_POINT('Ctrl Pts',(-18.3865324702208,6.26656892454612,-326.685541579356)) ;
#27975=CARTESIAN_POINT('Ctrl Pts',(-18.4421916635148,6.10153948923378,-326.683380897827)) ;
#27976=CARTESIAN_POINT('Ctrl Pts',(-18.4771318030187,5.99489931297739,-326.681977944361)) ;
#27977=CARTESIAN_POINT('Ctrl Pts',(-18.7188400377754,5.23499359142138,-326.671947710709)) ;
#27978=CARTESIAN_POINT('Ctrl Pts',(-18.8918391067089,4.57149274900552,-326.66303595763)) ;
#27979=CARTESIAN_POINT('Ctrl Pts',(-19.1071108013469,3.52117451989093,-326.649235247183)) ;
#27980=CARTESIAN_POINT('Ctrl Pts',(-19.17346007678,3.13986988593855,-326.644282771375)) ;
#27981=CARTESIAN_POINT('Ctrl Pts',(-19.2595432977273,2.53945717945131,-326.636619493037)) ;
#27982=CARTESIAN_POINT('Ctrl Pts',(-19.2870214234965,2.32156319290734,-326.633865593921)) ;
#27983=CARTESIAN_POINT('Ctrl Pts',(-19.3252768256865,1.9703246796273,-326.629472520394)) ;
#27984=CARTESIAN_POINT('Ctrl Pts',(-19.338381624878,1.83725336342452,-326.627818703396)) ;
#27985=CARTESIAN_POINT('Ctrl Pts',(-19.3611346243423,1.57888582739337,-326.624627892762)) ;
#27986=CARTESIAN_POINT('Ctrl Pts',(-19.3709429700669,1.45361029722551,-326.623089935928)) ;
#27987=CARTESIAN_POINT('Ctrl Pts',(-19.3899024665977,1.17698564934953,-326.61971326631)) ;
#27988=CARTESIAN_POINT('Ctrl Pts',(-19.398498497408,1.02560665391087,-326.617878197434)) ;
#27989=CARTESIAN_POINT('Ctrl Pts',(-19.4263394954064,0.407556900906628,
-326.61043281078)) ;
#27990=CARTESIAN_POINT('Ctrl Pts',(-19.4305227354124,-0.0596354283450282,
-326.604917585577)) ;
#27991=CARTESIAN_POINT('Ctrl Pts',(-19.415876213536,-0.599789694896713,
-326.598586530051)) ;
#27992=CARTESIAN_POINT('Ctrl Pts',(-19.4134749361234,-0.673043627672304,
-326.597728795079)) ;
#27993=CARTESIAN_POINT('Ctrl Pts',(-19.3932242648902,-1.19975974885412,
-326.591564750028)) ;
#27994=CARTESIAN_POINT('Ctrl Pts',(-19.3599033722535,-1.65248637867189,
-326.586287793001)) ;
#27995=CARTESIAN_POINT('Ctrl Pts',(-19.2929932086128,-2.26670402728339,
-326.578992214636)) ;
#27996=CARTESIAN_POINT('Ctrl Pts',(-19.2731635458214,-2.42954747176551,
-326.577044446651)) ;
#27997=CARTESIAN_POINT('Ctrl Pts',(-19.2346711467184,-2.71542456076907,
-326.573588771862)) ;
#27998=CARTESIAN_POINT('Ctrl Pts',(-19.2168843428523,-2.83856667193748,
-326.572088322599)) ;
#27999=CARTESIAN_POINT('Ctrl Pts',(-19.1870816040106,-3.03176093930503,
-326.569710313521)) ;
#28000=CARTESIAN_POINT('Ctrl Pts',(-19.1758621423515,-3.10193261591537,
-326.568841583785)) ;
#28001=CARTESIAN_POINT('Ctrl Pts',(-19.1541357999772,-3.23319485908132,
-326.5672059672)) ;
#28002=CARTESIAN_POINT('Ctrl Pts',(-19.1437210631545,-3.29429978671307,
-326.566440247877)) ;
#28003=CARTESIAN_POINT('Ctrl Pts',(-19.1135902942605,-3.46611249698711,
-326.56427612866)) ;
#28004=CARTESIAN_POINT('Ctrl Pts',(-19.0932051836634,-3.5767003703445,-326.5628702068)) ;
#28005=CARTESIAN_POINT('Ctrl Pts',(-18.9595464781687,-4.26806130310755,
-326.554012584145)) ;
#28006=CARTESIAN_POINT('Ctrl Pts',(-18.8207455204067,-4.84358205999536,
-326.546346905662)) ;
#28007=CARTESIAN_POINT('Ctrl Pts',(-18.5064327021914,-5.9270873115761,-326.531798750423)) ;
#28008=CARTESIAN_POINT('Ctrl Pts',(-18.3356934673468,-6.43589647271904,
-326.524915232974)) ;
#28009=CARTESIAN_POINT('Ctrl Pts',(-18.075896477473,-7.11541150258877,-326.515759403713)) ;
#28010=CARTESIAN_POINT('Ctrl Pts',(-18.005051215075,-7.29282148572337,-326.513371627074)) ;
#28011=CARTESIAN_POINT('Ctrl Pts',(-17.8821342853836,-7.58791463495438,
-326.50940558034)) ;
#28012=CARTESIAN_POINT('Ctrl Pts',(-17.8314892425379,-7.70617716854931,
-326.507817639474)) ;
#28013=CARTESIAN_POINT('Ctrl Pts',(-17.7267828129144,-7.94411981083961,
-326.504625409922)) ;
#28014=CARTESIAN_POINT('Ctrl Pts',(-17.6726750713459,-8.06377233943118,
-326.503021548296)) ;
#28015=CARTESIAN_POINT('Ctrl Pts',(-17.5304664418693,-8.36994135480655,
-326.498919776123)) ;
#28016=CARTESIAN_POINT('Ctrl Pts',(-17.4406003563519,-8.55561986964524,
-326.496434466652)) ;
#28017=CARTESIAN_POINT('Ctrl Pts',(-17.2097305422998,-9.01387604164141,
-326.49029689024)) ;
#28018=CARTESIAN_POINT('Ctrl Pts',(-17.0651926203697,-9.28461027162568,
-326.486667890694)) ;
#28019=CARTESIAN_POINT('Ctrl Pts',(-16.633843796164,-10.0484410616153,-326.476360866207)) ;
#28020=CARTESIAN_POINT('Ctrl Pts',(-16.3316492366972,-10.5324811302658,
-326.469752002778)) ;
#28021=CARTESIAN_POINT('Ctrl Pts',(-15.934135843127,-11.1108605326733,-326.46148319074)) ;
#28022=CARTESIAN_POINT('Ctrl Pts',(-15.8585774678224,-11.218441402047,-326.459928161646)) ;
#28023=CARTESIAN_POINT('Ctrl Pts',(-15.7353624836308,-11.3901436737998,
-326.457413081492)) ;
#28024=CARTESIAN_POINT('Ctrl Pts',(-15.6883921876064,-11.4547525487921,
-326.456459008982)) ;
#28025=CARTESIAN_POINT('Ctrl Pts',(-15.5716603185519,-11.6132554557697,
-326.454097302849)) ;
#28026=CARTESIAN_POINT('Ctrl Pts',(-15.5014466314936,-11.7068125306977,
-326.452684849241)) ;
#28027=CARTESIAN_POINT('Ctrl Pts',(-15.3881181419605,-11.855011100751,-326.450413385241)) ;
#28028=CARTESIAN_POINT('Ctrl Pts',(-15.3455472122291,-11.9100650252527,
-326.449561943308)) ;
#28029=CARTESIAN_POINT('Ctrl Pts',(-15.263796771605,-12.0146210261364,-326.447929174773)) ;
#28030=CARTESIAN_POINT('Ctrl Pts',(-15.2246700122831,-12.0641631824353,
-326.447148740501)) ;
#28031=CARTESIAN_POINT('Ctrl Pts',(-15.1110754485364,-12.2065634681421,
-326.444887025995)) ;
#28032=CARTESIAN_POINT('Ctrl Pts',(-15.0359948066638,-12.2989289380986,
-326.443397143485)) ;
#28033=CARTESIAN_POINT('Ctrl Pts',(-14.7079796367397,-12.6949654957752,
-326.436920168873)) ;
#28034=CARTESIAN_POINT('Ctrl Pts',(-14.4466595437442,-12.9915680756276,
-326.431842963322)) ;
#28035=CARTESIAN_POINT('Ctrl Pts',(-13.8293412900612,-13.6505591957493,
-326.420203443125)) ;
#28036=CARTESIAN_POINT('Ctrl Pts',(-13.4678107290303,-14.0073738668294,
-326.413637108092)) ;
#28037=CARTESIAN_POINT('Ctrl Pts',(-12.9289486446662,-14.4990364906767,
-326.404334248841)) ;
#28038=CARTESIAN_POINT('Ctrl Pts',(-12.7626346650623,-14.645645388478,-326.401524013453)) ;
#28039=CARTESIAN_POINT('Ctrl Pts',(-12.4515504324741,-14.9105482166596,
-326.396384851544)) ;
#28040=CARTESIAN_POINT('Ctrl Pts',(-12.3075117723127,-15.029661021551,-326.394049827619)) ;
#28041=CARTESIAN_POINT('Ctrl Pts',(-12.0620015696288,-15.2267894256519,
-326.390144942639)) ;
#28042=CARTESIAN_POINT('Ctrl Pts',(-11.9614374063831,-15.3059143243124,
-326.388566074749)) ;
#28043=CARTESIAN_POINT('Ctrl Pts',(-11.7553471741115,-15.4647965503637,
-326.385371662671)) ;
#28044=CARTESIAN_POINT('Ctrl Pts',(-11.6497734566204,-15.5444812712713,
-326.383756759582)) ;
#28045=CARTESIAN_POINT('Ctrl Pts',(-11.3732227603759,-15.7488157138312,
-326.379580508997)) ;
#28046=CARTESIAN_POINT('Ctrl Pts',(-11.2010083494869,-15.8717612288388,
-326.37703272424)) ;
#28047=CARTESIAN_POINT('Ctrl Pts',(-10.7850066413038,-16.1586054898234,
-326.370993066476)) ;
#28048=CARTESIAN_POINT('Ctrl Pts',(-10.539442647618,-16.3198360496331,-326.367519784772)) ;
#28049=CARTESIAN_POINT('Ctrl Pts',(-9.80464189680152,-16.7787818732795,
-326.357339156697)) ;
#28050=CARTESIAN_POINT('Ctrl Pts',(-9.30579190813018,-17.0605028990844,
-326.350704330877)) ;
#28051=CARTESIAN_POINT('Ctrl Pts',(-8.67779433068673,-17.3794090092136,
-326.342406119453)) ;
#28052=CARTESIAN_POINT('Ctrl Pts',(-8.55975720793982,-17.437847586399,-326.340848218291)) ;
#28053=CARTESIAN_POINT('Ctrl Pts',(-8.29193777083849,-17.5670667657182,
-326.337309469636)) ;
#28054=CARTESIAN_POINT('Ctrl Pts',(-8.14182597524522,-17.6371408222875,
-326.335323272179)) ;
#28055=CARTESIAN_POINT('Ctrl Pts',(-7.91908482008568,-17.7376694523077,
-326.332360689482)) ;
#28056=CARTESIAN_POINT('Ctrl Pts',(-7.84713698323759,-17.7696162910916,
-326.331401390081)) ;
#28057=CARTESIAN_POINT('Ctrl Pts',(-7.7139676181522,-17.8277806724376,-326.329619852116)) ;
#28058=CARTESIAN_POINT('Ctrl Pts',(-7.6528017566646,-17.8541223630844,-326.328799125861)) ;
#28059=CARTESIAN_POINT('Ctrl Pts',(-7.50001859569355,-17.9189905935569,
-326.326743670764)) ;
#28060=CARTESIAN_POINT('Ctrl Pts',(-7.40823883802229,-17.9571295063478,
-326.32550422923)) ;
#28061=CARTESIAN_POINT('Ctrl Pts',(-6.98812127312395,-18.127939537327,-326.319816112918)) ;
#28062=CARTESIAN_POINT('Ctrl Pts',(-6.65648651980135,-18.2523208701311,
-326.315286610653)) ;
#28063=CARTESIAN_POINT('Ctrl Pts',(-5.78858960379139,-18.5510283946736,
-326.303478920906)) ;
#28064=CARTESIAN_POINT('Ctrl Pts',(-5.24780573871246,-18.7111988137845,
-326.2961721002)) ;
#28065=CARTESIAN_POINT('Ctrl Pts',(-4.54557802093626,-18.8863428392721,
-326.286930803986)) ;
#28066=CARTESIAN_POINT('Ctrl Pts',(-4.38986001658318,-18.923143356745,-326.284896188374)) ;
#28067=CARTESIAN_POINT('Ctrl Pts',(-4.00862152712661,-19.0082815552744,
-326.27995443038)) ;
#28068=CARTESIAN_POINT('Ctrl Pts',(-3.78266041922966,-19.0545347533834,
-326.277059112407)) ;
#28069=CARTESIAN_POINT('Ctrl Pts',(-3.42252949552614,-19.1215932735807,
-326.272501140098)) ;
#28070=CARTESIAN_POINT('Ctrl Pts',(-3.28887318854987,-19.1450346220235,
-326.270821740463)) ;
#28071=CARTESIAN_POINT('Ctrl Pts',(-3.03049355255374,-19.1875650131771,
-326.26759848037)) ;
#28072=CARTESIAN_POINT('Ctrl Pts',(-2.90580818969529,-19.206843080534,-326.266053456598)) ;
#28073=CARTESIAN_POINT('Ctrl Pts',(-2.60736587899296,-19.2500137118308,
-326.262379239882)) ;
#28074=CARTESIAN_POINT('Ctrl Pts',(-2.4334557366044,-19.2727703777324,-326.26025751371)) ;
#28075=CARTESIAN_POINT('Ctrl Pts',(-1.5092198318398,-19.380999890506,-326.24907341693)) ;
#28076=CARTESIAN_POINT('Ctrl Pts',(-0.754693881584735,-19.4250183650223,
-326.240291315249)) ;
#28077=CARTESIAN_POINT('Ctrl Pts',(0.000472547765781872,-19.4249999942522,
-326.231461493639)) ;
#28078=CARTESIAN_POINT('Ctrl Pts',(0.000504483642990022,-19.4249999934491,
-326.018849108409)) ;
#28079=CARTESIAN_POINT('Ctrl Pts',(-0.417183116006538,-19.4250108411485,
-326.024236169794)) ;
#28080=CARTESIAN_POINT('Ctrl Pts',(-0.834763081159949,-19.4115496475603,
-326.029607004352)) ;
#28081=CARTESIAN_POINT('Ctrl Pts',(-1.46262225600774,-19.37101143102,-326.037594245163)) ;
#28082=CARTESIAN_POINT('Ctrl Pts',(-1.67342392998112,-19.3539401746368,
-326.040261445561)) ;
#28083=CARTESIAN_POINT('Ctrl Pts',(-2.00934202281247,-19.3212073505849,
-326.044484909349)) ;
#28084=CARTESIAN_POINT('Ctrl Pts',(-2.1346572109552,-19.3077639173627,-326.046054557209)) ;
#28085=CARTESIAN_POINT('Ctrl Pts',(-2.37660880868619,-19.2794237285403,
-326.049073501275)) ;
#28086=CARTESIAN_POINT('Ctrl Pts',(-2.49325832363575,-19.2646856113831,
-326.050523746003)) ;
#28087=CARTESIAN_POINT('Ctrl Pts',(-2.74063320141473,-19.2311464933607,
-326.053588413026)) ;
#28088=CARTESIAN_POINT('Ctrl Pts',(-2.87131523223212,-19.2120695055519,
-326.055200957389)) ;
#28089=CARTESIAN_POINT('Ctrl Pts',(-3.20971610912804,-19.1591397853971,
-326.059361341599)) ;
#28090=CARTESIAN_POINT('Ctrl Pts',(-3.41709751942014,-19.1232413456134,
-326.061895825569)) ;
#28091=CARTESIAN_POINT('Ctrl Pts',(-4.43296558334321,-18.9303382748923,
-326.074256759928)) ;
#28092=CARTESIAN_POINT('Ctrl Pts',(-5.23148311653603,-18.7253964223069,
-326.083763950563)) ;
#28093=CARTESIAN_POINT('Ctrl Pts',(-6.29996291227972,-18.3774637432828,
-326.096969733408)) ;
#28094=CARTESIAN_POINT('Ctrl Pts',(-6.5831561979217,-18.2779309573443,-326.100522725282)) ;
#28095=CARTESIAN_POINT('Ctrl Pts',(-6.93978497935403,-18.1432242064827,
-326.10511947458)) ;
#28096=CARTESIAN_POINT('Ctrl Pts',(-7.015461151484,-18.1140968579063,-326.106102037768)) ;
#28097=CARTESIAN_POINT('Ctrl Pts',(-7.14746080771023,-18.0623396353363,
-326.107830053798)) ;
#28098=CARTESIAN_POINT('Ctrl Pts',(-7.20386478530247,-18.039917994591,-326.108572992721)) ;
#28099=CARTESIAN_POINT('Ctrl Pts',(-7.31830365745087,-17.9938040955344,
-326.110090444645)) ;
#28100=CARTESIAN_POINT('Ctrl Pts',(-7.3763308009585,-17.9700945505292,-326.110865155662)) ;
#28101=CARTESIAN_POINT('Ctrl Pts',(-7.54187651551435,-17.9015166082095,
-326.11308934351)) ;
#28102=CARTESIAN_POINT('Ctrl Pts',(-7.64910749150483,-17.8559612671348,
-326.114547002543)) ;
#28103=CARTESIAN_POINT('Ctrl Pts',(-8.08222157450199,-17.6673422943036,
-326.120494175031)) ;
#28104=CARTESIAN_POINT('Ctrl Pts',(-8.40455377545699,-17.5162999629904,
-326.125056632679)) ;
#28105=CARTESIAN_POINT('Ctrl Pts',(-9.20353286995009,-17.1147707058398,
-326.136572019043)) ;
#28106=CARTESIAN_POINT('Ctrl Pts',(-9.67425787485637,-16.8531637977963,
-326.143542170827)) ;
#28107=CARTESIAN_POINT('Ctrl Pts',(-10.3276486622673,-16.4536342705895,
-326.153316185075)) ;
#28108=CARTESIAN_POINT('Ctrl Pts',(-10.5196878017921,-16.331520945544,-326.156202766444)) ;
#28109=CARTESIAN_POINT('Ctrl Pts',(-10.8579377110256,-16.1079934731872,
-326.161304940683)) ;
#28110=CARTESIAN_POINT('Ctrl Pts',(-11.0049842453181,-16.0078913964803,
-326.16352925462)) ;
#28111=CARTESIAN_POINT('Ctrl Pts',(-11.2447509485099,-15.839804673661,-326.167165523729)) ;
#28112=CARTESIAN_POINT('Ctrl Pts',(-11.3382791873913,-15.7729915076253,
-326.16858639451)) ;
#28113=CARTESIAN_POINT('Ctrl Pts',(-11.5336552200955,-15.6307862109798,
-326.171559879923)) ;
#28114=CARTESIAN_POINT('Ctrl Pts',(-11.6353694769942,-15.5552196221202,
-326.173111009631)) ;
#28115=CARTESIAN_POINT('Ctrl Pts',(-11.8790195454502,-15.3704776120871,
-326.176835205948)) ;
#28116=CARTESIAN_POINT('Ctrl Pts',(-12.0201993369405,-15.2603242237746,
-326.179000231612)) ;
#28117=CARTESIAN_POINT('Ctrl Pts',(-12.7952140340315,-14.6382021115376,
-326.190937187967)) ;
#28118=CARTESIAN_POINT('Ctrl Pts',(-13.3978713126674,-14.08870134432,-326.200376696002)) ;
#28119=CARTESIAN_POINT('Ctrl Pts',(-14.1380236654869,-13.3232658099767,
-326.212850090392)) ;
#28120=CARTESIAN_POINT('Ctrl Pts',(-14.3083214038202,-13.1402078870671,
-326.215790940702)) ;
#28121=CARTESIAN_POINT('Ctrl Pts',(-14.5860165191591,-12.8299042025996,
-326.220745961123)) ;
#28122=CARTESIAN_POINT('Ctrl Pts',(-14.6953966316696,-12.7044731268499,
-326.222741107501)) ;
#28123=CARTESIAN_POINT('Ctrl Pts',(-14.8542065809904,-12.5175632287752,
-326.225714342843)) ;
#28124=CARTESIAN_POINT('Ctrl Pts',(-14.9048954885932,-12.457163914408,-326.226675172374)) ;
#28125=CARTESIAN_POINT('Ctrl Pts',(-14.9976940020526,-12.3452108249675,
-326.22845781827)) ;
#28126=CARTESIAN_POINT('Ctrl Pts',(-15.0399089794738,-12.2937461152344,
-326.229278100201)) ;
#28127=CARTESIAN_POINT('Ctrl Pts',(-15.1443370911326,-12.1650938045637,
-326.231329965454)) ;
#28128=CARTESIAN_POINT('Ctrl Pts',(-15.2062253921845,-12.087645034796,-326.232566223194)) ;
#28129=CARTESIAN_POINT('Ctrl Pts',(-15.4689639182021,-11.7536353174374,
-326.237895926575)) ;
#28130=CARTESIAN_POINT('Ctrl Pts',(-15.6639343056643,-11.4925170967891,
-326.242057051588)) ;
#28131=CARTESIAN_POINT('Ctrl Pts',(-15.8970461667046,-11.1633578027091,
-326.247240465853)) ;
#28132=CARTESIAN_POINT('Ctrl Pts',(-15.9414691710518,-11.099828598737,-326.248238153613)) ;
#28133=CARTESIAN_POINT('Ctrl Pts',(-16.0674169511324,-10.917395365414,-326.251093920234)) ;
#28134=CARTESIAN_POINT('Ctrl Pts',(-16.1479998992553,-10.7978473915341,
-326.252954143089)) ;
#28135=CARTESIAN_POINT('Ctrl Pts',(-16.5318296622806,-10.2145132881092,
-326.26196337989)) ;
#28136=CARTESIAN_POINT('Ctrl Pts',(-16.81646896069,-9.73879091162881,-326.269097377645)) ;
#28137=CARTESIAN_POINT('Ctrl Pts',(-17.1841508641447,-9.05996996571856,
-326.278848902605)) ;
#28138=CARTESIAN_POINT('Ctrl Pts',(-17.284690113923,-8.86665577359058,-326.281580700346)) ;
#28139=CARTESIAN_POINT('Ctrl Pts',(-17.4415088068861,-8.55232081375976,
-326.285947973971)) ;
#28140=CARTESIAN_POINT('Ctrl Pts',(-17.499830257207,-8.43234023204501,-326.28759777327)) ;
#28141=CARTESIAN_POINT('Ctrl Pts',(-17.6107478825292,-8.19804942612475,
-326.290786465122)) ;
#28142=CARTESIAN_POINT('Ctrl Pts',(-17.6634784320572,-8.08381006107575,
-326.292326259148)) ;
#28143=CARTESIAN_POINT('Ctrl Pts',(-17.7776100228906,-7.83009752777707,
-326.295713865107)) ;
#28144=CARTESIAN_POINT('Ctrl Pts',(-17.8384872601975,-7.69039776402468,
-326.297557938864)) ;
#28145=CARTESIAN_POINT('Ctrl Pts',(-18.0831141308431,-7.11049522523312,
-326.305131029254)) ;
#28146=CARTESIAN_POINT('Ctrl Pts',(-18.2522623338474,-6.66431392536628,
-326.310760411905)) ;
#28147=CARTESIAN_POINT('Ctrl Pts',(-18.564810536716,-5.73835461150738,-326.322206576312)) ;
#28148=CARTESIAN_POINT('Ctrl Pts',(-18.706434490215,-5.25834682397881,-326.328014663097)) ;
#28149=CARTESIAN_POINT('Ctrl Pts',(-18.8715498810197,-4.60702642197433,
-326.335940856829)) ;
#28150=CARTESIAN_POINT('Ctrl Pts',(-18.9115221644071,-4.44009196565381,
-326.337976839763)) ;
#28151=CARTESIAN_POINT('Ctrl Pts',(-18.9775461497973,-4.14727444332013,
-326.341570055708)) ;
#28152=CARTESIAN_POINT('Ctrl Pts',(-19.0045705749389,-4.0216216084666,-326.343118989666)) ;
#28153=CARTESIAN_POINT('Ctrl Pts',(-19.0447612838984,-3.8252920324257,-326.345555829049)) ;
#28154=CARTESIAN_POINT('Ctrl Pts',(-19.0587856063218,-3.75479462686017,
-326.346434182434)) ;
#28155=CARTESIAN_POINT('Ctrl Pts',(-19.0840812370409,-3.62384459931966,
-326.34807318371)) ;
#28156=CARTESIAN_POINT('Ctrl Pts',(-19.0954573907817,-3.56341316168039,
-326.348832524501)) ;
#28157=CARTESIAN_POINT('Ctrl Pts',(-19.1262882817015,-3.39524764038206,
-326.350952824574)) ;
#28158=CARTESIAN_POINT('Ctrl Pts',(-19.1451194963724,-3.2874016173381,-326.35232083144)) ;
#28159=CARTESIAN_POINT('Ctrl Pts',(-19.2617534728501,-2.58442001629184,
-326.361278917417)) ;
#28160=CARTESIAN_POINT('Ctrl Pts',(-19.3327054174368,-1.98516349694068,
-326.369094774385)) ;
#28161=CARTESIAN_POINT('Ctrl Pts',(-19.4135551854647,-0.852942967973674,
-326.383731202071)) ;
#28162=CARTESIAN_POINT('Ctrl Pts',(-19.4296324368513,-0.320971838339124,
-326.390555701397)) ;
#28163=CARTESIAN_POINT('Ctrl Pts',(-19.4217853942311,0.40143836211972,-326.399647433405)) ;
#28164=CARTESIAN_POINT('Ctrl Pts',(-19.4169157293098,0.591848276379656,
-326.402028042702)) ;
#28165=CARTESIAN_POINT('Ctrl Pts',(-19.4040704711969,0.91060412856428,-326.405985768708)) ;
#28166=CARTESIAN_POINT('Ctrl Pts',(-19.3976192930046,1.03899785641799,-326.407572465259)) ;
#28167=CARTESIAN_POINT('Ctrl Pts',(-19.3819955857502,1.29851752842469,-326.410764897464)) ;
#28168=CARTESIAN_POINT('Ctrl Pts',(-19.3727656510467,1.42963342915828,-326.412370177779)) ;
#28169=CARTESIAN_POINT('Ctrl Pts',(-19.3455785415224,1.76693127132444,-326.416481552516)) ;
#28170=CARTESIAN_POINT('Ctrl Pts',(-19.3256557537582,1.97293819067365,-326.418974923173)) ;
#28171=CARTESIAN_POINT('Ctrl Pts',(-19.2682214071699,2.48181069053854,-326.425099669427)) ;
#28172=CARTESIAN_POINT('Ctrl Pts',(-19.2268575651396,2.78418553543426,-326.428708397974)) ;
#28173=CARTESIAN_POINT('Ctrl Pts',(-19.0877464440495,3.64886263065718,-326.438998951925)) ;
#28174=CARTESIAN_POINT('Ctrl Pts',(-18.9723227875187,4.20799586502152,-326.445611176658)) ;
#28175=CARTESIAN_POINT('Ctrl Pts',(-18.8002227631502,4.88871551045755,-326.453883795848)) ;
#28176=CARTESIAN_POINT('Ctrl Pts',(-18.7666992383657,5.01586631932116,-326.45543919765)) ;
#28177=CARTESIAN_POINT('Ctrl Pts',(-18.7107365703249,5.2197073280047,-326.457954813923)) ;
#28178=CARTESIAN_POINT('Ctrl Pts',(-18.6891107449705,5.29661657489869,-326.458909047071)) ;
#28179=CARTESIAN_POINT('Ctrl Pts',(-18.6346501320464,5.48581126088675,-326.461271084028)) ;
#28180=CARTESIAN_POINT('Ctrl Pts',(-18.601274289553,5.59793760944688,-326.462683708287)) ;
#28181=CARTESIAN_POINT('Ctrl Pts',(-18.5464308537617,5.77627657972418,-326.464955378113)) ;
#28182=CARTESIAN_POINT('Ctrl Pts',(-18.5256166996999,5.84268726129053,-326.465806852828)) ;
#28183=CARTESIAN_POINT('Ctrl Pts',(-18.4852433312548,5.96911961220802,-326.467439621567)) ;
#28184=CARTESIAN_POINT('Ctrl Pts',(-18.4657475535596,6.0291605748689,-326.468220022683)) ;
#28185=CARTESIAN_POINT('Ctrl Pts',(-18.4086522976568,6.20212141369821,-326.470481520566)) ;
#28186=CARTESIAN_POINT('Ctrl Pts',(-18.3703073048129,6.31479207182117,-326.471971217166)) ;
#28187=CARTESIAN_POINT('Ctrl Pts',(-18.1757514643359,6.86969049614925,-326.479377466814)) ;
#28188=CARTESIAN_POINT('Ctrl Pts',(-18.0045956924264,7.30651227905421,-326.485423242565)) ;
#28189=CARTESIAN_POINT('Ctrl Pts',(-17.6351801819628,8.15728368714465,-326.497389157054)) ;
#28190=CARTESIAN_POINT('Ctrl Pts',(-17.4377276249001,8.57126092051048,-326.503305230595)) ;
#28191=CARTESIAN_POINT('Ctrl Pts',(-17.1597128363458,9.1046874695533,-326.510966440903)) ;
#28192=CARTESIAN_POINT('Ctrl Pts',(-17.0922149949562,9.23077814535845,-326.512780626114)) ;
#28193=CARTESIAN_POINT('Ctrl Pts',(-16.9204235871593,9.54335050121665,-326.517283503009)) ;
#28194=CARTESIAN_POINT('Ctrl Pts',(-16.8144340916416,9.72887863851595,-326.519961131176)) ;
#28195=CARTESIAN_POINT('Ctrl Pts',(-16.6377193158365,10.0266900924194,-326.524265151485)) ;
#28196=CARTESIAN_POINT('Ctrl Pts',(-16.5688664539945,10.1400632507185,-326.525905095414)) ;
#28197=CARTESIAN_POINT('Ctrl Pts',(-16.4322203865016,10.359956460082,-326.529088993722)) ;
#28198=CARTESIAN_POINT('Ctrl Pts',(-16.3645390768141,10.4665383741401,-326.530633694216)) ;
#28199=CARTESIAN_POINT('Ctrl Pts',(-16.211803027728,10.7019576948073,-326.534049881169)) ;
#28200=CARTESIAN_POINT('Ctrl Pts',(-16.1262417074583,10.8304563333017,-326.535917383032)) ;
#28201=CARTESIAN_POINT('Ctrl Pts',(-15.7603824333162,11.3659661551318,-326.543717928671)) ;
#28202=CARTESIAN_POINT('Ctrl Pts',(-15.4661370481975,11.76322435966,-326.549543464933)) ;
#28203=CARTESIAN_POINT('Ctrl Pts',(-15.0656645521474,12.2628599185116,-326.557038305064)) ;
#28204=CARTESIAN_POINT('Ctrl Pts',(-14.9729816596672,12.3758556071624,-326.558745437124)) ;
#28205=CARTESIAN_POINT('Ctrl Pts',(-14.6373134279127,12.7757996065916,-326.564843734692)) ;
#28206=CARTESIAN_POINT('Ctrl Pts',(-14.3872834467677,13.0567252514564,-326.569230499365)) ;
#28207=CARTESIAN_POINT('Ctrl Pts',(-13.9826765814699,13.4855851310261,-326.57620740386)) ;
#28208=CARTESIAN_POINT('Ctrl Pts',(-13.8335419401867,13.6385251329558,-326.578755097916)) ;
#28209=CARTESIAN_POINT('Ctrl Pts',(-13.6208870077426,13.8495289998455,-326.582377559289)) ;
#28210=CARTESIAN_POINT('Ctrl Pts',(-13.5594570123582,13.909677994085,-326.583422830523)) ;
#28211=CARTESIAN_POINT('Ctrl Pts',(-13.450403557329,14.015048400752,-326.585278427793)) ;
#28212=CARTESIAN_POINT('Ctrl Pts',(-13.4029464126472,14.0604397147933,-326.586086058009)) ;
#28213=CARTESIAN_POINT('Ctrl Pts',(-13.2919196433035,14.1655605502076,-326.587975791306)) ;
#28214=CARTESIAN_POINT('Ctrl Pts',(-13.2281762027638,14.2251041411655,-326.589060738497)) ;
#28215=CARTESIAN_POINT('Ctrl Pts',(-13.0036928778213,14.4319832617551,-326.592878049277)) ;
#28216=CARTESIAN_POINT('Ctrl Pts',(-12.8408753597593,14.5770397896641,-326.595640351685)) ;
#28217=CARTESIAN_POINT('Ctrl Pts',(-12.4854226354363,14.8831404312769,-326.601626730429)) ;
#28218=CARTESIAN_POINT('Ctrl Pts',(-12.2920368979304,15.0432535110859,-326.604856772879)) ;
#28219=CARTESIAN_POINT('Ctrl Pts',(-11.8013888222586,15.4337042188982,-326.612940931139)) ;
#28220=CARTESIAN_POINT('Ctrl Pts',(-11.5004388587213,15.6592436124706,-326.617800394264)) ;
#28221=CARTESIAN_POINT('Ctrl Pts',(-10.9654012677338,16.0364659855446,-326.626196764321)) ;
#28222=CARTESIAN_POINT('Ctrl Pts',(-10.7342407951735,16.1921073743383,-326.629749773492)) ;
#28223=CARTESIAN_POINT('Ctrl Pts',(-10.3152103388906,16.4613245202135,-326.636042206763)) ;
#28224=CARTESIAN_POINT('Ctrl Pts',(-10.1286121238894,16.5767905815426,-326.638793725256)) ;
#28225=CARTESIAN_POINT('Ctrl Pts',(-9.8252477072782,16.75747601166,-326.643184020207)) ;
#28226=CARTESIAN_POINT('Ctrl Pts',(-9.70969460043107,16.824693923377,-326.64483740475)) ;
#28227=CARTESIAN_POINT('Ctrl Pts',(-9.48417967702382,16.9527801429671,-326.648027983342)) ;
#28228=CARTESIAN_POINT('Ctrl Pts',(-9.37430274110752,17.0137846138908,-326.649566133985)) ;
#28229=CARTESIAN_POINT('Ctrl Pts',(-9.13050497006459,17.1460641694138,-326.652943963231)) ;
#28230=CARTESIAN_POINT('Ctrl Pts',(-8.99632546631366,17.2168454048308,-326.654779987933)) ;
#28231=CARTESIAN_POINT('Ctrl Pts',(-8.13862720077039,17.6565264678724,-326.666378870111)) ;
#28232=CARTESIAN_POINT('Ctrl Pts',(-7.3934038179297,17.9813169280277,-326.675802315083)) ;
#28233=CARTESIAN_POINT('Ctrl Pts',(-6.37883472138951,18.3497280544541,-326.688435679527)) ;
#28234=CARTESIAN_POINT('Ctrl Pts',(-6.12576988629633,18.4357531722914,-326.691575097347)) ;
#28235=CARTESIAN_POINT('Ctrl Pts',(-5.70534778763784,18.5690558471199,-326.69681806525)) ;
#28236=CARTESIAN_POINT('Ctrl Pts',(-5.53898708887837,18.6193568710062,-326.698899779634)) ;
#28237=CARTESIAN_POINT('Ctrl Pts',(-5.29502102269627,18.6895636533388,-326.701975830538)) ;
#28238=CARTESIAN_POINT('Ctrl Pts',(-5.21793177330242,18.7112325935651,-326.702951187957)) ;
#28239=CARTESIAN_POINT('Ctrl Pts',(-5.07678876141961,18.7499662566094,-326.704744824141)) ;
#28240=CARTESIAN_POINT('Ctrl Pts',(-5.01277756209331,18.7671809239495,-326.705561360914)) ;
#28241=CARTESIAN_POINT('Ctrl Pts',(-4.8549728558136,18.8087547158566,-326.707581380328)) ;
#28242=CARTESIAN_POINT('Ctrl Pts',(-4.76108285627282,18.8327402517897,-326.708789196085)) ;
#28243=CARTESIAN_POINT('Ctrl Pts',(-4.37929532780558,18.9272357411706,-326.71371914427)) ;
#28244=CARTESIAN_POINT('Ctrl Pts',(-4.08998137092024,18.9918543633728,-326.717497169695)) ;
#28245=CARTESIAN_POINT('Ctrl Pts',(-3.38409270725106,19.1326370003252,-326.726733920288)) ;
#28246=CARTESIAN_POINT('Ctrl Pts',(-2.96628603633385,19.2018496334634,-326.732215253516)) ;
#28247=CARTESIAN_POINT('Ctrl Pts',(-2.21547069081826,19.3011358853055,-326.741962961426)) ;
#28248=CARTESIAN_POINT('Ctrl Pts',(-1.88331468709704,19.3363720294197,-326.746240436351)) ;
#28249=CARTESIAN_POINT('Ctrl Pts',(-1.43374050038611,19.3723698468136,-326.751956792317)) ;
#28250=CARTESIAN_POINT('Ctrl Pts',(-1.31698350369383,19.3806573621626,-326.753434844355)) ;
#28251=CARTESIAN_POINT('Ctrl Pts',(-1.01465236074945,19.3993724137168,-326.757244160989)) ;
#28252=CARTESIAN_POINT('Ctrl Pts',(-0.828990618031794,19.4081927073741,
-326.759565907703)) ;
#28253=CARTESIAN_POINT('Ctrl Pts',(-0.51551396487016,19.4185787284142,-326.76345543232)) ;
#28254=CARTESIAN_POINT('Ctrl Pts',(-0.387758458352586,19.4215498328149,
-326.765032051854)) ;
#28255=CARTESIAN_POINT('Ctrl Pts',(-0.127468386899953,19.4250338491352,
-326.768227283868)) ;
#28256=CARTESIAN_POINT('Ctrl Pts',(0.00506085209851253,19.4254514149154,
-326.76984519909)) ;
#28257=CARTESIAN_POINT('Ctrl Pts',(0.350604160773705,19.4230039272076,-326.774041681859)) ;
#28258=CARTESIAN_POINT('Ctrl Pts',(0.563585213194563,19.4179910585613,-326.776606421316)) ;
#28259=CARTESIAN_POINT('Ctrl Pts',(1.06641434098791,19.3978762912909,-326.782620081931)) ;
#28260=CARTESIAN_POINT('Ctrl Pts',(1.35609168051833,19.379779665416,-326.786051630194)) ;
#28261=CARTESIAN_POINT('Ctrl Pts',(2.21643349375359,19.3066478154842,-326.796198434957)) ;
#28262=CARTESIAN_POINT('Ctrl Pts',(2.78518184728668,19.2328361847249,-326.802840276206)) ;
#28263=CARTESIAN_POINT('Ctrl Pts',(3.47963108027146,19.1112573385091,-326.811146429254)) ;
#28264=CARTESIAN_POINT('Ctrl Pts',(3.60919668228023,19.0872127030689,-326.812705103974)) ;
#28265=CARTESIAN_POINT('Ctrl Pts',(3.90112088561237,19.0299590408481,-326.816245283378)) ;
#28266=CARTESIAN_POINT('Ctrl Pts',(4.06331934401819,18.9959869714271,-326.818232137123)) ;
#28267=CARTESIAN_POINT('Ctrl Pts',(4.30190850520698,18.9428193966634,-326.821195501288)) ;
#28268=CARTESIAN_POINT('Ctrl Pts',(4.37864916820153,18.9252280018726,-326.822154913167)) ;
#28269=CARTESIAN_POINT('Ctrl Pts',(4.52009965707808,18.8918966459503,-326.823936532402)) ;
#28270=CARTESIAN_POINT('Ctrl Pts',(4.58483943251127,18.8762895488931,-326.824757225824)) ;
#28271=CARTESIAN_POINT('Ctrl Pts',(4.74597797907024,18.8365652969513,-326.826812416131)) ;
#28272=CARTESIAN_POINT('Ctrl Pts',(4.84227431934409,18.8120407861977,-326.828051622884)) ;
#28273=CARTESIAN_POINT('Ctrl Pts',(5.28051954548772,18.6968416508085,-326.833734939378)) ;
#28274=CARTESIAN_POINT('Ctrl Pts',(5.62013976179984,18.597575180194,-326.838259710248)) ;
#28275=CARTESIAN_POINT('Ctrl Pts',(6.14449427084479,18.4286374120117,-326.845346542195)) ;
#28276=CARTESIAN_POINT('Ctrl Pts',(6.33119880152189,18.3653316989743,-326.847890471851)) ;
#28277=CARTESIAN_POINT('Ctrl Pts',(6.92267888964475,18.1546874135974,-326.85599113061)) ;
#28278=CARTESIAN_POINT('Ctrl Pts',(7.32353232626315,17.9967228539168,-326.861541019357)) ;
#28279=CARTESIAN_POINT('Ctrl Pts',(7.84525898845189,17.7708054413704,-326.868775756652)) ;
#28280=CARTESIAN_POINT('Ctrl Pts',(7.97112910764784,17.7147033684803,-326.870522373045)) ;
#28281=CARTESIAN_POINT('Ctrl Pts',(8.28569430994319,17.5704656939094,-326.874888209231)) ;
#28282=CARTESIAN_POINT('Ctrl Pts',(8.4735890077257,17.4806259738571,-326.877496640646)) ;
#28283=CARTESIAN_POINT('Ctrl Pts',(8.77786350279586,17.3290817468366,-326.88171984838)) ;
#28284=CARTESIAN_POINT('Ctrl Pts',(8.89512423676782,17.2691843099321,-326.883347212538)) ;
#28285=CARTESIAN_POINT('Ctrl Pts',(9.12417182708066,17.1492336120069,-326.886525942127)) ;
#28286=CARTESIAN_POINT('Ctrl Pts',(9.23599725188932,17.0892679720819,-326.888077845917)) ;
#28287=CARTESIAN_POINT('Ctrl Pts',(9.51213956912431,16.93768628315,-326.891911194318)) ;
#28288=CARTESIAN_POINT('Ctrl Pts',(9.67572832927351,16.8447706204523,-326.894182984249)) ;
#28289=CARTESIAN_POINT('Ctrl Pts',(10.1432975643564,16.5701402892212,-326.900686451099)) ;
#28290=CARTESIAN_POINT('Ctrl Pts',(10.4436919697828,16.3824703078355,-326.904876303068)) ;
#28291=CARTESIAN_POINT('Ctrl Pts',(10.9263956157162,16.0622287328839,-326.911679817405)) ;
#28292=CARTESIAN_POINT('Ctrl Pts',(11.1118249508326,15.9345115816321,-326.914311551687)) ;
#28293=CARTESIAN_POINT('Ctrl Pts',(11.6138873146571,15.5756825500852,-326.921519803855)) ;
#28294=CARTESIAN_POINT('Ctrl Pts',(11.9258103246577,15.3381652355206,-326.926089391126)) ;
#28295=CARTESIAN_POINT('Ctrl Pts',(12.3138570314817,15.0236849062668,-326.931996915015)) ;
#28296=CARTESIAN_POINT('Ctrl Pts',(12.396817733595,14.9553031799335,-326.933273495691)) ;
#28297=CARTESIAN_POINT('Ctrl Pts',(12.532230505283,14.84178597579,-326.935382983852)) ;
#28298=CARTESIAN_POINT('Ctrl Pts',(12.5850166949285,14.7970526513474,-326.936211844289)) ;
#28299=CARTESIAN_POINT('Ctrl Pts',(12.7176539612149,14.6834268770724,-326.9383125494)) ;
#28300=CARTESIAN_POINT('Ctrl Pts',(12.797185043915,14.614164431753,-326.939588802726)) ;
#28301=CARTESIAN_POINT('Ctrl Pts',(12.9266949756125,14.4995082511701,-326.941697952982)) ;
#28302=CARTESIAN_POINT('Ctrl Pts',(12.9770082687524,14.4544954571736,-326.942525138341)) ;
#28303=CARTESIAN_POINT('Ctrl Pts',(13.0834603998713,14.3582542350868,-326.944292938768)) ;
#28304=CARTESIAN_POINT('Ctrl Pts',(13.1395352190539,14.3069568714883,-326.945234554135)) ;
#28305=CARTESIAN_POINT('Ctrl Pts',(13.3055221977264,14.1533126592461,-326.948050956018)) ;
#28306=CARTESIAN_POINT('Ctrl Pts',(13.4145499204461,14.0500188790203,-326.949939293338)) ;
#28307=CARTESIAN_POINT('Ctrl Pts',(13.9435881772821,13.5370315320262,-326.959268730439)) ;
#28308=CARTESIAN_POINT('Ctrl Pts',(14.3460860275177,13.1097173707736,-326.966881115572)) ;
#28309=CARTESIAN_POINT('Ctrl Pts',(15.0479269879425,12.2935089164111,-326.980748229276)) ;
#28310=CARTESIAN_POINT('Ctrl Pts',(15.3530730676705,11.910231643154,-326.98701626338)) ;
#28311=CARTESIAN_POINT('Ctrl Pts',(15.7530244135387,11.3669272550445,-326.995499113101)) ;
#28312=CARTESIAN_POINT('Ctrl Pts',(15.8605087765957,11.2164644559859,-326.997808573495)) ;
#28313=CARTESIAN_POINT('Ctrl Pts',(16.0385270504444,10.9595877914989,-327.001683897558)) ;
#28314=CARTESIAN_POINT('Ctrl Pts',(16.1101897736959,10.8539716239569,-327.003258450649)) ;
#28315=CARTESIAN_POINT('Ctrl Pts',(16.2542690027723,10.6370575408265,-327.006454546226)) ;
#28316=CARTESIAN_POINT('Ctrl Pts',(16.3265956981309,10.5257079052748,-327.008075338598)) ;
#28317=CARTESIAN_POINT('Ctrl Pts',(16.5127144504539,10.2326367289967,-327.01229112414)) ;
#28318=CARTESIAN_POINT('Ctrl Pts',(16.6246495012352,10.0497573166538,-327.014872034383)) ;
#28319=CARTESIAN_POINT('Ctrl Pts',(16.8792194207854,9.61794509212463,-327.020861112411)) ;
#28320=CARTESIAN_POINT('Ctrl Pts',(17.0194127028395,9.36763084537578,-327.024253050164)) ;
#28321=CARTESIAN_POINT('Ctrl Pts',(17.4232517264209,8.60756629500385,-327.034367776071)) ;
#28322=CARTESIAN_POINT('Ctrl Pts',(17.6699057975651,8.08914863716062,-327.04101630178)) ;
#28323=CARTESIAN_POINT('Ctrl Pts',(17.9445618546604,7.43913342215355,-327.049330020752)) ;
#28324=CARTESIAN_POINT('Ctrl Pts',(17.9946379332251,7.31717239310941,-327.050889431504)) ;
#28325=CARTESIAN_POINT('Ctrl Pts',(18.1048650624446,7.04073603725965,-327.054430972021)) ;
#28326=CARTESIAN_POINT('Ctrl Pts',(18.164288078721,6.88598150726406,-327.056418449987)) ;
#28327=CARTESIAN_POINT('Ctrl Pts',(18.249005064677,6.65662369761279,-327.059382557331)) ;
#28328=CARTESIAN_POINT('Ctrl Pts',(18.2758377904471,6.58259659547528,-327.06034207608)) ;
#28329=CARTESIAN_POINT('Ctrl Pts',(18.3245314776524,6.44566564471362,-327.062123772411)) ;
#28330=CARTESIAN_POINT('Ctrl Pts',(18.346520441426,6.38280871839717,-327.06294443451)) ;
#28331=CARTESIAN_POINT('Ctrl Pts',(18.400509248801,6.22589391674672,-327.064999372723)) ;
#28332=CARTESIAN_POINT('Ctrl Pts',(18.4321115094623,6.13170130891736,-327.066238356017)) ;
#28333=CARTESIAN_POINT('Ctrl Pts',(18.5725357075435,5.70226046808324,-327.071905136891)) ;
#28334=CARTESIAN_POINT('Ctrl Pts',(18.6729431250667,5.36433138867651,-327.07641297421)) ;
#28335=CARTESIAN_POINT('Ctrl Pts',(18.7798106867995,4.96518130934419,-327.081728324813)) ;
#28336=CARTESIAN_POINT('Ctrl Pts',(18.7952455618037,4.90643038635758,-327.082510498498)) ;
#28337=CARTESIAN_POINT('Ctrl Pts',(18.8309155779598,4.76801832205315,-327.084352213789)) ;
#28338=CARTESIAN_POINT('Ctrl Pts',(18.8509212114941,4.68829923311079,-327.085412165662)) ;
#28339=CARTESIAN_POINT('Ctrl Pts',(18.981086972907,4.15530448543709,-327.092489940947)) ;
#28340=CARTESIAN_POINT('Ctrl Pts',(19.0753950898941,3.69831333694448,-327.098511001347)) ;
#28341=CARTESIAN_POINT('Ctrl Pts',(19.1772426807593,3.09594157992855,-327.106293653917)) ;
#28342=CARTESIAN_POINT('Ctrl Pts',(19.1997348651637,2.9532477496082,-327.108126448232)) ;
#28343=CARTESIAN_POINT('Ctrl Pts',(19.2517566517433,2.5974544506631,-327.112666858757)) ;
#28344=CARTESIAN_POINT('Ctrl Pts',(19.2793417520502,2.38409010747144,-327.115363339038)) ;
#28345=CARTESIAN_POINT('Ctrl Pts',(19.3182263570742,2.03823918787935,-327.11968937501)) ;
#28346=CARTESIAN_POINT('Ctrl Pts',(19.3317196393601,1.9060179465516,-327.121332749321)) ;
#28347=CARTESIAN_POINT('Ctrl Pts',(19.3553685856004,1.64809952955765,-327.124518247665)) ;
#28348=CARTESIAN_POINT('Ctrl Pts',(19.3656592611102,1.52242128688295,-327.126061172561)) ;
#28349=CARTESIAN_POINT('Ctrl Pts',(19.3857736734706,1.2433887798575,-327.129467113427)) ;
#28350=CARTESIAN_POINT('Ctrl Pts',(19.3950028745052,1.0900000722004,-327.131326233167)) ;
#28351=CARTESIAN_POINT('Ctrl Pts',(19.4203187599284,0.565515471158907,-327.137642767645)) ;
#28352=CARTESIAN_POINT('Ctrl Pts',(19.4275815287433,0.194075331456793,-327.142045639433)) ;
#28353=CARTESIAN_POINT('Ctrl Pts',(19.4188878079119,-0.758129904308238,
-327.15324050368)) ;
#28354=CARTESIAN_POINT('Ctrl Pts',(19.3875395894411,-1.33838394875235,-327.159968867587)) ;
#28355=CARTESIAN_POINT('Ctrl Pts',(19.3171599756559,-2.04830057614149,-327.168372876977)) ;
#28356=CARTESIAN_POINT('Ctrl Pts',(19.3027289955938,-2.18010505419259,-327.169941003362)) ;
#28357=CARTESIAN_POINT('Ctrl Pts',(19.2671475067596,-2.47696154579646,-327.17349864906)) ;
#28358=CARTESIAN_POINT('Ctrl Pts',(19.2452233374695,-2.64191030987806,-327.175493506102)) ;
#28359=CARTESIAN_POINT('Ctrl Pts',(19.2097909069459,-2.88457535717359,-327.178466397096)) ;
#28360=CARTESIAN_POINT('Ctrl Pts',(19.1979242139874,-2.96252384513382,-327.179427177242)) ;
#28361=CARTESIAN_POINT('Ctrl Pts',(19.1751646178104,-3.10614193384714,-327.181209787227)) ;
#28362=CARTESIAN_POINT('Ctrl Pts',(19.1644081246981,-3.17183180952745,-327.182030083349)) ;
#28363=CARTESIAN_POINT('Ctrl Pts',(19.1367901629798,-3.33522368853037,-327.184082063747)) ;
#28364=CARTESIAN_POINT('Ctrl Pts',(19.1195179375013,-3.43285429249027,-327.185318423672)) ;
#28365=CARTESIAN_POINT('Ctrl Pts',(19.0420080899544,-3.85223339227551,-327.190667176932)) ;
#28366=CARTESIAN_POINT('Ctrl Pts',(18.9743904370142,-4.17256288354558,-327.194847928542)) ;
#28367=CARTESIAN_POINT('Ctrl Pts',(18.8810942157753,-4.56516289976145,-327.200034068147)) ;
#28368=CARTESIAN_POINT('Ctrl Pts',(18.8630413877299,-4.63919181395662,-327.201014766755)) ;
#28369=CARTESIAN_POINT('Ctrl Pts',(18.8102783724116,-4.85015547072424,-327.203816128341)) ;
#28370=CARTESIAN_POINT('Ctrl Pts',(18.774509391943,-4.98682039187714,-327.205638843419)) ;
#28371=CARTESIAN_POINT('Ctrl Pts',(18.6225570124736,-5.54257367454252,-327.213072340069)) ;
#28372=CARTESIAN_POINT('Ctrl Pts',(18.4938059199857,-5.95809502764049,-327.218676949637)) ;
#28373=CARTESIAN_POINT('Ctrl Pts',(18.2837437210495,-6.5633596971502,-327.226830804255)) ;
#28374=CARTESIAN_POINT('Ctrl Pts',(18.2131849662172,-6.75669065016525,-327.229434306104)) ;
#28375=CARTESIAN_POINT('Ctrl Pts',(18.0761830509373,-7.11432543246064,-327.234243838602)) ;
#28376=CARTESIAN_POINT('Ctrl Pts',(18.01053751618,-7.27891190774359,-327.236454622286)) ;
#28377=CARTESIAN_POINT('Ctrl Pts',(17.894209358965,-7.55935713985805,-327.240216487136)) ;
#28378=CARTESIAN_POINT('Ctrl Pts',(17.8446303598341,-7.67566129532896,-327.241775057365)) ;
#28379=CARTESIAN_POINT('Ctrl Pts',(17.7397433524522,-7.91519891632897,-327.244982329021)) ;
#28380=CARTESIAN_POINT('Ctrl Pts',(17.6842782326749,-8.03835627128352,-327.246629820291)) ;
#28381=CARTESIAN_POINT('Ctrl Pts',(17.5321069189807,-8.36704509027079,-327.251024339532)) ;
#28382=CARTESIAN_POINT('Ctrl Pts',(17.4330726928829,-8.57147556109847,-327.253754844565)) ;
#28383=CARTESIAN_POINT('Ctrl Pts',(17.2497861146696,-8.93349964869672,-327.258595143417)) ;
#28384=CARTESIAN_POINT('Ctrl Pts',(17.166901407133,-9.09175632912777,-327.260712814534)) ;
#28385=CARTESIAN_POINT('Ctrl Pts',(16.775653698174,-9.81435804617473,-327.270408558365)) ;
#28386=CARTESIAN_POINT('Ctrl Pts',(16.4415688540731,-10.3643134021324,-327.27784875193)) ;
#28387=CARTESIAN_POINT('Ctrl Pts',(15.9258105210219,-11.1254458842784,-327.288670960781)) ;
#28388=CARTESIAN_POINT('Ctrl Pts',(15.7659326777758,-11.350874551876,-327.291948587657)) ;
#28389=CARTESIAN_POINT('Ctrl Pts',(15.5458449519907,-11.6475745995569,-327.296406047861)) ;
#28390=CARTESIAN_POINT('Ctrl Pts',(15.4898527694988,-11.7219345873691,-327.297535615674)) ;
#28391=CARTESIAN_POINT('Ctrl Pts',(15.3933077424548,-11.8482507200985,-327.299478208889)) ;
#28392=CARTESIAN_POINT('Ctrl Pts',(15.3530210190997,-11.9004081428921,-327.300287437464)) ;
#28393=CARTESIAN_POINT('Ctrl Pts',(15.2616897803332,-12.0174148975402,-327.302119351405)) ;
#28394=CARTESIAN_POINT('Ctrl Pts',(15.2104959819746,-12.0821458247054,-327.303144145037)) ;
#28395=CARTESIAN_POINT('Ctrl Pts',(15.0404706456332,-12.2943374273616,-327.306538184947)) ;
#28396=CARTESIAN_POINT('Ctrl Pts',(14.9198952264532,-12.4403864989065,-327.308929938267)) ;
#28397=CARTESIAN_POINT('Ctrl Pts',(14.2348467673596,-13.2458759318782,-327.322382459771)) ;
#28398=CARTESIAN_POINT('Ctrl Pts',(13.6288001022259,-13.8686665222032,-327.333731456611)) ;
#28399=CARTESIAN_POINT('Ctrl Pts',(12.7848484682549,-14.6270071331188,-327.34813954358)) ;
#28400=CARTESIAN_POINT('Ctrl Pts',(12.5829148230552,-14.8010791164603,-327.351496854248)) ;
#28401=CARTESIAN_POINT('Ctrl Pts',(12.2680753927485,-15.0613776135139,-327.356589441689)) ;
#28402=CARTESIAN_POINT('Ctrl Pts',(12.1577003724024,-15.1506135579832,-327.358349082568)) ;
#28403=CARTESIAN_POINT('Ctrl Pts',(11.9486771657956,-15.3158494025382,-327.361633720247)) ;
#28404=CARTESIAN_POINT('Ctrl Pts',(11.8502568530145,-15.3921259577127,-327.36316094445)) ;
#28405=CARTESIAN_POINT('Ctrl Pts',(11.6243782033614,-15.5637330852144,-327.366622955208)) ;
#28406=CARTESIAN_POINT('Ctrl Pts',(11.4964678627484,-15.6584540404362,-327.368552761204)) ;
#28407=CARTESIAN_POINT('Ctrl Pts',(11.047361194786,-15.9825595979927,-327.375227595896)) ;
#28408=CARTESIAN_POINT('Ctrl Pts',(10.7203492351549,-16.2037191385582,-327.379909129434)) ;
#28409=CARTESIAN_POINT('Ctrl Pts',(9.89504163043827,-16.7259519144703,-327.391391715019)) ;
#28410=CARTESIAN_POINT('Ctrl Pts',(9.38952089888908,-17.0148820705078,-327.398133363672)) ;
#28411=CARTESIAN_POINT('Ctrl Pts',(8.75373157925027,-17.3412923698082,-327.406552383494)) ;
#28412=CARTESIAN_POINT('Ctrl Pts',(8.63505115936703,-17.4006933494354,-327.408121946701)) ;
#28413=CARTESIAN_POINT('Ctrl Pts',(8.36612745928314,-17.5318640565301,-327.411682245256)) ;
#28414=CARTESIAN_POINT('Ctrl Pts',(8.21555138894398,-17.6029276310768,-327.413678316559)) ;
#28415=CARTESIAN_POINT('Ctrl Pts',(7.99233402880609,-17.704785827853,-327.41665265265)) ;
#28416=CARTESIAN_POINT('Ctrl Pts',(7.92038876206054,-17.7370878747095,-327.417613640019)) ;
#28417=CARTESIAN_POINT('Ctrl Pts',(7.78736326845427,-17.7958430136533,-327.41939640075)) ;
#28418=CARTESIAN_POINT('Ctrl Pts',(7.72634007583802,-17.822421952097,-327.420216637401)) ;
#28419=CARTESIAN_POINT('Ctrl Pts',(7.57411262774205,-17.8877965671262,-327.42226813498)) ;
#28420=CARTESIAN_POINT('Ctrl Pts',(7.48274582578998,-17.9262088293292,-327.423504066407)) ;
#28421=CARTESIAN_POINT('Ctrl Pts',(7.09120926126737,-18.0873029356201,-327.42881389943)) ;
#28422=CARTESIAN_POINT('Ctrl Pts',(6.78828727432972,-18.2031571831574,-327.43295479199)) ;
#28423=CARTESIAN_POINT('Ctrl Pts',(6.34418467701447,-18.360378763321,-327.43900869954)) ;
#28424=CARTESIAN_POINT('Ctrl Pts',(6.20520995065933,-18.4078123901962,-327.440900955598)) ;
#28425=CARTESIAN_POINT('Ctrl Pts',(5.60697026383333,-18.6044534814421,-327.449022699918)) ;
#28426=CARTESIAN_POINT('Ctrl Pts',(5.14276569758894,-18.7380833411738,-327.455260464921)) ;
#28427=CARTESIAN_POINT('Ctrl Pts',(4.53106214377643,-18.8897275630234,-327.46329263949)) ;
#28428=CARTESIAN_POINT('Ctrl Pts',(4.3876606325768,-18.9235505598868,-327.465162792236)) ;
#28429=CARTESIAN_POINT('Ctrl Pts',(4.03109937961599,-19.0033789474859,-327.469778282066)) ;
#28430=CARTESIAN_POINT('Ctrl Pts',(3.81752330056982,-19.0474326280615,-327.472512342319)) ;
#28431=CARTESIAN_POINT('Ctrl Pts',(3.47213376834506,-19.11263237607,-327.47688225734)) ;
#28432=CARTESIAN_POINT('Ctrl Pts',(3.34076527546002,-19.1360318948384,-327.478532468078)) ;
#28433=CARTESIAN_POINT('Ctrl Pts',(3.08509292417461,-19.178859526517,-327.481721372759)) ;
#28434=CARTESIAN_POINT('Ctrl Pts',(2.96082076117948,-19.1984372165268,-327.483260974537)) ;
#28435=CARTESIAN_POINT('Ctrl Pts',(2.68569648657068,-19.2390450797176,-327.486647442526)) ;
#28436=CARTESIAN_POINT('Ctrl Pts',(2.53476941735258,-19.25951103426,-327.488490580372)) ;
#28437=CARTESIAN_POINT('Ctrl Pts',(1.59268795407757,-19.3759929441759,-327.499912650502)) ;
#28438=CARTESIAN_POINT('Ctrl Pts',(0.796488855829417,-19.425018978354,-327.509167151829)) ;
#28439=CARTESIAN_POINT('Ctrl Pts',(-0.000462715166402311,-19.4249999944889,
-327.51849135163)) ;
#28440=CARTESIAN_POINT('Origin',(0.,0.,-328.125)) ;
#28441=CARTESIAN_POINT('',(0.000354632730933767,-19.4249999967628,-329.231156838445)) ;
#28442=CARTESIAN_POINT('',(0.000234857373855835,-19.4249998715866,-329.01970498129)) ;
#28443=CARTESIAN_POINT('',(-2.37887640734373E-15,-19.425,-328.125)) ;
#28444=CARTESIAN_POINT('Ctrl Pts',(0.000354632730933767,-19.4249999967628,
-329.231156838445)) ;
#28445=CARTESIAN_POINT('Ctrl Pts',(0.415569471354703,-19.4249924163884,
-329.226055010052)) ;
#28446=CARTESIAN_POINT('Ctrl Pts',(0.83072768051785,-19.4116674955667,-329.220953181658)) ;
#28447=CARTESIAN_POINT('Ctrl Pts',(1.2449867673168,-19.3850621084691,-329.215851353265)) ;
#28448=CARTESIAN_POINT('Ctrl Pts',(1.65937670872291,-19.3584483173617,-329.210747913325)) ;
#28449=CARTESIAN_POINT('Ctrl Pts',(2.07286675400417,-19.3185456871708,-329.205644473386)) ;
#28450=CARTESIAN_POINT('Ctrl Pts',(2.48461808999774,-19.2654431027904,-329.200541033446)) ;
#28451=CARTESIAN_POINT('Ctrl Pts',(2.84751853597314,-19.2186407007835,-329.19604307444)) ;
#28452=CARTESIAN_POINT('Ctrl Pts',(3.20906834148811,-19.1615854409615,-329.191545115434)) ;
#28453=CARTESIAN_POINT('Ctrl Pts',(3.56869801950147,-19.094371407449,-329.187047156428)) ;
#28454=CARTESIAN_POINT('Ctrl Pts',(3.96544946344926,-19.0202193936415,-329.182084908205)) ;
#28455=CARTESIAN_POINT('Ctrl Pts',(4.359941694972,-18.9336874237587,-329.177122659982)) ;
#28456=CARTESIAN_POINT('Ctrl Pts',(4.7513935665189,-18.8349378596279,-329.17216041176)) ;
#28457=CARTESIAN_POINT('Ctrl Pts',(5.1425489128499,-18.7362630983986,-329.167201922445)) ;
#28458=CARTESIAN_POINT('Ctrl Pts',(5.53066827328683,-18.6253893036814,-329.162243433131)) ;
#28459=CARTESIAN_POINT('Ctrl Pts',(5.91498411383876,-18.5025292307034,-329.157284943817)) ;
#28460=CARTESIAN_POINT('Ctrl Pts',(6.29925871129465,-18.3796823425314,-329.152326986626)) ;
#28461=CARTESIAN_POINT('Ctrl Pts',(6.6797303781206,-18.2448518175426,-329.147369029435)) ;
#28462=CARTESIAN_POINT('Ctrl Pts',(7.05564710108361,-18.0983001683852,-329.142411072244)) ;
#28463=CARTESIAN_POINT('Ctrl Pts',(7.43154097862795,-17.9517574255455,-329.137453416361)) ;
#28464=CARTESIAN_POINT('Ctrl Pts',(7.8028802442326,-17.7934950677717,-329.132495760477)) ;
#28465=CARTESIAN_POINT('Ctrl Pts',(8.16893166101332,-17.6238242307875,-329.127538104594)) ;
#28466=CARTESIAN_POINT('Ctrl Pts',(8.53555551838824,-17.4538880581968,-329.122572695801)) ;
#28467=CARTESIAN_POINT('Ctrl Pts',(8.8968747532441,-17.2725077847233,-329.117607287009)) ;
#28468=CARTESIAN_POINT('Ctrl Pts',(9.25217472367527,-17.0800435562262,-329.112641878216)) ;
#28469=CARTESIAN_POINT('Ctrl Pts',(9.60695632518435,-16.8878601255984,-329.107683713763)) ;
#28470=CARTESIAN_POINT('Ctrl Pts',(9.95573601117668,-16.6846251848545,-329.10272554931)) ;
#28471=CARTESIAN_POINT('Ctrl Pts',(10.2978273866379,-16.4707430346967,-329.097767384856)) ;
#28472=CARTESIAN_POINT('Ctrl Pts',(10.6406685030812,-16.2563921319634,-329.092798353894)) ;
#28473=CARTESIAN_POINT('Ctrl Pts',(10.9767917494116,-16.031347413386,-329.087829322931)) ;
#28474=CARTESIAN_POINT('Ctrl Pts',(11.3055345829969,-15.7960600401702,-329.082860291969)) ;
#28475=CARTESIAN_POINT('Ctrl Pts',(11.6342774165822,-15.5607726669543,-329.077891261006)) ;
#28476=CARTESIAN_POINT('Ctrl Pts',(11.9556396463903,-15.3152427840079,-329.072922230044)) ;
#28477=CARTESIAN_POINT('Ctrl Pts',(12.2689900757296,-15.0599637290948,-329.067953199082)) ;
#28478=CARTESIAN_POINT('Ctrl Pts',(12.5819127809508,-14.8050331307286,-329.062990950859)) ;
#28479=CARTESIAN_POINT('Ctrl Pts',(12.8869287333671,-14.5403121997181,-329.058028702636)) ;
#28480=CARTESIAN_POINT('Ctrl Pts',(13.1834296627393,-14.2663172307223,-329.053066454413)) ;
#28481=CARTESIAN_POINT('Ctrl Pts',(13.4797059923366,-13.9925298132121,-329.048107965099)) ;
#28482=CARTESIAN_POINT('Ctrl Pts',(13.7674800198178,-13.7094825637859,-329.043149475785)) ;
#28483=CARTESIAN_POINT('Ctrl Pts',(14.0461795388355,-13.4177295159352,-329.03819098647)) ;
#28484=CARTESIAN_POINT('Ctrl Pts',(14.3248491490381,-13.1260077777474,-329.033233029279)) ;
#28485=CARTESIAN_POINT('Ctrl Pts',(14.5944460319504,-12.825582278749,-329.028275072088)) ;
#28486=CARTESIAN_POINT('Ctrl Pts',(14.8544354156144,-12.5170433203429,-329.023317114897)) ;
#28487=CARTESIAN_POINT('Ctrl Pts',(15.1144089990605,-12.2085231126362,-329.018359459014)) ;
#28488=CARTESIAN_POINT('Ctrl Pts',(15.3647760967842,-11.8918906120237,-329.013401803131)) ;
#28489=CARTESIAN_POINT('Ctrl Pts',(15.6050416873464,-11.5677698341635,-329.008444147248)) ;
#28490=CARTESIAN_POINT('Ctrl Pts',(15.8456830114029,-11.2431421879156,-329.003478738455)) ;
#28491=CARTESIAN_POINT('Ctrl Pts',(16.0761910565558,-10.9110030089518,-328.998513329663)) ;
#28492=CARTESIAN_POINT('Ctrl Pts',(16.2961105777967,-10.5720104538457,-328.99354792087)) ;
#28493=CARTESIAN_POINT('Ctrl Pts',(16.5157092449555,-10.2335124757761,-328.988589756417)) ;
#28494=CARTESIAN_POINT('Ctrl Pts',(16.7247501452136,-9.88818131222814,-328.983631591964)) ;
#28495=CARTESIAN_POINT('Ctrl Pts',(16.9228239627251,-9.53670037940891,-328.97867342751)) ;
#28496=CARTESIAN_POINT('Ctrl Pts',(17.1213318866479,-9.18444912707794,-328.973704396548)) ;
#28497=CARTESIAN_POINT('Ctrl Pts',(17.308824473051,-8.82602132105644,-328.968735365586)) ;
#28498=CARTESIAN_POINT('Ctrl Pts',(17.4849357707604,-8.46213011554323,-328.963766334623)) ;
#28499=CARTESIAN_POINT('Ctrl Pts',(17.6610470684698,-8.09823891003003,-328.958797303661)) ;
#28500=CARTESIAN_POINT('Ctrl Pts',(17.8257769790622,-7.72888452366728,-328.953828272698)) ;
#28501=CARTESIAN_POINT('Ctrl Pts',(17.9788072554305,-7.35480215043743,-328.948859241736)) ;
#28502=CARTESIAN_POINT('Ctrl Pts',(18.1316286450887,-6.98123040058307,-328.943896993513)) ;
#28503=CARTESIAN_POINT('Ctrl Pts',(18.2728229536204,-6.60284426211896,-328.938934745291)) ;
#28504=CARTESIAN_POINT('Ctrl Pts',(18.4021030494348,-6.22038811956168,-328.933972497068)) ;
#28505=CARTESIAN_POINT('Ctrl Pts',(18.5312852154367,-5.83822168794605,-328.929014007754)) ;
#28506=CARTESIAN_POINT('Ctrl Pts',(18.6485711358642,-5.45199164099182,-328.924055518439)) ;
#28507=CARTESIAN_POINT('Ctrl Pts',(18.7537234030452,-5.06245824892152,-328.919097029125)) ;
#28508=CARTESIAN_POINT('Ctrl Pts',(18.8588643857443,-4.67296665987346,-328.914139071934)) ;
#28509=CARTESIAN_POINT('Ctrl Pts',(18.9518742541405,-4.28017266283976,-328.909181114743)) ;
#28510=CARTESIAN_POINT('Ctrl Pts',(19.0325658242294,-3.88485046641099,-328.904223157552)) ;
#28511=CARTESIAN_POINT('Ctrl Pts',(19.1132524904863,-3.48955229471847,-328.899265501669)) ;
#28512=CARTESIAN_POINT('Ctrl Pts',(19.181622306525,-3.09172646307406,-328.894307845786)) ;
#28513=CARTESIAN_POINT('Ctrl Pts',(19.2375391241372,-2.69215776790513,-328.889350189903)) ;
#28514=CARTESIAN_POINT('Ctrl Pts',(19.2935433859028,-2.29196421696319,-328.88438478111)) ;
#28515=CARTESIAN_POINT('Ctrl Pts',(19.3370556235782,-1.89002258157972,-328.879419372317)) ;
#28516=CARTESIAN_POINT('Ctrl Pts',(19.36799095163,-1.48712860828419,-328.874453963525)) ;
#28517=CARTESIAN_POINT('Ctrl Pts',(19.3988811462339,-1.08482244172293,-328.869495799072)) ;
#28518=CARTESIAN_POINT('Ctrl Pts',(19.417231099536,-0.681566952346034,-328.864537634618)) ;
#28519=CARTESIAN_POINT('Ctrl Pts',(19.4230083425457,-0.278158094259134,
-328.859579470165)) ;
#28520=CARTESIAN_POINT('Ctrl Pts',(19.4287982471895,0.12613489063155,-328.854610439203)) ;
#28521=CARTESIAN_POINT('Ctrl Pts',(19.4219602533177,0.530581678137673,-328.84964140824)) ;
#28522=CARTESIAN_POINT('Ctrl Pts',(19.4025141990856,0.934380947087321,-328.844672377278)) ;
#28523=CARTESIAN_POINT('Ctrl Pts',(19.3830681448536,1.33818021603692,-328.839703346316)) ;
#28524=CARTESIAN_POINT('Ctrl Pts',(19.3510140484364,1.74133172734594,-328.834734315353)) ;
#28525=CARTESIAN_POINT('Ctrl Pts',(19.306424182672,2.14303762886651,-328.829765284391)) ;
#28526=CARTESIAN_POINT('Ctrl Pts',(19.2618951821857,2.54419520082795,-328.824803036168)) ;
#28527=CARTESIAN_POINT('Ctrl Pts',(19.2048527866065,2.94401774602782,-328.819840787945)) ;
#28528=CARTESIAN_POINT('Ctrl Pts',(19.1354009891766,3.3417142282694,-328.814878539723)) ;
#28529=CARTESIAN_POINT('Ctrl Pts',(19.0660018015586,3.73910945499445,-328.809920050408)) ;
#28530=CARTESIAN_POINT('Ctrl Pts',(18.9842120460907,4.13438160453245,-328.804961561094)) ;
#28531=CARTESIAN_POINT('Ctrl Pts',(18.8901869801266,4.52674948012969,-328.80000307178)) ;
#28532=CARTESIAN_POINT('Ctrl Pts',(18.7961720045218,4.91907524852091,-328.795045114589)) ;
#28533=CARTESIAN_POINT('Ctrl Pts',(18.6899243962863,5.30849713474285,-328.790087157398)) ;
#28534=CARTESIAN_POINT('Ctrl Pts',(18.5716501840751,5.69424573059011,-328.785129200207)) ;
#28535=CARTESIAN_POINT('Ctrl Pts',(18.4533831596888,6.07997088351307,-328.780171544324)) ;
#28536=CARTESIAN_POINT('Ctrl Pts',(18.3230910610183,6.46202296516201,-328.77521388844)) ;
#28537=CARTESIAN_POINT('Ctrl Pts',(18.1810297981968,6.83964768661962,-328.770256232557)) ;
#28538=CARTESIAN_POINT('Ctrl Pts',(18.0387463763287,7.2178629473024,-328.765290823765)) ;
#28539=CARTESIAN_POINT('Ctrl Pts',(17.884657022939,7.59163676160008,-328.760325414972)) ;
#28540=CARTESIAN_POINT('Ctrl Pts',(17.719067902185,7.96022975031234,-328.755360006179)) ;
#28541=CARTESIAN_POINT('Ctrl Pts',(17.5537203695582,8.32828497609991,-328.750401841726)) ;
#28542=CARTESIAN_POINT('Ctrl Pts',(17.3769067115698,8.69117427168043,-328.745443677273)) ;
#28543=CARTESIAN_POINT('Ctrl Pts',(17.1889792201584,9.04818315292986,-328.74048551282)) ;
#28544=CARTESIAN_POINT('Ctrl Pts',(17.0006398594255,9.40597446896082,-328.735516481857)) ;
#28545=CARTESIAN_POINT('Ctrl Pts',(16.8011379953144,9.75785934829109,-328.730547450895)) ;
#28546=CARTESIAN_POINT('Ctrl Pts',(16.5908744199071,10.1031436188382,-328.725578419933)) ;
#28547=CARTESIAN_POINT('Ctrl Pts',(16.3806108444999,10.4484278893853,-328.72060938897)) ;
#28548=CARTESIAN_POINT('Ctrl Pts',(16.1595856881402,10.7871113498981,-328.715640358008)) ;
#28549=CARTESIAN_POINT('Ctrl Pts',(15.9282441276453,11.118527960577,-328.710671327045)) ;
#28550=CARTESIAN_POINT('Ctrl Pts',(15.6972183489589,11.4494921867537,-328.705709078823)) ;
#28551=CARTESIAN_POINT('Ctrl Pts',(15.4558429079907,11.7732973736191,-328.7007468306)) ;
#28552=CARTESIAN_POINT('Ctrl Pts',(15.2045875752387,12.0892986424729,-328.695784582377)) ;
#28553=CARTESIAN_POINT('Ctrl Pts',(14.953522568673,12.4050605400237,-328.690826093063)) ;
#28554=CARTESIAN_POINT('Ctrl Pts',(14.6925927805345,12.7130301521005,-328.685867603749)) ;
#28555=CARTESIAN_POINT('Ctrl Pts',(14.4223082903802,13.0125957663039,-328.680909114434)) ;
#28556=CARTESIAN_POINT('Ctrl Pts',(14.1520528059764,13.3121292324346,-328.675951157244)) ;
#28557=CARTESIAN_POINT('Ctrl Pts',(13.8724447836342,13.6032603258739,-328.670993200053)) ;
#28558=CARTESIAN_POINT('Ctrl Pts',(13.584033246719,13.8854119763165,-328.666035242862)) ;
#28559=CARTESIAN_POINT('Ctrl Pts',(13.295639237308,14.1675464796841,-328.661077586978)) ;
#28560=CARTESIAN_POINT('Ctrl Pts',(12.998442951767,14.4407024642955,-328.656119931095)) ;
#28561=CARTESIAN_POINT('Ctrl Pts',(12.6930299823837,14.7043400010442,-328.651162275212)) ;
#28562=CARTESIAN_POINT('Ctrl Pts',(12.3871394003657,14.9683898209346,-328.646196866419)) ;
#28563=CARTESIAN_POINT('Ctrl Pts',(12.0730065872004,15.2228912330626,-328.641231457627)) ;
#28564=CARTESIAN_POINT('Ctrl Pts',(11.7512541315046,15.4673414437258,-328.636266048834)) ;
#28565=CARTESIAN_POINT('Ctrl Pts',(11.4299711002049,15.7114350109803,-328.631307884381)) ;
#28566=CARTESIAN_POINT('Ctrl Pts',(11.1010908420707,15.9455065519856,-328.626349719928)) ;
#28567=CARTESIAN_POINT('Ctrl Pts',(10.765264541436,16.1690972027786,-328.621391555475)) ;
#28568=CARTESIAN_POINT('Ctrl Pts',(10.428702230603,16.3931778836821,-328.616422524512)) ;
#28569=CARTESIAN_POINT('Ctrl Pts',(10.0851635885213,16.6067315384875,-328.61145349355)) ;
#28570=CARTESIAN_POINT('Ctrl Pts',(9.73533267111695,16.8093403434722,-328.606484462588)) ;
#28571=CARTESIAN_POINT('Ctrl Pts',(9.38550175371263,17.011949148457,-328.601515431625)) ;
#28572=CARTESIAN_POINT('Ctrl Pts',(9.0293787717279,17.2036129892565,-328.596546400663)) ;
#28573=CARTESIAN_POINT('Ctrl Pts',(8.66767329742823,17.383959980656,-328.5915773697)) ;
#28574=CARTESIAN_POINT('Ctrl Pts',(8.30646155200444,17.5640607979618,-328.586615121478)) ;
#28575=CARTESIAN_POINT('Ctrl Pts',(7.93958653014361,17.7329235258746,-328.581652873255)) ;
#28576=CARTESIAN_POINT('Ctrl Pts',(7.56776927654216,17.8902066275665,-328.576690625032)) ;
#28577=CARTESIAN_POINT('Ctrl Pts',(7.19623367491283,18.0473705871386,-328.571732135718)) ;
#28578=CARTESIAN_POINT('Ctrl Pts',(6.81976354496309,18.1929723644495,-328.566773646404)) ;
#28579=CARTESIAN_POINT('Ctrl Pts',(6.43909946036323,18.3267188317917,-328.561815157089)) ;
#28580=CARTESIAN_POINT('Ctrl Pts',(6.05847622696971,18.4604509460475,-328.556857199898)) ;
#28581=CARTESIAN_POINT('Ctrl Pts',(5.67366016173786,18.5823302128011,-328.551899242707)) ;
#28582=CARTESIAN_POINT('Ctrl Pts',(5.28540946239075,18.6921125562327,-328.546941285516)) ;
#28583=CARTESIAN_POINT('Ctrl Pts',(4.89718235802834,18.8018882279113,-328.541983629633)) ;
#28584=CARTESIAN_POINT('Ctrl Pts',(4.50552126488381,18.8995683803713,-328.53702597375)) ;
#28585=CARTESIAN_POINT('Ctrl Pts',(4.11119872364413,18.9849590480124,-328.532068317867)) ;
#28586=CARTESIAN_POINT('Ctrl Pts',(3.71625953069999,19.0704832517698,-328.527102909074)) ;
#28587=CARTESIAN_POINT('Ctrl Pts',(3.31865078938638,19.1436794396047,-328.522137500281)) ;
#28588=CARTESIAN_POINT('Ctrl Pts',(2.91915976144519,19.2044039555296,-328.517172091488)) ;
#28589=CARTESIAN_POINT('Ctrl Pts',(2.52025157547297,19.2650398767327,-328.512213927035)) ;
#28590=CARTESIAN_POINT('Ctrl Pts',(2.11946682860372,19.3132404698375,-328.507255762582)) ;
#28591=CARTESIAN_POINT('Ctrl Pts',(1.7175968762395,19.3489143357123,-328.502297598129)) ;
#28592=CARTESIAN_POINT('Ctrl Pts',(1.31484616979748,19.3846663858421,-328.497328567166)) ;
#28593=CARTESIAN_POINT('Ctrl Pts',(0.911005732975615,19.4078367046179,-328.492359536204)) ;
#28594=CARTESIAN_POINT('Ctrl Pts',(0.506876152011263,19.4183856580953,-328.487390505242)) ;
#28595=CARTESIAN_POINT('Ctrl Pts',(0.102746571046912,19.4289346115727,-328.482421474279)) ;
#28596=CARTESIAN_POINT('Ctrl Pts',(-0.301671914286292,19.426862200149,-328.477452443317)) ;
#28597=CARTESIAN_POINT('Ctrl Pts',(-0.705578289224847,19.4121813374431,
-328.472483412354)) ;
#28598=CARTESIAN_POINT('Ctrl Pts',(-1.10893333095202,19.3975205141515,-328.467521164131)) ;
#28599=CARTESIAN_POINT('Ctrl Pts',(-1.51188488185458,19.3702817519047,-328.462558915909)) ;
#28600=CARTESIAN_POINT('Ctrl Pts',(-1.91363637230772,19.3305101028033,-328.457596667686)) ;
#28601=CARTESIAN_POINT('Ctrl Pts',(-2.31508353557163,19.2907685807692,-328.452638178372)) ;
#28602=CARTESIAN_POINT('Ctrl Pts',(-2.715332219408,19.2385131754269,-328.447679689057)) ;
#28603=CARTESIAN_POINT('Ctrl Pts',(-3.11359186534508,19.1738407914548,-328.442721199743)) ;
#28604=CARTESIAN_POINT('Ctrl Pts',(-3.51180877179723,19.1091753478404,-328.437763242552)) ;
#28605=CARTESIAN_POINT('Ctrl Pts',(-3.90803683248095,19.0320956251393,-328.432805285361)) ;
#28606=CARTESIAN_POINT('Ctrl Pts',(-4.30149348035884,18.9427500336786,-328.42784732817)) ;
#28607=CARTESIAN_POINT('Ctrl Pts',(-4.69492621687323,18.8534098719773,-328.422889672287)) ;
#28608=CARTESIAN_POINT('Ctrl Pts',(-5.08558764565361,18.7518053832431,-328.417932016403)) ;
#28609=CARTESIAN_POINT('Ctrl Pts',(-5.47270657864753,18.6381358430512,-328.41297436052)) ;
#28610=CARTESIAN_POINT('Ctrl Pts',(-5.86043089815883,18.5242885435165,-328.408008951728)) ;
#28611=CARTESIAN_POINT('Ctrl Pts',(-6.24460140074579,18.3983384818859,-328.403043542935)) ;
#28612=CARTESIAN_POINT('Ctrl Pts',(-6.62445804072266,18.2605361549628,-328.398078134142)) ;
#28613=CARTESIAN_POINT('Ctrl Pts',(-7.00376048454349,18.1229348763086,-328.393119969689)) ;
#28614=CARTESIAN_POINT('Ctrl Pts',(-7.37876142559328,17.9735159862364,-328.388161805236)) ;
#28615=CARTESIAN_POINT('Ctrl Pts',(-7.74872222438242,17.8125778283033,-328.383203640783)) ;
#28616=CARTESIAN_POINT('Ctrl Pts',(-8.11949384388696,17.6512869519395,-328.37823460982)) ;
#28617=CARTESIAN_POINT('Ctrl Pts',(-8.48520297924535,17.4784263421979,-328.373265578858)) ;
#28618=CARTESIAN_POINT('Ctrl Pts',(-8.84512765083664,17.2943442153903,-328.368296547895)) ;
#28619=CARTESIAN_POINT('Ctrl Pts',(-9.20505232242797,17.1102620885828,-328.363327516933)) ;
#28620=CARTESIAN_POINT('Ctrl Pts',(-9.55919231989017,16.9149585597718,-328.358358485971)) ;
#28621=CARTESIAN_POINT('Ctrl Pts',(-9.90685042733949,16.7088281938119,-328.353389455008)) ;
#28622=CARTESIAN_POINT('Ctrl Pts',(-10.2540339806029,16.5029791963169,-328.348427206785)) ;
#28623=CARTESIAN_POINT('Ctrl Pts',(-10.5948456236609,16.2862781891673,-328.343464958563)) ;
#28624=CARTESIAN_POINT('Ctrl Pts',(-10.9286074198686,16.0591458322787,-328.33850271034)) ;
#28625=CARTESIAN_POINT('Ctrl Pts',(-11.2621163911543,15.8321855283963,-328.333544221026)) ;
#28626=CARTESIAN_POINT('Ctrl Pts',(-11.5885859956914,15.5948098059353,-328.328585731711)) ;
#28627=CARTESIAN_POINT('Ctrl Pts',(-11.9073683829411,15.3474819821668,-328.323627242397)) ;
#28628=CARTESIAN_POINT('Ctrl Pts',(-12.2261165598585,15.1001807005392,-328.318669285206)) ;
#28629=CARTESIAN_POINT('Ctrl Pts',(-12.5371789797316,14.8429295962303,-328.313711328015)) ;
#28630=CARTESIAN_POINT('Ctrl Pts',(-12.8399394510907,14.5762333918034,-328.308753370824)) ;
#28631=CARTESIAN_POINT('Ctrl Pts',(-13.1426815229238,14.309553395185,-328.303795714941)) ;
#28632=CARTESIAN_POINT('Ctrl Pts',(-13.4371224761093,14.0334296020142,-328.298838059058)) ;
#28633=CARTESIAN_POINT('Ctrl Pts',(-13.7226804465684,13.7484059571053,-328.293880403175)) ;
#28634=CARTESIAN_POINT('Ctrl Pts',(-14.0086849799063,13.4629365849096,-328.288914994382)) ;
#28635=CARTESIAN_POINT('Ctrl Pts',(-14.2857785474108,13.1685396624901,-328.283949585589)) ;
#28636=CARTESIAN_POINT('Ctrl Pts',(-14.5534135749228,12.8657987827128,-328.278984176797)) ;
#28637=CARTESIAN_POINT('Ctrl Pts',(-14.8206581332742,12.5634995901775,-328.274026012344)) ;
#28638=CARTESIAN_POINT('Ctrl Pts',(-15.078471584423,12.252880957598,-328.26906784789)) ;
#28639=CARTESIAN_POINT('Ctrl Pts',(-15.3263480426619,11.9345582522017,-328.264109683437)) ;
#28640=CARTESIAN_POINT('Ctrl Pts',(-15.5747677567474,11.615537898178,-328.259140652475)) ;
#28641=CARTESIAN_POINT('Ctrl Pts',(-15.8132067149351,11.2887798450214,-328.254171621513)) ;
#28642=CARTESIAN_POINT('Ctrl Pts',(-16.0411975213713,10.9549352841699,-328.24920259055)) ;
#28643=CARTESIAN_POINT('Ctrl Pts',(-16.2691883278076,10.6210907233183,-328.244233559588)) ;
#28644=CARTESIAN_POINT('Ctrl Pts',(-16.4867308528162,10.2801598564539,-328.239264528625)) ;
#28645=CARTESIAN_POINT('Ctrl Pts',(-16.6934016205675,9.93282272742416,-328.234295497663)) ;
#28646=CARTESIAN_POINT('Ctrl Pts',(-16.8997902822045,9.58595971444351,-328.22933324944)) ;
#28647=CARTESIAN_POINT('Ctrl Pts',(-17.0953917198708,9.23261571757025,-328.224371001217)) ;
#28648=CARTESIAN_POINT('Ctrl Pts',(-17.2798118719054,8.87348447181585,-328.219408752995)) ;
#28649=CARTESIAN_POINT('Ctrl Pts',(-17.4640923254751,8.51462526836899,-328.21445026368)) ;
#28650=CARTESIAN_POINT('Ctrl Pts',(-17.6372083181478,8.14998779171401,-328.209491774366)) ;
#28651=CARTESIAN_POINT('Ctrl Pts',(-17.7988126160577,7.78028884158328,-328.204533285052)) ;
#28652=CARTESIAN_POINT('Ctrl Pts',(-17.9603995713005,7.41062956592835,-328.199575327861)) ;
#28653=CARTESIAN_POINT('Ctrl Pts',(-18.1104772042123,7.03591011910896,-328.19461737067)) ;
#28654=CARTESIAN_POINT('Ctrl Pts',(-18.2487458909687,6.65686851356201,-328.189659413479)) ;
#28655=CARTESIAN_POINT('Ctrl Pts',(-18.3870061747845,6.27784994333961,-328.184701757596)) ;
#28656=CARTESIAN_POINT('Ctrl Pts',(-18.5134588648321,5.89450996205973,-328.179744101712)) ;
#28657=CARTESIAN_POINT('Ctrl Pts',(-18.6278532460382,5.50760460128204,-328.174786445829)) ;
#28658=CARTESIAN_POINT('Ctrl Pts',(-18.7424265201119,5.12009418797716,-328.169821037037)) ;
#28659=CARTESIAN_POINT('Ctrl Pts',(-18.8449036609417,4.72900746014064,-328.164855628244)) ;
#28660=CARTESIAN_POINT('Ctrl Pts',(-18.9350830330146,4.33511886028998,-328.159890219451)) ;
#28661=CARTESIAN_POINT('Ctrl Pts',(-19.0251308368694,3.94180492868166,-328.154932054998)) ;
#28662=CARTESIAN_POINT('Ctrl Pts',(-19.1029166911701,3.54569752989965,-328.149973890545)) ;
#28663=CARTESIAN_POINT('Ctrl Pts',(-19.1682907698617,3.14757906366712,-328.145015726092)) ;
#28664=CARTESIAN_POINT('Ctrl Pts',(-19.2338081249689,2.74858806526303,-328.140046695129)) ;
#28665=CARTESIAN_POINT('Ctrl Pts',(-19.2868591872791,2.34757740845687,-328.135077664167)) ;
#28666=CARTESIAN_POINT('Ctrl Pts',(-19.3273450689611,1.94534253675375,-328.130108633204)) ;
#28667=CARTESIAN_POINT('Ctrl Pts',(-19.3678309506432,1.54310766505063,-328.125139602242)) ;
#28668=CARTESIAN_POINT('Ctrl Pts',(-19.3957516343142,1.1396488175936,-328.120170571279)) ;
#28669=CARTESIAN_POINT('Ctrl Pts',(-19.4110606032759,0.735765761604836,
-328.115201540317)) ;
#28670=CARTESIAN_POINT('Ctrl Pts',(-19.4263486754567,0.332434006996665,
-328.110239292094)) ;
#28671=CARTESIAN_POINT('Ctrl Pts',(-19.4290635153354,-0.0714280142283438,
-328.105277043872)) ;
#28672=CARTESIAN_POINT('Ctrl Pts',(-19.419190985827,-0.47502258470058,-328.100314795649)) ;
#28673=CARTESIAN_POINT('Ctrl Pts',(-19.4093259347704,-0.878311431849071,
-328.095356306334)) ;
#28674=CARTESIAN_POINT('Ctrl Pts',(-19.3868925827909,-1.28133299581268,
-328.09039781702)) ;
#28675=CARTESIAN_POINT('Ctrl Pts',(-19.3519289483619,-1.68329170898924,
-328.085439327706)) ;
#28676=CARTESIAN_POINT('Ctrl Pts',(-19.3169690660775,-2.08520728571259,
-328.080481370515)) ;
#28677=CARTESIAN_POINT('Ctrl Pts',(-19.2694816077016,-2.48606000308133,
-328.075523413324)) ;
#28678=CARTESIAN_POINT('Ctrl Pts',(-19.2095565481291,-2.88505844381516,
-328.070565456133)) ;
#28679=CARTESIAN_POINT('Ctrl Pts',(-19.1496351303553,-3.28403263639661,
-328.06560780025)) ;
#28680=CARTESIAN_POINT('Ctrl Pts',(-19.0772776566582,-3.68115254280761,
-328.060650144366)) ;
#28681=CARTESIAN_POINT('Ctrl Pts',(-18.9926256709009,-4.07563432180022,
-328.055692488483)) ;
#28682=CARTESIAN_POINT('Ctrl Pts',(-18.9078413041969,-4.47073300151744,
-328.05072707969)) ;
#28683=CARTESIAN_POINT('Ctrl Pts',(-18.8107239791508,-4.86318506006524,
-328.045761670898)) ;
#28684=CARTESIAN_POINT('Ctrl Pts',(-18.701467146049,-5.25221396986548,-328.040796262105)) ;
#28685=CARTESIAN_POINT('Ctrl Pts',(-18.5923697144437,-5.64067530152309,
-328.035838097652)) ;
#28686=CARTESIAN_POINT('Ctrl Pts',(-18.4711682497348,-6.02572324068312,
-328.030879933199)) ;
#28687=CARTESIAN_POINT('Ctrl Pts',(-18.3381055045038,-6.40659905922707,
-328.025921768746)) ;
#28688=CARTESIAN_POINT('Ctrl Pts',(-18.204751133699,-6.7883096202745,-328.020952737783)) ;
#28689=CARTESIAN_POINT('Ctrl Pts',(-18.0594834991421,-7.16582952231242,
-328.015983706821)) ;
#28690=CARTESIAN_POINT('Ctrl Pts',(-17.9025963241962,-7.53841295319364,
-328.011014675858)) ;
#28691=CARTESIAN_POINT('Ctrl Pts',(-17.7457091492502,-7.9109963840749,-328.006045644896)) ;
#28692=CARTESIAN_POINT('Ctrl Pts',(-17.5772025330628,-8.27864312548473,
-328.001076613934)) ;
#28693=CARTESIAN_POINT('Ctrl Pts',(-17.3974182561651,-8.64062862412527,
-327.996107582971)) ;
#28694=CARTESIAN_POINT('Ctrl Pts',(-17.2178793852547,-9.00212001165545,
-327.991145334748)) ;
#28695=CARTESIAN_POINT('Ctrl Pts',(-17.027045905362,-9.35806169999152,-327.986183086526)) ;
#28696=CARTESIAN_POINT('Ctrl Pts',(-16.8252870497874,-9.70774642706828,
-327.981220838303)) ;
#28697=CARTESIAN_POINT('Ctrl Pts',(-16.6236810267648,-10.0571662675849,
-327.976262348989)) ;
#28698=CARTESIAN_POINT('Ctrl Pts',(-16.4111662924579,-10.4003384168076,
-327.971303859674)) ;
#28699=CARTESIAN_POINT('Ctrl Pts',(-16.1881568509599,-10.7365824529372,
-327.96634537036)) ;
#28700=CARTESIAN_POINT('Ctrl Pts',(-15.9651713418614,-11.0727904048252,
-327.961387413169)) ;
#28701=CARTESIAN_POINT('Ctrl Pts',(-15.7316935062015,-11.4020715308846,
-327.956429455978)) ;
#28702=CARTESIAN_POINT('Ctrl Pts',(-15.4881809868841,-11.7237739110545,
-327.951471498787)) ;
#28703=CARTESIAN_POINT('Ctrl Pts',(-15.2446832664427,-12.0454567405514,
-327.946513842904)) ;
#28704=CARTESIAN_POINT('Ctrl Pts',(-14.9911522238549,-12.3595615550819,
-327.941556187021)) ;
#28705=CARTESIAN_POINT('Ctrl Pts',(-14.728087161658,-12.6654677591712,-327.936598531138)) ;
#28706=CARTESIAN_POINT('Ctrl Pts',(-14.4646107115677,-12.9718523472307,
-327.931633122345)) ;
#28707=CARTESIAN_POINT('Ctrl Pts',(-14.1915705447016,-13.2700124726014,
-327.926667713552)) ;
#28708=CARTESIAN_POINT('Ctrl Pts',(-13.9095080450804,-13.5593587954535,
-327.92170230476)) ;
#28709=CARTESIAN_POINT('Ctrl Pts',(-13.6278570637449,-13.8482829732034,
-327.916744140307)) ;
#28710=CARTESIAN_POINT('Ctrl Pts',(-13.3372102336003,-14.1284188877619,
-327.911785975854)) ;
#28711=CARTESIAN_POINT('Ctrl Pts',(-13.0381437167325,-14.3992164169384,
-327.9068278114)) ;
#28712=CARTESIAN_POINT('Ctrl Pts',(-12.7384217538598,-14.6706074366885,
-327.901858780438)) ;
#28713=CARTESIAN_POINT('Ctrl Pts',(-12.4302433255165,-14.9326189219133,
-327.896889749476)) ;
#28714=CARTESIAN_POINT('Ctrl Pts',(-12.1142231733798,-15.1847364779751,
-327.891920718513)) ;
#28715=CARTESIAN_POINT('Ctrl Pts',(-11.798203021243,-15.4368540340369,-327.886951687551)) ;
#28716=CARTESIAN_POINT('Ctrl Pts',(-11.4743413368243,-15.6790775166619,
-327.881982656588)) ;
#28717=CARTESIAN_POINT('Ctrl Pts',(-11.1432848914274,-15.910934190942,-327.877013625626)) ;
#28718=CARTESIAN_POINT('Ctrl Pts',(-10.8126803389072,-16.1424743802812,
-327.872051377403)) ;
#28719=CARTESIAN_POINT('Ctrl Pts',(-10.4748127774727,-16.3637376024259,
-327.86708912918)) ;
#28720=CARTESIAN_POINT('Ctrl Pts',(-10.1303448129449,-16.5742794404716,
-327.862126880958)) ;
#28721=CARTESIAN_POINT('Ctrl Pts',(-9.78613778327344,-16.7846617928469,
-327.857168391643)) ;
#28722=CARTESIAN_POINT('Ctrl Pts',(-9.43534054901703,-16.9843388740011,
-327.852209902329)) ;
#28723=CARTESIAN_POINT('Ctrl Pts',(-9.07864218947691,-17.1729112556797,
-327.847251413015)) ;
#28724=CARTESIAN_POINT('Ctrl Pts',(-8.72198210924533,-17.3614634005946,
-327.842293455824)) ;
#28725=CARTESIAN_POINT('Ctrl Pts',(-8.35942237837064,-17.5389131153692,
-327.837335498633)) ;
#28726=CARTESIAN_POINT('Ctrl Pts',(-7.99167676071931,-17.7049068778172,
-327.832377541442)) ;
#28727=CARTESIAN_POINT('Ctrl Pts',(-7.62395349190861,-17.8708905524002,
-327.827419885559)) ;
#28728=CARTESIAN_POINT('Ctrl Pts',(-7.25104518221184,-18.0254195678817,
-327.822462229676)) ;
#28729=CARTESIAN_POINT('Ctrl Pts',(-6.87368719156906,-18.1681878400808,
-327.817504573792)) ;
#28730=CARTESIAN_POINT('Ctrl Pts',(-6.49573907881945,-18.3111793769667,
-327.812539165)) ;
#28731=CARTESIAN_POINT('Ctrl Pts',(-6.11332757553556,-18.442373261119,-327.807573756207)) ;
#28732=CARTESIAN_POINT('Ctrl Pts',(-5.72721004115265,-18.5615109876465,
-327.802608347414)) ;
#28733=CARTESIAN_POINT('Ctrl Pts',(-5.34165583732873,-18.6804748968357,
-327.797650182961)) ;
#28734=CARTESIAN_POINT('Ctrl Pts',(-4.95240664008152,-18.7874177457839,
-327.792692018508)) ;
#28735=CARTESIAN_POINT('Ctrl Pts',(-4.5602315857874,-18.8821321064118,-327.787733854055)) ;
#28736=CARTESIAN_POINT('Ctrl Pts',(-4.16719702513717,-18.9770540467776,
-327.782764823093)) ;
#28737=CARTESIAN_POINT('Ctrl Pts',(-3.77122399772105,-19.0596937687268,
-327.77779579213)) ;
#28738=CARTESIAN_POINT('Ctrl Pts',(-3.37309842482874,-19.1298936749899,
-327.772826761168)) ;
#28739=CARTESIAN_POINT('Ctrl Pts',(-2.97497285193639,-19.200093581253,-327.767857730205)) ;
#28740=CARTESIAN_POINT('Ctrl Pts',(-2.57469497076363,-19.2578536367626,
-327.762888699243)) ;
#28741=CARTESIAN_POINT('Ctrl Pts',(-2.17305889770295,-19.3030681506105,
-327.757919668281)) ;
#28742=CARTESIAN_POINT('Ctrl Pts',(-1.74947978310094,-19.3507529205489,
-327.752679158584)) ;
#28743=CARTESIAN_POINT('Ctrl Pts',(-1.32431853671982,-19.3844924495454,
-327.747438648887)) ;
#28744=CARTESIAN_POINT('Ctrl Pts',(-0.898462567284284,-19.4042106259232,
-327.74219813919)) ;
#28745=CARTESIAN_POINT('Ctrl Pts',(-0.599382236252206,-19.4180587791526,
-327.738517708511)) ;
#28746=CARTESIAN_POINT('Ctrl Pts',(-0.299959377809275,-19.4249922467247,
-327.734837277831)) ;
#28747=CARTESIAN_POINT('Ctrl Pts',(-0.000502513484877063,-19.4249999935001,
-327.731156847152)) ;
#28748=CARTESIAN_POINT('Ctrl Pts',(-0.000462715166386019,-19.4249999944889,
-327.51849135163)) ;
#28749=CARTESIAN_POINT('Ctrl Pts',(-0.0875504618603551,-19.4249979200065,
-327.51951026367)) ;
#28750=CARTESIAN_POINT('Ctrl Pts',(-0.174637192315756,-19.4244101871887,
-327.52053032404)) ;
#28751=CARTESIAN_POINT('Ctrl Pts',(-0.583156222337328,-19.4189056271317,
-327.525325080606)) ;
#28752=CARTESIAN_POINT('Ctrl Pts',(-0.904437827676747,-19.4065957419375,
-327.529123355872)) ;
#28753=CARTESIAN_POINT('Ctrl Pts',(-1.32409120042041,-19.3800725791597,
-327.534188979659)) ;
#28754=CARTESIAN_POINT('Ctrl Pts',(-1.42286835371274,-19.3730709050083,
-327.535388970211)) ;
#28755=CARTESIAN_POINT('Ctrl Pts',(-1.58793135333655,-19.3601014380791,
-327.537409909657)) ;
#28756=CARTESIAN_POINT('Ctrl Pts',(-1.6542478829034,-19.3545477246516,-327.538226148633)) ;
#28757=CARTESIAN_POINT('Ctrl Pts',(-1.79913386337507,-19.3416640706631,
-327.540019594531)) ;
#28758=CARTESIAN_POINT('Ctrl Pts',(-1.87768966295884,-19.3341959540435,
-327.540998312023)) ;
#28759=CARTESIAN_POINT('Ctrl Pts',(-2.12211761287909,-19.3094550235214,
-327.544060979465)) ;
#28760=CARTESIAN_POINT('Ctrl Pts',(-2.28781417049907,-19.2905246853991,
-327.546162031428)) ;
#28761=CARTESIAN_POINT('Ctrl Pts',(-2.58521889389346,-19.252661306604,-327.549966124065)) ;
#28762=CARTESIAN_POINT('Ctrl Pts',(-2.71701549882846,-19.2345041746206,
-327.551663631084)) ;
#28763=CARTESIAN_POINT('Ctrl Pts',(-3.42733183246168,-19.1292000703169,
-327.56085938714)) ;
#28764=CARTESIAN_POINT('Ctrl Pts',(-4.0018774113232,-19.0173046861576,-327.568456382094)) ;
#28765=CARTESIAN_POINT('Ctrl Pts',(-4.62835111285505,-18.8656442881826,
-327.57671843398)) ;
#28766=CARTESIAN_POINT('Ctrl Pts',(-4.68614198174414,-18.8513724105741,
-327.577480494774)) ;
#28767=CARTESIAN_POINT('Ctrl Pts',(-5.07470334456549,-18.7535171625303,
-327.582602852089)) ;
#28768=CARTESIAN_POINT('Ctrl Pts',(-5.40328839243028,-18.6614976730265,
-327.586926368301)) ;
#28769=CARTESIAN_POINT('Ctrl Pts',(-5.87956901118637,-18.5144816882297,
-327.593163028833)) ;
#28770=CARTESIAN_POINT('Ctrl Pts',(-6.02928939306963,-18.4662674476857,
-327.595119327925)) ;
#28771=CARTESIAN_POINT('Ctrl Pts',(-6.2961097124211,-18.3767527186552,-327.598597946213)) ;
#28772=CARTESIAN_POINT('Ctrl Pts',(-6.41343041863843,-18.3361377695898,
-327.600124796865)) ;
#28773=CARTESIAN_POINT('Ctrl Pts',(-6.66687158684052,-18.2456696257398,
-327.603417875488)) ;
#28774=CARTESIAN_POINT('Ctrl Pts',(-6.80283974071304,-18.1954117398044,
-327.605181223814)) ;
#28775=CARTESIAN_POINT('Ctrl Pts',(-7.20459842630199,-18.041776869807,-327.610384246399)) ;
#28776=CARTESIAN_POINT('Ctrl Pts',(-7.46868901250923,-17.9340635660464,
-327.613794328311)) ;
#28777=CARTESIAN_POINT('Ctrl Pts',(-8.11569024270686,-17.653403611891,-327.622154760609)) ;
#28778=CARTESIAN_POINT('Ctrl Pts',(-8.49554402994306,-17.4737751879205,
-327.627066974282)) ;
#28779=CARTESIAN_POINT('Ctrl Pts',(-9.34594352841898,-17.0373419898732,
-327.638231163116)) ;
#28780=CARTESIAN_POINT('Ctrl Pts',(-9.8122858686368,-16.7730952776925,-327.644472418995)) ;
#28781=CARTESIAN_POINT('Ctrl Pts',(-10.365208327018,-16.4288294310756,-327.652289173024)) ;
#28782=CARTESIAN_POINT('Ctrl Pts',(-10.4627640056774,-16.3668735390041,
-327.653684986233)) ;
#28783=CARTESIAN_POINT('Ctrl Pts',(-10.6122358801313,-16.2700640243478,
-327.655853571851)) ;
#28784=CARTESIAN_POINT('Ctrl Pts',(-10.6645464568458,-16.2358240502541,
-327.656618236636)) ;
#28785=CARTESIAN_POINT('Ctrl Pts',(-10.7753323086322,-16.1625425629803,
-327.658250832286)) ;
#28786=CARTESIAN_POINT('Ctrl Pts',(-10.8337627389026,-16.1234349118448,
-327.65911977435)) ;
#28787=CARTESIAN_POINT('Ctrl Pts',(-10.9918688591171,-16.0163665552893,
-327.66149105469)) ;
#28788=CARTESIAN_POINT('Ctrl Pts',(-11.0911258067423,-15.9477931678159,
-327.663001483979)) ;
#28789=CARTESIAN_POINT('Ctrl Pts',(-11.9249176232268,-15.3602043433064,
-327.675853058101)) ;
#28790=CARTESIAN_POINT('Ctrl Pts',(-12.6232290523684,-14.7916745942156,
-327.687641646055)) ;
#28791=CARTESIAN_POINT('Ctrl Pts',(-13.5081919684354,-13.9627164337976,
-327.703106522724)) ;
#28792=CARTESIAN_POINT('Ctrl Pts',(-13.7315400811651,-13.7431258503417,
-327.70706605129)) ;
#28793=CARTESIAN_POINT('Ctrl Pts',(-14.0545557157477,-13.4098055655803,
-327.712865575638)) ;
#28794=CARTESIAN_POINT('Ctrl Pts',(-14.1583619135899,-13.3001582577333,
-327.71474125546)) ;
#28795=CARTESIAN_POINT('Ctrl Pts',(-14.3450195712004,-13.098335572006,-327.718135884983)) ;
#28796=CARTESIAN_POINT('Ctrl Pts',(-14.4282873802844,-13.0065562149735,
-327.719658442122)) ;
#28797=CARTESIAN_POINT('Ctrl Pts',(-14.6105714554529,-12.8017345403403,
-327.723010527185)) ;
#28798=CARTESIAN_POINT('Ctrl Pts',(-14.7091657556736,-12.6883272478202,
-327.72483636482)) ;
#28799=CARTESIAN_POINT('Ctrl Pts',(-15.0140380604009,-12.3293207168525,
-327.730526010657)) ;
#28800=CARTESIAN_POINT('Ctrl Pts',(-15.215555652452,-12.0797497909713,-327.734350565174)) ;
#28801=CARTESIAN_POINT('Ctrl Pts',(-15.7283613059349,-11.4114586055765,
-327.744305891026)) ;
#28802=CARTESIAN_POINT('Ctrl Pts',(-16.0291217978085,-10.9849893599266,
-327.750372355706)) ;
#28803=CARTESIAN_POINT('Ctrl Pts',(-16.3415791284692,-10.5017291097709,
-327.757104294624)) ;
#28804=CARTESIAN_POINT('Ctrl Pts',(-16.37061864433,-10.4564032012761,-327.75773442795)) ;
#28805=CARTESIAN_POINT('Ctrl Pts',(-16.5913556505341,-10.1086955206593,
-327.76256029579)) ;
#28806=CARTESIAN_POINT('Ctrl Pts',(-16.7748483169206,-9.80118718528197,
-327.76678046217)) ;
#28807=CARTESIAN_POINT('Ctrl Pts',(-16.9986916894915,-9.4013376396414,-327.772299194441)) ;
#28808=CARTESIAN_POINT('Ctrl Pts',(-17.0469687853949,-9.31351296554688,
-327.773513332704)) ;
#28809=CARTESIAN_POINT('Ctrl Pts',(-17.1262458260637,-9.16661219314292,
-327.775550420558)) ;
#28810=CARTESIAN_POINT('Ctrl Pts',(-17.1576249752709,-9.10774288237239,
-327.776368475831)) ;
#28811=CARTESIAN_POINT('Ctrl Pts',(-17.2251759874745,-8.97942473321593,
-327.778156115374)) ;
#28812=CARTESIAN_POINT('Ctrl Pts',(-17.2612323543557,-8.90991660608215,
-327.779127106549)) ;
#28813=CARTESIAN_POINT('Ctrl Pts',(-17.3711421197179,-8.69486533267194,
-327.782137139557)) ;
#28814=CARTESIAN_POINT('Ctrl Pts',(-17.4435822327408,-8.5486080997419,-327.784192491514)) ;
#28815=CARTESIAN_POINT('Ctrl Pts',(-17.5698800013233,-8.28532031359845,
-327.78789601854)) ;
#28816=CARTESIAN_POINT('Ctrl Pts',(-17.6244329586573,-8.16863383910826,
-327.789538623193)) ;
#28817=CARTESIAN_POINT('Ctrl Pts',(-17.9044144906519,-7.55390159856788,
-327.798184370866)) ;
#28818=CARTESIAN_POINT('Ctrl Pts',(-18.1099043209476,-7.04704576123368,
-327.805278442457)) ;
#28819=CARTESIAN_POINT('Ctrl Pts',(-18.4299567344089,-6.15072336292275,
-327.817500569215)) ;
#28820=CARTESIAN_POINT('Ctrl Pts',(-18.5542060066141,-5.76507969884636,
-327.822660738808)) ;
#28821=CARTESIAN_POINT('Ctrl Pts',(-18.7145393192184,-5.2083602612631,-327.829932752344)) ;
#28822=CARTESIAN_POINT('Ctrl Pts',(-18.7605150291436,-5.04024548104869,
-327.832106367436)) ;
#28823=CARTESIAN_POINT('Ctrl Pts',(-18.8358229250807,-4.74955547962341,
-327.835825844672)) ;
#28824=CARTESIAN_POINT('Ctrl Pts',(-18.8662359727767,-4.62727163535486,
-327.837378753196)) ;
#28825=CARTESIAN_POINT('Ctrl Pts',(-18.9270179645635,-4.37231494533072,
-327.840592562787)) ;
#28826=CARTESIAN_POINT('Ctrl Pts',(-18.9571867050428,-4.23960131407512,
-327.842252060928)) ;
#28827=CARTESIAN_POINT('Ctrl Pts',(-19.0351914873101,-3.87896180438932,
-327.846727166939)) ;
#28828=CARTESIAN_POINT('Ctrl Pts',(-19.0803273789256,-3.6504749029966,-327.849525102332)) ;
#28829=CARTESIAN_POINT('Ctrl Pts',(-19.1499347249954,-3.26143779399589,
-327.854236118045)) ;
#28830=CARTESIAN_POINT('Ctrl Pts',(-19.1765211977967,-3.10129187239817,
-327.856160358225)) ;
#28831=CARTESIAN_POINT('Ctrl Pts',(-19.2889847794236,-2.36700151958446,
-327.864928287907)) ;
#28832=CARTESIAN_POINT('Ctrl Pts',(-19.3511044448623,-1.7895211434636,-327.871661108941)) ;
#28833=CARTESIAN_POINT('Ctrl Pts',(-19.4079322895241,-0.879091330808883,
-327.882361781228)) ;
#28834=CARTESIAN_POINT('Ctrl Pts',(-19.4201130868161,-0.547580203657073,
-327.886278288567)) ;
#28835=CARTESIAN_POINT('Ctrl Pts',(-19.4249011936842,-0.116852268629662,
-327.891467491982)) ;
#28836=CARTESIAN_POINT('Ctrl Pts',(-19.4252445233405,-0.0177765970544005,
-327.892668090084)) ;
#28837=CARTESIAN_POINT('Ctrl Pts',(-19.4245513318986,0.147851710666956,
-327.894689720622)) ;
#28838=CARTESIAN_POINT('Ctrl Pts',(-19.4239307403101,0.214404239399394,
-327.895506035233)) ;
#28839=CARTESIAN_POINT('Ctrl Pts',(-19.4218272108245,0.35982669676706,-327.89729922046)) ;
#28840=CARTESIAN_POINT('Ctrl Pts',(-19.4202058603158,0.438693265072396,
-327.8982775971)) ;
#28841=CARTESIAN_POINT('Ctrl Pts',(-19.4136651284702,0.684097918810671,
-327.901337926387)) ;
#28842=CARTESIAN_POINT('Ctrl Pts',(-19.4070835133104,0.850583940071773,
-327.903436945489)) ;
#28843=CARTESIAN_POINT('Ctrl Pts',(-19.3914059212147,1.14963039464501,-327.90723654428)) ;
#28844=CARTESIAN_POINT('Ctrl Pts',(-19.3830900955522,1.2822214869906,-327.908931588346)) ;
#28845=CARTESIAN_POINT('Ctrl Pts',(-19.3309370403932,1.99641590309156,-327.918101731131)) ;
#28846=CARTESIAN_POINT('Ctrl Pts',(-19.2622820041996,2.57590698486401,-327.925675215487)) ;
#28847=CARTESIAN_POINT('Ctrl Pts',(-19.1652868113706,3.1658521879522,-327.933339322707)) ;
#28848=CARTESIAN_POINT('Ctrl Pts',(-19.1628992368409,3.18027223312467,-327.933526634876)) ;
#28849=CARTESIAN_POINT('Ctrl Pts',(-19.098528555165,3.5663423417311,-327.938540941272)) ;
#28850=CARTESIAN_POINT('Ctrl Pts',(-19.0257614235174,3.93611408048295,-327.943325971691)) ;
#28851=CARTESIAN_POINT('Ctrl Pts',(-18.9068865748296,4.45934928392815,-327.950045265111)) ;
#28852=CARTESIAN_POINT('Ctrl Pts',(-18.8695657925242,4.61472023953373,-327.952034233729)) ;
#28853=CARTESIAN_POINT('Ctrl Pts',(-18.7997437351827,4.89037625064205,-327.955551545897)) ;
#28854=CARTESIAN_POINT('Ctrl Pts',(-18.7679941210356,5.01084235446707,-327.957084751049)) ;
#28855=CARTESIAN_POINT('Ctrl Pts',(-18.6976984268474,5.26751694916318,-327.960343658998)) ;
#28856=CARTESIAN_POINT('Ctrl Pts',(-18.6588178232343,5.40362644688988,-327.962067022582)) ;
#28857=CARTESIAN_POINT('Ctrl Pts',(-18.5430858897196,5.79261963843345,-327.966980871184)) ;
#28858=CARTESIAN_POINT('Ctrl Pts',(-18.4625565609238,6.0443760799163,-327.97014684446)) ;
#28859=CARTESIAN_POINT('Ctrl Pts',(-18.2569675181771,6.64460576565063,-327.977683463269)) ;
#28860=CARTESIAN_POINT('Ctrl Pts',(-18.1270341365808,6.99130049699873,-327.982026272134)) ;
#28861=CARTESIAN_POINT('Ctrl Pts',(-17.7477311490485,7.92156516897305,-327.993770961313)) ;
#28862=CARTESIAN_POINT('Ctrl Pts',(-17.4795500406759,8.49696888257827,-328.001127490372)) ;
#28863=CARTESIAN_POINT('Ctrl Pts',(-17.1336482373289,9.15315474311764,-328.01004562201)) ;
#28864=CARTESIAN_POINT('Ctrl Pts',(-17.0828147637338,9.24767989134375,-328.011343940473)) ;
#28865=CARTESIAN_POINT('Ctrl Pts',(-16.9989057045247,9.40065632672372,-328.013470902948)) ;
#28866=CARTESIAN_POINT('Ctrl Pts',(-16.9663057094028,9.45936599930026,-328.014293460279)) ;
#28867=CARTESIAN_POINT('Ctrl Pts',(-16.8966524543524,9.58328680956738,-328.016043998878)) ;
#28868=CARTESIAN_POINT('Ctrl Pts',(-16.859524680645,9.64845468258854,-328.016972904328)) ;
#28869=CARTESIAN_POINT('Ctrl Pts',(-16.7496263004419,9.83878059205885,-328.019708390291)) ;
#28870=CARTESIAN_POINT('Ctrl Pts',(-16.6758328624322,9.9633419585146,-328.021527439188)) ;
#28871=CARTESIAN_POINT('Ctrl Pts',(-16.5445552142952,10.1793903807148,-328.024725469698)) ;
#28872=CARTESIAN_POINT('Ctrl Pts',(-16.4876872576234,10.2712445509051,-328.026098922453)) ;
#28873=CARTESIAN_POINT('Ctrl Pts',(-16.2192340189682,10.6968803446237,-328.032520083794)) ;
#28874=CARTESIAN_POINT('Ctrl Pts',(-15.9982606271777,11.0246296024608,-328.037626670119)) ;
#28875=CARTESIAN_POINT('Ctrl Pts',(-15.6316426828024,11.5341421044106,-328.045723772713)) ;
#28876=CARTESIAN_POINT('Ctrl Pts',(-15.4924631778218,11.720421146313,-328.048719860984)) ;
#28877=CARTESIAN_POINT('Ctrl Pts',(-15.1672884594444,12.1397220107385,-328.055525761193)) ;
#28878=CARTESIAN_POINT('Ctrl Pts',(-14.9792051310224,12.3710510408541,-328.05932550012)) ;
#28879=CARTESIAN_POINT('Ctrl Pts',(-14.6498080327277,12.7576551792302,-328.065734463548)) ;
#28880=CARTESIAN_POINT('Ctrl Pts',(-14.5111651439612,12.9151355954244,-328.068362699002)) ;
#28881=CARTESIAN_POINT('Ctrl Pts',(-14.2812164998254,13.1679493546265,-328.072609034282)) ;
#28882=CARTESIAN_POINT('Ctrl Pts',(-14.1914423413766,13.264652247545,-328.07423999536)) ;
#28883=CARTESIAN_POINT('Ctrl Pts',(-14.0125298009809,13.4534777319322,-328.077438316816)) ;
#28884=CARTESIAN_POINT('Ctrl Pts',(-13.9234509162741,13.5456476087286,-328.079006086041)) ;
#28885=CARTESIAN_POINT('Ctrl Pts',(-13.7013245503481,13.7709752873562,-328.082856378434)) ;
#28886=CARTESIAN_POINT('Ctrl Pts',(-13.5672413571309,13.9030937889803,-328.085129388247)) ;
#28887=CARTESIAN_POINT('Ctrl Pts',(-13.0595226335151,14.3890329128252,-328.09355805165)) ;
#28888=CARTESIAN_POINT('Ctrl Pts',(-12.6737954045668,14.7299121166464,-328.099603966987)) ;
#28889=CARTESIAN_POINT('Ctrl Pts',(-11.7867392338451,15.4531636738416,-328.112983197014)) ;
#28890=CARTESIAN_POINT('Ctrl Pts',(-11.2794137507289,15.8272647355028,-328.120289609384)) ;
#28891=CARTESIAN_POINT('Ctrl Pts',(-10.6656083675607,16.2353594966201,-328.129151822134)) ;
#28892=CARTESIAN_POINT('Ctrl Pts',(-10.5759153109872,16.2939287810693,-328.130447720425)) ;
#28893=CARTESIAN_POINT('Ctrl Pts',(-10.4292427979209,16.3879841520384,-328.132571832571)) ;
#28894=CARTESIAN_POINT('Ctrl Pts',(-10.3725556956901,16.4239221337203,-328.133393992149)) ;
#28895=CARTESIAN_POINT('Ctrl Pts',(-10.2520694051062,16.4994343591286,-328.135145056372)) ;
#28896=CARTESIAN_POINT('Ctrl Pts',(-10.1882248457873,16.5389339357645,-328.136074898614)) ;
#28897=CARTESIAN_POINT('Ctrl Pts',(-10.0002597944637,16.6537234020935,-328.138816294909)) ;
#28898=CARTESIAN_POINT('Ctrl Pts',(-9.87552249824322,16.7279931369871,-328.140640395017)) ;
#28899=CARTESIAN_POINT('Ctrl Pts',(-9.57340816236359,16.9033177640869,-328.145059377197)) ;
#28900=CARTESIAN_POINT('Ctrl Pts',(-9.39524773944961,17.0029884141334,-328.147666048256)) ;
#28901=CARTESIAN_POINT('Ctrl Pts',(-8.52006113134286,17.4746495162777,-328.160421872988)) ;
#28902=CARTESIAN_POINT('Ctrl Pts',(-7.80234867035075,17.8066892439386,-328.170699647395)) ;
#28903=CARTESIAN_POINT('Ctrl Pts',(-6.85126365716647,18.1781231647068,-328.183617118768)) ;
#28904=CARTESIAN_POINT('Ctrl Pts',(-6.63462999414935,18.2583038811386,-328.186516920105)) ;
#28905=CARTESIAN_POINT('Ctrl Pts',(-6.28848315555995,18.3794459665695,-328.1910801135)) ;
#28906=CARTESIAN_POINT('Ctrl Pts',(-6.15988186663016,18.422945201186,-328.192760319243)) ;
#28907=CARTESIAN_POINT('Ctrl Pts',(-5.91092959732751,18.5042548426715,-328.195984095111)) ;
#28908=CARTESIAN_POINT('Ctrl Pts',(-5.79064542670328,18.5422480184539,-328.197528840129)) ;
#28909=CARTESIAN_POINT('Ctrl Pts',(-5.50241931714543,18.6302094831768,-328.201200700974)) ;
#28910=CARTESIAN_POINT('Ctrl Pts',(-5.33415456343649,18.6790823903147,-328.203320377013)) ;
#28911=CARTESIAN_POINT('Ctrl Pts',(-4.58304801967351,18.8862660988725,-328.212685189116)) ;
#28912=CARTESIAN_POINT('Ctrl Pts',(-3.99367099082209,19.019620657785,-328.219763796531)) ;
#28913=CARTESIAN_POINT('Ctrl Pts',(-2.85075675345324,19.2227449147989,-328.233323400113)) ;
#28914=CARTESIAN_POINT('Ctrl Pts',(-2.29853727687148,19.2965659824724,-328.239804063995)) ;
#28915=CARTESIAN_POINT('Ctrl Pts',(-1.63054495472792,19.3567793016164,-328.247856128942)) ;
#28916=CARTESIAN_POINT('Ctrl Pts',(-1.51708922322488,19.3660017043853,-328.249231402219)) ;
#28917=CARTESIAN_POINT('Ctrl Pts',(-1.34150149314783,19.3787220968429,-328.251375654006)) ;
#28918=CARTESIAN_POINT('Ctrl Pts',(-1.27942264897695,19.3829196468775,-328.25213681154)) ;
#28919=CARTESIAN_POINT('Ctrl Pts',(-1.14674808015745,19.3912504637301,-328.253771028205)) ;
#28920=CARTESIAN_POINT('Ctrl Pts',(-1.07614779048985,19.3952966365952,-328.254645172534)) ;
#28921=CARTESIAN_POINT('Ctrl Pts',(-0.883008938816952,19.405307810807,-328.257047413063)) ;
#28922=CARTESIAN_POINT('Ctrl Pts',(-0.760433538934665,19.4104975923624,
-328.258583943438)) ;
#28923=CARTESIAN_POINT('Ctrl Pts',(-0.4770327765349,19.419808040223,-328.262157836714)) ;
#28924=CARTESIAN_POINT('Ctrl Pts',(-0.316188912043937,19.4230926747799,
-328.264202054021)) ;
#28925=CARTESIAN_POINT('Ctrl Pts',(0.280529308760709,19.4278642091606,-328.271824201158)) ;
#28926=CARTESIAN_POINT('Ctrl Pts',(0.716375330055747,19.4166786717865,-328.277464415724)) ;
#28927=CARTESIAN_POINT('Ctrl Pts',(1.64383212011842,19.3616040490396,-328.289441166289)) ;
#28928=CARTESIAN_POINT('Ctrl Pts',(2.13489813713932,19.3136249209026,-328.29576586133)) ;
#28929=CARTESIAN_POINT('Ctrl Pts',(2.82210247795921,19.219950462699,-328.304506387869)) ;
#28930=CARTESIAN_POINT('Ctrl Pts',(3.02016925046345,19.1898237634445,-328.30701335451)) ;
#28931=CARTESIAN_POINT('Ctrl Pts',(3.333389318249,19.1372122844123,-328.310956903586)) ;
#28932=CARTESIAN_POINT('Ctrl Pts',(3.44886565933088,19.1167388450256,-328.312406289383)) ;
#28933=CARTESIAN_POINT('Ctrl Pts',(3.68929967144744,19.0718615017091,-328.315414889356)) ;
#28934=CARTESIAN_POINT('Ctrl Pts',(3.81421716603853,19.0472722631414,-328.316972810427)) ;
#28935=CARTESIAN_POINT('Ctrl Pts',(4.11800216615945,18.984365731484,-328.32074986184)) ;
#28936=CARTESIAN_POINT('Ctrl Pts',(4.29658764890146,18.9447464691426,-328.32296033885)) ;
#28937=CARTESIAN_POINT('Ctrl Pts',(4.58592423128139,18.8762553098497,-328.326529341337)) ;
#28938=CARTESIAN_POINT('Ctrl Pts',(4.69702643109369,18.8489166350012,-328.327896851862)) ;
#28939=CARTESIAN_POINT('Ctrl Pts',(5.1207545749154,18.7406717029069,-328.333104256076)) ;
#28940=CARTESIAN_POINT('Ctrl Pts',(5.43158704647897,18.6529559552165,-328.336906449447)) ;
#28941=CARTESIAN_POINT('Ctrl Pts',(6.14384608956865,18.432644884267,-328.345640440425)) ;
#28942=CARTESIAN_POINT('Ctrl Pts',(6.54342013044681,18.2946138186444,-328.350555108372)) ;
#28943=CARTESIAN_POINT('Ctrl Pts',(7.23126063713109,18.0315821955327,-328.359201022238)) ;
#28944=CARTESIAN_POINT('Ctrl Pts',(7.52158930831235,17.9124197234087,-328.362910550602)) ;
#28945=CARTESIAN_POINT('Ctrl Pts',(7.89913067769083,17.7466636248394,-328.36787842997)) ;
#28946=CARTESIAN_POINT('Ctrl Pts',(7.98905554481765,17.7063640180782,-328.369072698009)) ;
#28947=CARTESIAN_POINT('Ctrl Pts',(8.13913274411021,17.6377312460158,-328.371087138981)) ;
#28948=CARTESIAN_POINT('Ctrl Pts',(8.19945329742817,17.6097703268403,-328.371902676444)) ;
#28949=CARTESIAN_POINT('Ctrl Pts',(8.3312808262468,17.5478389503597,-328.373698629495)) ;
#28950=CARTESIAN_POINT('Ctrl Pts',(8.40272592842685,17.5137400056105,-328.374680598938)) ;
#28951=CARTESIAN_POINT('Ctrl Pts',(8.62538791531918,17.4057929420576,-328.377765650427)) ;
#28952=CARTESIAN_POINT('Ctrl Pts',(8.77585474530485,17.3304159778611,-328.379886176734)) ;
#28953=CARTESIAN_POINT('Ctrl Pts',(9.39414740862465,17.0105625191951,-328.388720696626)) ;
#28954=CARTESIAN_POINT('Ctrl Pts',(9.85289134556037,16.7490230926985,-328.395558970818)) ;
#28955=CARTESIAN_POINT('Ctrl Pts',(10.76960464394,16.1756760325585,-328.409496001678)) ;
#28956=CARTESIAN_POINT('Ctrl Pts',(11.2260433501576,15.8623085791451,-328.416583652633)) ;
#28957=CARTESIAN_POINT('Ctrl Pts',(11.791563928678,15.4374009301672,-328.425457193509)) ;
#28958=CARTESIAN_POINT('Ctrl Pts',(11.9135446029793,15.3434605758474,-328.427377568888)) ;
#28959=CARTESIAN_POINT('Ctrl Pts',(12.133428209973,15.1699196223859,-328.430850526408)) ;
#28960=CARTESIAN_POINT('Ctrl Pts',(12.2316969456628,15.0907962465439,-328.432406844608)) ;
#28961=CARTESIAN_POINT('Ctrl Pts',(12.4318045921049,14.9264360691077,-328.435585120368)) ;
#28962=CARTESIAN_POINT('Ctrl Pts',(12.5335542943512,14.8411009008113,-328.437206140261)) ;
#28963=CARTESIAN_POINT('Ctrl Pts',(12.7973574017057,14.6152072555017,-328.441423451381)) ;
#28964=CARTESIAN_POINT('Ctrl Pts',(12.9579716186118,14.4729959349308,-328.444005639473)) ;
#28965=CARTESIAN_POINT('Ctrl Pts',(13.2223035620439,14.2310226751055,-328.448287237365)) ;
#28966=CARTESIAN_POINT('Ctrl Pts',(13.3273273051481,14.1327161162044,-328.44999717113)) ;
#28967=CARTESIAN_POINT('Ctrl Pts',(13.7658223450253,13.7130317652644,-328.457182081507)) ;
#28968=CARTESIAN_POINT('Ctrl Pts',(14.0888366531669,13.3809486644664,-328.462584199108)) ;
#28969=CARTESIAN_POINT('Ctrl Pts',(14.523415987501,12.9009691178902,-328.470147717985)) ;
#28970=CARTESIAN_POINT('Ctrl Pts',(14.6452069443666,12.7625440109993,-328.472302774086)) ;
#28971=CARTESIAN_POINT('Ctrl Pts',(14.9711996524403,12.3812153556524,-328.478191645861)) ;
#28972=CARTESIAN_POINT('Ctrl Pts',(15.1714492825501,12.1350087990501,-328.481941903477)) ;
#28973=CARTESIAN_POINT('Ctrl Pts',(15.4260241849358,11.8058529949963,-328.486955100602)) ;
#28974=CARTESIAN_POINT('Ctrl Pts',(15.4858737690684,11.7272375546989,-328.488152480239)) ;
#28975=CARTESIAN_POINT('Ctrl Pts',(15.5850091957751,11.5949358864183,-328.490170452266)) ;
#28976=CARTESIAN_POINT('Ctrl Pts',(15.6246237566944,11.5414982698249,-328.490986368716)) ;
#28977=CARTESIAN_POINT('Ctrl Pts',(15.7106981854784,11.4241337739055,-328.492780946795)) ;
#28978=CARTESIAN_POINT('Ctrl Pts',(15.757043910693,11.3601248732004,-328.493761138643)) ;
#28979=CARTESIAN_POINT('Ctrl Pts',(15.900373890429,11.1596046514029,-328.496833937232)) ;
#28980=CARTESIAN_POINT('Ctrl Pts',(15.9959843169556,11.0221210032187,-328.498943800484)) ;
#28981=CARTESIAN_POINT('Ctrl Pts',(16.164805327881,10.7725397598502,-328.502767393576)) ;
#28982=CARTESIAN_POINT('Ctrl Pts',(16.2386574684142,10.6608886935786,-328.504475598661)) ;
#28983=CARTESIAN_POINT('Ctrl Pts',(16.6333256709286,10.0506046527205,-328.513783709302)) ;
#28984=CARTESIAN_POINT('Ctrl Pts',(16.9323376134122,9.53824519432217,-328.521483935989)) ;
#28985=CARTESIAN_POINT('Ctrl Pts',(17.3837203324637,8.67647524791353,-328.533948471815)) ;
#28986=CARTESIAN_POINT('Ctrl Pts',(17.5500836194091,8.33483781685596,-328.538773630745)) ;
#28987=CARTESIAN_POINT('Ctrl Pts',(17.7719648702282,7.84304581583767,-328.545529756818)) ;
#28988=CARTESIAN_POINT('Ctrl Pts',(17.8358122197019,7.69674642814802,-328.547516604124)) ;
#28989=CARTESIAN_POINT('Ctrl Pts',(17.9462605208759,7.43490911529878,-328.551031579928)) ;
#28990=CARTESIAN_POINT('Ctrl Pts',(17.9935668112125,7.31967852391603,-328.552564546232)) ;
#28991=CARTESIAN_POINT('Ctrl Pts',(18.0922940469317,7.07245259582448,-328.55582440529)) ;
#28992=CARTESIAN_POINT('Ctrl Pts',(18.1433861041146,6.94033359033269,-328.557548942601)) ;
#28993=CARTESIAN_POINT('Ctrl Pts',(18.2858621492871,6.55957604548678,-328.562471087437)) ;
#28994=CARTESIAN_POINT('Ctrl Pts',(18.3736114261812,6.30961139634169,-328.565644044003)) ;
#28995=CARTESIAN_POINT('Ctrl Pts',(18.5178237990721,5.87025085931974,-328.571136712812)) ;
#28996=CARTESIAN_POINT('Ctrl Pts',(18.5765599670062,5.68164265930143,-328.57346801455)) ;
#28997=CARTESIAN_POINT('Ctrl Pts',(18.7390434990264,5.13041083008669,-328.580222060576)) ;
#28998=CARTESIAN_POINT('Ctrl Pts',(18.835119323012,4.76562133162026,-328.584616196779)) ;
#28999=CARTESIAN_POINT('Ctrl Pts',(18.9457287663866,4.28980037581498,-328.590326853063)) ;
#29000=CARTESIAN_POINT('Ctrl Pts',(18.9700097425174,4.18111900222879,-328.591629958322)) ;
#29001=CARTESIAN_POINT('Ctrl Pts',(19.0635272449003,3.74494300758538,-328.596862228875)) ;
#29002=CARTESIAN_POINT('Ctrl Pts',(19.1252279979171,3.4158925936385,-328.600814090908)) ;
#29003=CARTESIAN_POINT('Ctrl Pts',(19.1941138378297,2.98771015971316,-328.606038789843)) ;
#29004=CARTESIAN_POINT('Ctrl Pts',(19.2090854597564,2.88988819503593,-328.607238022498)) ;
#29005=CARTESIAN_POINT('Ctrl Pts',(19.2328726949179,2.72610719882213,-328.609258100138)) ;
#29006=CARTESIAN_POINT('Ctrl Pts',(19.2420980601437,2.66020954257854,-328.610074245071)) ;
#29007=CARTESIAN_POINT('Ctrl Pts',(19.2615277079114,2.5160300716269,-328.611868017614)) ;
#29008=CARTESIAN_POINT('Ctrl Pts',(19.2715937206496,2.43773099606517,-328.612847161481)) ;
#29009=CARTESIAN_POINT('Ctrl Pts',(19.3014619344503,2.19364304700804,-328.615912755867)) ;
#29010=CARTESIAN_POINT('Ctrl Pts',(19.3196040811624,2.02765890125357,-328.618016352966)) ;
#29011=CARTESIAN_POINT('Ctrl Pts',(19.3483756561692,1.72879927397616,-328.621826074587)) ;
#29012=CARTESIAN_POINT('Ctrl Pts',(19.3597815846282,1.59600889892476,-328.623526667964)) ;
#29013=CARTESIAN_POINT('Ctrl Pts',(19.4140560922293,0.877480454101865,-328.6327546531)) ;
#29014=CARTESIAN_POINT('Ctrl Pts',(19.4317102667252,0.290144060602212,-328.640381243504)) ;
#29015=CARTESIAN_POINT('Ctrl Pts',(19.4211375599041,-0.401067422563322,
-328.649241150573)) ;
#29016=CARTESIAN_POINT('Ctrl Pts',(19.4187121536292,-0.505032187418889,
-328.650571014867)) ;
#29017=CARTESIAN_POINT('Ctrl Pts',(19.4056527125555,-0.92139738290081,-328.655883612525)) ;
#29018=CARTESIAN_POINT('Ctrl Pts',(19.3883137091128,-1.23354064513692,-328.65983549798)) ;
#29019=CARTESIAN_POINT('Ctrl Pts',(19.3514473338134,-1.69554727671923,-328.665626386004)) ;
#29020=CARTESIAN_POINT('Ctrl Pts',(19.3376922992548,-1.84581990003371,-328.667500912717)) ;
#29021=CARTESIAN_POINT('Ctrl Pts',(19.3094549899377,-2.11918124803914,-328.670894375396)) ;
#29022=CARTESIAN_POINT('Ctrl Pts',(19.2955429734247,-2.24232080165343,-328.672416905486)) ;
#29023=CARTESIAN_POINT('Ctrl Pts',(19.2621451709096,-2.51455673009521,-328.675770019596)) ;
#29024=CARTESIAN_POINT('Ctrl Pts',(19.2421045967728,-2.66357708739031,-328.677596900015)) ;
#29025=CARTESIAN_POINT('Ctrl Pts',(19.1738103485886,-3.13031787574574,-328.683295116365)) ;
#29026=CARTESIAN_POINT('Ctrl Pts',(19.1194015183647,-3.4470827487168,-328.687127015382)) ;
#29027=CARTESIAN_POINT('Ctrl Pts',(18.9557263236737,-4.27613439621117,-328.697113591652)) ;
#29028=CARTESIAN_POINT('Ctrl Pts',(18.833557101158,-4.78560473702088,-328.703203357151)) ;
#29029=CARTESIAN_POINT('Ctrl Pts',(18.6640288810854,-5.38464725988825,-328.710486763052)) ;
#29030=CARTESIAN_POINT('Ctrl Pts',(18.6363803460844,-5.47957368540066,-328.711644876675)) ;
#29031=CARTESIAN_POINT('Ctrl Pts',(18.5180095844289,-5.87471748854718,-328.716487795794)) ;
#29032=CARTESIAN_POINT('Ctrl Pts',(18.42074832925,-6.17292594519729,-328.720195441116)) ;
#29033=CARTESIAN_POINT('Ctrl Pts',(18.2835001178679,-6.56155134176968,-328.725161207465)) ;
#29034=CARTESIAN_POINT('Ctrl Pts',(18.2499836720626,-6.65420382184506,-328.726355312801)) ;
#29035=CARTESIAN_POINT('Ctrl Pts',(18.1926729738228,-6.80894229425044,-328.728369569298)) ;
#29036=CARTESIAN_POINT('Ctrl Pts',(18.1692622368004,-6.87116837787449,-328.729185087108)) ;
#29037=CARTESIAN_POINT('Ctrl Pts',(18.1172739931451,-7.00723028406511,-328.730981112833)) ;
#29038=CARTESIAN_POINT('Ctrl Pts',(18.0885636643284,-7.0810138918785,-328.731963175847)) ;
#29039=CARTESIAN_POINT('Ctrl Pts',(17.9974044190267,-7.31111438525707,-328.735048873475)) ;
#29040=CARTESIAN_POINT('Ctrl Pts',(17.9333742789148,-7.46679624694865,-328.737169962277)) ;
#29041=CARTESIAN_POINT('Ctrl Pts',(17.6602429619318,-8.1070962461664,-328.746004464597)) ;
#29042=CARTESIAN_POINT('Ctrl Pts',(17.4334571860961,-8.58392458218402,-328.752842102091)) ;
#29043=CARTESIAN_POINT('Ctrl Pts',(16.9296851257332,-9.54057833566551,-328.766778429147)) ;
#29044=CARTESIAN_POINT('Ctrl Pts',(16.6510266556395,-10.0189913769374,-328.773866006283)) ;
#29045=CARTESIAN_POINT('Ctrl Pts',(16.2692257675936,-10.6144533087036,-328.782739423047)) ;
#29046=CARTESIAN_POINT('Ctrl Pts',(16.1845908557538,-10.7430603199628,-328.784659746744)) ;
#29047=CARTESIAN_POINT('Ctrl Pts',(16.027834385079,-10.9752023296477,-328.788132641318)) ;
#29048=CARTESIAN_POINT('Ctrl Pts',(15.9562157940351,-11.0790666951431,-328.789688947763)) ;
#29049=CARTESIAN_POINT('Ctrl Pts',(15.8071453887112,-11.2908110515374,-328.792867229578)) ;
#29050=CARTESIAN_POINT('Ctrl Pts',(15.72958882447,-11.3986093454665,-328.794488266968)) ;
#29051=CARTESIAN_POINT('Ctrl Pts',(15.5238717078849,-11.6784438335292,-328.798705695407)) ;
#29052=CARTESIAN_POINT('Ctrl Pts',(15.3939559513521,-11.8491672094131,-328.801287981765)) ;
#29053=CARTESIAN_POINT('Ctrl Pts',(15.1722379539842,-12.130726098726,-328.805569772342)) ;
#29054=CARTESIAN_POINT('Ctrl Pts',(15.0819840011969,-12.2427561788938,-328.807279800864)) ;
#29055=CARTESIAN_POINT('Ctrl Pts',(14.6959333734352,-12.7112032986595,-328.81446533437)) ;
#29056=CARTESIAN_POINT('Ctrl Pts',(14.3886831821545,-13.0579839052764,-328.819867967277)) ;
#29057=CARTESIAN_POINT('Ctrl Pts',(13.9436264774696,-13.5254997984984,-328.827408064073)) ;
#29058=CARTESIAN_POINT('Ctrl Pts',(13.8160675971733,-13.655773147065,-328.829539140338)) ;
#29059=CARTESIAN_POINT('Ctrl Pts',(13.4602783048246,-14.0090448654444,-328.835424021284)) ;
#29060=CARTESIAN_POINT('Ctrl Pts',(13.2283584410324,-14.2282452255454,-328.839194564661)) ;
#29061=CARTESIAN_POINT('Ctrl Pts',(12.9176113072446,-14.507781568872,-328.844230048485)) ;
#29062=CARTESIAN_POINT('Ctrl Pts',(12.8435729370392,-14.5733675623781,-328.845428677288)) ;
#29063=CARTESIAN_POINT('Ctrl Pts',(12.7188985370547,-14.6821208166604,-328.847448068536)) ;
#29064=CARTESIAN_POINT('Ctrl Pts',(12.6685357819987,-14.7255985555529,-328.848264138786)) ;
#29065=CARTESIAN_POINT('Ctrl Pts',(12.5757823455232,-14.8048437851223,-328.849768335297)) ;
#29066=CARTESIAN_POINT('Ctrl Pts',(12.5334600553495,-14.84069001554,-328.850455045954)) ;
#29067=CARTESIAN_POINT('Ctrl Pts',(12.4316346643341,-14.9261880734865,-328.852107476155)) ;
#29068=CARTESIAN_POINT('Ctrl Pts',(12.3719868276337,-14.9756660202979,-328.853075637098)) ;
#29069=CARTESIAN_POINT('Ctrl Pts',(12.2162677354234,-15.1032698640578,-328.85560185962)) ;
#29070=CARTESIAN_POINT('Ctrl Pts',(12.1197427333562,-15.1808364061166,-328.857166498434)) ;
#29071=CARTESIAN_POINT('Ctrl Pts',(11.8114886010359,-15.4237324353542,-328.862150817487)) ;
#29072=CARTESIAN_POINT('Ctrl Pts',(11.5970685372586,-15.5855954733917,-328.865599291756)) ;
#29073=CARTESIAN_POINT('Ctrl Pts',(10.7605296986841,-16.1902643483047,-328.878893990631)) ;
#29074=CARTESIAN_POINT('Ctrl Pts',(10.1158588581006,-16.6006948005297,-328.888781954592)) ;
#29075=CARTESIAN_POINT('Ctrl Pts',(9.28707959837534,-17.0620924036585,-328.900715462584)) ;
#29076=CARTESIAN_POINT('Ctrl Pts',(9.12417581604499,-17.1497597792226,-328.90302732312)) ;
#29077=CARTESIAN_POINT('Ctrl Pts',(8.84806662081084,-17.2933013052925,-328.906888340963)) ;
#29078=CARTESIAN_POINT('Ctrl Pts',(8.73552390719892,-17.3504229077495,-328.908446363769)) ;
#29079=CARTESIAN_POINT('Ctrl Pts',(8.52207399768947,-17.4561571665108,-328.911372094351)) ;
#29080=CARTESIAN_POINT('Ctrl Pts',(8.4212874200101,-17.5050017557113,-328.91274142855)) ;
#29081=CARTESIAN_POINT('Ctrl Pts',(8.15565048331308,-17.6309132893874,-328.916319601425)) ;
#29082=CARTESIAN_POINT('Ctrl Pts',(7.99012972785903,-17.7065401840973,-328.918518181041)) ;
#29083=CARTESIAN_POINT('Ctrl Pts',(7.62523327087576,-17.8671037649761,-328.923302711856)) ;
#29084=CARTESIAN_POINT('Ctrl Pts',(7.42544924867052,-17.9510524211035,-328.92588214141)) ;
#29085=CARTESIAN_POINT('Ctrl Pts',(6.77554638210064,-18.2114333173945,-328.934164740703)) ;
#29086=CARTESIAN_POINT('Ctrl Pts',(6.32023468587314,-18.3744106309521,-328.939797666943)) ;
#29087=CARTESIAN_POINT('Ctrl Pts',(5.74812072314533,-18.5554125739758,-328.946809590416)) ;
#29088=CARTESIAN_POINT('Ctrl Pts',(5.63660815978807,-18.5895905301772,-328.94817351863)) ;
#29089=CARTESIAN_POINT('Ctrl Pts',(5.18622949860399,-18.7232038781322,-328.953679466404)) ;
#29090=CARTESIAN_POINT('Ctrl Pts',(4.84498893126302,-18.8143939847388,-328.957843935287)) ;
#29091=CARTESIAN_POINT('Ctrl Pts',(4.40480269374701,-18.9192549998506,-328.963294756656)) ;
#29092=CARTESIAN_POINT('Ctrl Pts',(4.30797659548703,-18.9415372695713,-328.964498680015)) ;
#29093=CARTESIAN_POINT('Ctrl Pts',(4.14597519600303,-18.9775116705646,-328.966524096919)) ;
#29094=CARTESIAN_POINT('Ctrl Pts',(4.08089272225523,-18.9916132577066,-328.967340829337)) ;
#29095=CARTESIAN_POINT('Ctrl Pts',(3.9550880828026,-19.0181951301683,-328.968926127317)) ;
#29096=CARTESIAN_POINT('Ctrl Pts',(3.8943763013049,-19.0307199276687,-328.969693982674)) ;
#29097=CARTESIAN_POINT('Ctrl Pts',(3.75509229619976,-19.0587596925301,-328.971461176781)) ;
#29098=CARTESIAN_POINT('Ctrl Pts',(3.67648199704405,-19.0740797753528,-328.972462628536)) ;
#29099=CARTESIAN_POINT('Ctrl Pts',(3.46917677656013,-19.1131515870996,-328.97511228646)) ;
#29100=CARTESIAN_POINT('Ctrl Pts',(3.34033273678266,-19.1360896799641,-328.976767895768)) ;
#29101=CARTESIAN_POINT('Ctrl Pts',(2.91965497893381,-19.2066047663371,-328.98219205468)) ;
#29102=CARTESIAN_POINT('Ctrl Pts',(2.62696522986092,-19.2488208781446,-328.98599446048)) ;
#29103=CARTESIAN_POINT('Ctrl Pts',(1.75320651242472,-19.3545466566369,-328.997340702496)) ;
#29104=CARTESIAN_POINT('Ctrl Pts',(1.1701118523581,-19.3985321784804,-329.004897823376)) ;
#29105=CARTESIAN_POINT('Ctrl Pts',(0.390749323107679,-19.4220510608801,
-329.014795385046)) ;
#29106=CARTESIAN_POINT('Ctrl Pts',(0.195497788728379,-19.4249976374814,
-329.017259094025)) ;
#29107=CARTESIAN_POINT('Ctrl Pts',(0.000234885055415066,-19.4249999985799,
-329.01970520092)) ;
#29108=CARTESIAN_POINT('Origin',(0.,0.,-328.125)) ;
#29109=CARTESIAN_POINT('',(-0.000119142683527153,-19.4253123583886,-330.73193689292)) ;
#29110=CARTESIAN_POINT('',(5.03575626882774E-5,-19.4249999999347,-330.517882160562)) ;
#29111=CARTESIAN_POINT('',(-2.37887640734373E-15,-19.425,-328.125)) ;
#29112=CARTESIAN_POINT('Ctrl Pts',(-0.000108465306112585,-19.4254057326986,
-330.731859656045)) ;
#29113=CARTESIAN_POINT('Ctrl Pts',(0.402674651299642,-19.4253741486293,
-330.726849257756)) ;
#29114=CARTESIAN_POINT('Ctrl Pts',(0.805509665086475,-19.4127567695453,
-330.721745417837)) ;
#29115=CARTESIAN_POINT('Ctrl Pts',(1.20759860177362,-19.3876107506117,-330.716618925219)) ;
#29116=CARTESIAN_POINT('Ctrl Pts',(1.60962475126056,-19.3624686582923,-330.711493233116)) ;
#29117=CARTESIAN_POINT('Ctrl Pts',(2.01090509352846,-19.3248020034305,-330.706345044419)) ;
#29118=CARTESIAN_POINT('Ctrl Pts',(2.41065213885928,-19.2747078749785,-330.701224744958)) ;
#29119=CARTESIAN_POINT('Ctrl Pts',(2.81035664497823,-19.2246190773094,-330.696104990376)) ;
#29120=CARTESIAN_POINT('Ctrl Pts',(3.20852822676042,-19.1621055444608,-330.69101320624)) ;
#29121=CARTESIAN_POINT('Ctrl Pts',(3.60438911586109,-19.0873023567467,-330.685977631048)) ;
#29122=CARTESIAN_POINT('Ctrl Pts',(4.00022756142526,-19.0125034100378,-330.680942341351)) ;
#29123=CARTESIAN_POINT('Ctrl Pts',(4.39375352994971,-18.9254076404805,-330.675968388971)) ;
#29124=CARTESIAN_POINT('Ctrl Pts',(4.78420335923599,-18.8262087064853,-330.671048234656)) ;
#29125=CARTESIAN_POINT('Ctrl Pts',(5.17469155317068,-18.7270000254446,-330.666127596899)) ;
#29126=CARTESIAN_POINT('Ctrl Pts',(5.56209903036803,-18.6156685406528,-330.66127095472)) ;
#29127=CARTESIAN_POINT('Ctrl Pts',(5.94566583029117,-18.4924280199309,-330.656457881628)) ;
#29128=CARTESIAN_POINT('Ctrl Pts',(6.3292385142747,-18.3691856086525,-330.651644734702)) ;
#29129=CARTESIAN_POINT('Ctrl Pts',(6.70897049216514,-18.2340336797976,-330.646875082202)) ;
#29130=CARTESIAN_POINT('Ctrl Pts',(7.08410902033399,-18.0872198197287,-330.642108681419)) ;
#29131=CARTESIAN_POINT('Ctrl Pts',(7.45932563463387,-17.9403753999454,-330.637341288495)) ;
#29132=CARTESIAN_POINT('Ctrl Pts',(7.82994684780494,-17.7818640425076,-330.632577014357)) ;
#29133=CARTESIAN_POINT('Ctrl Pts',(8.19522780036955,-17.6119735047545,-330.627754785151)) ;
#29134=CARTESIAN_POINT('Ctrl Pts',(8.46600107051254,-17.4860380675224,-330.624180192054)) ;
#29135=CARTESIAN_POINT('Ctrl Pts',(8.73384009414484,-17.3538507208123,-330.620573300167)) ;
#29136=CARTESIAN_POINT('Ctrl Pts',(8.99844474090565,-17.2155437140451,-330.616902657059)) ;
#29137=CARTESIAN_POINT('Ctrl Pts',(9.35615722376798,-17.0285698895354,-330.611940405353)) ;
#29138=CARTESIAN_POINT('Ctrl Pts',(9.70805425730376,-16.8303596312534,-330.60686136969)) ;
#29139=CARTESIAN_POINT('Ctrl Pts',(10.0534516520941,-16.6213392975729,-330.601742006995)) ;
#29140=CARTESIAN_POINT('Ctrl Pts',(10.398587407984,-16.4124772970214,-330.596626522223)) ;
#29141=CARTESIAN_POINT('Ctrl Pts',(10.7372334913246,-16.1928217428675,-330.591470937802)) ;
#29142=CARTESIAN_POINT('Ctrl Pts',(11.068735856015,-15.962828706399,-330.586331682058)) ;
#29143=CARTESIAN_POINT('Ctrl Pts',(11.40020264532,-15.7328603517783,-330.581192977835)) ;
#29144=CARTESIAN_POINT('Ctrl Pts',(11.724527346361,-15.492556809596,-330.576070702434)) ;
#29145=CARTESIAN_POINT('Ctrl Pts',(12.0410830588788,-15.2424030075675,-330.570999388913)) ;
#29146=CARTESIAN_POINT('Ctrl Pts',(12.3576195334984,-14.9922644080237,-330.565928383588)) ;
#29147=CARTESIAN_POINT('Ctrl Pts',(12.6663880271718,-14.7322767624914,-330.560908380111)) ;
#29148=CARTESIAN_POINT('Ctrl Pts',(12.9667874752304,-14.4629532264957,-330.555950911202)) ;
#29149=CARTESIAN_POINT('Ctrl Pts',(13.2676566956521,-14.1932085154454,-330.550985689675)) ;
#29150=CARTESIAN_POINT('Ctrl Pts',(13.5601306894737,-13.9140986506533,-330.546083196941)) ;
#29151=CARTESIAN_POINT('Ctrl Pts',(13.8436307850831,-13.6261678064441,-330.541231609387)) ;
#29152=CARTESIAN_POINT('Ctrl Pts',(14.1267172650108,-13.3386570422077,-330.536387100111)) ;
#29153=CARTESIAN_POINT('Ctrl Pts',(14.4008559908154,-13.0423509503839,-330.531593280308)) ;
#29154=CARTESIAN_POINT('Ctrl Pts',(14.6654959701515,-12.7378206348702,-330.526815586168)) ;
#29155=CARTESIAN_POINT('Ctrl Pts',(14.9307159449308,-12.4326228986753,-330.522027421045)) ;
#29156=CARTESIAN_POINT('Ctrl Pts',(15.186395394976,-12.1191647291519,-330.517255339955)) ;
#29157=CARTESIAN_POINT('Ctrl Pts',(15.4320058807281,-11.7980519082937,-330.512442964679)) ;
#29158=CARTESIAN_POINT('Ctrl Pts',(15.6776163664798,-11.4769390874361,-330.507630589403)) ;
#29159=CARTESIAN_POINT('Ctrl Pts',(15.9131577290167,-11.1481714825423,-330.502777734163)) ;
#29160=CARTESIAN_POINT('Ctrl Pts',(16.1381295772808,-10.8123876582478,-330.497808699713)) ;
#29161=CARTESIAN_POINT('Ctrl Pts',(16.3627943384096,-10.477062179713,-330.492846448007)) ;
#29162=CARTESIAN_POINT('Ctrl Pts',(16.5769766019597,-10.1346519189442,-330.487767412344)) ;
#29163=CARTESIAN_POINT('Ctrl Pts',(16.7802795418121,-9.78585860641153,-330.482648049649)) ;
#29164=CARTESIAN_POINT('Ctrl Pts',(16.983428479467,-9.43732950519144,-330.477532564877)) ;
#29165=CARTESIAN_POINT('Ctrl Pts',(17.1757147494581,-9.08242709239955,-330.472376980456)) ;
#29166=CARTESIAN_POINT('Ctrl Pts',(17.3567822107624,-8.72186476897166,-330.467237724712)) ;
#29167=CARTESIAN_POINT('Ctrl Pts',(17.5378302406982,-8.36134113951656,-330.462099020489)) ;
#29168=CARTESIAN_POINT('Ctrl Pts',(17.707661991502,-7.99515883449741,-330.456976745088)) ;
#29169=CARTESIAN_POINT('Ctrl Pts',(17.8659589653153,-7.62404360727233,-330.451905431567)) ;
#29170=CARTESIAN_POINT('Ctrl Pts',(18.0242463190186,-7.25295093366409,-330.446834426242)) ;
#29171=CARTESIAN_POINT('Ctrl Pts',(18.1710003612529,-6.8769259217238,-330.441814422765)) ;
#29172=CARTESIAN_POINT('Ctrl Pts',(18.3059387860068,-6.49670675208336,-330.436856953856)) ;
#29173=CARTESIAN_POINT('Ctrl Pts',(18.44108823093,-6.11589298595449,-330.431891732329)) ;
#29174=CARTESIAN_POINT('Ctrl Pts',(18.5643850678305,-5.73087189082319,-330.426989239595)) ;
#29175=CARTESIAN_POINT('Ctrl Pts',(18.6755814948354,-5.3423981724351,-330.422137652041)) ;
#29176=CARTESIAN_POINT('Ctrl Pts',(18.786615690552,-4.95449122218408,-330.417293142765)) ;
#29177=CARTESIAN_POINT('Ctrl Pts',(18.8855847067103,-4.56314166631443,-330.412499322962)) ;
#29178=CARTESIAN_POINT('Ctrl Pts',(18.9722779311626,-4.16911461576395,-330.407721628822)) ;
#29179=CARTESIAN_POINT('Ctrl Pts',(19.0591611559129,-3.77422399995261,-330.402933463699)) ;
#29180=CARTESIAN_POINT('Ctrl Pts',(19.1337145786862,-3.37664408047978,-330.398161382609)) ;
#29181=CARTESIAN_POINT('Ctrl Pts',(19.1957639824324,-2.97715963031415,-330.393349007333)) ;
#29182=CARTESIAN_POINT('Ctrl Pts',(19.2578133861786,-2.57767518014851,-330.388536632057)) ;
#29183=CARTESIAN_POINT('Ctrl Pts',(19.3073585678561,-2.17628615879326,-330.383683776818)) ;
#29184=CARTESIAN_POINT('Ctrl Pts',(19.3442656246268,-1.77379270750654,-330.378714742367)) ;
#29185=CARTESIAN_POINT('Ctrl Pts',(19.3811223031729,-1.37184866078595,-330.373752490662)) ;
#29186=CARTESIAN_POINT('Ctrl Pts',(19.4053844665361,-0.968698346227976,
-330.368673454999)) ;
#29187=CARTESIAN_POINT('Ctrl Pts',(19.4170393753042,-0.565147824828563,
-330.363554092304)) ;
#29188=CARTESIAN_POINT('Ctrl Pts',(19.4286854554663,-0.161902993386298,
-330.358438607532)) ;
#29189=CARTESIAN_POINT('Ctrl Pts',(19.4277435671211,0.241741460408317,-330.353283023111)) ;
#29190=CARTESIAN_POINT('Ctrl Pts',(19.4142422810442,0.644988692133317,-330.348143767366)) ;
#29191=CARTESIAN_POINT('Ctrl Pts',(19.4007424438665,1.04819264912468,-330.343005063144)) ;
#29192=CARTESIAN_POINT('Ctrl Pts',(19.3746860211204,1.45099950969481,-330.337882787743)) ;
#29193=CARTESIAN_POINT('Ctrl Pts',(19.3361405488261,1.85261959181327,-330.332811474221)) ;
#29194=CARTESIAN_POINT('Ctrl Pts',(19.2975974190382,2.25421526645776,-330.327740468897)) ;
#29195=CARTESIAN_POINT('Ctrl Pts',(19.2465668059578,2.6546243510754,-330.32272046542)) ;
#29196=CARTESIAN_POINT('Ctrl Pts',(19.1831539722185,3.0530635659536,-330.31776299651)) ;
#29197=CARTESIAN_POINT('Ctrl Pts',(19.1196419718631,3.45212587029724,-330.312797774984)) ;
#29198=CARTESIAN_POINT('Ctrl Pts',(19.0437089669166,3.8492121738211,-330.30789528225)) ;
#29199=CARTESIAN_POINT('Ctrl Pts',(18.9554984251055,4.24354119325974,-330.303043694696)) ;
#29200=CARTESIAN_POINT('Ctrl Pts',(18.8674165790657,4.63729490189939,-330.29819918542)) ;
#29201=CARTESIAN_POINT('Ctrl Pts',(18.7670929256151,5.02829938473267,-330.293405365617)) ;
#29202=CARTESIAN_POINT('Ctrl Pts',(18.6547085679444,5.41578201386611,-330.288627671477)) ;
#29203=CARTESIAN_POINT('Ctrl Pts',(18.5420779042709,5.80411386525304,-330.283839506354)) ;
#29204=CARTESIAN_POINT('Ctrl Pts',(18.4173334587013,6.18890839291264,-330.279067425264)) ;
#29205=CARTESIAN_POINT('Ctrl Pts',(18.2806977008023,6.56939311546342,-330.274255049988)) ;
#29206=CARTESIAN_POINT('Ctrl Pts',(18.1440619429034,6.94987783801368,-330.269442674711)) ;
#29207=CARTESIAN_POINT('Ctrl Pts',(17.9955346750036,7.32605269387698,-330.264589819473)) ;
#29208=CARTESIAN_POINT('Ctrl Pts',(17.8353811203026,7.69715099363916,-330.259620785022)) ;
#29209=CARTESIAN_POINT('Ctrl Pts',(17.6754461756045,8.06774274329367,-330.254658533316)) ;
#29210=CARTESIAN_POINT('Ctrl Pts',(17.5038745173134,8.43336822759492,-330.249579497653)) ;
#29211=CARTESIAN_POINT('Ctrl Pts',(17.3210405978621,8.79331352638083,-330.244460134959)) ;
#29212=CARTESIAN_POINT('Ctrl Pts',(17.138345175303,9.15298616621259,-330.239344650187)) ;
#29213=CARTESIAN_POINT('Ctrl Pts',(16.9444047068852,9.50698733420804,-330.234189065765)) ;
#29214=CARTESIAN_POINT('Ctrl Pts',(16.7396255112679,9.85463096734606,-330.229049810021)) ;
#29215=CARTESIAN_POINT('Ctrl Pts',(16.5348682916581,10.2022372928901,-330.223911105798)) ;
#29216=CARTESIAN_POINT('Ctrl Pts',(16.3192747541773,10.5434875393202,-330.218788830397)) ;
#29217=CARTESIAN_POINT('Ctrl Pts',(16.0932820073231,10.8777205750419,-330.213717516876)) ;
#29218=CARTESIAN_POINT('Ctrl Pts',(15.8673029946267,11.2119332985663,-330.208646511551)) ;
#29219=CARTESIAN_POINT('Ctrl Pts',(15.6309260577843,11.5391297261789,-330.203626508074)) ;
#29220=CARTESIAN_POINT('Ctrl Pts',(15.3846183710913,11.8586723976787,-330.198669039165)) ;
#29221=CARTESIAN_POINT('Ctrl Pts',(15.1379255021176,12.1787147782076,-330.193703817638)) ;
#29222=CARTESIAN_POINT('Ctrl Pts',(14.8812707592671,12.4910794635653,-330.188801324904)) ;
#29223=CARTESIAN_POINT('Ctrl Pts',(14.6151539106746,12.7951490249379,-330.18394973735)) ;
#29224=CARTESIAN_POINT('Ctrl Pts',(14.3494253162779,13.0987749605738,-330.179105228074)) ;
#29225=CARTESIAN_POINT('Ctrl Pts',(14.0742621359218,13.3941299422748,-330.174311408271)) ;
#29226=CARTESIAN_POINT('Ctrl Pts',(13.7901930455831,13.6806221474832,-330.169533714131)) ;
#29227=CARTESIAN_POINT('Ctrl Pts',(13.5055013781947,13.9677422403357,-330.164745549008)) ;
#29228=CARTESIAN_POINT('Ctrl Pts',(13.2118645930312,14.2459605783631,-330.159973467918)) ;
#29229=CARTESIAN_POINT('Ctrl Pts',(12.909847620977,14.5147052583501,-330.155161092642)) ;
#29230=CARTESIAN_POINT('Ctrl Pts',(12.6078306489231,14.7834499383368,-330.150348717366)) ;
#29231=CARTESIAN_POINT('Ctrl Pts',(12.2974333458584,15.0427208116386,-330.145495862126)) ;
#29232=CARTESIAN_POINT('Ctrl Pts',(11.9792554148419,15.2919715155149,-330.140526827676)) ;
#29233=CARTESIAN_POINT('Ctrl Pts',(11.6615117974963,15.5408819915575,-330.13556457597)) ;
#29234=CARTESIAN_POINT('Ctrl Pts',(11.3359256303457,15.7798641592174,-330.130485540307)) ;
#29235=CARTESIAN_POINT('Ctrl Pts',(11.0031672876764,16.0084702518838,-330.125366177613)) ;
#29236=CARTESIAN_POINT('Ctrl Pts',(10.6706610098141,16.2369031751859,-330.120250692841)) ;
#29237=CARTESIAN_POINT('Ctrl Pts',(10.3309935048472,16.4549759114473,-330.11509510842)) ;
#29238=CARTESIAN_POINT('Ctrl Pts',(9.98484980217588,16.6622804017955,-330.109955852675)) ;
#29239=CARTESIAN_POINT('Ctrl Pts',(9.63874324613229,16.8695626451329,-330.104817148452)) ;
#29240=CARTESIAN_POINT('Ctrl Pts',(9.28616191162137,17.0660790735682,-330.099694873052)) ;
#29241=CARTESIAN_POINT('Ctrl Pts',(8.9278059376802,17.251458251842,-330.09462355953)) ;
#29242=CARTESIAN_POINT('Ctrl Pts',(8.56947174194395,17.4368261641511,-330.089552554205)) ;
#29243=CARTESIAN_POINT('Ctrl Pts',(8.20536359771144,17.6110582444914,-330.084532550729)) ;
#29244=CARTESIAN_POINT('Ctrl Pts',(7.83619672068672,17.7738182283462,-330.079575081819)) ;
#29245=CARTESIAN_POINT('Ctrl Pts',(7.46645253103106,17.9368327404384,-330.074609860293)) ;
#29246=CARTESIAN_POINT('Ctrl Pts',(7.09163373071272,18.0883392439755,-330.069707367559)) ;
#29247=CARTESIAN_POINT('Ctrl Pts',(6.71247457351918,18.2280346582659,-330.064855780004)) ;
#29248=CARTESIAN_POINT('Ctrl Pts',(6.33386859488192,18.367526262346,-330.060011270729)) ;
#29249=CARTESIAN_POINT('Ctrl Pts',(5.95093486173872,18.4952411677311,-330.055217450926)) ;
#29250=CARTESIAN_POINT('Ctrl Pts',(5.56442076202264,18.6109126095375,-330.050439756786)) ;
#29251=CARTESIAN_POINT('Ctrl Pts',(5.17705956272058,18.72683756145,-330.045651591662)) ;
#29252=CARTESIAN_POINT('Ctrl Pts',(4.78610221554313,18.830666063824,-330.040879510572)) ;
#29253=CARTESIAN_POINT('Ctrl Pts',(4.39231841500205,18.9221661887551,-330.036067135296)) ;
#29254=CARTESIAN_POINT('Ctrl Pts',(3.9985346144603,19.0136663136863,-330.03125476002)) ;
#29255=CARTESIAN_POINT('Ctrl Pts',(3.60192430511406,19.0928378616947,-330.026401904781)) ;
#29256=CARTESIAN_POINT('Ctrl Pts',(3.20327549673131,19.1594879685595,-330.021432870331)) ;
#29257=CARTESIAN_POINT('Ctrl Pts',(2.80517084496984,19.2260470978615,-330.016470618625)) ;
#29258=CARTESIAN_POINT('Ctrl Pts',(2.40492937024616,19.2801358269128,-330.011391582962)) ;
#29259=CARTESIAN_POINT('Ctrl Pts',(2.00335396996647,19.3216816824276,-330.006272220267)) ;
#29260=CARTESIAN_POINT('Ctrl Pts',(1.6020827634881,19.3631960669117,-330.001156735495)) ;
#29261=CARTESIAN_POINT('Ctrl Pts',(1.19947964438572,19.3921867675156,-329.996001151074)) ;
#29262=CARTESIAN_POINT('Ctrl Pts',(0.796341381989622,19.4086231908243,-329.990861895329)) ;
#29263=CARTESIAN_POINT('Ctrl Pts',(0.393246382627672,19.4250578502481,-329.985723191107)) ;
#29264=CARTESIAN_POINT('Ctrl Pts',(-0.0103836768102819,19.4289410461147,
-329.980600915706)) ;
#29265=CARTESIAN_POINT('Ctrl Pts',(-0.413756280420004,19.4202815740748,
-329.975529602185)) ;
#29266=CARTESIAN_POINT('Ctrl Pts',(-0.817104370046287,19.4116226282931,
-329.97045859686)) ;
#29267=CARTESIAN_POINT('Ctrl Pts',(-1.22019507561338,19.3904225905207,-329.965438593383)) ;
#29268=CARTESIAN_POINT('Ctrl Pts',(-1.6222394685035,19.3567283538937,-329.960481124473)) ;
#29269=CARTESIAN_POINT('Ctrl Pts',(-2.02491258872684,19.3229814253553,-329.955515902947)) ;
#29270=CARTESIAN_POINT('Ctrl Pts',(-2.42653615787623,19.2767011661808,-329.950613410213)) ;
#29271=CARTESIAN_POINT('Ctrl Pts',(-2.82632040539988,19.2179727174615,-329.945761822659)) ;
#29272=CARTESIAN_POINT('Ctrl Pts',(-3.22552138315938,19.1593299512789,-329.940917313383)) ;
#29273=CARTESIAN_POINT('Ctrl Pts',(-3.62288842607095,19.0882752241637,-329.93612349358)) ;
#29274=CARTESIAN_POINT('Ctrl Pts',(-4.01763760448166,19.0049318508567,-329.93134579944)) ;
#29275=CARTESIAN_POINT('Ctrl Pts',(-4.4132519307991,18.9214058189177,-329.926557634317)) ;
#29276=CARTESIAN_POINT('Ctrl Pts',(-4.80623690085269,18.8255370621331,-329.921785553227)) ;
#29277=CARTESIAN_POINT('Ctrl Pts',(-5.19580566380469,18.7174901586082,-329.916973177951)) ;
#29278=CARTESIAN_POINT('Ctrl Pts',(-5.58537442675735,18.609443255083,-329.912160802675)) ;
#29279=CARTESIAN_POINT('Ctrl Pts',(-5.97152693585674,18.4892180031243,-329.907307947436)) ;
#29280=CARTESIAN_POINT('Ctrl Pts',(-6.35347894613258,18.3570220462464,-329.902338912985)) ;
#29281=CARTESIAN_POINT('Ctrl Pts',(-6.73490959095979,18.2250065371801,-329.897376661279)) ;
#29282=CARTESIAN_POINT('Ctrl Pts',(-7.11225049723722,18.0810181030995,-329.892297625616)) ;
#29283=CARTESIAN_POINT('Ctrl Pts',(-7.48476194469701,17.9253772288684,-329.887178262922)) ;
#29284=CARTESIAN_POINT('Ctrl Pts',(-7.85699121433129,17.7698542527684,-329.88206277815)) ;
#29285=CARTESIAN_POINT('Ctrl Pts',(-8.22439843833507,17.6026966505424,-329.876907193728)) ;
#29286=CARTESIAN_POINT('Ctrl Pts',(-8.58626931403335,17.424258751148,-329.871767937984)) ;
#29287=CARTESIAN_POINT('Ctrl Pts',(-8.948101355329,17.24584000093,-329.866629233761)) ;
#29288=CARTESIAN_POINT('Ctrl Pts',(-9.30439832140479,17.0561434641823,-329.86150695836)) ;
#29289=CARTESIAN_POINT('Ctrl Pts',(-9.6544684893318,16.8555560235912,-329.856435644839)) ;
#29290=CARTESIAN_POINT('Ctrl Pts',(-10.0045173826051,16.6549807732087,-329.851364639514)) ;
#29291=CARTESIAN_POINT('Ctrl Pts',(-10.3483402947084,16.4435159685035,-329.846344636037)) ;
#29292=CARTESIAN_POINT('Ctrl Pts',(-10.6852668795819,16.2215802304122,-329.841387167128)) ;
#29293=CARTESIAN_POINT('Ctrl Pts',(-11.0227203588905,15.9992974235214,-329.836421945601)) ;
#29294=CARTESIAN_POINT('Ctrl Pts',(-11.3532559456396,15.7665108698316,-329.831519452867)) ;
#29295=CARTESIAN_POINT('Ctrl Pts',(-11.6762208531975,15.5236731797096,-329.826667865313)) ;
#29296=CARTESIAN_POINT('Ctrl Pts',(-11.998714567437,15.2811897803923,-329.821823356038)) ;
#29297=CARTESIAN_POINT('Ctrl Pts',(-12.3136596654231,15.0286844808624,-329.817029536234)) ;
#29298=CARTESIAN_POINT('Ctrl Pts',(-12.6204267527925,14.7666406184365,-329.812251842094)) ;
#29299=CARTESIAN_POINT('Ctrl Pts',(-12.9278661630434,14.5040224503178,-329.807463676971)) ;
#29300=CARTESIAN_POINT('Ctrl Pts',(-13.2270915988808,14.2318237292235,-329.802691595881)) ;
#29301=CARTESIAN_POINT('Ctrl Pts',(-13.517490842168,13.9505654245815,-329.797879220605)) ;
#29302=CARTESIAN_POINT('Ctrl Pts',(-13.8078900854546,13.66930711994,-329.793066845329)) ;
#29303=CARTESIAN_POINT('Ctrl Pts',(-14.0894629986418,13.3789890770053,-329.78821399009)) ;
#29304=CARTESIAN_POINT('Ctrl Pts',(-14.3616202554224,13.0801688354689,-329.783244955639)) ;
#29305=CARTESIAN_POINT('Ctrl Pts',(-14.6334060168663,12.7817564843102,-329.778282703933)) ;
#29306=CARTESIAN_POINT('Ctrl Pts',(-14.895872321534,12.4747869945993,-329.773203668271)) ;
#29307=CARTESIAN_POINT('Ctrl Pts',(-15.1485229275982,12.1598956935516,-329.768084305576)) ;
#29308=CARTESIAN_POINT('Ctrl Pts',(-15.4009821505541,11.8452429230061,-329.762968820804)) ;
#29309=CARTESIAN_POINT('Ctrl Pts',(-15.6436407073037,11.5226804374807,-329.757813236383)) ;
#29310=CARTESIAN_POINT('Ctrl Pts',(-15.876040867779,11.1928611232644,-329.752673980638)) ;
#29311=CARTESIAN_POINT('Ctrl Pts',(-16.1084160880843,10.8630772038162,-329.747535276416)) ;
#29312=CARTESIAN_POINT('Ctrl Pts',(-16.3305352311991,10.5260380512659,-329.742413001015)) ;
#29313=CARTESIAN_POINT('Ctrl Pts',(-16.5419759694787,10.1824143355649,-329.737341687493)) ;
#29314=CARTESIAN_POINT('Ctrl Pts',(-16.7534038579647,9.83881150275446,-329.732270682169)) ;
#29315=CARTESIAN_POINT('Ctrl Pts',(-16.9541547046722,9.48862490098346,-329.727250678692)) ;
#29316=CARTESIAN_POINT('Ctrl Pts',(-17.1438401379526,9.13254284325703,-329.722293209782)) ;
#29317=CARTESIAN_POINT('Ctrl Pts',(-17.3338222061812,8.77590393527117,-329.717327988256)) ;
#29318=CARTESIAN_POINT('Ctrl Pts',(-17.5127042251083,8.41335107430971,-329.712425495522)) ;
#29319=CARTESIAN_POINT('Ctrl Pts',(-17.6801295038996,8.04559401961159,-329.707573907968)) ;
#29320=CARTESIAN_POINT('Ctrl Pts',(-17.8473105156807,7.67837350824137,-329.702729398692)) ;
#29321=CARTESIAN_POINT('Ctrl Pts',(-18.0030681487466,7.30596392084994,-329.697935578889)) ;
#29322=CARTESIAN_POINT('Ctrl Pts',(-18.1470809542084,6.9290908074623,-329.693157884749)) ;
#29323=CARTESIAN_POINT('Ctrl Pts',(-18.2914093838285,6.55139172405881,-329.688369719625)) ;
#29324=CARTESIAN_POINT('Ctrl Pts',(-18.4239413159214,6.1692094479231,-329.683597638536)) ;
#29325=CARTESIAN_POINT('Ctrl Pts',(-18.5443883886575,5.78329435739147,-329.678785263259)) ;
#29326=CARTESIAN_POINT('Ctrl Pts',(-18.6648354613935,5.39737926686037,-329.673972887983)) ;
#29327=CARTESIAN_POINT('Ctrl Pts',(-18.7731974799528,5.00773129185362,-329.669120032744)) ;
#29328=CARTESIAN_POINT('Ctrl Pts',(-18.8692236805865,4.61512197209525,-329.664150998294)) ;
#29329=CARTESIAN_POINT('Ctrl Pts',(-18.9651188052163,4.22304856504,-329.659188746588)) ;
#29330=CARTESIAN_POINT('Ctrl Pts',(-19.0487363029649,3.82791954463094,-329.654109710925)) ;
#29331=CARTESIAN_POINT('Ctrl Pts',(-19.1199443656912,3.43053022416198,-329.648990348231)) ;
#29332=CARTESIAN_POINT('Ctrl Pts',(-19.1910984882332,3.03344192653243,-329.643874863459)) ;
#29333=CARTESIAN_POINT('Ctrl Pts',(-19.2498621633251,2.63409675913522,-329.638719279037)) ;
#29334=CARTESIAN_POINT('Ctrl Pts',(-19.2961458017985,2.23328702942527,-329.633580023292)) ;
#29335=CARTESIAN_POINT('Ctrl Pts',(-19.3424244733139,1.83252031286454,-329.62844131907)) ;
#29336=CARTESIAN_POINT('Ctrl Pts',(-19.3762259080336,1.43028932561657,-329.623319043669)) ;
#29337=CARTESIAN_POINT('Ctrl Pts',(-19.3975001128118,1.02738505409656,-329.618247730148)) ;
#29338=CARTESIAN_POINT('Ctrl Pts',(-19.4187730247023,0.624505268099502,
-329.613176724823)) ;
#29339=CARTESIAN_POINT('Ctrl Pts',(-19.4275202835506,0.220952243111883,
-329.608156721346)) ;
#29340=CARTESIAN_POINT('Ctrl Pts',(-19.4237301548154,-0.182483786957448,
-329.603199252437)) ;
#29341=CARTESIAN_POINT('Ctrl Pts',(-19.4199340989795,-0.586550720641379,
-329.59823403091)) ;
#29342=CARTESIAN_POINT('Ctrl Pts',(-19.4035613913778,-0.99050033152334,
-329.593331538176)) ;
#29343=CARTESIAN_POINT('Ctrl Pts',(-19.3746383777031,-1.39353871001521,
-329.588479950622)) ;
#29344=CARTESIAN_POINT('Ctrl Pts',(-19.3457575615872,-1.7959890710923,-329.583635441346)) ;
#29345=CARTESIAN_POINT('Ctrl Pts',(-19.3043629677051,-2.19753088539806,
-329.578841621543)) ;
#29346=CARTESIAN_POINT('Ctrl Pts',(-19.2505194434125,-2.59737323761063,
-329.574063927403)) ;
#29347=CARTESIAN_POINT('Ctrl Pts',(-19.1965579135233,-2.99809190012976,
-329.56927576228)) ;
#29348=CARTESIAN_POINT('Ctrl Pts',(-19.1300926713332,-3.39710365032791,
-329.56450368119)) ;
#29349=CARTESIAN_POINT('Ctrl Pts',(-19.0512294973661,-3.79361160008601,
-329.559691305914)) ;
#29350=CARTESIAN_POINT('Ctrl Pts',(-18.972366323399,-4.19011954984452,-329.554878930638)) ;
#29351=CARTESIAN_POINT('Ctrl Pts',(-18.8811050130503,-4.58412366749528,
-329.550026075399)) ;
#29352=CARTESIAN_POINT('Ctrl Pts',(-18.7775944869237,-4.97482647033875,
-329.545057040948)) ;
#29353=CARTESIAN_POINT('Ctrl Pts',(-18.6742252529241,-5.36499596287974,
-329.540094789242)) ;
#29354=CARTESIAN_POINT('Ctrl Pts',(-18.5586128019716,-5.7519747605986,-329.53501575358)) ;
#29355=CARTESIAN_POINT('Ctrl Pts',(-18.4310218868634,-6.13500141580958,
-329.529896390885)) ;
#29356=CARTESIAN_POINT('Ctrl Pts',(-18.3035276220115,-6.51773792791467,
-329.524780906113)) ;
#29357=CARTESIAN_POINT('Ctrl Pts',(-18.1640732076723,-6.89652836939212,
-329.519625321692)) ;
#29358=CARTESIAN_POINT('Ctrl Pts',(-18.0129590322685,-7.27063413065785,
-329.514486065947)) ;
#29359=CARTESIAN_POINT('Ctrl Pts',(-17.8618610737785,-7.64469974452619,
-329.509347361725)) ;
#29360=CARTESIAN_POINT('Ctrl Pts',(-17.6991059523496,-8.01408176160161,
-329.504225086323)) ;
#29361=CARTESIAN_POINT('Ctrl Pts',(-17.5250281947923,-8.37806167604782,
-329.499153772802)) ;
#29362=CARTESIAN_POINT('Ctrl Pts',(-17.3509610163828,-8.74201947050942,
-329.494082767477)) ;
#29363=CARTESIAN_POINT('Ctrl Pts',(-17.165572608229,-9.10057587700563,-329.489062764001)) ;
#29364=CARTESIAN_POINT('Ctrl Pts',(-16.9692307331029,-9.45303135434919,
-329.484105295091)) ;
#29365=CARTESIAN_POINT('Ctrl Pts',(-16.7725818135176,-9.80603801060642,
-329.479140073565)) ;
#29366=CARTESIAN_POINT('Ctrl Pts',(-16.5649451048215,-10.1529246648428,
-329.47423758083)) ;
#29367=CARTESIAN_POINT('Ctrl Pts',(-16.3467235676692,-10.4930067666653,
-329.469385993276)) ;
#29368=CARTESIAN_POINT('Ctrl Pts',(-16.1288204073066,-10.8325927018433,
-329.464541484001)) ;
#29369=CARTESIAN_POINT('Ctrl Pts',(-15.9003632101785,-11.1653939189612,
-329.459747664198)) ;
#29370=CARTESIAN_POINT('Ctrl Pts',(-15.6617873138256,-11.4907469171131,
-329.454969970058)) ;
#29371=CARTESIAN_POINT('Ctrl Pts',(-15.4226885451021,-11.816812971764,-329.450181804934)) ;
#29372=CARTESIAN_POINT('Ctrl Pts',(-15.1734265359729,-12.1353980561948,
-329.445409723845)) ;
#29373=CARTESIAN_POINT('Ctrl Pts',(-14.9144754261016,-12.4458530080436,
-329.440597348569)) ;
#29374=CARTESIAN_POINT('Ctrl Pts',(-14.6555243162303,-12.7563079598923,
-329.435784973292)) ;
#29375=CARTESIAN_POINT('Ctrl Pts',(-14.3868839410984,-13.0586326534627,
-329.430932118053)) ;
#29376=CARTESIAN_POINT('Ctrl Pts',(-14.109066607375,-13.3521980435425,-329.425963083603)) ;
#29377=CARTESIAN_POINT('Ctrl Pts',(-13.8316284950075,-13.6453627161301,
-329.421000831897)) ;
#29378=CARTESIAN_POINT('Ctrl Pts',(-13.5449657684854,-13.9298680937984,
-329.415921796234)) ;
#29379=CARTESIAN_POINT('Ctrl Pts',(-13.2496752100234,-14.205172191667,-329.41080243354)) ;
#29380=CARTESIAN_POINT('Ctrl Pts',(-12.9546083344793,-14.4802677463833,
-329.405686948768)) ;
#29381=CARTESIAN_POINT('Ctrl Pts',(-12.6509268046961,-14.7461761153773,
-329.400531364346)) ;
#29382=CARTESIAN_POINT('Ctrl Pts',(-12.3392477692486,-15.0023924175166,
-329.395392108602)) ;
#29383=CARTESIAN_POINT('Ctrl Pts',(-12.0276021818338,-15.2585812236415,
-329.390253404379)) ;
#29384=CARTESIAN_POINT('Ctrl Pts',(-11.7079608519094,-15.5050801572995,
-329.385131128978)) ;
#29385=CARTESIAN_POINT('Ctrl Pts',(-11.3809612878261,-15.7414183236748,
-329.380059815457)) ;
#29386=CARTESIAN_POINT('Ctrl Pts',(-11.0539815963396,-15.9777421271773,
-329.374988810132)) ;
#29387=CARTESIAN_POINT('Ctrl Pts',(-10.7196445637678,-16.2039064638128,
-329.369968806655)) ;
#29388=CARTESIAN_POINT('Ctrl Pts',(-10.3786078107617,-16.4194729930648,
-329.365011337746)) ;
#29389=CARTESIAN_POINT('Ctrl Pts',(-10.0370377357319,-16.6353766307857,
-329.360046116219)) ;
#29390=CARTESIAN_POINT('Ctrl Pts',(-9.68874692593803,-16.8406492921397,
-329.355143623485)) ;
#29391=CARTESIAN_POINT('Ctrl Pts',(-9.33441673834071,-17.0348826399849,
-329.350292035931)) ;
#29392=CARTESIAN_POINT('Ctrl Pts',(-8.98060350479251,-17.2288326088827,
-329.345447526656)) ;
#29393=CARTESIAN_POINT('Ctrl Pts',(-8.62076844326921,-17.4117754128841,
-329.340653706852)) ;
#29394=CARTESIAN_POINT('Ctrl Pts',(-8.25561127121673,-17.5833366889,-329.335876012712)) ;
#29395=CARTESIAN_POINT('Ctrl Pts',(-7.88965380626628,-17.7552739653926,
-329.331087847589)) ;
#29396=CARTESIAN_POINT('Ctrl Pts',(-7.5183507868964,-17.9157796444934,-329.326315766499)) ;
#29397=CARTESIAN_POINT('Ctrl Pts',(-7.14242914390155,-18.064510518084,-329.321503391223)) ;
#29398=CARTESIAN_POINT('Ctrl Pts',(-6.76650750090671,-18.2132413916746,
-329.316691015947)) ;
#29399=CARTESIAN_POINT('Ctrl Pts',(-6.38596714995471,-18.3501972706682,
-329.311838160707)) ;
#29400=CARTESIAN_POINT('Ctrl Pts',(-6.00155891284836,-18.4750708724202,
-329.306869126257)) ;
#29401=CARTESIAN_POINT('Ctrl Pts',(-5.61714582334436,-18.5999460504558,
-329.301900029083)) ;
#29402=CARTESIAN_POINT('Ctrl Pts',(-5.22876506703618,-18.7127705519045,
-329.296813838182)) ;
#29403=CARTESIAN_POINT('Ctrl Pts',(-4.83720163750646,-18.8133536643378,
-329.291687298428)) ;
#29404=CARTESIAN_POINT('Ctrl Pts',(-4.44269726062567,-18.9146922345483,
-329.286522254354)) ;
#29405=CARTESIAN_POINT('Ctrl Pts',(-4.0449622374953,-19.0036049824047,-329.281316452944)) ;
#29406=CARTESIAN_POINT('Ctrl Pts',(-3.64480127510044,-19.0799397939025,
-329.276127822886)) ;
#29407=CARTESIAN_POINT('Ctrl Pts',(-3.24773361572114,-19.1556845260952,
-329.2709793017)) ;
#29408=CARTESIAN_POINT('Ctrl Pts',(-2.84827736176992,-19.2190452047198,
-329.265847764364)) ;
#29409=CARTESIAN_POINT('Ctrl Pts',(-2.44722057878536,-19.2699127853372,
-329.260767661831)) ;
#29410=CARTESIAN_POINT('Ctrl Pts',(-2.04147722616975,-19.3213747816799,
-329.255628195498)) ;
#29411=CARTESIAN_POINT('Ctrl Pts',(-1.63409567639069,-19.3600499784979,
-329.250541467613)) ;
#29412=CARTESIAN_POINT('Ctrl Pts',(-1.2258943436162,-19.3858651114941,-329.245518998991)) ;
#29413=CARTESIAN_POINT('Ctrl Pts',(-0.817693010841706,-19.4116802444903,
-329.240496530368)) ;
#29414=CARTESIAN_POINT('Ctrl Pts',(-0.408671848873124,-19.4246353027172,
-329.235538311889)) ;
#29415=CARTESIAN_POINT('Ctrl Pts',(0.00034766423293037,-19.4246965399752,
-329.230631277206)) ;
#29416=CARTESIAN_POINT('Ctrl Pts',(0.000234860130568747,-19.4249999985802,
-329.019705201232)) ;
#29417=CARTESIAN_POINT('Ctrl Pts',(-0.126046610261835,-19.4250015254004,
-329.021287160577)) ;
#29418=CARTESIAN_POINT('Ctrl Pts',(-0.252325183923784,-19.4237716230069,
-329.022861695855)) ;
#29419=CARTESIAN_POINT('Ctrl Pts',(-0.497313765973587,-19.4189960193607,
-329.025901815613)) ;
#29420=CARTESIAN_POINT('Ctrl Pts',(-0.616021015960607,-19.415592845199,
-329.027368237702)) ;
#29421=CARTESIAN_POINT('Ctrl Pts',(-0.860833286120161,-19.4063269595396,
-329.030379035671)) ;
#29422=CARTESIAN_POINT('Ctrl Pts',(-0.986927450483557,-19.4003230453251,
-329.031922428832)) ;
#29423=CARTESIAN_POINT('Ctrl Pts',(-1.29779130204551,-19.3824828132906,
-329.035710337357)) ;
#29424=CARTESIAN_POINT('Ctrl Pts',(-1.48246744420815,-19.3692331466568,
-329.03794568431)) ;
#29425=CARTESIAN_POINT('Ctrl Pts',(-2.16575504279031,-19.3103807931307,
-329.046170321658)) ;
#29426=CARTESIAN_POINT('Ctrl Pts',(-2.66273693011824,-19.2481462644099,
-329.05205648756)) ;
#29427=CARTESIAN_POINT('Ctrl Pts',(-3.77474229733379,-19.0649995822922,
-329.065233742579)) ;
#29428=CARTESIAN_POINT('Ctrl Pts',(-4.38743975061462,-18.9333899647806,
-329.0724950833)) ;
#29429=CARTESIAN_POINT('Ctrl Pts',(-5.08872671248827,-18.7468759528274,
-329.08120333217)) ;
#29430=CARTESIAN_POINT('Ctrl Pts',(-5.18455191753345,-18.7206014573183,
-329.082402285589)) ;
#29431=CARTESIAN_POINT('Ctrl Pts',(-5.33991150447989,-18.6767187633371,
-329.084363620134)) ;
#29432=CARTESIAN_POINT('Ctrl Pts',(-5.39957052763507,-18.6595583213338,
-329.085120998125)) ;
#29433=CARTESIAN_POINT('Ctrl Pts',(-5.52297683532595,-18.6234200838414,
-329.086697292404)) ;
#29434=CARTESIAN_POINT('Ctrl Pts',(-5.586710808117,-18.6044003142872,-329.087516875054)) ;
#29435=CARTESIAN_POINT('Ctrl Pts',(-5.74481467636614,-18.5563325740781,
-329.089563021076)) ;
#29436=CARTESIAN_POINT('Ctrl Pts',(-5.83906310599182,-18.526891705618,-329.090794197824)) ;
#29437=CARTESIAN_POINT('Ctrl Pts',(-6.23431758458721,-18.4001083704002,
-329.095999567488)) ;
#29438=CARTESIAN_POINT('Ctrl Pts',(-6.53314649935522,-18.2961389348601,
-329.100037404475)) ;
#29439=CARTESIAN_POINT('Ctrl Pts',(-7.22487132458085,-18.0363633532905,
-329.109529116724)) ;
#29440=CARTESIAN_POINT('Ctrl Pts',(-7.61548811129174,-17.874940831897,-329.114999464136)) ;
#29441=CARTESIAN_POINT('Ctrl Pts',(-8.29335589944453,-17.5685553684375,
-329.124567755624)) ;
#29442=CARTESIAN_POINT('Ctrl Pts',(-8.58285359440435,-17.4289562096154,
-329.12867980861)) ;
#29443=CARTESIAN_POINT('Ctrl Pts',(-9.02457781680675,-17.2022758719631,
-329.134968444941)) ;
#29444=CARTESIAN_POINT('Ctrl Pts',(-9.17931211165127,-17.1202082120269,
-329.137174332155)) ;
#29445=CARTESIAN_POINT('Ctrl Pts',(-9.4433807839012,-16.9755426773974,-329.140942054621)) ;
#29446=CARTESIAN_POINT('Ctrl Pts',(-9.55325490127617,-16.9139531352362,
-329.1425107172)) ;
#29447=CARTESIAN_POINT('Ctrl Pts',(-9.75414939261759,-16.7987603854043,
-329.145380519007)) ;
#29448=CARTESIAN_POINT('Ctrl Pts',(-9.84534649879981,-16.7454750069123,
-329.146683920128)) ;
#29449=CARTESIAN_POINT('Ctrl Pts',(-10.0448274114636,-16.6267277810303,
-329.149536571307)) ;
#29450=CARTESIAN_POINT('Ctrl Pts',(-10.152915411835,-16.5609463231864,-329.151083340673)) ;
#29451=CARTESIAN_POINT('Ctrl Pts',(-10.4189464164537,-16.3954586758336,
-329.154894109615)) ;
#29452=CARTESIAN_POINT('Ctrl Pts',(-10.5761087717045,-16.2945215644385,
-329.157148679774)) ;
#29453=CARTESIAN_POINT('Ctrl Pts',(-11.2217079366288,-15.8666114497986,
-329.166434849004)) ;
#29454=CARTESIAN_POINT('Ctrl Pts',(-11.6966346693122,-15.5198204466108,
-329.173315766768)) ;
#29455=CARTESIAN_POINT('Ctrl Pts',(-12.4536934339356,-14.9125006154747,
-329.184651691979)) ;
#29456=CARTESIAN_POINT('Ctrl Pts',(-12.7451357523674,-14.6641968302286,
-329.189116228882)) ;
#29457=CARTESIAN_POINT('Ctrl Pts',(-13.1408028699748,-14.3063841291079,
-329.195427485265)) ;
#29458=CARTESIAN_POINT('Ctrl Pts',(-13.2513756455363,-14.2040265532576,
-329.197220005716)) ;
#29459=CARTESIAN_POINT('Ctrl Pts',(-13.3642585895728,-14.097064969841,-329.19908573432)) ;
#29460=CARTESIAN_POINT('Ctrl Pts',(-13.3677696945875,-14.0937355518455,
-329.199143802005)) ;
#29461=CARTESIAN_POINT('Ctrl Pts',(-13.3737856463479,-14.0880266333443,
-329.199243357919)) ;
#29462=CARTESIAN_POINT('Ctrl Pts',(-13.3762911025314,-14.0856477762512,
-329.199284838399)) ;
#29463=CARTESIAN_POINT('Ctrl Pts',(-13.3838704089354,-14.0784476014184,
-329.19941037819)) ;
#29464=CARTESIAN_POINT('Ctrl Pts',(-13.3889422878783,-14.0736242098798,
-329.199494462675)) ;
#29465=CARTESIAN_POINT('Ctrl Pts',(-13.3984984242318,-14.0645264177258,
-329.199653035017)) ;
#29466=CARTESIAN_POINT('Ctrl Pts',(-13.4029832460212,-14.0602526110279,
-329.199727515537)) ;
#29467=CARTESIAN_POINT('Ctrl Pts',(-13.4114343038745,-14.0521914656687,
-329.199867979011)) ;
#29468=CARTESIAN_POINT('Ctrl Pts',(-13.4154009821426,-14.048404591386,-329.199933956143)) ;
#29469=CARTESIAN_POINT('Ctrl Pts',(-13.4228770996811,-14.0412613019108,
-329.200058395737)) ;
#29470=CARTESIAN_POINT('Ctrl Pts',(-13.4263868850787,-14.0379052494973,
-329.200116853592)) ;
#29471=CARTESIAN_POINT('Ctrl Pts',(-13.4330035202074,-14.0315736798233,
-329.200227129547)) ;
#29472=CARTESIAN_POINT('Ctrl Pts',(-13.4361106407303,-14.0285984458985,
-329.200278944008)) ;
#29473=CARTESIAN_POINT('Ctrl Pts',(-13.4419698702036,-14.0229841883633,
-329.200376709096)) ;
#29474=CARTESIAN_POINT('Ctrl Pts',(-13.4447221910157,-14.0203453860793,
-329.200422656852)) ;
#29475=CARTESIAN_POINT('Ctrl Pts',(-13.4499140189637,-14.0153647586434,
-329.200509374685)) ;
#29476=CARTESIAN_POINT('Ctrl Pts',(-13.452353691896,-14.0130231065059,-329.200550142497)) ;
#29477=CARTESIAN_POINT('Ctrl Pts',(-13.4569573188365,-14.008602133164,-329.200627105909)) ;
#29478=CARTESIAN_POINT('Ctrl Pts',(-13.4591214026975,-14.0065229473171,
-329.200663299723)) ;
#29479=CARTESIAN_POINT('Ctrl Pts',(-13.4632064246332,-14.0025963617682,
-329.200731648588)) ;
#29480=CARTESIAN_POINT('Ctrl Pts',(-13.4651274645359,-14.0007490680566,
-329.20076380223)) ;
#29481=CARTESIAN_POINT('Ctrl Pts',(-13.4687549837879,-13.9972593673283,
-329.200824540279)) ;
#29482=CARTESIAN_POINT('Ctrl Pts',(-13.4704615430534,-13.9956170434423,
-329.200853123576)) ;
#29483=CARTESIAN_POINT('Ctrl Pts',(-13.4736851815328,-13.9925136078305,
-329.200907133981)) ;
#29484=CARTESIAN_POINT('Ctrl Pts',(-13.4752023235606,-13.9910525613866,
-329.200932560213)) ;
#29485=CARTESIAN_POINT('Ctrl Pts',(-13.4780691361253,-13.9882908489626,
-329.200980619797)) ;
#29486=CARTESIAN_POINT('Ctrl Pts',(-13.4794188561093,-13.986990234318,-329.201003252456)) ;
#29487=CARTESIAN_POINT('Ctrl Pts',(-13.4819701456136,-13.9845310532327,
-329.201046044502)) ;
#29488=CARTESIAN_POINT('Ctrl Pts',(-13.4831717541051,-13.983372527232,-329.201066203341)) ;
#29489=CARTESIAN_POINT('Ctrl Pts',(-13.4854437931989,-13.9811813847254,
-329.201104329031)) ;
#29490=CARTESIAN_POINT('Ctrl Pts',(-13.4865142545722,-13.9801488001144,
-329.201122295448)) ;
#29491=CARTESIAN_POINT('Ctrl Pts',(-13.4885389211562,-13.9781953245404,
-329.201156284003)) ;
#29492=CARTESIAN_POINT('Ctrl Pts',(-13.4894931506702,-13.9772744587981,
-329.201172305796)) ;
#29493=CARTESIAN_POINT('Ctrl Pts',(-13.4912984845053,-13.9755318897551,
-329.201202623409)) ;
#29494=CARTESIAN_POINT('Ctrl Pts',(-13.4921496081091,-13.9747102063683,
-329.201216918956)) ;
#29495=CARTESIAN_POINT('Ctrl Pts',(-13.4937602971788,-13.9731549464448,
-329.201243976639)) ;
#29496=CARTESIAN_POINT('Ctrl Pts',(-13.4945198778563,-13.972421385759,-329.201256738557)) ;
#29497=CARTESIAN_POINT('Ctrl Pts',(-13.4959576813893,-13.9710326086315,
-329.201280898995)) ;
#29498=CARTESIAN_POINT('Ctrl Pts',(-13.4966359163656,-13.9703774047219,
-329.201292297343)) ;
#29499=CARTESIAN_POINT('Ctrl Pts',(-13.497920033498,-13.9691367120228,-329.201313880893)) ;
#29500=CARTESIAN_POINT('Ctrl Pts',(-13.498525925335,-13.9685512331433,-329.201324065959)) ;
#29501=CARTESIAN_POINT('Ctrl Pts',(-13.500890695743,-13.966265836113,-329.201363822469)) ;
#29502=CARTESIAN_POINT('Ctrl Pts',(-13.5026492912326,-13.9645656252299,
-329.20139339796)) ;
#29503=CARTESIAN_POINT('Ctrl Pts',(-13.5060934635385,-13.9612345390759,
-329.201451340562)) ;
#29504=CARTESIAN_POINT('Ctrl Pts',(-13.5077790662557,-13.9596036905833,
-329.201479707301)) ;
#29505=CARTESIAN_POINT('Ctrl Pts',(-13.5580221773944,-13.9109750292108,
-329.20232551594)) ;
#29506=CARTESIAN_POINT('Ctrl Pts',(-13.6063343725602,-13.8637244835447,
-329.203146486416)) ;
#29507=CARTESIAN_POINT('Ctrl Pts',(-13.6885866029149,-13.7824356404178,
-329.204558331305)) ;
#29508=CARTESIAN_POINT('Ctrl Pts',(-13.7226486895035,-13.7485216772645,
-329.205147200894)) ;
#29509=CARTESIAN_POINT('Ctrl Pts',(-13.8007238732929,-13.6702068058699,
-329.206507137861)) ;
#29510=CARTESIAN_POINT('Ctrl Pts',(-13.8446491755584,-13.6257191640261,
-329.207279720744)) ;
#29511=CARTESIAN_POINT('Ctrl Pts',(-13.9691498612876,-13.4984010264772,
-329.209489832114)) ;
#29512=CARTESIAN_POINT('Ctrl Pts',(-14.049201894453,-13.4150625861286,-329.210935386781)) ;
#29513=CARTESIAN_POINT('Ctrl Pts',(-14.4970275654825,-12.9404470026636,
-329.219148791015)) ;
#29514=CARTESIAN_POINT('Ctrl Pts',(-14.8491956150212,-12.5347662675792,
-329.226090168281)) ;
#29515=CARTESIAN_POINT('Ctrl Pts',(-15.5710466732553,-11.6300494945189,
-329.241021774506)) ;
#29516=CARTESIAN_POINT('Ctrl Pts',(-15.9345359981257,-11.1268195428766,
-329.248994545562)) ;
#29517=CARTESIAN_POINT('Ctrl Pts',(-16.3690329904371,-10.4602154831915,
-329.258984022886)) ;
#29518=CARTESIAN_POINT('Ctrl Pts',(-16.4627545307046,-10.3120833194354,
-329.261170458734)) ;
#29519=CARTESIAN_POINT('Ctrl Pts',(-16.6204567244288,-10.0551955165625,
-329.264904530834)) ;
#29520=CARTESIAN_POINT('Ctrl Pts',(-16.6854062078596,-9.94704771943078,
-329.266459365622)) ;
#29521=CARTESIAN_POINT('Ctrl Pts',(-16.818041072939,-9.72124178614683,-329.26967075392)) ;
#29522=CARTESIAN_POINT('Ctrl Pts',(-16.8855560032346,-9.603491339979,-329.271325972388)) ;
#29523=CARTESIAN_POINT('Ctrl Pts',(-17.0645445670757,-9.28359990869937,
-329.275772317734)) ;
#29524=CARTESIAN_POINT('Ctrl Pts',(-17.1736582386741,-9.08016362778839,
-329.278546186021)) ;
#29525=CARTESIAN_POINT('Ctrl Pts',(-17.6401858251183,-8.17184363294039,
-329.290721113284)) ;
#29526=CARTESIAN_POINT('Ctrl Pts',(-17.9580128596447,-7.44747975160154,
-329.299846525682)) ;
#29527=CARTESIAN_POINT('Ctrl Pts',(-18.3013067436693,-6.51417484900391,
-329.31153587164)) ;
#29528=CARTESIAN_POINT('Ctrl Pts',(-18.3687573969846,-6.32147561813183,
-329.313948008058)) ;
#29529=CARTESIAN_POINT('Ctrl Pts',(-18.4789553415451,-5.98998423307379,
-329.318117787057)) ;
#29530=CARTESIAN_POINT('Ctrl Pts',(-18.5232067821707,-5.85171017963855,
-329.319863117471)) ;
#29531=CARTESIAN_POINT('Ctrl Pts',(-18.5879842264298,-5.64119702708577,
-329.322537304368)) ;
#29532=CARTESIAN_POINT('Ctrl Pts',(-18.6096482943204,-5.56931340865173,
-329.323453454193)) ;
#29533=CARTESIAN_POINT('Ctrl Pts',(-18.6498895712344,-5.43293187960375,
-329.325198746452)) ;
#29534=CARTESIAN_POINT('Ctrl Pts',(-18.668550258484,-5.36845983848395,-329.326026921109)) ;
#29535=CARTESIAN_POINT('Ctrl Pts',(-18.7161239010457,-5.20084656551007,
-329.328187029729)) ;
#29536=CARTESIAN_POINT('Ctrl Pts',(-18.744518528706,-5.09756058883894,-329.329524952954)) ;
#29537=CARTESIAN_POINT('Ctrl Pts',(-18.9340199637367,-4.38524588410929,
-329.33878630526)) ;
#29538=CARTESIAN_POINT('Ctrl Pts',(-19.0662705213906,-3.76892839954168,
-329.346958674151)) ;
#29539=CARTESIAN_POINT('Ctrl Pts',(-19.2517110642867,-2.63951186555944,
-329.361711786254)) ;
#29540=CARTESIAN_POINT('Ctrl Pts',(-19.3148732133948,-2.12863270367683,
-329.368306573883)) ;
#29541=CARTESIAN_POINT('Ctrl Pts',(-19.3733345527792,-1.4282728158781,-329.377147957782)) ;
#29542=CARTESIAN_POINT('Ctrl Pts',(-19.3862649088912,-1.24047892788992,
-329.379499989339)) ;
#29543=CARTESIAN_POINT('Ctrl Pts',(-19.40340911906,-0.92453722504556,-329.383424571532)) ;
#29544=CARTESIAN_POINT('Ctrl Pts',(-19.409087325017,-0.796482129985812,
-329.385006341726)) ;
#29545=CARTESIAN_POINT('Ctrl Pts',(-19.4180377512594,-0.536511686249656,
-329.388199869549)) ;
#29546=CARTESIAN_POINT('Ctrl Pts',(-19.4212340889775,-0.404600315161816,
-329.38981105662)) ;
#29547=CARTESIAN_POINT('Ctrl Pts',(-19.4260311445044,-0.062887590516012,
-329.393962301736)) ;
#29548=CARTESIAN_POINT('Ctrl Pts',(-19.4255773139515,0.146925479434508,
-329.396489122477)) ;
#29549=CARTESIAN_POINT('Ctrl Pts',(-19.4162509773394,0.654743038639132,
-329.402561257111)) ;
#29550=CARTESIAN_POINT('Ctrl Pts',(-19.4039167620585,0.952630647513047,
-329.406086443771)) ;
#29551=CARTESIAN_POINT('Ctrl Pts',(-19.3479290612677,1.82079502743547,-329.416309169884)) ;
#29552=CARTESIAN_POINT('Ctrl Pts',(-19.2859433831771,2.38956892535373,-329.422935304786)) ;
#29553=CARTESIAN_POINT('Ctrl Pts',(-19.1789344061941,3.08487037432564,-329.431223676442)) ;
#29554=CARTESIAN_POINT('Ctrl Pts',(-19.1575908769915,3.21475689959559,-329.432780617861)) ;
#29555=CARTESIAN_POINT('Ctrl Pts',(-19.1064198175111,3.50752983442487,-329.436317591298)) ;
#29556=CARTESIAN_POINT('Ctrl Pts',(-19.0758262616216,3.67027193388655,-329.438302974392)) ;
#29557=CARTESIAN_POINT('Ctrl Pts',(-19.0276262464499,3.90976464252415,-329.441264587557)) ;
#29558=CARTESIAN_POINT('Ctrl Pts',(-19.0116278932979,3.98683144371374,-329.442223747549)) ;
#29559=CARTESIAN_POINT('Ctrl Pts',(-18.9812286249278,4.12892485006904,-329.444005185271)) ;
#29560=CARTESIAN_POINT('Ctrl Pts',(-18.966960855422,4.19397858870562,-329.444825952714)) ;
#29561=CARTESIAN_POINT('Ctrl Pts',(-18.9305629948807,4.35594904608031,-329.446881738122)) ;
#29562=CARTESIAN_POINT('Ctrl Pts',(-18.9080229550369,4.45277164114303,-329.448121472296)) ;
#29563=CARTESIAN_POINT('Ctrl Pts',(-18.8054594578311,4.87851523013988,-329.453614078224)) ;
#29564=CARTESIAN_POINT('Ctrl Pts',(-18.7175892256608,5.20548451773665,-329.45794031994)) ;
#29565=CARTESIAN_POINT('Ctrl Pts',(-18.4297523065071,6.17472227755628,-329.470940152228)) ;
#29566=CARTESIAN_POINT('Ctrl Pts',(-18.2049283834514,6.809078681661,-329.479667819195)) ;
#29567=CARTESIAN_POINT('Ctrl Pts',(-17.8442157184515,7.68034614028408,-329.491646923635)) ;
#29568=CARTESIAN_POINT('Ctrl Pts',(-17.7355682358456,7.92801180864771,-329.495053692921)) ;
#29569=CARTESIAN_POINT('Ctrl Pts',(-17.5617977989332,8.30266275922816,-329.500203035459)) ;
#29570=CARTESIAN_POINT('Ctrl Pts',(-17.5003880386997,8.43133259866922,-329.501970857903)) ;
#29571=CARTESIAN_POINT('Ctrl Pts',(-17.3827437547907,8.67100483424224,-329.505262622015)) ;
#29572=CARTESIAN_POINT('Ctrl Pts',(-17.3268483205266,8.78216559878099,-329.506788892475)) ;
#29573=CARTESIAN_POINT('Ctrl Pts',(-17.1974887996662,9.0333833386592,-329.510237900127)) ;
#29574=CARTESIAN_POINT('Ctrl Pts',(-17.1233744423508,9.17309562559524,-329.51215580403)) ;
#29575=CARTESIAN_POINT('Ctrl Pts',(-16.8696308244936,9.637631968042,-329.518536451193)) ;
#29576=CARTESIAN_POINT('Ctrl Pts',(-16.6823992933428,9.95821011869755,-329.522944439844)) ;
#29577=CARTESIAN_POINT('Ctrl Pts',(-16.4734472567714,10.2935286792378,-329.527595103698)) ;
#29578=CARTESIAN_POINT('Ctrl Pts',(-16.4607590036743,10.3138067761155,-329.527876514739)) ;
#29579=CARTESIAN_POINT('Ctrl Pts',(-16.1374153711969,10.8284511781678,-329.535023065582)) ;
#29580=CARTESIAN_POINT('Ctrl Pts',(-15.8046657047995,11.3085839077288,-329.541786412174)) ;
#29581=CARTESIAN_POINT('Ctrl Pts',(-15.3702417526816,11.878718769304,-329.550229940245)) ;
#29582=CARTESIAN_POINT('Ctrl Pts',(-15.2886030453137,11.9836099739594,-329.551801842031)) ;
#29583=CARTESIAN_POINT('Ctrl Pts',(-15.102183644944,12.2181197873783,-329.555366457079)) ;
#29584=CARTESIAN_POINT('Ctrl Pts',(-14.9967983046114,12.3472443258574,-329.557364503377)) ;
#29585=CARTESIAN_POINT('Ctrl Pts',(-14.8390991464197,12.5354690955653,-329.56034118974)) ;
#29586=CARTESIAN_POINT('Ctrl Pts',(-14.7880658507319,12.5956324691032,-329.56130251395)) ;
#29587=CARTESIAN_POINT('Ctrl Pts',(-14.693307992945,12.7059731822496,-329.563085520106)) ;
#29588=CARTESIAN_POINT('Ctrl Pts',(-14.6496894294661,12.7562398013074,-329.563905660478)) ;
#29589=CARTESIAN_POINT('Ctrl Pts',(-14.5405082472926,12.880763068274,-329.565956375087)) ;
#29590=CARTESIAN_POINT('Ctrl Pts',(-14.4746343527734,12.9547442130536,-329.567191611471)) ;
#29591=CARTESIAN_POINT('Ctrl Pts',(-14.1853759424155,13.2746415514943,-329.57260045997)) ;
#29592=CARTESIAN_POINT('Ctrl Pts',(-13.9562694592616,13.5153076536035,-329.576844703964)) ;
#29593=CARTESIAN_POINT('Ctrl Pts',(-13.6019245600803,13.8689084406734,-329.583279392369)) ;
#29594=CARTESIAN_POINT('Ctrl Pts',(-13.4812035339259,13.9862834348667,-329.585450276993)) ;
#29595=CARTESIAN_POINT('Ctrl Pts',(-13.0225004063363,14.4208154165743,-329.593601396861)) ;
#29596=CARTESIAN_POINT('Ctrl Pts',(-12.6747284697147,14.7274129991098,-329.599582958634)) ;
#29597=CARTESIAN_POINT('Ctrl Pts',(-12.2050356319801,15.1125259804316,-329.607319964546)) ;
#29598=CARTESIAN_POINT('Ctrl Pts',(-12.0927366806281,15.2025345228885,-329.609145797043)) ;
#29599=CARTESIAN_POINT('Ctrl Pts',(-11.8105346642878,15.4236162641598,-329.613672176451)) ;
#29600=CARTESIAN_POINT('Ctrl Pts',(-11.6394402857428,15.5531378758439,-329.61636161435)) ;
#29601=CARTESIAN_POINT('Ctrl Pts',(-11.3590349398232,15.758191124415,-329.620679426373)) ;
#29602=CARTESIAN_POINT('Ctrl Pts',(-11.2510336382605,15.8354824494095,-329.622321519226)) ;
#29603=CARTESIAN_POINT('Ctrl Pts',(-11.0389115975896,15.9840223492637,-329.625506410988)) ;
#29604=CARTESIAN_POINT('Ctrl Pts',(-10.9348725019958,16.0553761442925,-329.627049990396)) ;
#29605=CARTESIAN_POINT('Ctrl Pts',(-10.7023652046694,16.2115297441868,-329.630459720165)) ;
#29606=CARTESIAN_POINT('Ctrl Pts',(-10.5735691368235,16.2958262574358,-329.632321941622)) ;
#29607=CARTESIAN_POINT('Ctrl Pts',(-9.97721786341936,16.6760889606876,-329.64082948912)) ;
#29608=CARTESIAN_POINT('Ctrl Pts',(-9.49815124838969,16.9535230515074,-329.647335031457)) ;
#29609=CARTESIAN_POINT('Ctrl Pts',(-8.54061355179574,17.4547046982999,-329.659969082736)) ;
#29610=CARTESIAN_POINT('Ctrl Pts',(-8.06356561379674,17.6801499752187,-329.666097009389)) ;
#29611=CARTESIAN_POINT('Ctrl Pts',(-7.42263720389651,17.9516999052366,-329.674377280215)) ;
#29612=CARTESIAN_POINT('Ctrl Pts',(-7.26648673273136,18.0154723211392,-329.676398810078)) ;
#29613=CARTESIAN_POINT('Ctrl Pts',(-7.03579486704565,18.106200393726,-329.679403425369)) ;
#29614=CARTESIAN_POINT('Ctrl Pts',(-6.96188722351389,18.1347464381203,-329.680368735014)) ;
#29615=CARTESIAN_POINT('Ctrl Pts',(-6.82565549421285,18.1864089476938,-329.682154680872)) ;
#29616=CARTESIAN_POINT('Ctrl Pts',(-6.7633835539294,18.2096591458001,-329.682973718172)) ;
#29617=CARTESIAN_POINT('Ctrl Pts',(-6.60861307331499,18.2665416859719,-329.685015339672)) ;
#29618=CARTESIAN_POINT('Ctrl Pts',(-6.51597598391044,18.2997914976492,-329.686242488885)) ;
#29619=CARTESIAN_POINT('Ctrl Pts',(-6.12823723989252,18.4356433059545,-329.691394268673)) ;
#29620=CARTESIAN_POINT('Ctrl Pts',(-5.8309351381501,18.531822104761,-329.695380968365)) ;
#29621=CARTESIAN_POINT('Ctrl Pts',(-5.34904594947418,18.6749708733267,-329.70183735162)) ;
#29622=CARTESIAN_POINT('Ctrl Pts',(-5.16586200375946,18.7264705537524,-329.704290569241)) ;
#29623=CARTESIAN_POINT('Ctrl Pts',(-4.53445142570174,18.8940131010588,-329.712718020036)) ;
#29624=CARTESIAN_POINT('Ctrl Pts',(-4.08284870326067,18.9967188896844,-329.718693126352)) ;
#29625=CARTESIAN_POINT('Ctrl Pts',(-3.4867131694502,19.1100534330141,-329.726422667093)) ;
#29626=CARTESIAN_POINT('Ctrl Pts',(-3.34512383873779,19.1353457638368,-329.728247357277)) ;
#29627=CARTESIAN_POINT('Ctrl Pts',(-2.99171757097076,19.1944329162501,-329.732771433222)) ;
#29628=CARTESIAN_POINT('Ctrl Pts',(-2.77959701936612,19.2262963058545,-329.735459714409)) ;
#29629=CARTESIAN_POINT('Ctrl Pts',(-2.43536753442395,19.2721883275814,-329.739776175621)) ;
#29630=CARTESIAN_POINT('Ctrl Pts',(-2.30356638045084,19.288386141651,-329.741418057993)) ;
#29631=CARTESIAN_POINT('Ctrl Pts',(-2.04623715102699,19.3173356252656,-329.744602851125)) ;
#29632=CARTESIAN_POINT('Ctrl Pts',(-1.92073036912962,19.3302182355755,-329.74614653903)) ;
#29633=CARTESIAN_POINT('Ctrl Pts',(-1.64179812927608,19.3561057533673,-329.749556895494)) ;
#29634=CARTESIAN_POINT('Ctrl Pts',(-1.48832548328144,19.3685110003754,-329.751419629746)) ;
#29635=CARTESIAN_POINT('Ctrl Pts',(-0.782618687420034,19.4171160687365,
-329.759928377173)) ;
#29636=CARTESIAN_POINT('Ctrl Pts',(-0.229142436903726,19.4315306616868,
-329.76643458717)) ;
#29637=CARTESIAN_POINT('Ctrl Pts',(0.852082647786337,19.4134830869873,-329.779075691845)) ;
#29638=CARTESIAN_POINT('Ctrl Pts',(1.37939265059248,19.3831536112505,-329.785209916209)) ;
#29639=CARTESIAN_POINT('Ctrl Pts',(2.07217604052569,19.3148905002749,-329.7934914149)) ;
#29640=CARTESIAN_POINT('Ctrl Pts',(2.2393213137948,19.2962262755618,-329.795507228865)) ;
#29641=CARTESIAN_POINT('Ctrl Pts',(2.48473988405587,19.2655899701118,-329.798505049115)) ;
#29642=CARTESIAN_POINT('Ctrl Pts',(2.56321622626901,19.2553060672706,-329.799469392061)) ;
#29643=CARTESIAN_POINT('Ctrl Pts',(2.70749982302108,19.2355007898599,-329.801254618865)) ;
#29644=CARTESIAN_POINT('Ctrl Pts',(2.77332511123636,19.2261206102772,-329.802073917687)) ;
#29645=CARTESIAN_POINT('Ctrl Pts',(2.93661672440895,19.2019953161281,-329.804117716235)) ;
#29646=CARTESIAN_POINT('Ctrl Pts',(3.03402137604771,19.1868459148034,-329.805346804255)) ;
#29647=CARTESIAN_POINT('Ctrl Pts',(3.44139029456022,19.1203079232232,-329.810522829321)) ;
#29648=CARTESIAN_POINT('Ctrl Pts',(3.75019931043715,19.0621443362934,-329.814532537657)) ;
#29649=CARTESIAN_POINT('Ctrl Pts',(4.24142142460484,18.9572243412917,-329.820984351117)) ;
#29650=CARTESIAN_POINT('Ctrl Pts',(4.42480165834261,18.9152621093813,-329.823409664787)) ;
#29651=CARTESIAN_POINT('Ctrl Pts',(5.05736211567749,18.7608132273843,-329.831809789347)) ;
#29652=CARTESIAN_POINT('Ctrl Pts',(5.50311082982857,18.6349348544389,-329.837785518647)) ;
#29653=CARTESIAN_POINT('Ctrl Pts',(6.08087035233225,18.4492365463619,-329.845515779874)) ;
#29654=CARTESIAN_POINT('Ctrl Pts',(6.21731269528264,18.4037044176976,-329.847340580353)) ;
#29655=CARTESIAN_POINT('Ctrl Pts',(6.55593420055569,18.2865075806495,-329.85186487872)) ;
#29656=CARTESIAN_POINT('Ctrl Pts',(6.75745590092216,18.2130014746607,-329.854553271605)) ;
#29657=CARTESIAN_POINT('Ctrl Pts',(7.08169931576495,18.0886094871706,-329.85886986326)) ;
#29658=CARTESIAN_POINT('Ctrl Pts',(7.20518863757643,18.0397759169091,-329.860511765958)) ;
#29659=CARTESIAN_POINT('Ctrl Pts',(7.44500765626171,17.9420846866245,-329.863696568602)) ;
#29660=CARTESIAN_POINT('Ctrl Pts',(7.56138131868501,17.8933522433812,-329.865240246017)) ;
#29661=CARTESIAN_POINT('Ctrl Pts',(7.81870035685193,17.7826391310795,-329.86865054191)) ;
#29662=CARTESIAN_POINT('Ctrl Pts',(7.95940031105361,17.7201093819379,-329.870513226602)) ;
#29663=CARTESIAN_POINT('Ctrl Pts',(8.60234784879894,17.4251684223834,-329.879021872229)) ;
#29664=CARTESIAN_POINT('Ctrl Pts',(9.09526374345616,17.1730329928343,-329.885528031184)) ;
#29665=CARTESIAN_POINT('Ctrl Pts',(10.0360385137874,16.6399293712994,-329.898168508318)) ;
#29666=CARTESIAN_POINT('Ctrl Pts',(10.4845341954365,16.3610469968299,-329.904302164253)) ;
#29667=CARTESIAN_POINT('Ctrl Pts',(10.9883381970162,16.0185410370371,-329.911549411892)) ;
#29668=CARTESIAN_POINT('Ctrl Pts',(11.0552776022657,15.9724159227267,-329.912520029171)) ;
#29669=CARTESIAN_POINT('Ctrl Pts',(11.2190410091295,15.8580507939716,-329.914915749324)) ;
#29670=CARTESIAN_POINT('Ctrl Pts',(11.3155340792936,15.7893427535045,-329.916345719318)) ;
#29671=CARTESIAN_POINT('Ctrl Pts',(11.4679435376613,15.6787046432279,-329.918638322728)) ;
#29672=CARTESIAN_POINT('Ctrl Pts',(11.5242725878605,15.6373479077846,-329.919493140801)) ;
#29673=CARTESIAN_POINT('Ctrl Pts',(11.6308543099371,15.5582070236111,-329.921126028849)) ;
#29674=CARTESIAN_POINT('Ctrl Pts',(11.6811490893172,15.5204811043532,-329.921903147994)) ;
#29675=CARTESIAN_POINT('Ctrl Pts',(11.8249685551808,15.411507602585,-329.924143179281)) ;
#29676=CARTESIAN_POINT('Ctrl Pts',(11.9180306606808,15.3396542668313,-329.925614450232)) ;
#29677=CARTESIAN_POINT('Ctrl Pts',(12.530944631856,14.8574781905786,-329.935434095091)) ;
#29678=CARTESIAN_POINT('Ctrl Pts',(13.0301727123745,14.4216445271644,-329.944041450593)) ;
#29679=CARTESIAN_POINT('Ctrl Pts',(13.7527387155712,13.7226274193422,-329.956986459446)) ;
#29680=CARTESIAN_POINT('Ctrl Pts',(13.9929517170713,13.4775972776863,-329.961383478991)) ;
#29681=CARTESIAN_POINT('Ctrl Pts',(14.3980848492097,13.0418267506142,-329.968928244738)) ;
#29682=CARTESIAN_POINT('Ctrl Pts',(14.5660147501345,12.8539996491689,-329.972097133833)) ;
#29683=CARTESIAN_POINT('Ctrl Pts',(14.8211459938935,12.5572170883597,-329.976972598279)) ;
#29684=CARTESIAN_POINT('Ctrl Pts',(14.9109068062645,12.4504991007317,-329.978700289798)) ;
#29685=CARTESIAN_POINT('Ctrl Pts',(15.0789347481953,12.2463045845789,-329.98195841114)) ;
#29686=CARTESIAN_POINT('Ctrl Pts',(15.1574252350588,12.1490209239088,-329.983490662288)) ;
#29687=CARTESIAN_POINT('Ctrl Pts',(15.3364476016038,11.9226991496856,-329.987010323259)) ;
#29688=CARTESIAN_POINT('Ctrl Pts',(15.4362995158311,11.7931351814819,-329.988992106712)) ;
#29689=CARTESIAN_POINT('Ctrl Pts',(15.7877770424613,11.3249585053423,-329.996041309069)) ;
#29690=CARTESIAN_POINT('Ctrl Pts',(16.0299939242519,10.979430084686,-330.00103525652)) ;
#29691=CARTESIAN_POINT('Ctrl Pts',(16.5620966495462,10.1651854458793,-330.012452887739)) ;
#29692=CARTESIAN_POINT('Ctrl Pts',(16.8436746087177,9.69147381567583,-330.018838674233)) ;
#29693=CARTESIAN_POINT('Ctrl Pts',(17.1660121301032,9.09259953020383,-330.026854255297)) ;
#29694=CARTESIAN_POINT('Ctrl Pts',(17.2261467234629,8.97815168514524,-330.028383985516)) ;
#29695=CARTESIAN_POINT('Ctrl Pts',(17.3597854876978,8.71752495064118,-330.031870509975)) ;
#29696=CARTESIAN_POINT('Ctrl Pts',(17.432594262541,8.5710005586371,-330.033832684312)) ;
#29697=CARTESIAN_POINT('Ctrl Pts',(17.5375289033438,8.35295439600053,-330.036766648313)) ;
#29698=CARTESIAN_POINT('Ctrl Pts',(17.5710869078076,8.28212967992373,-330.037721814283)) ;
#29699=CARTESIAN_POINT('Ctrl Pts',(17.6324060024832,8.15066446374064,-330.039500411068)) ;
#29700=CARTESIAN_POINT('Ctrl Pts',(17.6602851247482,8.09008046395288,-330.040322389622)) ;
#29701=CARTESIAN_POINT('Ctrl Pts',(17.7292190593585,7.93822600730525,-330.042387788954)) ;
#29702=CARTESIAN_POINT('Ctrl Pts',(17.7698815436645,7.84677962494043,-330.043636028261)) ;
#29703=CARTESIAN_POINT('Ctrl Pts',(17.9587281726829,7.41308299936894,-330.049569896015)) ;
#29704=CARTESIAN_POINT('Ctrl Pts',(18.0977421370436,7.0669261867291,-330.054345337509)) ;
#29705=CARTESIAN_POINT('Ctrl Pts',(18.3726347461828,6.32099814188781,-330.064578500043)) ;
#29706=CARTESIAN_POINT('Ctrl Pts',(18.5056218614875,5.92036189891185,-330.070039834706)) ;
#29707=CARTESIAN_POINT('Ctrl Pts',(18.7078947623865,5.23732697135032,-330.079184498698)) ;
#29708=CARTESIAN_POINT('Ctrl Pts',(18.7840839296965,4.95712735499223,-330.082890437858)) ;
#29709=CARTESIAN_POINT('Ctrl Pts',(18.9082752036702,4.45630704415951,-330.089414286316)) ;
#29710=CARTESIAN_POINT('Ctrl Pts',(18.9587659637942,4.23635893725976,-330.092245753194)) ;
#29711=CARTESIAN_POINT('Ctrl Pts',(19.0332794884967,3.88369256885976,-330.096729320622)) ;
#29712=CARTESIAN_POINT('Ctrl Pts',(19.059772072674,3.75151764677148,-330.098397204061)) ;
#29713=CARTESIAN_POINT('Ctrl Pts',(19.108463893334,3.4947456211699,-330.101613405512)) ;
#29714=CARTESIAN_POINT('Ctrl Pts',(19.1308255109528,3.37018614293166,-330.10316271848)) ;
#29715=CARTESIAN_POINT('Ctrl Pts',(19.1817059851789,3.06992850458334,-330.106872330538)) ;
#29716=CARTESIAN_POINT('Ctrl Pts',(19.2090302010524,2.89403945852976,-330.109024756651)) ;
#29717=CARTESIAN_POINT('Ctrl Pts',(19.3370075946335,1.98834035795882,-330.120013319429)) ;
#29718=CARTESIAN_POINT('Ctrl Pts',(19.3985007088822,1.25360707187879,-330.128586401666)) ;
#29719=CARTESIAN_POINT('Ctrl Pts',(19.4289544576065,0.110147357720164,-330.141957838631)) ;
#29720=CARTESIAN_POINT('Ctrl Pts',(19.4269948692778,-0.297107080162094,
-330.146731886919)) ;
#29721=CARTESIAN_POINT('Ctrl Pts',(19.4079079471966,-0.823415874174811,
-330.153047216981)) ;
#29722=CARTESIAN_POINT('Ctrl Pts',(19.4024753011762,-0.9427919776234,-330.154489529161)) ;
#29723=CARTESIAN_POINT('Ctrl Pts',(19.3921094443329,-1.13209018345098,-330.1567970516)) ;
#29724=CARTESIAN_POINT('Ctrl Pts',(19.3878986820907,-1.20204890547807,-330.157654271325)) ;
#29725=CARTESIAN_POINT('Ctrl Pts',(19.3792037612119,-1.33454777108671,-330.159287389927)) ;
#29726=CARTESIAN_POINT('Ctrl Pts',(19.3747952291614,-1.39709197583418,-330.160062297965)) ;
#29727=CARTESIAN_POINT('Ctrl Pts',(19.361323142618,-1.57587588909988,-330.162287785291)) ;
#29728=CARTESIAN_POINT('Ctrl Pts',(19.3515157696895,-1.69205673864896,-330.163746561227)) ;
#29729=CARTESIAN_POINT('Ctrl Pts',(19.3074242499004,-2.1636785377513,-330.169709887209)) ;
#29730=CARTESIAN_POINT('Ctrl Pts',(19.2643881515232,-2.51823040209902,-330.174287874772)) ;
#29731=CARTESIAN_POINT('Ctrl Pts',(19.1321730462123,-3.40284075193063,-330.185806709429)) ;
#29732=CARTESIAN_POINT('Ctrl Pts',(19.0307241587448,-3.93076461554458,-330.192764279617)) ;
#29733=CARTESIAN_POINT('Ctrl Pts',(18.8717201503551,-4.60577697688609,-330.201614460744)) ;
#29734=CARTESIAN_POINT('Ctrl Pts',(18.8340902751248,-4.75731505957141,-330.203598861156)) ;
#29735=CARTESIAN_POINT('Ctrl Pts',(18.737317073765,-5.12786829685356,-330.208441729512)) ;
#29736=CARTESIAN_POINT('Ctrl Pts',(18.6761561933707,-5.34633280887128,-330.211288527478)) ;
#29737=CARTESIAN_POINT('Ctrl Pts',(18.5725122925584,-5.69303443887426,-330.215789968112)) ;
#29738=CARTESIAN_POINT('Ctrl Pts',(18.5324939498157,-5.82198609062626,-330.217460622785)) ;
#29739=CARTESIAN_POINT('Ctrl Pts',(18.4523984751142,-6.07088175785231,-330.220678468924)) ;
#29740=CARTESIAN_POINT('Ctrl Pts',(18.4124880041225,-6.19087234153317,-330.222226696371)) ;
#29741=CARTESIAN_POINT('Ctrl Pts',(18.3137968376767,-6.47818806682719,-330.225927486203)) ;
#29742=CARTESIAN_POINT('Ctrl Pts',(18.2538907121145,-6.6451146895395,-330.228072277041)) ;
#29743=CARTESIAN_POINT('Ctrl Pts',(17.9320982838824,-7.50457492864761,-330.239098476883)) ;
#29744=CARTESIAN_POINT('Ctrl Pts',(17.6330591901992,-8.18254346902189,-330.24771337926)) ;
#29745=CARTESIAN_POINT('Ctrl Pts',(17.1115484562098,-9.20270851882717,-330.261107227162)) ;
#29746=CARTESIAN_POINT('Ctrl Pts',(16.9157906619508,-9.55776958613195,-330.265860643072)) ;
#29747=CARTESIAN_POINT('Ctrl Pts',(16.6482306281246,-10.0090595496097,-330.272152113662)) ;
#29748=CARTESIAN_POINT('Ctrl Pts',(16.58644851546,-10.1111117932829,-330.27359202634)) ;
#29749=CARTESIAN_POINT('Ctrl Pts',(16.486904582115,-10.2721715620907,-330.275896646844)) ;
#29750=CARTESIAN_POINT('Ctrl Pts',(16.4497568097972,-10.3315551681954,-330.276753398276)) ;
#29751=CARTESIAN_POINT('Ctrl Pts',(16.3787324048448,-10.4437390382676,-330.278386462983)) ;
#29752=CARTESIAN_POINT('Ctrl Pts',(16.3449196062418,-10.4965786494179,-330.279161793123)) ;
#29753=CARTESIAN_POINT('Ctrl Pts',(16.2474314927806,-10.6473110342797,-330.281390062468)) ;
#29754=CARTESIAN_POINT('Ctrl Pts',(16.1831286178432,-10.7447945746771,-330.282851229269)) ;
#29755=CARTESIAN_POINT('Ctrl Pts',(15.7466166015083,-11.3937411615886,-330.292697711069)) ;
#29756=CARTESIAN_POINT('Ctrl Pts',(15.347165847278,-11.9263478388706,-330.30134540886)) ;
#29757=CARTESIAN_POINT('Ctrl Pts',(14.7020796762253,-12.7002587857508,-330.314317731273)) ;
#29758=CARTESIAN_POINT('Ctrl Pts',(14.476074232971,-12.9572757744647,-330.318703156046)) ;
#29759=CARTESIAN_POINT('Ctrl Pts',(14.0723804993433,-13.3926095285967,-330.326231120311)) ;
#29760=CARTESIAN_POINT('Ctrl Pts',(13.897797527134,-13.5736917292507,-330.329394662299)) ;
#29761=CARTESIAN_POINT('Ctrl Pts',(13.621083254794,-13.8497704134581,-330.334263945175)) ;
#29762=CARTESIAN_POINT('Ctrl Pts',(13.5213625299281,-13.9471432537138,-330.335990712906)) ;
#29763=CARTESIAN_POINT('Ctrl Pts',(13.3302232323978,-14.1298054449018,-330.339248102491)) ;
#29764=CARTESIAN_POINT('Ctrl Pts',(13.2390122540193,-14.2153018934401,-330.340780533645)) ;
#29765=CARTESIAN_POINT('Ctrl Pts',(13.0264656530984,-14.4107119350479,-330.344302045213)) ;
#29766=CARTESIAN_POINT('Ctrl Pts',(12.9045530645632,-14.5199840286034,-330.346285478662)) ;
#29767=CARTESIAN_POINT('Ctrl Pts',(12.450911539559,-14.9163632034542,-330.353539056599)) ;
#29768=CARTESIAN_POINT('Ctrl Pts',(12.1108648617341,-15.1937501258125,-330.358728467319)) ;
#29769=CARTESIAN_POINT('Ctrl Pts',(11.3341713003241,-15.7846695223877,-330.370176712069)) ;
#29770=CARTESIAN_POINT('Ctrl Pts',(10.8933149469342,-16.0920762802304,-330.376406960397)) ;
#29771=CARTESIAN_POINT('Ctrl Pts',(10.3325948795987,-16.449450337789,-330.384245305199)) ;
#29772=CARTESIAN_POINT('Ctrl Pts',(10.2242296705161,-16.5170233686163,-330.385756720922)) ;
#29773=CARTESIAN_POINT('Ctrl Pts',(9.97667259589361,-16.6680220954688,-330.389209164512)) ;
#29774=CARTESIAN_POINT('Ctrl Pts',(9.83708585449466,-16.7507820238262,-330.391155589243)) ;
#29775=CARTESIAN_POINT('Ctrl Pts',(9.62876909556282,-16.8707894540805,-330.394070773089)) ;
#29776=CARTESIAN_POINT('Ctrl Pts',(9.56082467379982,-16.9093868202285,-330.395023208434)) ;
#29777=CARTESIAN_POINT('Ctrl Pts',(9.43440719750226,-16.9801955876855,-330.396799904291)) ;
#29778=CARTESIAN_POINT('Ctrl Pts',(9.37599753475988,-17.0125174961228,-330.397622752435)) ;
#29779=CARTESIAN_POINT('Ctrl Pts',(9.22919724359832,-17.0927660989602,-330.399694922638)) ;
#29780=CARTESIAN_POINT('Ctrl Pts',(9.14059896808375,-17.1403087819225,-330.400949135163)) ;
#29781=CARTESIAN_POINT('Ctrl Pts',(8.72895003226867,-17.3571041041459,-330.406786052973)) ;
#29782=CARTESIAN_POINT('Ctrl Pts',(8.40154287486246,-17.5179253327682,-330.411454153591)) ;
#29783=CARTESIAN_POINT('Ctrl Pts',(7.95537784495177,-17.721693279478,-330.417766639287)) ;
#29784=CARTESIAN_POINT('Ctrl Pts',(7.84044697423284,-17.7728399694747,-330.419388607912)) ;
#29785=CARTESIAN_POINT('Ctrl Pts',(7.29560097256129,-18.0089944781337,-330.427048879598)) ;
#29786=CARTESIAN_POINT('Ctrl Pts',(6.8595871410745,-18.1795418331174,-330.433090521909)) ;
#29787=CARTESIAN_POINT('Ctrl Pts',(6.2812378385883,-18.3819918070808,-330.44089693956)) ;
#29788=CARTESIAN_POINT('Ctrl Pts',(6.14410566080346,-18.4282809092375,-330.44273334278)) ;
#29789=CARTESIAN_POINT('Ctrl Pts',(5.80161605941945,-18.5396407017903,-330.447281021887)) ;
#29790=CARTESIAN_POINT('Ctrl Pts',(5.5956692156963,-18.6028361416602,-330.449981147973)) ;
#29791=CARTESIAN_POINT('Ctrl Pts',(5.26097648977465,-18.6994766922756,-330.454311441326)) ;
#29792=CARTESIAN_POINT('Ctrl Pts',(5.13286383151931,-18.7350476683488,-330.455955479026)) ;
#29793=CARTESIAN_POINT('Ctrl Pts',(4.8825852219394,-18.8017786189703,-330.459141295461)) ;
#29794=CARTESIAN_POINT('Ctrl Pts',(4.76046108048249,-18.8330700640084,-330.460683885563)) ;
#29795=CARTESIAN_POINT('Ctrl Pts',(4.48895598576786,-18.8998272263996,-330.464087882715)) ;
#29796=CARTESIAN_POINT('Ctrl Pts',(4.33944161609734,-18.934715249318,-330.465945410294)) ;
#29797=CARTESIAN_POINT('Ctrl Pts',(3.72773599019687,-19.0698260660903,-330.473481372213)) ;
#29798=CARTESIAN_POINT('Ctrl Pts',(3.2623712842438,-19.1549266967292,-330.479062504468)) ;
#29799=CARTESIAN_POINT('Ctrl Pts',(2.29855048969756,-19.2950334940898,-330.490469943193)) ;
#29800=CARTESIAN_POINT('Ctrl Pts',(1.8001337712822,-19.3478983106631,-330.496286567124)) ;
#29801=CARTESIAN_POINT('Ctrl Pts',(1.12885643116695,-19.3929319654646,-330.504222820823)) ;
#29802=CARTESIAN_POINT('Ctrl Pts',(0.957335222378236,-19.4021554525485,
-330.506260143751)) ;
#29803=CARTESIAN_POINT('Ctrl Pts',(0.657234931424957,-19.4143040385478,
-330.50985544195)) ;
#29804=CARTESIAN_POINT('Ctrl Pts',(0.528707000938554,-19.4182292675448,
-330.511405105086)) ;
#29805=CARTESIAN_POINT('Ctrl Pts',(0.328274487591244,-19.4223589995926,
-330.51384282867)) ;
#29806=CARTESIAN_POINT('Ctrl Pts',(0.25639159959772,-19.4234409047298,-330.514721326051)) ;
#29807=CARTESIAN_POINT('Ctrl Pts',(0.123021396673552,-19.4247077517276,
-330.516360385086)) ;
#29808=CARTESIAN_POINT('Ctrl Pts',(0.0615360145035663,-19.4249998405387,
-330.517119637573)) ;
#29809=CARTESIAN_POINT('Ctrl Pts',(5.03575626769576E-5,-19.4249999999347,
-330.517882160562)) ;
#29810=CARTESIAN_POINT('Origin',(0.,0.,-328.125)) ;
#29811=CARTESIAN_POINT('',(-0.000189941651959998,-19.4249999990714,-332.23026054535)) ;
#29812=CARTESIAN_POINT('',(-0.000307709618470118,-19.4249998857984,-332.019601644739)) ;
#29813=CARTESIAN_POINT('',(-2.37887640734373E-15,-19.425,-328.125)) ;
#29814=CARTESIAN_POINT('Ctrl Pts',(-0.000189941651381996,-19.4249999990714,
-332.23026054535)) ;
#29815=CARTESIAN_POINT('Ctrl Pts',(0.145183061578013,-19.4250014205585,
-332.228446617012)) ;
#29816=CARTESIAN_POINT('Ctrl Pts',(0.290551611289528,-19.4233709264318,
-332.22664282915)) ;
#29817=CARTESIAN_POINT('Ctrl Pts',(0.559970945372767,-19.4173237550444,
-332.223318412199)) ;
#29818=CARTESIAN_POINT('Ctrl Pts',(0.684024165112581,-19.4133495372617,
-332.221795018015)) ;
#29819=CARTESIAN_POINT('Ctrl Pts',(0.964611173299925,-19.4016677163885,
-332.21836521505)) ;
#29820=CARTESIAN_POINT('Ctrl Pts',(1.1211069864383,-19.3932540876237,-332.216463457601)) ;
#29821=CARTESIAN_POINT('Ctrl Pts',(1.64778164968142,-19.3585422135905,-332.210096697832)) ;
#29822=CARTESIAN_POINT('Ctrl Pts',(2.01730434183639,-19.3235303464314,-332.205686909149)) ;
#29823=CARTESIAN_POINT('Ctrl Pts',(3.11839476728218,-19.1872732378065,-332.192621682752)) ;
#29824=CARTESIAN_POINT('Ctrl Pts',(3.8454224700446,-19.0548828285682,-332.184113525765)) ;
#29825=CARTESIAN_POINT('Ctrl Pts',(4.73247214919932,-18.8405063487433,-332.173265741295)) ;
#29826=CARTESIAN_POINT('Ctrl Pts',(4.901243260989,-18.7973079573857,-332.171179181993)) ;
#29827=CARTESIAN_POINT('Ctrl Pts',(5.14677633285928,-18.7309300718365,-332.168097389376)) ;
#29828=CARTESIAN_POINT('Ctrl Pts',(5.22401227178006,-18.7095361711371,-332.167121233573)) ;
#29829=CARTESIAN_POINT('Ctrl Pts',(5.3584339170233,-18.6714049008776,-332.165408952922)) ;
#29830=CARTESIAN_POINT('Ctrl Pts',(5.4156790013102,-18.6548812901269,-332.164675401307)) ;
#29831=CARTESIAN_POINT('Ctrl Pts',(5.56061613963103,-18.6123222825573,-332.162807406222)) ;
#29832=CARTESIAN_POINT('Ctrl Pts',(5.64820188983442,-18.5859303771073,-332.161668718322)) ;
#29833=CARTESIAN_POINT('Ctrl Pts',(5.98412901790217,-18.4821127610899,-332.157267863808)) ;
#29834=CARTESIAN_POINT('Ctrl Pts',(6.2310918948355,-18.4003202570807,-332.153962142931)) ;
#29835=CARTESIAN_POINT('Ctrl Pts',(7.00055523704415,-18.1282106884239,-332.143514486035)) ;
#29836=CARTESIAN_POINT('Ctrl Pts',(7.51657217514077,-17.920405691037,-332.136297820485)) ;
#29837=CARTESIAN_POINT('Ctrl Pts',(8.37952140627743,-17.5290481232115,-332.124134920143)) ;
#29838=CARTESIAN_POINT('Ctrl Pts',(8.7311104163697,-17.3566016034502,-332.119149427255)) ;
#29839=CARTESIAN_POINT('Ctrl Pts',(9.23199444589439,-17.0918559530118,-332.112037175361)) ;
#29840=CARTESIAN_POINT('Ctrl Pts',(9.38562827163967,-17.0079758772757,-332.109853938412)) ;
#29841=CARTESIAN_POINT('Ctrl Pts',(9.64797072652297,-16.8601064763324,-332.106123510751)) ;
#29842=CARTESIAN_POINT('Ctrl Pts',(9.75722826446648,-16.7971136263695,-332.104569159518)) ;
#29843=CARTESIAN_POINT('Ctrl Pts',(9.98286204189661,-16.6640792528831,-332.101357184621)) ;
#29844=CARTESIAN_POINT('Ctrl Pts',(10.0991327673247,-16.593872040654,-332.099700912792)) ;
#29845=CARTESIAN_POINT('Ctrl Pts',(10.4114274206998,-16.4008024436098,-332.095247491828)) ;
#29846=CARTESIAN_POINT('Ctrl Pts',(10.6060085039264,-16.275648239215,-332.092467702735)) ;
#29847=CARTESIAN_POINT('Ctrl Pts',(10.9319162620003,-16.057698045176,-332.087793320668)) ;
#29848=CARTESIAN_POINT('Ctrl Pts',(11.0644105451957,-15.9666928017923,-332.08588761199)) ;
#29849=CARTESIAN_POINT('Ctrl Pts',(11.6606826503562,-15.5461499688412,-332.077273464015)) ;
#29850=CARTESIAN_POINT('Ctrl Pts',(12.1109744539353,-15.1979799924377,-332.070671742748)) ;
#29851=CARTESIAN_POINT('Ctrl Pts',(12.8105859332824,-14.6061705364964,-332.059929377883)) ;
#29852=CARTESIAN_POINT('Ctrl Pts',(13.0697697607249,-14.374715546004,-332.0558308824)) ;
#29853=CARTESIAN_POINT('Ctrl Pts',(13.3947723799751,-14.0684232067241,-332.050451049101)) ;
#29854=CARTESIAN_POINT('Ctrl Pts',(13.4664170002983,-13.9998597053941,-332.049249387131)) ;
#29855=CARTESIAN_POINT('Ctrl Pts',(13.5852722199482,-13.8843593608555,-332.047226546011)) ;
#29856=CARTESIAN_POINT('Ctrl Pts',(13.6327722284112,-13.8377229892832,-332.04641009854)) ;
#29857=CARTESIAN_POINT('Ctrl Pts',(13.7360014314585,-13.7353232493974,-332.044617367667)) ;
#29858=CARTESIAN_POINT('Ctrl Pts',(13.7916326485883,-13.6794630360962,-332.043639586189)) ;
#29859=CARTESIAN_POINT('Ctrl Pts',(13.9635761062621,-13.5046967410677,-332.040583335402)) ;
#29860=CARTESIAN_POINT('Ctrl Pts',(14.0787021108828,-13.384634416601,-332.038487861583)) ;
#29861=CARTESIAN_POINT('Ctrl Pts',(14.2827527636636,-13.1662887475904,-332.034696095332)) ;
#29862=CARTESIAN_POINT('Ctrl Pts',(14.3722406182465,-13.0685456517839,-332.033005341881)) ;
#29863=CARTESIAN_POINT('Ctrl Pts',(14.8480758432325,-12.5380154714742,-332.023879596559)) ;
#29864=CARTESIAN_POINT('Ctrl Pts',(15.2158886002915,-12.0890001132909,-332.016346844542)) ;
#29865=CARTESIAN_POINT('Ctrl Pts',(15.7319625990933,-11.3980546067838,-332.005289862359)) ;
#29866=CARTESIAN_POINT('Ctrl Pts',(15.8959224334734,-11.1682561957224,-332.001692856113)) ;
#29867=CARTESIAN_POINT('Ctrl Pts',(16.1745491797759,-10.7591738876472,-331.995444926376)) ;
#29868=CARTESIAN_POINT('Ctrl Pts',(16.2913865873953,-10.5814265199878,-331.992779600584)) ;
#29869=CARTESIAN_POINT('Ctrl Pts',(16.4762155032514,-10.2899220178838,-331.988489948021)) ;
#29870=CARTESIAN_POINT('Ctrl Pts',(16.5460032924671,-10.1773251665681,-331.986852242614)) ;
#29871=CARTESIAN_POINT('Ctrl Pts',(16.680859824846,-9.95469134763043,-331.983651304628)) ;
#29872=CARTESIAN_POINT('Ctrl Pts',(16.7460049393203,-9.84470837279573,-331.982087549643)) ;
#29873=CARTESIAN_POINT('Ctrl Pts',(16.9033149498739,-9.57304552699521,-331.978266718079)) ;
#29874=CARTESIAN_POINT('Ctrl Pts',(16.9942510935242,-9.41066877916073,-331.976018807149)) ;
#29875=CARTESIAN_POINT('Ctrl Pts',(17.1386599867603,-9.14388914501315,-331.972379375948)) ;
#29876=CARTESIAN_POINT('Ctrl Pts',(17.1935450362668,-9.04026459545534,-331.970978696809)) ;
#29877=CARTESIAN_POINT('Ctrl Pts',(17.4015354542087,-8.63882632729048,-331.965598756246)) ;
#29878=CARTESIAN_POINT('Ctrl Pts',(17.547868631977,-8.33756939353622,-331.961659792414)) ;
#29879=CARTESIAN_POINT('Ctrl Pts',(17.9709482516761,-7.40603345718022,-331.949681911)) ;
#29880=CARTESIAN_POINT('Ctrl Pts',(18.2220486622741,-6.76470604059831,-331.941725831355)) ;
#29881=CARTESIAN_POINT('Ctrl Pts',(18.4736973084831,-6.00546341794311,-331.932118568671)) ;
#29882=CARTESIAN_POINT('Ctrl Pts',(18.5078995812386,-5.89921487556642,-331.930769464782)) ;
#29883=CARTESIAN_POINT('Ctrl Pts',(18.5596270560921,-5.73364573708061,-331.928656118261)) ;
#29884=CARTESIAN_POINT('Ctrl Pts',(18.5777878853142,-5.67452616352374,-331.927899335838)) ;
#29885=CARTESIAN_POINT('Ctrl Pts',(18.6162719118137,-5.54708267132632,-331.926262349003)) ;
#29886=CARTESIAN_POINT('Ctrl Pts',(18.6365019847742,-5.47873158792611,-331.925380961635)) ;
#29887=CARTESIAN_POINT('Ctrl Pts',(18.6913140242785,-5.28972202966955,-331.922935778102)) ;
#29888=CARTESIAN_POINT('Ctrl Pts',(18.7251034368335,-5.16883742374057,-331.921363064997)) ;
#29889=CARTESIAN_POINT('Ctrl Pts',(18.8008697492577,-4.88727913632979,-331.917686195177)) ;
#29890=CARTESIAN_POINT('Ctrl Pts',(18.8419625989181,-4.72637768170358,-331.915574650318)) ;
#29891=CARTESIAN_POINT('Ctrl Pts',(18.990419540356,-4.11235086217358,-331.907500506545)) ;
#29892=CARTESIAN_POINT('Ctrl Pts',(19.0835410384605,-3.65594384115663,-331.901469366308)) ;
#29893=CARTESIAN_POINT('Ctrl Pts',(19.2388388600166,-2.72511031791686,-331.889313621042)) ;
#29894=CARTESIAN_POINT('Ctrl Pts',(19.3000738742438,-2.2508437299137,-331.883195438394)) ;
#29895=CARTESIAN_POINT('Ctrl Pts',(19.3609659263224,-1.58717469476144,-331.874810973372)) ;
#29896=CARTESIAN_POINT('Ctrl Pts',(19.3754500400912,-1.39930733366558,-331.872456557579)) ;
#29897=CARTESIAN_POINT('Ctrl Pts',(19.3951138116733,-1.08457241748325,-331.868545031217)) ;
#29898=CARTESIAN_POINT('Ctrl Pts',(19.4017868898804,-0.95781137292958,-331.866978509954)) ;
#29899=CARTESIAN_POINT('Ctrl Pts',(19.4128469572975,-0.699512103697202,
-331.863804109812)) ;
#29900=CARTESIAN_POINT('Ctrl Pts',(19.4171405487011,-0.567976352789986,
-331.862196913271)) ;
#29901=CARTESIAN_POINT('Ctrl Pts',(19.4247674339681,-0.228580240947926,
-331.85807258392)) ;
#29902=CARTESIAN_POINT('Ctrl Pts',(19.4261012774139,-0.0206916773786139,
-331.855568341005)) ;
#29903=CARTESIAN_POINT('Ctrl Pts',(19.4216149522909,0.44486853013388,-331.850000704656)) ;
#29904=CARTESIAN_POINT('Ctrl Pts',(19.4140040167574,0.70248393352843,-331.846947842104)) ;
#29905=CARTESIAN_POINT('Ctrl Pts',(19.3639925052298,1.71333444094908,-331.835031566279)) ;
#29906=CARTESIAN_POINT('Ctrl Pts',(19.2828551746358,2.46398241000536,-331.826344588909)) ;
#29907=CARTESIAN_POINT('Ctrl Pts',(19.1319614578613,3.36512328443824,-331.815464527323)) ;
#29908=CARTESIAN_POINT('Ctrl Pts',(19.1037202554312,3.52191371448126,-331.813553539969)) ;
#29909=CARTESIAN_POINT('Ctrl Pts',(19.0586733397916,3.75549871709915,-331.810669442696)) ;
#29910=CARTESIAN_POINT('Ctrl Pts',(19.0433249563059,3.83256763474922,-331.809711792714)) ;
#29911=CARTESIAN_POINT('Ctrl Pts',(19.0140984886371,3.97481115013713,-331.807931437525)) ;
#29912=CARTESIAN_POINT('Ctrl Pts',(19.0003519094621,4.04001142270088,-331.807110220716)) ;
#29913=CARTESIAN_POINT('Ctrl Pts',(18.9652086770134,4.20254886742442,-331.805050840987)) ;
#29914=CARTESIAN_POINT('Ctrl Pts',(18.943397910721,4.29979449540964,-331.803807923576)) ;
#29915=CARTESIAN_POINT('Ctrl Pts',(18.8376944509196,4.75466334579143,-331.797950406501)) ;
#29916=CARTESIAN_POINT('Ctrl Pts',(18.7444170238787,5.11002791269658,-331.793248596988)) ;
#29917=CARTESIAN_POINT('Ctrl Pts',(18.4146725110056,6.23529479487276,-331.778157495301)) ;
#29918=CARTESIAN_POINT('Ctrl Pts',(18.1403904340824,6.99323323157091,-331.767716400128)) ;
#29919=CARTESIAN_POINT('Ctrl Pts',(17.7472338864107,7.89934219163304,-331.755301613081)) ;
#29920=CARTESIAN_POINT('Ctrl Pts',(17.6722512209016,8.06569616394171,-331.753023343509)) ;
#29921=CARTESIAN_POINT('Ctrl Pts',(17.5415549493129,8.34507912297241,-331.749199630797)) ;
#29922=CARTESIAN_POINT('Ctrl Pts',(17.4870651022486,8.45866713891524,-331.747645723418)) ;
#29923=CARTESIAN_POINT('Ctrl Pts',(17.3727364855567,8.69116621621547,-331.744466119297)) ;
#29924=CARTESIAN_POINT('Ctrl Pts',(17.3127725646518,8.81000847761039,-331.742841425203)) ;
#29925=CARTESIAN_POINT('Ctrl Pts',(17.1521909530555,9.12029281623065,-331.738599490998)) ;
#29926=CARTESIAN_POINT('Ctrl Pts',(17.0495893622681,9.31068731832818,-331.735996681663)) ;
#29927=CARTESIAN_POINT('Ctrl Pts',(16.8726434363274,9.62630346965445,-331.731674593841)) ;
#29928=CARTESIAN_POINT('Ctrl Pts',(16.8000318651307,9.75247375823509,-331.72994472089)) ;
#29929=CARTESIAN_POINT('Ctrl Pts',(16.4856041523759,10.2848911192371,-331.722627467802)) ;
#29930=CARTESIAN_POINT('Ctrl Pts',(16.2304183255159,10.6830543810869,-331.717115752371)) ;
#29931=CARTESIAN_POINT('Ctrl Pts',(15.7058696099165,11.4392567127996,-331.70636365177)) ;
#29932=CARTESIAN_POINT('Ctrl Pts',(15.438145079093,11.7980764918677,-331.701126965723)) ;
#29933=CARTESIAN_POINT('Ctrl Pts',(15.0839428810739,12.240074279329,-331.694334025471)) ;
#29934=CARTESIAN_POINT('Ctrl Pts',(15.0087687247099,12.3321373860809,-331.692899320292)) ;
#29935=CARTESIAN_POINT('Ctrl Pts',(14.8923993896484,12.4720105345549,-331.690684507595)) ;
#29936=CARTESIAN_POINT('Ctrl Pts',(14.8518082039201,12.5203194614866,-331.689913059907)) ;
#29937=CARTESIAN_POINT('Ctrl Pts',(14.7659324756137,12.6215177757053,-331.688282321056)) ;
#29938=CARTESIAN_POINT('Ctrl Pts',(14.7205975219702,12.6743631557729,-331.687422153422)) ;
#29939=CARTESIAN_POINT('Ctrl Pts',(14.5982276757477,12.8154631890887,-331.685103659509)) ;
#29940=CARTESIAN_POINT('Ctrl Pts',(14.5206769381909,12.9032666104526,-331.683637820034)) ;
#29941=CARTESIAN_POINT('Ctrl Pts',(14.3888086845939,13.0498741938686,-331.681155076116)) ;
#29942=CARTESIAN_POINT('Ctrl Pts',(14.3349132574999,13.1090538835616,-331.680143046149)) ;
#29943=CARTESIAN_POINT('Ctrl Pts',(14.1912763778585,13.2648288154611,-331.677454810346)) ;
#29944=CARTESIAN_POINT('Ctrl Pts',(14.1009146274485,13.3608463562341,-331.675772751248)) ;
#29945=CARTESIAN_POINT('Ctrl Pts',(13.6120280139532,13.8698482651593,-331.666736121505)) ;
#29946=CARTESIAN_POINT('Ctrl Pts',(13.196325332094,14.265938335449,-331.659285049867)) ;
#29947=CARTESIAN_POINT('Ctrl Pts',(12.5478290072065,14.8312041481034,-331.648251896928)) ;
#29948=CARTESIAN_POINT('Ctrl Pts',(12.3278261885927,15.0145706293054,-331.644601329447)) ;
#29949=CARTESIAN_POINT('Ctrl Pts',(11.9359971651274,15.3267300233875,-331.638275907073)) ;
#29950=CARTESIAN_POINT('Ctrl Pts',(11.7659397493424,15.4576629404534,-331.635586056566)) ;
#29951=CARTESIAN_POINT('Ctrl Pts',(11.4871858024061,15.6650191878181,-331.631267762876)) ;
#29952=CARTESIAN_POINT('Ctrl Pts',(11.3798138182809,15.7431922217855,-331.629625595117)) ;
#29953=CARTESIAN_POINT('Ctrl Pts',(11.1677215703687,15.8943041232146,-331.626422746484)) ;
#29954=CARTESIAN_POINT('Ctrl Pts',(11.0630674282216,15.9673243770922,-331.62486146989)) ;
#29955=CARTESIAN_POINT('Ctrl Pts',(10.8051447725305,16.143531442446,-331.621059083091)) ;
#29956=CARTESIAN_POINT('Ctrl Pts',(10.6511088968725,16.245572947636,-331.618826922081)) ;
#29957=CARTESIAN_POINT('Ctrl Pts',(10.3979809418721,16.408110407635,-331.615217155277)) ;
#29958=CARTESIAN_POINT('Ctrl Pts',(10.2997611428721,16.469942782157,-331.613830463344)) ;
#29959=CARTESIAN_POINT('Ctrl Pts',(9.44878637246384,16.9950679920014,-331.601928374943)) ;
#29960=CARTESIAN_POINT('Ctrl Pts',(8.66577910616792,17.4073594147061,-331.591781831453)) ;
#29961=CARTESIAN_POINT('Ctrl Pts',(7.67737204769751,17.8445326499902,-331.578978450184)) ;
#29962=CARTESIAN_POINT('Ctrl Pts',(7.49611701379523,17.9214289758924,-331.576628211505)) ;
#29963=CARTESIAN_POINT('Ctrl Pts',(7.23407970049879,18.0279257539974,-331.573208953416)) ;
#29964=CARTESIAN_POINT('Ctrl Pts',(7.15422067673161,18.0597658508473,-331.572164032097)) ;
#29965=CARTESIAN_POINT('Ctrl Pts',(7.01300957922743,18.1149836266799,-331.570309308251)) ;
#29966=CARTESIAN_POINT('Ctrl Pts',(6.95174558882464,18.1385823152968,-331.569502199694)) ;
#29967=CARTESIAN_POINT('Ctrl Pts',(6.8088222228855,18.1928054690851,-331.567613513103)) ;
#29968=CARTESIAN_POINT('Ctrl Pts',(6.72707411148477,18.2231913991497,-331.566529087482)) ;
#29969=CARTESIAN_POINT('Ctrl Pts',(6.43547579214956,18.3293495278886,-331.562649752165)) ;
#29970=CARTESIAN_POINT('Ctrl Pts',(6.22452825124152,18.402055605892,-331.559823078078)) ;
#29971=CARTESIAN_POINT('Ctrl Pts',(5.62542245516853,18.5970654761727,-331.5517811508)) ;
#29972=CARTESIAN_POINT('Ctrl Pts',(5.23460710018778,18.7108286924396,-331.546520495896)) ;
#29973=CARTESIAN_POINT('Ctrl Pts',(4.79050246733825,18.8250996604329,-331.540606014974)) ;
#29974=CARTESIAN_POINT('Ctrl Pts',(4.74044574905439,18.8377669912263,-331.53994023261)) ;
#29975=CARTESIAN_POINT('Ctrl Pts',(4.18408516602188,18.976201332403,-331.532551111083)) ;
#29976=CARTESIAN_POINT('Ctrl Pts',(3.67296095157779,19.0817228347984,-331.525868754511)) ;
#29977=CARTESIAN_POINT('Ctrl Pts',(2.9792747107328,19.1960265196259,-331.517033784981)) ;
#29978=CARTESIAN_POINT('Ctrl Pts',(2.7999357611646,19.2230037148001,-331.514769780853)) ;
#29979=CARTESIAN_POINT('Ctrl Pts',(2.49558946317666,19.2644357630188,-331.510962456308)) ;
#29980=CARTESIAN_POINT('Ctrl Pts',(2.37077170894318,19.2801943348318,-331.509410846289)) ;
#29981=CARTESIAN_POINT('Ctrl Pts',(2.11327886946166,19.3101651927803,-331.506229803252)) ;
#29982=CARTESIAN_POINT('Ctrl Pts',(1.98059263133643,19.3242252170197,-331.504601436768)) ;
#29983=CARTESIAN_POINT('Ctrl Pts',(1.6307434255086,19.3576556525071,-331.500334913811)) ;
#29984=CARTESIAN_POINT('Ctrl Pts',(1.4133809057161,19.374738994857,-331.497711518008)) ;
#29985=CARTESIAN_POINT('Ctrl Pts',(1.04876343398794,19.3972270022643,-331.493348896814)) ;
#29986=CARTESIAN_POINT('Ctrl Pts',(0.901651694841911,19.4046217277171,-331.491599008477)) ;
#29987=CARTESIAN_POINT('Ctrl Pts',(0.272172070881169,19.4290892764116,-331.48414634572)) ;
#29988=CARTESIAN_POINT('Ctrl Pts',(-0.210657321659002,19.429853615345,-331.478522171617)) ;
#29989=CARTESIAN_POINT('Ctrl Pts',(-0.857525756742793,19.4067610302219,
-331.47095862306)) ;
#29990=CARTESIAN_POINT('Ctrl Pts',(-1.02195766698405,19.3987970398744,-331.4690330048)) ;
#29991=CARTESIAN_POINT('Ctrl Pts',(-1.49472725504589,19.3698714114922,-331.46347056873)) ;
#29992=CARTESIAN_POINT('Ctrl Pts',(-1.80269132314621,19.3436405902285,-331.459815864918)) ;
#29993=CARTESIAN_POINT('Ctrl Pts',(-2.20740205846246,19.2994202455134,-331.454910134814)) ;
#29994=CARTESIAN_POINT('Ctrl Pts',(-2.30482453628656,19.2880281387308,-331.453721268001)) ;
#29995=CARTESIAN_POINT('Ctrl Pts',(-2.46807440058971,19.2676839918965,-331.451712942153)) ;
#29996=CARTESIAN_POINT('Ctrl Pts',(-2.53394971701626,19.2591312498112,-331.450898048381)) ;
#29997=CARTESIAN_POINT('Ctrl Pts',(-2.67847661660683,19.2396126294239,-331.449099641192)) ;
#29998=CARTESIAN_POINT('Ctrl Pts',(-2.75710726738437,19.2285020376209,-331.448114532312)) ;
#29999=CARTESIAN_POINT('Ctrl Pts',(-3.00360809940843,19.1921281142128,-331.4450077374)) ;
#30000=CARTESIAN_POINT('Ctrl Pts',(-3.17121642209234,19.1651462142298,-331.442868271512)) ;
#30001=CARTESIAN_POINT('Ctrl Pts',(-3.85795317980455,19.0453385594749,-331.434019652971)) ;
#30002=CARTESIAN_POINT('Ctrl Pts',(-4.37355068944828,18.9335886096018,-331.427187546371)) ;
#30003=CARTESIAN_POINT('Ctrl Pts',(-5.4183967982167,18.6621675421631,-331.413273094881)) ;
#30004=CARTESIAN_POINT('Ctrl Pts',(-5.9466718113193,18.5006113154178,-331.40620172262)) ;
#30005=CARTESIAN_POINT('Ctrl Pts',(-6.61235440309683,18.2655698793065,-331.397346078729)) ;
#30006=CARTESIAN_POINT('Ctrl Pts',(-6.75674945712199,18.2126497420973,-331.395427932506)) ;
#30007=CARTESIAN_POINT('Ctrl Pts',(-7.01839704791395,18.1132171273544,-331.391957689612)) ;
#30008=CARTESIAN_POINT('Ctrl Pts',(-7.13585402567213,18.0672665115155,-331.390401878052)) ;
#30009=CARTESIAN_POINT('Ctrl Pts',(-7.37610560545495,17.9705687875472,-331.387223338295)) ;
#30010=CARTESIAN_POINT('Ctrl Pts',(-7.49884387351457,17.9196991344049,-331.38560156125)) ;
#30011=CARTESIAN_POINT('Ctrl Pts',(-7.81869503445604,17.78327312194,-331.381379173044)) ;
#30012=CARTESIAN_POINT('Ctrl Pts',(-8.01492718843297,17.695698272446,-331.378792732357)) ;
#30013=CARTESIAN_POINT('Ctrl Pts',(-8.34035800174749,17.5439404947011,-331.374502793489)) ;
#30014=CARTESIAN_POINT('Ctrl Pts',(-8.47036715907341,17.4815416918333,-331.372788756653)) ;
#30015=CARTESIAN_POINT('Ctrl Pts',(-9.01669629313318,17.2118017302532,-331.365576814086)) ;
#30016=CARTESIAN_POINT('Ctrl Pts',(-9.42619412550397,16.9909915989308,-331.360152335424)) ;
#30017=CARTESIAN_POINT('Ctrl Pts',(-9.91875193730231,16.7021019026936,-331.353481819009)) ;
#30018=CARTESIAN_POINT('Ctrl Pts',(-10.0096928089832,16.6477595437041,-331.352243746245)) ;
#30019=CARTESIAN_POINT('Ctrl Pts',(-10.4054628321071,16.4068490190876,-331.346820433181)) ;
#30020=CARTESIAN_POINT('Ctrl Pts',(-10.7055540384789,16.2126328265006,-331.342617157296)) ;
#30021=CARTESIAN_POINT('Ctrl Pts',(-11.0962296247897,15.9442124902621,-331.336929884951)) ;
#30022=CARTESIAN_POINT('Ctrl Pts',(-11.1917471523464,15.8773114676175,-331.335521660125)) ;
#30023=CARTESIAN_POINT('Ctrl Pts',(-11.3376888021515,15.7731217355167,-331.333338341927)) ;
#30024=CARTESIAN_POINT('Ctrl Pts',(-11.3885445195097,15.736442112944,-331.332571531048)) ;
#30025=CARTESIAN_POINT('Ctrl Pts',(-11.4958613239839,15.6582473044546,-331.33093969124)) ;
#30026=CARTESIAN_POINT('Ctrl Pts',(-11.5522771202698,15.6166715256386,-331.330073694845)) ;
#30027=CARTESIAN_POINT('Ctrl Pts',(-11.7042590679014,15.5033937732473,-331.327720044719)) ;
#30028=CARTESIAN_POINT('Ctrl Pts',(-11.7993906854033,15.4311139651934,-331.326224493936)) ;
#30029=CARTESIAN_POINT('Ctrl Pts',(-12.2155905345387,15.1087913461664,-331.319593546571)) ;
#30030=CARTESIAN_POINT('Ctrl Pts',(-12.5294219555271,14.8495728079125,-331.314362474225)) ;
#30031=CARTESIAN_POINT('Ctrl Pts',(-13.3881918424572,14.0936272529455,-331.299611735002)) ;
#30032=CARTESIAN_POINT('Ctrl Pts',(-13.9133341702555,13.5754613423282,-331.29008804216)) ;
#30033=CARTESIAN_POINT('Ctrl Pts',(-14.5270836557819,12.8967483345373,-331.278595076019)) ;
#30034=CARTESIAN_POINT('Ctrl Pts',(-14.6445931160055,12.7631567312836,-331.276375032726)) ;
#30035=CARTESIAN_POINT('Ctrl Pts',(-14.8425103502254,12.5318204100332,-331.272602574181)) ;
#30036=CARTESIAN_POINT('Ctrl Pts',(-14.9238283723514,12.4348696433832,-331.271042558816)) ;
#30037=CARTESIAN_POINT('Ctrl Pts',(-15.0898236597302,12.2329892103144,-331.267836696898)) ;
#30038=CARTESIAN_POINT('Ctrl Pts',(-15.1743674369943,12.1279584451394,-331.266192014314)) ;
#30039=CARTESIAN_POINT('Ctrl Pts',(-15.3975558965813,11.8446984654067,-331.261816306679)) ;
#30040=CARTESIAN_POINT('Ctrl Pts',(-15.5341979193056,11.6649176839494,-331.259101540744)) ;
#30041=CARTESIAN_POINT('Ctrl Pts',(-15.8394661575855,11.248395114483,-331.252940539209)) ;
#30042=CARTESIAN_POINT('Ctrl Pts',(-16.0059758350177,11.010168878258,-331.249509062683)) ;
#30043=CARTESIAN_POINT('Ctrl Pts',(-16.4010222887596,10.41706236079,-331.241142833796)) ;
#30044=CARTESIAN_POINT('Ctrl Pts',(-16.6234582152476,10.0582979240445,-331.236233557358)) ;
#30045=CARTESIAN_POINT('Ctrl Pts',(-17.0157179024034,9.37702254855795,-331.227026665904)) ;
#30046=CARTESIAN_POINT('Ctrl Pts',(-17.1884951408275,9.05642541069598,-331.222738703137)) ;
#30047=CARTESIAN_POINT('Ctrl Pts',(-17.3989377270437,8.63819554004497,-331.217105491648)) ;
#30048=CARTESIAN_POINT('Ctrl Pts',(-17.4449686597368,8.54485369300976,-331.215845680376)) ;
#30049=CARTESIAN_POINT('Ctrl Pts',(-17.5192329167675,8.39115854581083,-331.213763833116)) ;
#30050=CARTESIAN_POINT('Ctrl Pts',(-17.5479098209778,8.33102182555669,-331.212947371418)) ;
#30051=CARTESIAN_POINT('Ctrl Pts',(-17.6087414185538,8.2017476411726,-331.21118726001)) ;
#30052=CARTESIAN_POINT('Ctrl Pts',(-17.6407995088479,8.13256610083372,-331.210242462108)) ;
#30053=CARTESIAN_POINT('Ctrl Pts',(-17.7353603690866,7.92531308687257,-331.207405543751)) ;
#30054=CARTESIAN_POINT('Ctrl Pts',(-17.7966553838376,7.78669711603526,-331.205499591473)) ;
#30055=CARTESIAN_POINT('Ctrl Pts',(-17.9418964534058,7.44756503803881,-331.20082801241)) ;
#30056=CARTESIAN_POINT('Ctrl Pts',(-18.0241110520805,7.246329686057,-331.198048881185)) ;
#30057=CARTESIAN_POINT('Ctrl Pts',(-18.4078383340327,6.26012471535239,-331.184457460101)) ;
#30058=CARTESIAN_POINT('Ctrl Pts',(-18.6615438059373,5.45751492504185,-331.17352600709)) ;
#30059=CARTESIAN_POINT('Ctrl Pts',(-18.9084208581279,4.4541305363446,-331.160518479094)) ;
#30060=CARTESIAN_POINT('Ctrl Pts',(-18.9516190265467,4.26659051511602,-331.158112550982)) ;
#30061=CARTESIAN_POINT('Ctrl Pts',(-19.0163859465048,3.96499112006096,-331.154284912674)) ;
#30062=CARTESIAN_POINT('Ctrl Pts',(-19.039731394866,3.85132671920606,-331.152851743723)) ;
#30063=CARTESIAN_POINT('Ctrl Pts',(-19.086773875808,3.61139733433789,-331.149845963584)) ;
#30064=CARTESIAN_POINT('Ctrl Pts',(-19.1102395940689,3.48509259576566,-331.148274937152)) ;
#30065=CARTESIAN_POINT('Ctrl Pts',(-19.1652895313905,3.17149424870167,-331.144401062335)) ;
#30066=CARTESIAN_POINT('Ctrl Pts',(-19.1953829449298,2.98395246974467,-331.142108007504)) ;
#30067=CARTESIAN_POINT('Ctrl Pts',(-19.2986898218603,2.27370936039285,-331.133502633434)) ;
#30068=CARTESIAN_POINT('Ctrl Pts',(-19.3533406346527,1.74853959813532,-331.12730638308)) ;
#30069=CARTESIAN_POINT('Ctrl Pts',(-19.4248319342674,0.614170808014305,
-331.114023253272)) ;
#30070=CARTESIAN_POINT('Ctrl Pts',(-19.4345380838159,0.00508200935372204,
-331.106955117943)) ;
#30071=CARTESIAN_POINT('Ctrl Pts',(-19.4122294674355,-0.712681329477538,
-331.098325319068)) ;
#30072=CARTESIAN_POINT('Ctrl Pts',(-19.4079128409369,-0.821879968633598,
-331.097003834431)) ;
#30073=CARTESIAN_POINT('Ctrl Pts',(-19.3997291682074,-0.992426653349981,
-331.094922963838)) ;
#30074=CARTESIAN_POINT('Ctrl Pts',(-19.3964920087444,-1.05380273969823,
-331.094170661844)) ;
#30075=CARTESIAN_POINT('Ctrl Pts',(-19.3888339309363,-1.18697869874726,
-331.092529909088)) ;
#30076=CARTESIAN_POINT('Ctrl Pts',(-19.3843053549776,-1.25877143327545,
-331.091640164774)) ;
#30077=CARTESIAN_POINT('Ctrl Pts',(-19.3705551367299,-1.45904442080467,
-331.089145104652)) ;
#30078=CARTESIAN_POINT('Ctrl Pts',(-19.3604541808115,-1.58746047584606,
-331.087530297816)) ;
#30079=CARTESIAN_POINT('Ctrl Pts',(-19.3338682327726,-1.88727608978324,
-331.083732471144)) ;
#30080=CARTESIAN_POINT('Ctrl Pts',(-19.3163800236605,-2.05857585171063,
-331.081541412064)) ;
#30081=CARTESIAN_POINT('Ctrl Pts',(-19.2387950090773,-2.73004819154784,
-331.072895872852)) ;
#30082=CARTESIAN_POINT('Ctrl Pts',(-19.1615284085456,-3.22803746948053,
-331.066364867967)) ;
#30083=CARTESIAN_POINT('Ctrl Pts',(-18.9749274874972,-4.18373507064429,
-331.053838058016)) ;
#30084=CARTESIAN_POINT('Ctrl Pts',(-18.8681515431548,-4.64159151181229,
-331.047839442751)) ;
#30085=CARTESIAN_POINT('Ctrl Pts',(-18.7046641370253,-5.24305883587811,
-331.040021539713)) ;
#30086=CARTESIAN_POINT('Ctrl Pts',(-18.6627036336701,-5.39051199823045,
-331.038109534483)) ;
#30087=CARTESIAN_POINT('Ctrl Pts',(-18.5830784803378,-5.65824173993203,
-331.034646763535)) ;
#30088=CARTESIAN_POINT('Ctrl Pts',(-18.5459803184889,-5.77867800357317,
-331.033092341189)) ;
#30089=CARTESIAN_POINT('Ctrl Pts',(-18.4673126107459,-6.02550328362981,
-331.029913036015)) ;
#30090=CARTESIAN_POINT('Ctrl Pts',(-18.4256111792053,-6.1518434321073,-331.028289141783)) ;
#30091=CARTESIAN_POINT('Ctrl Pts',(-18.3128463043304,-6.48204371838377,
-331.024052565633)) ;
#30092=CARTESIAN_POINT('Ctrl Pts',(-18.2396765042545,-6.6851650518102,-331.021454242966)) ;
#30093=CARTESIAN_POINT('Ctrl Pts',(-18.1116586833711,-7.02278618811575,
-331.017140974204)) ;
#30094=CARTESIAN_POINT('Ctrl Pts',(-18.058660651361,-7.15796630620107,-331.015415448825)) ;
#30095=CARTESIAN_POINT('Ctrl Pts',(-17.8274634880234,-7.72875633338713,
-331.008127264169)) ;
#30096=CARTESIAN_POINT('Ctrl Pts',(-17.634979747844,-8.15840784149597,-331.002639648016)) ;
#30097=CARTESIAN_POINT('Ctrl Pts',(-17.3995424610263,-8.63657536145363,
-330.996412990582)) ;
#30098=CARTESIAN_POINT('Ctrl Pts',(-17.3717338276901,-8.69237456889157,
-330.995684419256)) ;
#30099=CARTESIAN_POINT('Ctrl Pts',(-17.1674965137336,-9.09729068326911,
-330.990380881024)) ;
#30100=CARTESIAN_POINT('Ctrl Pts',(-16.9808271065427,-9.44114101991094,
-330.985789306889)) ;
#30101=CARTESIAN_POINT('Ctrl Pts',(-16.7248235438796,-9.88051997812779,
-330.979688802644)) ;
#30102=CARTESIAN_POINT('Ctrl Pts',(-16.6648250242299,-9.98138289336614,
-330.978271794879)) ;
#30103=CARTESIAN_POINT('Ctrl Pts',(-16.5713053719243,-10.1354038547098,
-330.976078039556)) ;
#30104=CARTESIAN_POINT('Ctrl Pts',(-16.538434104238,-10.1889533513697,-330.975309699002)) ;
#30105=CARTESIAN_POINT('Ctrl Pts',(-16.4684341509548,-10.301756696567,-330.973678298799)) ;
#30106=CARTESIAN_POINT('Ctrl Pts',(-16.4312441854975,-10.3609714269547,
-330.972814302207)) ;
#30107=CARTESIAN_POINT('Ctrl Pts',(-16.3300739797615,-10.5201422646501,
-330.970472670263)) ;
#30108=CARTESIAN_POINT('Ctrl Pts',(-16.2654961231903,-10.6197149329542,
-330.968987269506)) ;
#30109=CARTESIAN_POINT('Ctrl Pts',(-16.1550346448633,-10.7866641723192,
-330.966466050456)) ;
#30110=CARTESIAN_POINT('Ctrl Pts',(-16.1096319930367,-10.8543551340401,
-330.965435157717)) ;
#30111=CARTESIAN_POINT('Ctrl Pts',(-15.7672491658867,-11.3579343855912,
-330.957706666126)) ;
#30112=CARTESIAN_POINT('Ctrl Pts',(-15.4530517845319,-11.7818508726733,
-330.950873599303)) ;
#30113=CARTESIAN_POINT('Ctrl Pts',(-14.7746704770437,-12.6232301223945,
-330.936942382117)) ;
#30114=CARTESIAN_POINT('Ctrl Pts',(-14.4090979695469,-13.0389694989348,
-330.929855391493)) ;
#30115=CARTESIAN_POINT('Ctrl Pts',(-13.9197885755823,-13.5496790992831,
-330.920982898976)) ;
#30116=CARTESIAN_POINT('Ctrl Pts',(-13.8119838383127,-13.6595541735275,
-330.919062926041)) ;
#30117=CARTESIAN_POINT('Ctrl Pts',(-13.6134688231621,-13.8571283579793,
-330.915590458838)) ;
#30118=CARTESIAN_POINT('Ctrl Pts',(-13.5231882670627,-13.9452471785663,
-330.914034232333)) ;
#30119=CARTESIAN_POINT('Ctrl Pts',(-13.346716337236,-14.1141681907648,-330.911035974264)) ;
#30120=CARTESIAN_POINT('Ctrl Pts',(-13.2606335339846,-14.1950758723145,
-330.909593032186)) ;
#30121=CARTESIAN_POINT('Ctrl Pts',(-13.1699067672301,-14.2788027883436,
-330.908092150886)) ;
#30122=CARTESIAN_POINT('Ctrl Pts',(-13.1659940537106,-14.2824106474933,
-330.90802746166)) ;
#30123=CARTESIAN_POINT('Ctrl Pts',(-13.1579043470016,-14.289863905213,-330.907893792867)) ;
#30124=CARTESIAN_POINT('Ctrl Pts',(-13.1537271496615,-14.2937090815021,
-330.9078248152)) ;
#30125=CARTESIAN_POINT('Ctrl Pts',(-13.1450454851963,-14.3016936625354,
-330.907681545887)) ;
#30126=CARTESIAN_POINT('Ctrl Pts',(-13.1405407471776,-14.3058327718681,
-330.90760725676)) ;
#30127=CARTESIAN_POINT('Ctrl Pts',(-13.1311302780127,-14.3144712417989,
-330.907452170609)) ;
#30128=CARTESIAN_POINT('Ctrl Pts',(-13.1262241878562,-14.3189702101993,
-330.907371376918)) ;
#30129=CARTESIAN_POINT('Ctrl Pts',(-13.1159235063309,-14.3284063682432,
-330.90720186952)) ;
#30130=CARTESIAN_POINT('Ctrl Pts',(-13.110528437521,-14.3333430352586,-330.907113160237)) ;
#30131=CARTESIAN_POINT('Ctrl Pts',(-13.0991448293914,-14.3437476099942,
-330.906926134182)) ;
#30132=CARTESIAN_POINT('Ctrl Pts',(-13.0931556511202,-14.3492148167117,
-330.90682782332)) ;
#30133=CARTESIAN_POINT('Ctrl Pts',(-13.0804569693467,-14.360792207424,-330.906619563303)) ;
#30134=CARTESIAN_POINT('Ctrl Pts',(-13.0737466040408,-14.366901443425,-330.906509622107)) ;
#30135=CARTESIAN_POINT('Ctrl Pts',(-13.0594515520137,-14.379897604564,-330.906275647762)) ;
#30136=CARTESIAN_POINT('Ctrl Pts',(-13.0518656929647,-14.3867832363587,
-330.906151625416)) ;
#30137=CARTESIAN_POINT('Ctrl Pts',(-13.0356324391991,-14.4014946422293,
-330.905886522223)) ;
#30138=CARTESIAN_POINT('Ctrl Pts',(-13.0269834365479,-14.4093186363547,
-330.905745456151)) ;
#30139=CARTESIAN_POINT('Ctrl Pts',(-13.0083967774867,-14.4261019442397,
-330.905442690165)) ;
#30140=CARTESIAN_POINT('Ctrl Pts',(-12.9984568996897,-14.435058789388,-330.905281010596)) ;
#30141=CARTESIAN_POINT('Ctrl Pts',(-12.9770147644486,-14.4543402375308,
-330.904932742837)) ;
#30142=CARTESIAN_POINT('Ctrl Pts',(-12.9655094221139,-14.4646613968036,
-330.904746182784)) ;
#30143=CARTESIAN_POINT('Ctrl Pts',(-12.9487538038036,-14.4796563957236,
-330.904474940548)) ;
#30144=CARTESIAN_POINT('Ctrl Pts',(-12.9435132910517,-14.4843411342772,
-330.904390170528)) ;
#30145=CARTESIAN_POINT('Ctrl Pts',(-12.9303581890717,-14.4960882523597,
-330.904177535307)) ;
#30146=CARTESIAN_POINT('Ctrl Pts',(-12.9224403554353,-14.5031469956744,
-330.904049699289)) ;
#30147=CARTESIAN_POINT('Ctrl Pts',(-12.5958014799049,-14.7938654864636,
-330.898781981125)) ;
#30148=CARTESIAN_POINT('Ctrl Pts',(-12.2678263181999,-15.0669542219889,
-330.893730121574)) ;
#30149=CARTESIAN_POINT('Ctrl Pts',(-11.6482163253446,-15.5492188085486,
-330.884513168464)) ;
#30150=CARTESIAN_POINT('Ctrl Pts',(-11.3592662970941,-15.7615423839009,
-330.880336402993)) ;
#30151=CARTESIAN_POINT('Ctrl Pts',(-10.7377138213715,-16.1922916213235,
-330.871494332941)) ;
#30152=CARTESIAN_POINT('Ctrl Pts',(-10.4039410716307,-16.4087420247496,
-330.866827909134)) ;
#30153=CARTESIAN_POINT('Ctrl Pts',(-9.96463563821109,-16.6748341016949,
-330.860667380911)) ;
#30154=CARTESIAN_POINT('Ctrl Pts',(-9.86497531991412,-16.7339869009585,
-330.859268449241)) ;
#30155=CARTESIAN_POINT('Ctrl Pts',(-9.72082005359146,-16.8178140616465,
-330.857239088423)) ;
#30156=CARTESIAN_POINT('Ctrl Pts',(-9.6767481048739,-16.8432110488327,-330.856617879281)) ;
#30157=CARTESIAN_POINT('Ctrl Pts',(-9.59049287432927,-16.8924663687887,
-330.85540009264)) ;
#30158=CARTESIAN_POINT('Ctrl Pts',(-9.54831914442612,-16.9163404759529,
-330.854803686318)) ;
#30159=CARTESIAN_POINT('Ctrl Pts',(-9.45018271606108,-16.9714105656705,
-330.853413739131)) ;
#30160=CARTESIAN_POINT('Ctrl Pts',(-9.39415419047365,-17.002487964705,-330.852618639159)) ;
#30161=CARTESIAN_POINT('Ctrl Pts',(-9.26180208748804,-17.0750459107955,
-330.850737750977)) ;
#30162=CARTESIAN_POINT('Ctrl Pts',(-9.18535200016055,-17.1162928045992,
-330.849649215486)) ;
#30163=CARTESIAN_POINT('Ctrl Pts',(-8.97644632944115,-17.2272003754551,
-330.846671659059)) ;
#30164=CARTESIAN_POINT('Ctrl Pts',(-8.84345834150711,-17.2958453378883,
-330.844772879892)) ;
#30165=CARTESIAN_POINT('Ctrl Pts',(-8.37195213015958,-17.5323647091539,
-330.838045192709)) ;
#30166=CARTESIAN_POINT('Ctrl Pts',(-8.02934256317685,-17.6918922796249,
-330.83316607053)) ;
#30167=CARTESIAN_POINT('Ctrl Pts',(-7.54474823325048,-17.9005538277824,
-330.826359167467)) ;
#30168=CARTESIAN_POINT('Ctrl Pts',(-7.40651686480447,-17.9581892515512,
-330.82442771812)) ;
#30169=CARTESIAN_POINT('Ctrl Pts',(-6.81527791660644,-18.1967178971547,
-330.816221325694)) ;
#30170=CARTESIAN_POINT('Ctrl Pts',(-6.35620850284429,-18.3621123822784,
-330.809990091716)) ;
#30171=CARTESIAN_POINT('Ctrl Pts',(-5.74424953347748,-18.5568873800967,
-330.801933132721)) ;
#30172=CARTESIAN_POINT('Ctrl Pts',(-5.59654524475661,-18.6019663840019,
-330.800006756453)) ;
#30173=CARTESIAN_POINT('Ctrl Pts',(-5.32712333760844,-18.6806938984724,
-330.796526486237)) ;
#30174=CARTESIAN_POINT('Ctrl Pts',(-5.20558514273602,-18.7149258869327,
-330.794968799171)) ;
#30175=CARTESIAN_POINT('Ctrl Pts',(-4.97151285361023,-18.7783972044567,
-330.791992001037)) ;
#30176=CARTESIAN_POINT('Ctrl Pts',(-4.85903298081444,-18.8078159325072,
-330.790571745174)) ;
#30177=CARTESIAN_POINT('Ctrl Pts',(-4.61901284084109,-18.8682954964984,
-330.787561947591)) ;
#30178=CARTESIAN_POINT('Ctrl Pts',(-4.49140806555949,-18.8990769141542,
-330.785974290612)) ;
#30179=CARTESIAN_POINT('Ctrl Pts',(-3.90025969869142,-19.0353512079354,
-330.778672806022)) ;
#30180=CARTESIAN_POINT('Ctrl Pts',(-3.43325378105262,-19.125098462191,-330.77306078346)) ;
#30181=CARTESIAN_POINT('Ctrl Pts',(-2.34524013258419,-19.2930488491088,
-330.760164813077)) ;
#30182=CARTESIAN_POINT('Ctrl Pts',(-1.72280752052367,-19.3585592239145,
-330.752925013063)) ;
#30183=CARTESIAN_POINT('Ctrl Pts',(-0.941296574230398,-19.402817218473,
-330.743602996482)) ;
#30184=CARTESIAN_POINT('Ctrl Pts',(-0.784187582285233,-19.4098017754061,
-330.741716527415)) ;
#30185=CARTESIAN_POINT('Ctrl Pts',(-0.548155794540502,-19.4174245180445,
-330.738853805589)) ;
#30186=CARTESIAN_POINT('Ctrl Pts',(-0.46928548701264,-19.419490745122,-330.737892423873)) ;
#30187=CARTESIAN_POINT('Ctrl Pts',(-0.327535873861351,-19.4223402132059,
-330.736154365708)) ;
#30188=CARTESIAN_POINT('Ctrl Pts',(-0.264661332178073,-19.4232987274662,
-330.735379694964)) ;
#30189=CARTESIAN_POINT('Ctrl Pts',(-0.134559580638513,-19.4246502730836,
-330.733769429841)) ;
#30190=CARTESIAN_POINT('Ctrl Pts',(-0.0673327622802353,-19.4249996344579,
-330.732933396708)) ;
#30191=CARTESIAN_POINT('Ctrl Pts',(-0.00010553887512245,-19.4249999997133,
-330.732093850011)) ;
#30192=CARTESIAN_POINT('Ctrl Pts',(5.03575626651515E-5,-19.4249999999347,
-330.517882160562)) ;
#30193=CARTESIAN_POINT('Ctrl Pts',(-0.109383643921926,-19.4250002836325,
-330.519239321665)) ;
#30194=CARTESIAN_POINT('Ctrl Pts',(-0.218815588222075,-19.4240757949738,
-330.520606794212)) ;
#30195=CARTESIAN_POINT('Ctrl Pts',(-0.401044244614562,-19.420996148449,
-330.522897922524)) ;
#30196=CARTESIAN_POINT('Ctrl Pts',(-0.473847218249506,-19.4193562376763,
-330.523816981607)) ;
#30197=CARTESIAN_POINT('Ctrl Pts',(-0.763832435112605,-19.4111925264556,
-330.52749040625)) ;
#30198=CARTESIAN_POINT('Ctrl Pts',(-0.980907588565217,-19.401434364168,
-330.530268396036)) ;
#30199=CARTESIAN_POINT('Ctrl Pts',(-2.03944657170865,-19.3360389151549,
-330.543889642085)) ;
#30200=CARTESIAN_POINT('Ctrl Pts',(-2.87684738347944,-19.2292876972037,
-330.554852659341)) ;
#30201=CARTESIAN_POINT('Ctrl Pts',(-3.89251083549517,-19.0319627524741,
-330.567875055589)) ;
#30202=CARTESIAN_POINT('Ctrl Pts',(-4.07981718600254,-18.9926917184026,
-330.57026726666)) ;
#30203=CARTESIAN_POINT('Ctrl Pts',(-4.37955302673366,-18.9252098020816,
-330.574079200534)) ;
#30204=CARTESIAN_POINT('Ctrl Pts',(-4.49236330780916,-18.8987492367985,
-330.575510203298)) ;
#30205=CARTESIAN_POINT('Ctrl Pts',(-4.72990659535361,-18.8407844248779,
-330.578515926537)) ;
#30206=CARTESIAN_POINT('Ctrl Pts',(-4.85457708568074,-18.8090471719321,
-330.580089019906)) ;
#30207=CARTESIAN_POINT('Ctrl Pts',(-5.16354214344152,-18.7271177277252,
-330.583977725882)) ;
#30208=CARTESIAN_POINT('Ctrl Pts',(-5.34742914969837,-18.6754412932905,
-330.586283367834)) ;
#30209=CARTESIAN_POINT('Ctrl Pts',(-6.04461305722028,-18.4683750866107,
-330.595002001604)) ;
#30210=CARTESIAN_POINT('Ctrl Pts',(-6.55215884262199,-18.2944647695834,
-330.60129475374)) ;
#30211=CARTESIAN_POINT('Ctrl Pts',(-7.60397983251672,-17.8846646187067,
-330.614484949302)) ;
#30212=CARTESIAN_POINT('Ctrl Pts',(-8.14596864611218,-17.6444021721716,
-330.621368588068)) ;
#30213=CARTESIAN_POINT('Ctrl Pts',(-8.77644848501478,-17.3296610002707,
-330.629831615065)) ;
#30214=CARTESIAN_POINT('Ctrl Pts',(-8.87633772169011,-17.2787102236215,
-330.631186815447)) ;
#30215=CARTESIAN_POINT('Ctrl Pts',(-9.03070414909833,-17.1982802387979,
-330.63330735105)) ;
#30216=CARTESIAN_POINT('Ctrl Pts',(-9.08549102029803,-17.1694004995042,
-330.634065142394)) ;
#30217=CARTESIAN_POINT('Ctrl Pts',(-9.20291603010773,-17.1067829583898,
-330.635701417219)) ;
#30218=CARTESIAN_POINT('Ctrl Pts',(-9.26550881887964,-17.0729620439434,
-330.636581060354)) ;
#30219=CARTESIAN_POINT('Ctrl Pts',(-9.43741154310013,-16.9788536520004,
-330.639015884429)) ;
#30220=CARTESIAN_POINT('Ctrl Pts',(-9.54632825747328,-16.9178552038756,
-330.640579864895)) ;
#30221=CARTESIAN_POINT('Ctrl Pts',(-9.79765324946986,-16.773901607098,-330.64423179819)) ;
#30222=CARTESIAN_POINT('Ctrl Pts',(-9.93960891715943,-16.6901755167978,
-330.646327008174)) ;
#30223=CARTESIAN_POINT('Ctrl Pts',(-10.4721870967643,-16.366853823257,-330.65428898829)) ;
#30224=CARTESIAN_POINT('Ctrl Pts',(-10.8553550838812,-16.1152683074099,
-330.660222740504)) ;
#30225=CARTESIAN_POINT('Ctrl Pts',(-11.3797767304201,-15.7437393804565,
-330.668502957782)) ;
#30226=CARTESIAN_POINT('Ctrl Pts',(-11.5287603961236,-15.6349714395217,
-330.6708746482)) ;
#30227=CARTESIAN_POINT('Ctrl Pts',(-11.9730957657495,-15.3007725488647,
-330.677994615142)) ;
#30228=CARTESIAN_POINT('Ctrl Pts',(-12.2635512886728,-15.0689738763107,
-330.6827107555)) ;
#30229=CARTESIAN_POINT('Ctrl Pts',(-12.6679914644066,-14.7267668430725,
-330.689343109839)) ;
#30230=CARTESIAN_POINT('Ctrl Pts',(-12.7875486623785,-14.6230731617917,
-330.6913125079)) ;
#30231=CARTESIAN_POINT('Ctrl Pts',(-12.9988221246711,-14.4352599934615,
-330.694808338038)) ;
#30232=CARTESIAN_POINT('Ctrl Pts',(-13.0910223209699,-14.3516982391118,
-330.696339412337)) ;
#30233=CARTESIAN_POINT('Ctrl Pts',(-13.2870765208819,-14.1705514621277,
-330.69960749561)) ;
#30234=CARTESIAN_POINT('Ctrl Pts',(-13.390672476077,-14.0726977484564,-330.701342012162)) ;
#30235=CARTESIAN_POINT('Ctrl Pts',(-13.6874134023531,-13.7861612017981,
-330.706335127412)) ;
#30236=CARTESIAN_POINT('Ctrl Pts',(-13.8777130980579,-13.5945800188833,
-330.709567868658)) ;
#30237=CARTESIAN_POINT('Ctrl Pts',(-14.5346164437145,-12.9050811120067,
-330.720873816135)) ;
#30238=CARTESIAN_POINT('Ctrl Pts',(-14.9789182179962,-12.386613789824,-330.728775681188)) ;
#30239=CARTESIAN_POINT('Ctrl Pts',(-15.5962871770699,-11.5842730369867,
-330.7406521795)) ;
#30240=CARTESIAN_POINT('Ctrl Pts',(-15.7908579681024,-11.3176127876404,
-330.744549737181)) ;
#30241=CARTESIAN_POINT('Ctrl Pts',(-16.0349031381681,-10.9645944095316,
-330.749719699498)) ;
#30242=CARTESIAN_POINT('Ctrl Pts',(-16.0906417276774,-10.8826328601742,
-330.750920798574)) ;
#30243=CARTESIAN_POINT('Ctrl Pts',(-16.1827580401535,-10.7449242682418,
-330.752942999139)) ;
#30244=CARTESIAN_POINT('Ctrl Pts',(-16.2194809354834,-10.6894103442735,
-330.753759376281)) ;
#30245=CARTESIAN_POINT('Ctrl Pts',(-16.2990879908049,-10.5677137856019,
-330.755552347349)) ;
#30246=CARTESIAN_POINT('Ctrl Pts',(-16.3418558202475,-10.5014566758946,
-330.756530443555)) ;
#30247=CARTESIAN_POINT('Ctrl Pts',(-16.4736501247837,-10.294522421551,-330.759588850281)) ;
#30248=CARTESIAN_POINT('Ctrl Pts',(-16.5612723386543,-10.1529600952451,
-330.761686198041)) ;
#30249=CARTESIAN_POINT('Ctrl Pts',(-16.7154441866806,-9.89657303695557,
-330.765482103599)) ;
#30250=CARTESIAN_POINT('Ctrl Pts',(-16.7826574781856,-9.78215927861785,
-330.767175124178)) ;
#30251=CARTESIAN_POINT('Ctrl Pts',(-17.1382223352435,-9.16244661736475,
-330.776324293651)) ;
#30252=CARTESIAN_POINT('Ctrl Pts',(-17.4049353997936,-8.64507478365913,
-330.783878532853)) ;
#30253=CARTESIAN_POINT('Ctrl Pts',(-17.8130191564934,-7.7577637368678,-330.796399308548)) ;
#30254=CARTESIAN_POINT('Ctrl Pts',(-17.9670351678522,-7.39406506878113,
-330.801417049817)) ;
#30255=CARTESIAN_POINT('Ctrl Pts',(-18.1674321508323,-6.87752649898721,
-330.808354400557)) ;
#30256=CARTESIAN_POINT('Ctrl Pts',(-18.2231788022412,-6.72842597773595,
-330.810335577701)) ;
#30257=CARTESIAN_POINT('Ctrl Pts',(-18.3192566071755,-6.46149879788646,
-330.813844317712)) ;
#30258=CARTESIAN_POINT('Ctrl Pts',(-18.3602991120824,-6.34393772956422,
-330.8153766548)) ;
#30259=CARTESIAN_POINT('Ctrl Pts',(-18.4456960153687,-6.0915568552642,-330.81863910699)) ;
#30260=CARTESIAN_POINT('Ctrl Pts',(-18.4897089444165,-5.95662904927668,
-330.82036682283)) ;
#30261=CARTESIAN_POINT('Ctrl Pts',(-18.6121069816489,-5.56696752573591,
-330.825311487338)) ;
#30262=CARTESIAN_POINT('Ctrl Pts',(-18.6867334791185,-5.31108708168226,
-330.828503405246)) ;
#30263=CARTESIAN_POINT('Ctrl Pts',(-18.9834646161529,-4.20982401420183,
-330.842048519428)) ;
#30264=CARTESIAN_POINT('Ctrl Pts',(-19.1536387280904,-3.35151597096332,
-330.852077771041)) ;
#30265=CARTESIAN_POINT('Ctrl Pts',(-19.2888465797758,-2.30315448832917,
-330.864625399001)) ;
#30266=CARTESIAN_POINT('Ctrl Pts',(-19.3096908029976,-2.12131182845833,
-330.86681465962)) ;
#30267=CARTESIAN_POINT('Ctrl Pts',(-19.3362182933276,-1.8569132293746,-330.870031354084)) ;
#30268=CARTESIAN_POINT('Ctrl Pts',(-19.3439488482247,-1.77457250128458,
-330.871037838639)) ;
#30269=CARTESIAN_POINT('Ctrl Pts',(-19.3568380500606,-1.62717672532804,
-330.872849775708)) ;
#30270=CARTESIAN_POINT('Ctrl Pts',(-19.3621951373493,-1.5621404642525,-330.873652974005)) ;
#30271=CARTESIAN_POINT('Ctrl Pts',(-19.3743421431742,-1.40499853434457,
-330.875602349452)) ;
#30272=CARTESIAN_POINT('Ctrl Pts',(-19.3808031020424,-1.31286916722493,
-330.876752239382)) ;
#30273=CARTESIAN_POINT('Ctrl Pts',(-19.4034994741604,-0.952414834257095,
-330.881273907144)) ;
#30274=CARTESIAN_POINT('Ctrl Pts',(-19.414821346963,-0.683810967337861,
-330.884692250171)) ;
#30275=CARTESIAN_POINT('Ctrl Pts',(-19.4333941850321,0.185209165867029,
-330.895825645696)) ;
#30276=CARTESIAN_POINT('Ctrl Pts',(-19.4183858938385,0.785750027072752,
-330.903623998144)) ;
#30277=CARTESIAN_POINT('Ctrl Pts',(-19.3489830945429,1.75692650705994,-330.916094149874)) ;
#30278=CARTESIAN_POINT('Ctrl Pts',(-19.3116529470566,2.12837945326687,-330.920832691249)) ;
#30279=CARTESIAN_POINT('Ctrl Pts',(-19.2432337963619,2.65589124783422,-330.927492419551)) ;
#30280=CARTESIAN_POINT('Ctrl Pts',(-19.2208958041448,2.81300015002547,-330.929467301301)) ;
#30281=CARTESIAN_POINT('Ctrl Pts',(-19.1776056359031,3.09282390302031,-330.932969133975)) ;
#30282=CARTESIAN_POINT('Ctrl Pts',(-19.1573941168371,3.2156443087705,-330.934500788558)) ;
#30283=CARTESIAN_POINT('Ctrl Pts',(-19.1115612297677,3.478373320119,-330.937766208512)) ;
#30284=CARTESIAN_POINT('Ctrl Pts',(-19.0855808259822,3.618212016481,-330.939497525196)) ;
#30285=CARTESIAN_POINT('Ctrl Pts',(-19.0061536709267,4.02104000803802,-330.944467797047)) ;
#30286=CARTESIAN_POINT('Ctrl Pts',(-18.948789883894,4.2832233693699,-330.947681286156)) ;
#30287=CARTESIAN_POINT('Ctrl Pts',(-18.7972499771282,4.9130429138484,-330.955373094013)) ;
#30288=CARTESIAN_POINT('Ctrl Pts',(-18.6976973515694,5.27927188342988,-330.95982178649)) ;
#30289=CARTESIAN_POINT('Ctrl Pts',(-18.4082348089666,6.23284267538835,-330.971468881784)) ;
#30290=CARTESIAN_POINT('Ctrl Pts',(-18.2009509578486,6.81445635987414,-330.978630429769)) ;
#30291=CARTESIAN_POINT('Ctrl Pts',(-17.9252345924882,7.48520390493788,-330.987347795917)) ;
#30292=CARTESIAN_POINT('Ctrl Pts',(-17.8832982708335,7.58485040080098,-330.988655402369)) ;
#30293=CARTESIAN_POINT('Ctrl Pts',(-17.8139152370466,7.74593934730319,-330.990793320313)) ;
#30294=CARTESIAN_POINT('Ctrl Pts',(-17.7869772125323,7.80759848444304,-330.991617420497)) ;
#30295=CARTESIAN_POINT('Ctrl Pts',(-17.7294479002143,7.93743573431328,-330.993366028853)) ;
#30296=CARTESIAN_POINT('Ctrl Pts',(-17.6987825120908,8.00557970757228,-330.994291410488)) ;
#30297=CARTESIAN_POINT('Ctrl Pts',(-17.6081667408616,8.20387853485462,-330.997004737687)) ;
#30298=CARTESIAN_POINT('Ctrl Pts',(-17.5471684667196,8.33354892509288,-330.998804862371)) ;
#30299=CARTESIAN_POINT('Ctrl Pts',(-17.397463177574,8.64286038531919,-331.003150931144)) ;
#30300=CARTESIAN_POINT('Ctrl Pts',(-17.3074008334412,8.82182729780902,-331.005708189282)) ;
#30301=CARTESIAN_POINT('Ctrl Pts',(-16.8699117524567,9.65868528235885,-331.017820176187)) ;
#30302=CARTESIAN_POINT('Ctrl Pts',(-16.4876420828482,10.2976594043948,-331.027496797488)) ;
#30303=CARTESIAN_POINT('Ctrl Pts',(-15.924123175725,11.1274453814007,-331.040228694641)) ;
#30304=CARTESIAN_POINT('Ctrl Pts',(-15.7743053148953,11.3388285046095,-331.043490531975)) ;
#30305=CARTESIAN_POINT('Ctrl Pts',(-15.5358784895606,11.6613582105786,-331.048490760577)) ;
#30306=CARTESIAN_POINT('Ctrl Pts',(-15.4502026991812,11.7746351273239,-331.050251590252)) ;
#30307=CARTESIAN_POINT('Ctrl Pts',(-15.2947309151183,11.9755744748375,-331.05338363624)) ;
#30308=CARTESIAN_POINT('Ctrl Pts',(-15.2254041235981,12.0635917982819,-331.054758573104)) ;
#30309=CARTESIAN_POINT('Ctrl Pts',(-15.0585477967697,12.2717030686127,-331.058017300648)) ;
#30310=CARTESIAN_POINT('Ctrl Pts',(-14.9603373874767,12.391241394261,-331.059895347255)) ;
#30311=CARTESIAN_POINT('Ctrl Pts',(-14.6325596356343,12.7806233341624,-331.066037554248)) ;
#30312=CARTESIAN_POINT('Ctrl Pts',(-14.3970377085091,13.0453608723597,-331.070252134838)) ;
#30313=CARTESIAN_POINT('Ctrl Pts',(-13.7090266865031,13.777377372025,-331.082095264247)) ;
#30314=CARTESIAN_POINT('Ctrl Pts',(-13.2401313112787,14.2285789934572,-331.089615235417)) ;
#30315=CARTESIAN_POINT('Ctrl Pts',(-12.7064547124593,14.6928515837352,-331.097953515442)) ;
#30316=CARTESIAN_POINT('Ctrl Pts',(-12.6632524946571,14.7301023511176,-331.098627143809)) ;
#30317=CARTESIAN_POINT('Ctrl Pts',(-12.4617243056367,14.9023265668085,-331.101764427376)) ;
#30318=CARTESIAN_POINT('Ctrl Pts',(-12.3014007019916,15.0349409799813,-331.104245770373)) ;
#30319=CARTESIAN_POINT('Ctrl Pts',(-12.0713018612641,15.2191264893781,-331.107807888769)) ;
#30320=CARTESIAN_POINT('Ctrl Pts',(-12.0032637410207,15.2728451593789,-331.108861299042)) ;
#30321=CARTESIAN_POINT('Ctrl Pts',(-11.8830645250443,15.366447655184,-331.110724564635)) ;
#30322=CARTESIAN_POINT('Ctrl Pts',(-11.8310566653302,15.4065257023405,-331.111531616058)) ;
#30323=CARTESIAN_POINT('Ctrl Pts',(-11.7100692391109,15.4987865468811,-331.113411205779)) ;
#30324=CARTESIAN_POINT('Ctrl Pts',(-11.640942540443,15.5507737027415,-331.114486479666)) ;
#30325=CARTESIAN_POINT('Ctrl Pts',(-11.3967472830981,15.7318815403067,-331.118286277072)) ;
#30326=CARTESIAN_POINT('Ctrl Pts',(-11.2198593801426,15.85852138844,-331.121040936249)) ;
#30327=CARTESIAN_POINT('Ctrl Pts',(-10.7212332974238,16.2029848856168,-331.128772615892)) ;
#30328=CARTESIAN_POINT('Ctrl Pts',(-10.3950316962106,16.414167001091,-331.133791522867)) ;
#30329=CARTESIAN_POINT('Ctrl Pts',(-9.88495471592185,16.7230824041626,-331.141484406092)) ;
#30330=CARTESIAN_POINT('Ctrl Pts',(-9.70547547893952,16.8278804557197,-331.144163293726)) ;
#30331=CARTESIAN_POINT('Ctrl Pts',(-9.1625393651518,17.1333252785833,-331.152163877547)) ;
#30332=CARTESIAN_POINT('Ctrl Pts',(-8.79429678800166,17.3252217356206,-331.157451926281)) ;
#30333=CARTESIAN_POINT('Ctrl Pts',(-8.28120864010469,17.5720230164607,-331.164594667441)) ;
#30334=CARTESIAN_POINT('Ctrl Pts',(-8.14143750739785,17.6372164706472,-331.16651845144)) ;
#30335=CARTESIAN_POINT('Ctrl Pts',(-7.88588942441923,17.7527266713724,-331.169995561824)) ;
#30336=CARTESIAN_POINT('Ctrl Pts',(-7.77037003803242,17.8035924971271,-331.171552656667)) ;
#30337=CARTESIAN_POINT('Ctrl Pts',(-7.53240447057082,17.9056168790374,-331.174730541355)) ;
#30338=CARTESIAN_POINT('Ctrl Pts',(-7.4099132463587,17.9566538827404,-331.176350414048)) ;
#30339=CARTESIAN_POINT('Ctrl Pts',(-7.08857207073964,18.0866954036499,-331.180560031698)) ;
#30340=CARTESIAN_POINT('Ctrl Pts',(-6.88892274665502,18.1636766164957,-331.183135775338)) ;
#30341=CARTESIAN_POINT('Ctrl Pts',(-6.55348934718931,18.2866875529465,-331.187404742255)) ;
#30342=CARTESIAN_POINT('Ctrl Pts',(-6.41839437260853,18.3345405727428,-331.189108467082)) ;
#30343=CARTESIAN_POINT('Ctrl Pts',(-5.84735609148978,18.5297274377507,-331.196252665333)) ;
#30344=CARTESIAN_POINT('Ctrl Pts',(-5.40677866210083,18.6630414739857,-331.201621130441)) ;
#30345=CARTESIAN_POINT('Ctrl Pts',(-4.88664933724325,18.8004611273291,-331.207905198598)) ;
#30346=CARTESIAN_POINT('Ctrl Pts',(-4.81129599690855,18.8198860563384,-331.208814409189)) ;
#30347=CARTESIAN_POINT('Ctrl Pts',(-4.35714428029066,18.9340535098657,-331.214290652005)) ;
#30348=CARTESIAN_POINT('Ctrl Pts',(-3.97567707510888,19.0178095230492,-331.218873863164)) ;
#30349=CARTESIAN_POINT('Ctrl Pts',(-3.47596619974279,19.1118343350458,-331.22497307401)) ;
#30350=CARTESIAN_POINT('Ctrl Pts',(-3.35978949627325,19.1325995921073,-331.226397870683)) ;
#30351=CARTESIAN_POINT('Ctrl Pts',(-3.1813651293406,19.1628156478985,-331.228600889527)) ;
#30352=CARTESIAN_POINT('Ctrl Pts',(-3.11924863708553,19.1730246849707,-331.229370593746)) ;
#30353=CARTESIAN_POINT('Ctrl Pts',(-2.98816267053531,19.1939151711428,-331.231001667201)) ;
#30354=CARTESIAN_POINT('Ctrl Pts',(-2.91918308001032,19.2045272230485,-331.231863946603)) ;
#30355=CARTESIAN_POINT('Ctrl Pts',(-2.73343258707251,19.2320798011709,-331.234195223227)) ;
#30356=CARTESIAN_POINT('Ctrl Pts',(-2.61656207658776,19.2483284995023,-331.23567187278)) ;
#30357=CARTESIAN_POINT('Ctrl Pts',(-2.41937249954605,19.2739149766195,-331.238175863511)) ;
#30358=CARTESIAN_POINT('Ctrl Pts',(-2.3391299330862,19.2838179040819,-331.239198301804)) ;
#30359=CARTESIAN_POINT('Ctrl Pts',(-2.1259891498276,19.3087721816363,-331.241921423551)) ;
#30360=CARTESIAN_POINT('Ctrl Pts',(-1.99299336661796,19.3229524249205,-331.243628118754)) ;
#30361=CARTESIAN_POINT('Ctrl Pts',(-1.27078286024051,19.3924201846598,-331.252920262184)) ;
#30362=CARTESIAN_POINT('Ctrl Pts',(-0.679421988398216,19.4221326613697,
-331.260605808213)) ;
#30363=CARTESIAN_POINT('Ctrl Pts',(0.294082953597015,19.4265243163244,-331.273079881172)) ;
#30364=CARTESIAN_POINT('Ctrl Pts',(0.675763093308313,19.4169945463091,-331.277928199104)) ;
#30365=CARTESIAN_POINT('Ctrl Pts',(1.21613940107922,19.3875490383569,-331.284704770253)) ;
#30366=CARTESIAN_POINT('Ctrl Pts',(1.37525128023383,19.3769124674497,-331.286689602766)) ;
#30367=CARTESIAN_POINT('Ctrl Pts',(1.6583697248742,19.3544812948215,-331.290202361248)) ;
#30368=CARTESIAN_POINT('Ctrl Pts',(1.78242778168078,19.3434507672801,-331.291735102424)) ;
#30369=CARTESIAN_POINT('Ctrl Pts',(2.04743223517123,19.3173170485515,-331.294995874371)) ;
#30370=CARTESIAN_POINT('Ctrl Pts',(2.18833682487586,19.3018625712689,-331.296721534203)) ;
#30371=CARTESIAN_POINT('Ctrl Pts',(2.59260769684783,19.2530382263045,-331.301651623129)) ;
#30372=CARTESIAN_POINT('Ctrl Pts',(2.85547576797671,19.2158100044674,-331.304831267606)) ;
#30373=CARTESIAN_POINT('Ctrl Pts',(3.31312860541289,19.1413972008253,-331.31033834568)) ;
#30374=CARTESIAN_POINT('Ctrl Pts',(3.50826058420085,19.1065961317247,-331.312677366791)) ;
#30375=CARTESIAN_POINT('Ctrl Pts',(4.14713309221299,18.9825384146899,-331.320325578312)) ;
#30376=CARTESIAN_POINT('Ctrl Pts',(4.58828883765788,18.8807595941433,-331.325588122022)) ;
#30377=CARTESIAN_POINT('Ctrl Pts',(5.37854189113753,18.6691055552241,-331.335171335634)) ;
#30378=CARTESIAN_POINT('Ctrl Pts',(5.72885818746038,18.5646006623749,-331.339477409204)) ;
#30379=CARTESIAN_POINT('Ctrl Pts',(6.17160663977121,18.4187954281179,-331.345090650365)) ;
#30380=CARTESIAN_POINT('Ctrl Pts',(6.26695107226405,18.3865733011086,-331.346309800873)) ;
#30381=CARTESIAN_POINT('Ctrl Pts',(6.42512708956755,18.3317436429507,-331.348352636374)) ;
#30382=CARTESIAN_POINT('Ctrl Pts',(6.48810028677848,18.3095504528684,-331.34917136159)) ;
#30383=CARTESIAN_POINT('Ctrl Pts',(6.62447888903119,18.2606955902884,-331.3509570715)) ;
#30384=CARTESIAN_POINT('Ctrl Pts',(6.69784030912312,18.2339150805707,-331.351925427461)) ;
#30385=CARTESIAN_POINT('Ctrl Pts',(6.92288414697814,18.1502216596197,-331.354917680029)) ;
#30386=CARTESIAN_POINT('Ctrl Pts',(7.07401754044474,18.0918530533116,-331.356957623321)) ;
#30387=CARTESIAN_POINT('Ctrl Pts',(7.34265980990761,17.9842209029808,-331.360627456576)) ;
#30388=CARTESIAN_POINT('Ctrl Pts',(7.46044775047311,17.9356787963735,-331.362251767212)) ;
#30389=CARTESIAN_POINT('Ctrl Pts',(8.06999595128347,17.6774316557039,-331.370723279508)) ;
#30390=CARTESIAN_POINT('Ctrl Pts',(8.55342321120576,17.4486497086714,-331.377658905016)) ;
#30391=CARTESIAN_POINT('Ctrl Pts',(9.41813592380486,16.9948423548979,-331.390206336027)) ;
#30392=CARTESIAN_POINT('Ctrl Pts',(9.8023523837135,16.7761688260788,-331.395837017219)) ;
#30393=CARTESIAN_POINT('Ctrl Pts',(10.3182349396405,16.4587807320057,-331.40342784363)) ;
#30394=CARTESIAN_POINT('Ctrl Pts',(10.4566037209068,16.3712209130232,-331.405467394155)) ;
#30395=CARTESIAN_POINT('Ctrl Pts',(10.6986374708936,16.2137414092363,-331.409040918764)) ;
#30396=CARTESIAN_POINT('Ctrl Pts',(10.8027653145149,16.1445506542111,-331.410580323744)) ;
#30397=CARTESIAN_POINT('Ctrl Pts',(11.0215371979506,15.9961171278713,-331.413819361293)) ;
#30398=CARTESIAN_POINT('Ctrl Pts',(11.1360111170614,15.916636008884,-331.415517017434)) ;
#30399=CARTESIAN_POINT('Ctrl Pts',(11.4545901149544,15.6903220085739,-331.420251574801)) ;
#30400=CARTESIAN_POINT('Ctrl Pts',(11.6567141952946,15.5407481779227,-331.423266881358)) ;
#30401=CARTESIAN_POINT('Ctrl Pts',(12.1267959399637,15.1785511448863,-331.430325725985)) ;
#30402=CARTESIAN_POINT('Ctrl Pts',(12.3921539857327,14.9626907564532,-331.434346521763)) ;
#30403=CARTESIAN_POINT('Ctrl Pts',(13.1570025657176,14.3062011665578,-331.446142919059)) ;
#30404=CARTESIAN_POINT('Ctrl Pts',(13.6396895262847,13.8467675469215,-331.453848006321)) ;
#30405=CARTESIAN_POINT('Ctrl Pts',(14.1780523753486,13.2788198189066,-331.463237489596)) ;
#30406=CARTESIAN_POINT('Ctrl Pts',(14.2575165484111,13.1934622731863,-331.464645771229)) ;
#30407=CARTESIAN_POINT('Ctrl Pts',(14.3785177479979,13.0611172621129,-331.466829156981)) ;
#30408=CARTESIAN_POINT('Ctrl Pts',(14.4206039870436,13.0146355078446,-331.467595977805)) ;
#30409=CARTESIAN_POINT('Ctrl Pts',(14.5092485848617,12.9157749124534,-331.469227814815)) ;
#30410=CARTESIAN_POINT('Ctrl Pts',(14.5557500237847,12.8633462717531,-331.470093798269)) ;
#30411=CARTESIAN_POINT('Ctrl Pts',(14.6807550183832,12.720861986213,-331.472447370338)) ;
#30412=CARTESIAN_POINT('Ctrl Pts',(14.7587131279826,12.6303319166457,-331.473942855147)) ;
#30413=CARTESIAN_POINT('Ctrl Pts',(15.0984885510165,12.2283209781896,-331.480573149272)) ;
#30414=CARTESIAN_POINT('Ctrl Pts',(15.3513163869708,11.9093775960655,-331.485803614236)) ;
#30415=CARTESIAN_POINT('Ctrl Pts',(16.033542328605,10.9908903366001,-331.500554969905)) ;
#30416=CARTESIAN_POINT('Ctrl Pts',(16.4390966795643,10.3745004117369,-331.510079911123)) ;
#30417=CARTESIAN_POINT('Ctrl Pts',(16.897800213983,9.58262067576621,-331.521573823901)) ;
#30418=CARTESIAN_POINT('Ctrl Pts',(16.9848485366414,9.4274700428485,-331.523793649394)) ;
#30419=CARTESIAN_POINT('Ctrl Pts',(17.1301451745573,9.15995425435194,-331.527565858801)) ;
#30420=CARTESIAN_POINT('Ctrl Pts',(17.1894489665443,9.04817550223545,-331.529125840211)) ;
#30421=CARTESIAN_POINT('Ctrl Pts',(17.3096813273314,8.81610667843185,-331.532331734902)) ;
#30422=CARTESIAN_POINT('Ctrl Pts',(17.3704581071726,8.69574550137857,-331.533976483134)) ;
#30423=CARTESIAN_POINT('Ctrl Pts',(17.5296641065612,8.37212635753797,-331.538352629366)) ;
#30424=CARTESIAN_POINT('Ctrl Pts',(17.625810187505,8.16776829460154,-331.541067762122)) ;
#30425=CARTESIAN_POINT('Ctrl Pts',(17.8375099440627,7.69664565295041,-331.54722982063)) ;
#30426=CARTESIAN_POINT('Ctrl Pts',(17.9506825314833,7.42887019106929,-331.550661979062)) ;
#30427=CARTESIAN_POINT('Ctrl Pts',(18.2133268869269,6.76634635651274,-331.559028852291)) ;
#30428=CARTESIAN_POINT('Ctrl Pts',(18.3560242844578,6.36907305596773,-331.563938108192)) ;
#30429=CARTESIAN_POINT('Ctrl Pts',(18.5977918864768,5.62013973394375,-331.573155077109)) ;
#30430=CARTESIAN_POINT('Ctrl Pts',(18.700103592785,5.26972087544843,-331.577453234272)) ;
#30431=CARTESIAN_POINT('Ctrl Pts',(18.8187032720011,4.81640576130231,-331.583091690668)) ;
#30432=CARTESIAN_POINT('Ctrl Pts',(18.8441222778304,4.71597421879959,-331.584345860284)) ;
#30433=CARTESIAN_POINT('Ctrl Pts',(18.8845487659721,4.55070014301087,-331.586421144224)) ;
#30434=CARTESIAN_POINT('Ctrl Pts',(18.9000285810633,4.48597520402972,-331.587236758795)) ;
#30435=CARTESIAN_POINT('Ctrl Pts',(18.9325746034242,4.3467329991501,-331.588998506909)) ;
#30436=CARTESIAN_POINT('Ctrl Pts',(18.9495341267605,4.27219208832658,-331.589945823497)) ;
#30437=CARTESIAN_POINT('Ctrl Pts',(18.9990398123436,4.04850761125286,-331.592799053409)) ;
#30438=CARTESIAN_POINT('Ctrl Pts',(19.0302683426821,3.89907865454126,-331.594719023881)) ;
#30439=CARTESIAN_POINT('Ctrl Pts',(19.1021332306195,3.53375006641528,-331.599434449502)) ;
#30440=CARTESIAN_POINT('Ctrl Pts',(19.1408746532084,3.31749917776198,-331.602243717838)) ;
#30441=CARTESIAN_POINT('Ctrl Pts',(19.2747221437745,2.48971750031321,-331.613015256119)) ;
#30442=CARTESIAN_POINT('Ctrl Pts',(19.3442535973299,1.87442326248503,-331.621047414326)) ;
#30443=CARTESIAN_POINT('Ctrl Pts',(19.4051245780302,0.935624312395659,-331.63305023746)) ;
#30444=CARTESIAN_POINT('Ctrl Pts',(19.4179648412124,0.613917664051277,-331.637121206606)) ;
#30445=CARTESIAN_POINT('Ctrl Pts',(19.4250662502585,0.141622268101417,-331.643022336498)) ;
#30446=CARTESIAN_POINT('Ctrl Pts',(19.4255805070409,-0.00881706035484106,
-331.644890966908)) ;
#30447=CARTESIAN_POINT('Ctrl Pts',(19.4233313279023,-0.283162925531712,
-331.648278481003)) ;
#30448=CARTESIAN_POINT('Ctrl Pts',(19.4211296882431,-0.407066081420953,
-331.649800890658)) ;
#30449=CARTESIAN_POINT('Ctrl Pts',(19.4136203739906,-0.68169974136198,-331.653159362784)) ;
#30450=CARTESIAN_POINT('Ctrl Pts',(19.4077425197806,-0.832406708846909,
-331.654991652664)) ;
#30451=CARTESIAN_POINT('Ctrl Pts',(19.3836808742657,-1.30726358108212,-331.660734603511)) ;
#30452=CARTESIAN_POINT('Ctrl Pts',(19.3591257274906,-1.63103464049096,-331.664604863635)) ;
#30453=CARTESIAN_POINT('Ctrl Pts',(19.2726884669947,-2.48594464710716,-331.674756787145)) ;
#30454=CARTESIAN_POINT('Ctrl Pts',(19.1969731522516,-3.01540431053611,-331.680970272482)) ;
#30455=CARTESIAN_POINT('Ctrl Pts',(19.0337967053702,-3.89553267246137,-331.691446789089)) ;
#30456=CARTESIAN_POINT('Ctrl Pts',(18.9582229621502,-4.24810226674831,-331.695685918897)) ;
#30457=CARTESIAN_POINT('Ctrl Pts',(18.8452227867904,-4.71188446832313,-331.701413104294)) ;
#30458=CARTESIAN_POINT('Ctrl Pts',(18.8165397460758,-4.82515378529315,-331.702824029085)) ;
#30459=CARTESIAN_POINT('Ctrl Pts',(18.7708862554957,-4.99883895135747,-331.705010554843)) ;
#30460=CARTESIAN_POINT('Ctrl Pts',(18.7546420560114,-5.05944295533292,-331.70577783511)) ;
#30461=CARTESIAN_POINT('Ctrl Pts',(18.7196458418115,-5.18752243341876,-331.707409531894)) ;
#30462=CARTESIAN_POINT('Ctrl Pts',(18.7008219816499,-5.25497731923986,-331.708274906458)) ;
#30463=CARTESIAN_POINT('Ctrl Pts',(18.6489665552764,-5.43699239445489,-331.710624823637)) ;
#30464=CARTESIAN_POINT('Ctrl Pts',(18.6152443889123,-5.55135264194645,-331.712117222362)) ;
#30465=CARTESIAN_POINT('Ctrl Pts',(18.5565463371486,-5.7438612802859,-331.714652236239)) ;
#30466=CARTESIAN_POINT('Ctrl Pts',(18.5321242968731,-5.82217514325223,-331.715689907923)) ;
#30467=CARTESIAN_POINT('Ctrl Pts',(18.3470665836207,-6.40263425173374,-331.723423153028)) ;
#30468=CARTESIAN_POINT('Ctrl Pts',(18.166543293511,-6.89820861068696,-331.730253415421)) ;
#30469=CARTESIAN_POINT('Ctrl Pts',(17.7560341800969,-7.89677581851751,-331.744169610642)) ;
#30470=CARTESIAN_POINT('Ctrl Pts',(17.5242809523818,-8.39853550809977,-331.751244501611)) ;
#30471=CARTESIAN_POINT('Ctrl Pts',(17.2010805163503,-9.02646678313865,-331.760103505472)) ;
#30472=CARTESIAN_POINT('Ctrl Pts',(17.1290824203861,-9.16235826844501,-331.762021641249)) ;
#30473=CARTESIAN_POINT('Ctrl Pts',(16.9951124918703,-9.40811793995196,-331.765491871602)) ;
#30474=CARTESIAN_POINT('Ctrl Pts',(16.9336696213793,-9.51826480963443,-331.767047680967)) ;
#30475=CARTESIAN_POINT('Ctrl Pts',(16.8053081033755,-9.74319742647594,-331.770226222535)) ;
#30476=CARTESIAN_POINT('Ctrl Pts',(16.738275665949,-9.85791074860768,-331.771848003521)) ;
#30477=CARTESIAN_POINT('Ctrl Pts',(16.5597650232949,-10.1563269993446,-331.776070417144)) ;
#30478=CARTESIAN_POINT('Ctrl Pts',(16.4464062461246,-10.3388837669153,-331.778656878971)) ;
#30479=CARTESIAN_POINT('Ctrl Pts',(16.2519482638245,-10.6407517504064,-331.782946859227)) ;
#30480=CARTESIAN_POINT('Ctrl Pts',(16.172506917948,-10.7611077601991,-331.784660916384)) ;
#30481=CARTESIAN_POINT('Ctrl Pts',(15.8312171286155,-11.2658556770832,-331.791872992881)) ;
#30482=CARTESIAN_POINT('Ctrl Pts',(15.5569478501701,-11.6416628477102,-331.797297582334)) ;
#30483=CARTESIAN_POINT('Ctrl Pts',(15.2041539933649,-12.0903054840791,-331.803964756729)) ;
#30484=CARTESIAN_POINT('Ctrl Pts',(15.1381763320924,-12.1728140823866,-331.805199370214)) ;
#30485=CARTESIAN_POINT('Ctrl Pts',(14.8459048393145,-12.5322638751701,-331.810622069613)) ;
#30486=CARTESIAN_POINT('Ctrl Pts',(14.612661027665,-12.8034630071606,-331.814828187538)) ;
#30487=CARTESIAN_POINT('Ctrl Pts',(14.2936007362832,-13.1543607239344,-331.820518624368)) ;
#30488=CARTESIAN_POINT('Ctrl Pts',(14.2143615330848,-13.2399454006237,-331.821927064301)) ;
#30489=CARTESIAN_POINT('Ctrl Pts',(14.0913424553331,-13.3704384694254,-331.824110638086)) ;
#30490=CARTESIAN_POINT('Ctrl Pts',(14.048107783899,-13.4158572122377,-331.824877486402)) ;
#30491=CARTESIAN_POINT('Ctrl Pts',(13.9716475714101,-13.4954050606076,-331.826233460196)) ;
#30492=CARTESIAN_POINT('Ctrl Pts',(13.9385150065128,-13.5296227964357,-331.826821000509)) ;
#30493=CARTESIAN_POINT('Ctrl Pts',(13.8606085807449,-13.609490930354,-331.828202022283)) ;
#30494=CARTESIAN_POINT('Ctrl Pts',(13.8157344951193,-13.6550428033593,-331.828997109471)) ;
#30495=CARTESIAN_POINT('Ctrl Pts',(13.7692616165892,-13.7017540239607,-331.82981972534)) ;
#30496=CARTESIAN_POINT('Ctrl Pts',(13.7678866789893,-13.7031355971437,-331.829844062378)) ;
#30497=CARTESIAN_POINT('Ctrl Pts',(13.7650823617773,-13.7059526001323,-331.829893698622)) ;
#30498=CARTESIAN_POINT('Ctrl Pts',(13.7636529655195,-13.7073880133427,-331.829918998064)) ;
#30499=CARTESIAN_POINT('Ctrl Pts',(13.7607365431826,-13.7103157960541,-331.829970615335)) ;
#30500=CARTESIAN_POINT('Ctrl Pts',(13.759249498805,-13.7118081472885,-331.829996933423)) ;
#30501=CARTESIAN_POINT('Ctrl Pts',(13.7562143858257,-13.7148531008645,-331.830050647834)) ;
#30502=CARTESIAN_POINT('Ctrl Pts',(13.7546662970794,-13.716405683089,-331.830078044441)) ;
#30503=CARTESIAN_POINT('Ctrl Pts',(13.7515054797994,-13.7195746017318,-331.830133979621)) ;
#30504=CARTESIAN_POINT('Ctrl Pts',(13.7498927290853,-13.7211909159549,-331.830162518506)) ;
#30505=CARTESIAN_POINT('Ctrl Pts',(13.7465987356688,-13.7244910237956,-331.830220806126)) ;
#30506=CARTESIAN_POINT('Ctrl Pts',(13.7449174684897,-13.7261747929328,-331.830250555202)) ;
#30507=CARTESIAN_POINT('Ctrl Pts',(13.7414823366226,-13.7296137727576,-331.830311335531)) ;
#30508=CARTESIAN_POINT('Ctrl Pts',(13.7397284448924,-13.7313689564231,-331.83034236716)) ;
#30509=CARTESIAN_POINT('Ctrl Pts',(13.7361436871001,-13.7349549803189,-331.830405789673)) ;
#30510=CARTESIAN_POINT('Ctrl Pts',(13.7343127911914,-13.7367857906339,-331.83043818097)) ;
#30511=CARTESIAN_POINT('Ctrl Pts',(13.7318804184366,-13.7392170772611,-331.830481211385)) ;
#30512=CARTESIAN_POINT('Ctrl Pts',(13.7312792681265,-13.7398178802729,-331.83049184601)) ;
#30513=CARTESIAN_POINT('Ctrl Pts',(13.7300057996842,-13.741090445955,-331.83051437392)) ;
#30514=CARTESIAN_POINT('Ctrl Pts',(13.7293334717162,-13.7417621987025,-331.830526267341)) ;
#30515=CARTESIAN_POINT('Ctrl Pts',(13.727908788006,-13.7431854545801,-331.830551469452)) ;
#30516=CARTESIAN_POINT('Ctrl Pts',(13.7271564198459,-13.7439369452817,-331.830564778311)) ;
#30517=CARTESIAN_POINT('Ctrl Pts',(13.7255616016073,-13.7455296419539,-331.830592988992)) ;
#30518=CARTESIAN_POINT('Ctrl Pts',(13.724719135905,-13.7463708322551,-331.830607891027)) ;
#30519=CARTESIAN_POINT('Ctrl Pts',(13.7229326966182,-13.7481542391314,-331.830639489967)) ;
#30520=CARTESIAN_POINT('Ctrl Pts',(13.7219887032735,-13.7490964359878,-331.830656187142)) ;
#30521=CARTESIAN_POINT('Ctrl Pts',(13.7199862039139,-13.7510947127911,-331.830691606132)) ;
#30522=CARTESIAN_POINT('Ctrl Pts',(13.7189276730188,-13.7521507677242,-331.830710328285)) ;
#30523=CARTESIAN_POINT('Ctrl Pts',(13.7166812751135,-13.7543913937036,-331.830750059085)) ;
#30524=CARTESIAN_POINT('Ctrl Pts',(13.7154933765718,-13.7555759331062,-331.83077106816)) ;
#30525=CARTESIAN_POINT('Ctrl Pts',(13.7129713221462,-13.7580902041727,-331.83081567165)) ;
#30526=CARTESIAN_POINT('Ctrl Pts',(13.7116371262557,-13.7594198956949,-331.830839266607)) ;
#30527=CARTESIAN_POINT('Ctrl Pts',(13.7088031344191,-13.7622434981691,-331.830889383391)) ;
#30528=CARTESIAN_POINT('Ctrl Pts',(13.7073032876514,-13.7637373580543,-331.830915905903)) ;
#30529=CARTESIAN_POINT('Ctrl Pts',(13.7041158552415,-13.7669110295604,-331.830972268592)) ;
#30530=CARTESIAN_POINT('Ctrl Pts',(13.7024282048685,-13.7685907761156,-331.831002109636)) ;
#30531=CARTESIAN_POINT('Ctrl Pts',(13.6988397977451,-13.7721610643623,-331.831065557031)) ;
#30532=CARTESIAN_POINT('Ctrl Pts',(13.6969389584011,-13.7740515229491,-331.831099164484)) ;
#30533=CARTESIAN_POINT('Ctrl Pts',(13.692895080019,-13.7780716522924,-331.831170657896)) ;
#30534=CARTESIAN_POINT('Ctrl Pts',(13.6907519353816,-13.7802012166716,-331.831208545256)) ;
#30535=CARTESIAN_POINT('Ctrl Pts',(13.6861900592354,-13.7847320713513,-331.831289187172)) ;
#30536=CARTESIAN_POINT('Ctrl Pts',(13.683771192387,-13.7871332252523,-331.831331943514)) ;
#30537=CARTESIAN_POINT('Ctrl Pts',(13.6786195459683,-13.7922444558256,-331.831422998825)) ;
#30538=CARTESIAN_POINT('Ctrl Pts',(13.6758865927008,-13.7949543571621,-331.83147130007)) ;
#30539=CARTESIAN_POINT('Ctrl Pts',(13.6700627845725,-13.8007256110362,-331.831574219964)) ;
#30540=CARTESIAN_POINT('Ctrl Pts',(13.6669717063328,-13.8037867378325,-331.831628841517)) ;
#30541=CARTESIAN_POINT('Ctrl Pts',(13.6603811915282,-13.8103090091323,-331.831745290105)) ;
#30542=CARTESIAN_POINT('Ctrl Pts',(13.656881467316,-13.8137698624688,-331.831807120845)) ;
#30543=CARTESIAN_POINT('Ctrl Pts',(13.64941585599,-13.821146944279,-331.831939004371)) ;
#30544=CARTESIAN_POINT('Ctrl Pts',(13.6454495979948,-13.8250627967355,-331.832009061882)) ;
#30545=CARTESIAN_POINT('Ctrl Pts',(13.6369848234021,-13.8334128046799,-331.83215856017)) ;
#30546=CARTESIAN_POINT('Ctrl Pts',(13.6324858282832,-13.8378464740736,-331.83223800697)) ;
#30547=CARTESIAN_POINT('Ctrl Pts',(13.5248819640244,-13.9437845153581,-331.834137890175)) ;
#30548=CARTESIAN_POINT('Ctrl Pts',(13.4206484766666,-14.0441358984069,-331.835972293926)) ;
#30549=CARTESIAN_POINT('Ctrl Pts',(13.0571938880751,-14.3863123139277,-331.842334198098)) ;
#30550=CARTESIAN_POINT('Ctrl Pts',(12.7924806054615,-14.6222000338135,-331.846907147341)) ;
#30551=CARTESIAN_POINT('Ctrl Pts',(12.0368699259241,-15.2592974549705,-331.859658796925)) ;
#30552=CARTESIAN_POINT('Ctrl Pts',(11.5325684342379,-15.6439210804992,-331.86782089299)) ;
#30553=CARTESIAN_POINT('Ctrl Pts',(10.8557137067247,-16.1096040968912,-331.878155817881)) ;
#30554=CARTESIAN_POINT('Ctrl Pts',(10.6995260174173,-16.2137598168998,-331.880501359426)) ;
#30555=CARTESIAN_POINT('Ctrl Pts',(10.4353333422919,-16.3844599024988,-331.884402626645)) ;
#30556=CARTESIAN_POINT('Ctrl Pts',(10.3281421015145,-16.4522396360513,-331.885967651436)) ;
#30557=CARTESIAN_POINT('Ctrl Pts',(10.1280936850837,-16.5760097265774,-331.888855868632)) ;
#30558=CARTESIAN_POINT('Ctrl Pts',(10.0354165986346,-16.6322816796704,-331.890181159595)) ;
#30559=CARTESIAN_POINT('Ctrl Pts',(9.80015059935628,-16.772448889877,-331.893514190319)) ;
#30560=CARTESIAN_POINT('Ctrl Pts',(9.65695198137309,-16.8553039742803,-331.895514152812)) ;
#30561=CARTESIAN_POINT('Ctrl Pts',(9.33334597599243,-17.0370654714374,-331.899973650054)) ;
#30562=CARTESIAN_POINT('Ctrl Pts',(9.15239033309964,-17.1349554519541,-331.902426150856)) ;
#30563=CARTESIAN_POINT('Ctrl Pts',(8.58442224059697,-17.4306396560204,-331.910012974524)) ;
#30564=CARTESIAN_POINT('Ctrl Pts',(8.1923038977197,-17.6183331030163,-331.915090653946)) ;
#30565=CARTESIAN_POINT('Ctrl Pts',(7.66602066844943,-17.8488750695102,-331.92180113646)) ;
#30566=CARTESIAN_POINT('Ctrl Pts',(7.53721722725401,-17.9036468518039,-331.923435695687)) ;
#30567=CARTESIAN_POINT('Ctrl Pts',(7.34270465750832,-17.9838893707481,-331.925897699522)) ;
#30568=CARTESIAN_POINT('Ctrl Pts',(7.27743047854187,-18.0104023889908,-331.926722822383)) ;
#30569=CARTESIAN_POINT('Ctrl Pts',(6.90069431434913,-18.1610423311331,-331.931481700634)) ;
#30570=CARTESIAN_POINT('Ctrl Pts',(6.58620492388242,-18.2774435932866,-331.935439991101)) ;
#30571=CARTESIAN_POINT('Ctrl Pts',(6.17521892875224,-18.4175754268229,-331.940671119721)) ;
#30572=CARTESIAN_POINT('Ctrl Pts',(6.08133368959512,-18.448788413838,-331.941870077088)) ;
#30573=CARTESIAN_POINT('Ctrl Pts',(5.92391672859546,-18.4997908838497,-331.943889841785)) ;
#30574=CARTESIAN_POINT('Ctrl Pts',(5.86051436307038,-18.5199736382629,-331.944705952644)) ;
#30575=CARTESIAN_POINT('Ctrl Pts',(5.73778777951122,-18.5583476229468,-331.946291398161)) ;
#30576=CARTESIAN_POINT('Ctrl Pts',(5.67847777592145,-18.5765810964998,-331.947060036303)) ;
#30577=CARTESIAN_POINT('Ctrl Pts',(5.52302576657717,-18.6235571428067,-331.949080058718)) ;
#30578=CARTESIAN_POINT('Ctrl Pts',(5.42674666363849,-18.6518394503323,-331.950336557173)) ;
#30579=CARTESIAN_POINT('Ctrl Pts',(5.30139047913159,-18.6876104640521,-331.951977601693)) ;
#30580=CARTESIAN_POINT('Ctrl Pts',(5.27250906713572,-18.6957795773398,-331.952356039048)) ;
#30581=CARTESIAN_POINT('Ctrl Pts',(4.94498569454738,-18.7876003276764,-331.95665115048)) ;
#30582=CARTESIAN_POINT('Ctrl Pts',(4.6444007520759,-18.8641551819347,-331.960625419525)) ;
#30583=CARTESIAN_POINT('Ctrl Pts',(3.89897388127834,-19.0351077689637,-331.970469728847)) ;
#30584=CARTESIAN_POINT('Ctrl Pts',(3.45240317785248,-19.1211463596962,-331.976355057538)) ;
#30585=CARTESIAN_POINT('Ctrl Pts',(2.61281186644438,-19.2525321724997,-331.987250745142)) ;
#30586=CARTESIAN_POINT('Ctrl Pts',(2.22062357708149,-19.3016997471526,-331.992272942745)) ;
#30587=CARTESIAN_POINT('Ctrl Pts',(1.66796369768334,-19.3539171064948,-331.999224795714)) ;
#30588=CARTESIAN_POINT('Ctrl Pts',(1.50853908457495,-19.3669956418256,-332.001215935438)) ;
#30589=CARTESIAN_POINT('Ctrl Pts',(1.22963635803475,-19.3864109415802,-332.004674157661)) ;
#30590=CARTESIAN_POINT('Ctrl Pts',(1.11022744190597,-19.3936156978999,-332.006146731842)) ;
#30591=CARTESIAN_POINT('Ctrl Pts',(0.874553115364349,-19.4056517797823,
-332.009037717497)) ;
#30592=CARTESIAN_POINT('Ctrl Pts',(0.758295660510367,-19.4105422870817,
-332.010456452545)) ;
#30593=CARTESIAN_POINT('Ctrl Pts',(0.42797158224745,-19.4214655497624,-332.01446774434)) ;
#30594=CARTESIAN_POINT('Ctrl Pts',(0.213839356670802,-19.4250033901669,
-332.017044336313)) ;
#30595=CARTESIAN_POINT('Ctrl Pts',(-0.000307738671744689,-19.4249999975623,
-332.019601838681)) ;
#30596=CARTESIAN_POINT('Origin',(0.,0.,-328.125)) ;
#30597=CARTESIAN_POINT('',(0.000433346557224641,-19.4249999951663,-333.731156854276)) ;
#30598=CARTESIAN_POINT('',(0.000492969430210768,-19.4249999937447,-333.518704187163)) ;
#30599=CARTESIAN_POINT('',(-2.37887640734373E-15,-19.425,-328.125)) ;
#30600=CARTESIAN_POINT('Ctrl Pts',(0.000438550581743774,-19.4249999950495,
-333.731600905675)) ;
#30601=CARTESIAN_POINT('Ctrl Pts',(0.240637510252596,-19.4249945721721,
-333.728785913431)) ;
#30602=CARTESIAN_POINT('Ctrl Pts',(0.480815547108525,-19.4205338949269,
-333.725958859962)) ;
#30603=CARTESIAN_POINT('Ctrl Pts',(0.851896410024764,-19.4067538423618,
-333.721539728974)) ;
#30604=CARTESIAN_POINT('Ctrl Pts',(0.982891383366073,-19.4005604725508,
-333.719969787331)) ;
#30605=CARTESIAN_POINT('Ctrl Pts',(1.1856194422729,-19.3889170571926,-333.717518864773)) ;
#30606=CARTESIAN_POINT('Ctrl Pts',(1.25740195541675,-19.3843941979241,-333.716646894659)) ;
#30607=CARTESIAN_POINT('Ctrl Pts',(1.38947859584908,-19.3753356091217,-333.715033671219)) ;
#30608=CARTESIAN_POINT('Ctrl Pts',(1.44977988429964,-19.3709168346406,-333.714293738554)) ;
#30609=CARTESIAN_POINT('Ctrl Pts',(1.57220891118611,-19.3613705653717,-333.712783745029)) ;
#30610=CARTESIAN_POINT('Ctrl Pts',(1.63433456706251,-19.3562253950017,-333.71201348384)) ;
#30611=CARTESIAN_POINT('Ctrl Pts',(1.81051038550961,-19.3407805040398,-333.709818819947)) ;
#30612=CARTESIAN_POINT('Ctrl Pts',(1.92449566265621,-19.3297712027147,-333.708386561347)) ;
#30613=CARTESIAN_POINT('Ctrl Pts',(2.5999750293889,-19.2584957632611,-333.699838990668)) ;
#30614=CARTESIAN_POINT('Ctrl Pts',(3.15872159764124,-19.1747752559848,-333.692530727464)) ;
#30615=CARTESIAN_POINT('Ctrl Pts',(4.24737628719546,-18.9627735279104,-333.678224856074)) ;
#30616=CARTESIAN_POINT('Ctrl Pts',(4.77711907509256,-18.8362979798261,-333.671231879681)) ;
#30617=CARTESIAN_POINT('Ctrl Pts',(5.40873053154289,-18.6571389482682,-333.662960360255)) ;
#30618=CARTESIAN_POINT('Ctrl Pts',(5.51634448419811,-18.6256045072849,-333.661553077209)) ;
#30619=CARTESIAN_POINT('Ctrl Pts',(5.70502109786341,-18.5685373961315,-333.659089687623)) ;
#30620=CARTESIAN_POINT('Ctrl Pts',(5.78620050290883,-18.5434012660412,-333.658031091294)) ;
#30621=CARTESIAN_POINT('Ctrl Pts',(5.97797491577687,-18.4826389040108,-333.65553345334)) ;
#30622=CARTESIAN_POINT('Ctrl Pts',(6.08842041596543,-18.4465514887318,-333.654097522711)) ;
#30623=CARTESIAN_POINT('Ctrl Pts',(6.31779703954782,-18.3693195669106,-333.651120324027)) ;
#30624=CARTESIAN_POINT('Ctrl Pts',(6.43666556746504,-18.3280058163714,-333.649580287407)) ;
#30625=CARTESIAN_POINT('Ctrl Pts',(6.69866248205231,-18.2340833859465,-333.64619124668)) ;
#30626=CARTESIAN_POINT('Ctrl Pts',(6.84158987289766,-18.180938481442,-333.644345993119)) ;
#30627=CARTESIAN_POINT('Ctrl Pts',(7.72305880153826,-17.8413141327266,-333.632979958776)) ;
#30628=CARTESIAN_POINT('Ctrl Pts',(8.44412843827558,-17.5115625117154,-333.623778977472)) ;
#30629=CARTESIAN_POINT('Ctrl Pts',(9.38866556836915,-17.0076771927583,-333.611255258856)) ;
#30630=CARTESIAN_POINT('Ctrl Pts',(9.6314419268088,-16.8713796318123,-333.60798790257)) ;
#30631=CARTESIAN_POINT('Ctrl Pts',(9.98008412303638,-16.6656691367316,-333.603178597004)) ;
#30632=CARTESIAN_POINT('Ctrl Pts',(10.0883338937597,-16.6003652389277,-333.601668449972)) ;
#30633=CARTESIAN_POINT('Ctrl Pts',(10.2814157660855,-16.4812984826206,-333.598938309033)) ;
#30634=CARTESIAN_POINT('Ctrl Pts',(10.3664830675631,-16.4279255720008,-333.597722542869)) ;
#30635=CARTESIAN_POINT('Ctrl Pts',(10.494207516735,-16.3464015905828,-333.595874829783)) ;
#30636=CARTESIAN_POINT('Ctrl Pts',(10.5371737812345,-16.3187378514082,-333.595249415472)) ;
#30637=CARTESIAN_POINT('Ctrl Pts',(10.6314799209429,-16.2574912953265,-333.593867677147)) ;
#30638=CARTESIAN_POINT('Ctrl Pts',(10.6827708388103,-16.2238341865602,-333.593110217067)) ;
#30639=CARTESIAN_POINT('Ctrl Pts',(10.8243970424172,-16.1299362351075,-333.591003098212)) ;
#30640=CARTESIAN_POINT('Ctrl Pts',(10.9143879648912,-16.0691801154643,-333.589646533754)) ;
#30641=CARTESIAN_POINT('Ctrl Pts',(11.5215268367352,-15.6518256337858,-333.58038651016)) ;
#30642=CARTESIAN_POINT('Ctrl Pts',(12.021622763175,-15.2710776274608,-333.572237469274)) ;
#30643=CARTESIAN_POINT('Ctrl Pts',(12.7873928977199,-14.6270940283031,-333.559340496345)) ;
#30644=CARTESIAN_POINT('Ctrl Pts',(13.0654454696614,-14.3792709244846,-333.554558504026)) ;
#30645=CARTESIAN_POINT('Ctrl Pts',(13.4742372492339,-13.9932697159809,-333.547419731746)) ;
#30646=CARTESIAN_POINT('Ctrl Pts',(13.6103537476888,-13.8609140320651,-333.545023222651)) ;
#30647=CARTESIAN_POINT('Ctrl Pts',(13.7544823748773,-13.7165972027297,-333.542466301195)) ;
#30648=CARTESIAN_POINT('Ctrl Pts',(13.7644455230011,-13.7065992743329,-333.542289447753)) ;
#30649=CARTESIAN_POINT('Ctrl Pts',(13.7830246751824,-13.6879145781381,-333.541959464384)) ;
#30650=CARTESIAN_POINT('Ctrl Pts',(13.7916433861455,-13.6792305121496,-333.541806311618)) ;
#30651=CARTESIAN_POINT('Ctrl Pts',(13.8077909014775,-13.6629297779574,-333.541519230739)) ;
#30652=CARTESIAN_POINT('Ctrl Pts',(13.8153216225214,-13.6553150151375,-333.541385286366)) ;
#30653=CARTESIAN_POINT('Ctrl Pts',(13.8294972378057,-13.6409574725932,-333.541133043452)) ;
#30654=CARTESIAN_POINT('Ctrl Pts',(13.8361435077236,-13.6342160556912,-333.54101473319)) ;
#30655=CARTESIAN_POINT('Ctrl Pts',(13.8487128104924,-13.6214481569775,-333.540790900817)) ;
#30656=CARTESIAN_POINT('Ctrl Pts',(13.8546368443151,-13.615422663762,-333.540685370147)) ;
#30657=CARTESIAN_POINT('Ctrl Pts',(13.8658920265613,-13.6039597652379,-333.540484801485)) ;
#30658=CARTESIAN_POINT('Ctrl Pts',(13.8712239129569,-13.5985230868316,-333.540389757162)) ;
#30659=CARTESIAN_POINT('Ctrl Pts',(13.8814001372614,-13.5881346481681,-333.54020830311)) ;
#30660=CARTESIAN_POINT('Ctrl Pts',(13.8862450259025,-13.5831834290828,-333.540121888645)) ;
#30661=CARTESIAN_POINT('Ctrl Pts',(13.8955331773685,-13.5736812681853,-333.539956176413)) ;
#30662=CARTESIAN_POINT('Ctrl Pts',(13.8999768555668,-13.5691307337038,-333.539876875067)) ;
#30663=CARTESIAN_POINT('Ctrl Pts',(13.9085334324928,-13.5603597844987,-333.539724135804)) ;
#30664=CARTESIAN_POINT('Ctrl Pts',(13.9126466472052,-13.5561396790471,-333.539650695158)) ;
#30665=CARTESIAN_POINT('Ctrl Pts',(13.9206014394819,-13.5479707304881,-333.539508629722)) ;
#30666=CARTESIAN_POINT('Ctrl Pts',(13.9244432587766,-13.5440221235859,-333.539440002842)) ;
#30667=CARTESIAN_POINT('Ctrl Pts',(13.9319053410319,-13.5363460937028,-333.539306676764)) ;
#30668=CARTESIAN_POINT('Ctrl Pts',(13.9355257892056,-13.5326188514406,-333.539241975963)) ;
#30669=CARTESIAN_POINT('Ctrl Pts',(13.9425882455676,-13.5253422307925,-333.539115736432)) ;
#30670=CARTESIAN_POINT('Ctrl Pts',(13.9460303950204,-13.5217929900834,-333.539054196478)) ;
#30671=CARTESIAN_POINT('Ctrl Pts',(13.9527741011949,-13.5148341612684,-333.53893360574)) ;
#30672=CARTESIAN_POINT('Ctrl Pts',(13.9560757641447,-13.5114246765845,-333.538874554035)) ;
#30673=CARTESIAN_POINT('Ctrl Pts',(13.9625724828677,-13.5047108738972,-333.538758334752)) ;
#30674=CARTESIAN_POINT('Ctrl Pts',(13.9657676160324,-13.501406631232,-333.538701166502)) ;
#30675=CARTESIAN_POINT('Ctrl Pts',(13.9720826110679,-13.4948713473917,-333.538588155489)) ;
#30676=CARTESIAN_POINT('Ctrl Pts',(13.9752025257003,-13.4916403576,-333.538532312267)) ;
#30677=CARTESIAN_POINT('Ctrl Pts',(13.9813968663759,-13.4852210320213,-333.538421419588)) ;
#30678=CARTESIAN_POINT('Ctrl Pts',(13.984471323107,-13.4820327262166,-333.538366369865)) ;
#30679=CARTESIAN_POINT('Ctrl Pts',(13.9906040330922,-13.4756685633107,-333.538256540576)) ;
#30680=CARTESIAN_POINT('Ctrl Pts',(13.9936622961041,-13.4724927159592,-333.538201760927)) ;
#30681=CARTESIAN_POINT('Ctrl Pts',(13.9997924986543,-13.4661224795987,-333.538091936751)) ;
#30682=CARTESIAN_POINT('Ctrl Pts',(14.0028644267675,-13.4629280799721,-333.538036892327)) ;
#30683=CARTESIAN_POINT('Ctrl Pts',(14.0090536557543,-13.4564876890003,-333.537925970241)) ;
#30684=CARTESIAN_POINT('Ctrl Pts',(14.0121709212934,-13.4532416660988,-333.537870092898)) ;
#30685=CARTESIAN_POINT('Ctrl Pts',(14.0969610276311,-13.3648878995049,-333.536349938729)) ;
#30686=CARTESIAN_POINT('Ctrl Pts',(14.1778581501325,-13.2790390125067,-333.534892481846)) ;
#30687=CARTESIAN_POINT('Ctrl Pts',(14.3437921448222,-13.099703096016,-333.531887900899)) ;
#30688=CARTESIAN_POINT('Ctrl Pts',(14.4287088015307,-13.0061122810377,-333.53034187031)) ;
#30689=CARTESIAN_POINT('Ctrl Pts',(14.6156678756097,-12.7959709185598,-333.526918072474)) ;
#30690=CARTESIAN_POINT('Ctrl Pts',(14.7172416424833,-12.67901485605,-333.525044355498)) ;
#30691=CARTESIAN_POINT('Ctrl Pts',(15.3832693379302,-11.8933357322318,-333.512657361094)) ;
#30692=CARTESIAN_POINT('Ctrl Pts',(15.9033764841782,-11.1883431515826,-333.502545468447)) ;
#30693=CARTESIAN_POINT('Ctrl Pts',(16.4948363777841,-10.2616420118615,-333.489644641934)) ;
#30694=CARTESIAN_POINT('Ctrl Pts',(16.6122131415321,-10.0705162834489,-333.487000214077)) ;
#30695=CARTESIAN_POINT('Ctrl Pts',(16.8049719276461,-9.74410123903481,-333.482481987595)) ;
#30696=CARTESIAN_POINT('Ctrl Pts',(16.882093585185,-9.60986506154454,-333.480623304129)) ;
#30697=CARTESIAN_POINT('Ctrl Pts',(16.9950777308637,-9.40764907160485,-333.477812999067)) ;
#30698=CARTESIAN_POINT('Ctrl Pts',(17.0321548694654,-9.34035484420517,-333.47687607463)) ;
#30699=CARTESIAN_POINT('Ctrl Pts',(17.1005348416455,-9.21448553897886,-333.475118932505)) ;
#30700=CARTESIAN_POINT('Ctrl Pts',(17.1319383526833,-9.15596657166212,-333.474299997191)) ;
#30701=CARTESIAN_POINT('Ctrl Pts',(17.2030771676023,-9.02175531729164,-333.472417988342)) ;
#30702=CARTESIAN_POINT('Ctrl Pts',(17.242614147293,-8.94595944447764,-333.471352434968)) ;
#30703=CARTESIAN_POINT('Ctrl Pts',(17.4089068035397,-8.6219637138026,-333.466790218713)) ;
#30704=CARTESIAN_POINT('Ctrl Pts',(17.5308133724107,-8.37131270202806,-333.463242772097)) ;
#30705=CARTESIAN_POINT('Ctrl Pts',(17.6766582056498,-8.05427338104472,-333.458769373237)) ;
#30706=CARTESIAN_POINT('Ctrl Pts',(17.7056851451043,-7.99026148217449,-333.457866826918)) ;
#30707=CARTESIAN_POINT('Ctrl Pts',(17.9065774092179,-7.54077188782342,-333.451536561651)) ;
#30708=CARTESIAN_POINT('Ctrl Pts',(18.0661870262132,-7.14993998904863,-333.44607308749)) ;
#30709=CARTESIAN_POINT('Ctrl Pts',(18.2909961221862,-6.54373610484607,-333.437762920931)) ;
#30710=CARTESIAN_POINT('Ctrl Pts',(18.3653988659806,-6.3319148780479,-333.434888503684)) ;
#30711=CARTESIAN_POINT('Ctrl Pts',(18.4791414337213,-5.98920826684635,-333.430294562081)) ;
#30712=CARTESIAN_POINT('Ctrl Pts',(18.5208007287333,-5.8591146267667,-333.428563567169)) ;
#30713=CARTESIAN_POINT('Ctrl Pts',(18.6221282529397,-5.53080557296592,-333.424229583725)) ;
#30714=CARTESIAN_POINT('Ctrl Pts',(18.6800068279149,-5.33205552028042,-333.421637317276)) ;
#30715=CARTESIAN_POINT('Ctrl Pts',(18.7694276428676,-5.00564565263722,-333.417432985661)) ;
#30716=CARTESIAN_POINT('Ctrl Pts',(18.8028696943002,-4.87852372702762,-333.415808554372)) ;
#30717=CARTESIAN_POINT('Ctrl Pts',(18.8660930589882,-4.62788276621338,-333.412630856239)) ;
#30718=CARTESIAN_POINT('Ctrl Pts',(18.895957867395,-4.50439147180606,-333.411077101227)) ;
#30719=CARTESIAN_POINT('Ctrl Pts',(18.9672562780315,-4.19637667499849,-333.407230124622)) ;
#30720=CARTESIAN_POINT('Ctrl Pts',(19.0072107745175,-4.01152422887809,-333.404946720168)) ;
#30721=CARTESIAN_POINT('Ctrl Pts',(19.1428539485452,-3.33636178791636,-333.396688758531)) ;
#30722=CARTESIAN_POINT('Ctrl Pts',(19.2223194384042,-2.84299208022768,-333.390816015683)) ;
#30723=CARTESIAN_POINT('Ctrl Pts',(19.3470593237684,-1.8181911737485,-333.378745123188)) ;
#30724=CARTESIAN_POINT('Ctrl Pts',(19.3896502954353,-1.2868498898905,-333.372556822471)) ;
#30725=CARTESIAN_POINT('Ctrl Pts',(19.4170699836498,-0.58138533240423,-333.364163615815)) ;
#30726=CARTESIAN_POINT('Ctrl Pts',(19.4214814729503,-0.408255901899993,
-333.362089097568)) ;
#30727=CARTESIAN_POINT('Ctrl Pts',(19.4245452607997,-0.155121042115437,
-333.35902157745)) ;
#30728=CARTESIAN_POINT('Ctrl Pts',(19.4250192841486,-0.0751459607953256,
-333.35804740894)) ;
#30729=CARTESIAN_POINT('Ctrl Pts',(19.42498291383,0.0711353845930604,-333.35625470279)) ;
#30730=CARTESIAN_POINT('Ctrl Pts',(19.4246269351351,0.13744032643945,-333.355437890318)) ;
#30731=CARTESIAN_POINT('Ctrl Pts',(19.4229132651343,0.30081453407795,-333.353415409582)) ;
#30732=CARTESIAN_POINT('Ctrl Pts',(19.4211673764434,0.397877856347019,-333.352205381687)) ;
#30733=CARTESIAN_POINT('Ctrl Pts',(19.4110232288516,0.79589075797672,-333.347214618815)) ;
#30734=CARTESIAN_POINT('Ctrl Pts',(19.3963565899525,1.09663818462654,-333.34337610559)) ;
#30735=CARTESIAN_POINT('Ctrl Pts',(19.3649781136623,1.53184404487331,-333.337775533208)) ;
#30736=CARTESIAN_POINT('Ctrl Pts',(19.3538411250613,1.66666049391692,-333.336034092772)) ;
#30737=CARTESIAN_POINT('Ctrl Pts',(19.2940586134025,2.30855218855928,-333.327724472805)) ;
#30738=CARTESIAN_POINT('Ctrl Pts',(19.2268873405422,2.81370144019565,-333.321136516688)) ;
#30739=CARTESIAN_POINT('Ctrl Pts',(19.1020428751769,3.53438463478772,-333.311808267238)) ;
#30740=CARTESIAN_POINT('Ctrl Pts',(19.0603993295577,3.75247843096919,-333.308993793443)) ;
#30741=CARTESIAN_POINT('Ctrl Pts',(18.9767904615134,4.15295719201776,-333.303847912289)) ;
#30742=CARTESIAN_POINT('Ctrl Pts',(18.9359104768492,4.33554197612063,-333.301510378501)) ;
#30743=CARTESIAN_POINT('Ctrl Pts',(18.8626337201872,4.64198831378599,-333.297602588198)) ;
#30744=CARTESIAN_POINT('Ctrl Pts',(18.8316386548188,4.76617162854907,-333.296023293535)) ;
#30745=CARTESIAN_POINT('Ctrl Pts',(18.7661338509389,5.01800030823523,-333.292829023471)) ;
#30746=CARTESIAN_POINT('Ctrl Pts',(18.7315435367731,5.14561790168791,-333.291214678661)) ;
#30747=CARTESIAN_POINT('Ctrl Pts',(18.6382919252303,5.47625357992298,-333.287042181389)) ;
#30748=CARTESIAN_POINT('Ctrl Pts',(18.5776158972644,5.67868531791672,-333.284497542635)) ;
#30749=CARTESIAN_POINT('Ctrl Pts',(18.4245379764094,6.16065623749146,-333.278453034908)) ;
#30750=CARTESIAN_POINT('Ctrl Pts',(18.3290603761536,6.43916384565315,-333.274971985635)) ;
#30751=CARTESIAN_POINT('Ctrl Pts',(18.1470893756267,6.93307949700225,-333.268786554412)) ;
#30752=CARTESIAN_POINT('Ctrl Pts',(18.0629953022918,7.14931079914399,-333.266074255217)) ;
#30753=CARTESIAN_POINT('Ctrl Pts',(17.8248729960615,7.73055324125156,-333.258737004916)) ;
#30754=CARTESIAN_POINT('Ctrl Pts',(17.663519593666,8.09244249423578,-333.254119711503)) ;
#30755=CARTESIAN_POINT('Ctrl Pts',(17.4441586451935,8.54655825261737,-333.24815564068)) ;
#30756=CARTESIAN_POINT('Ctrl Pts',(17.3962896764393,8.6435776311753,-333.246871197402)) ;
#30757=CARTESIAN_POINT('Ctrl Pts',(17.2824082550688,8.86961051525614,-333.243849920018)) ;
#30758=CARTESIAN_POINT('Ctrl Pts',(17.2157575925383,8.998295182807,-333.24210766899)) ;
#30759=CARTESIAN_POINT('Ctrl Pts',(17.1124238202571,9.19245370898263,-333.239437189531)) ;
#30760=CARTESIAN_POINT('Ctrl Pts',(17.0767909004466,9.25848079978737,-333.238521615424)) ;
#30761=CARTESIAN_POINT('Ctrl Pts',(17.008547787013,9.38319961716122,-333.236776611772)) ;
#30762=CARTESIAN_POINT('Ctrl Pts',(16.9760141219689,9.44193186655502,-333.235948141072)) ;
#30763=CARTESIAN_POINT('Ctrl Pts',(16.890721527033,9.59404263872836,-333.233786034316)) ;
#30764=CARTESIAN_POINT('Ctrl Pts',(16.8374925734254,9.68715498223381,-333.232446387797)) ;
#30765=CARTESIAN_POINT('Ctrl Pts',(16.4692086308292,10.3191799888549,-333.223255042643)) ;
#30766=CARTESIAN_POINT('Ctrl Pts',(16.1291054287192,10.8430745638096,-333.215158950642)) ;
#30767=CARTESIAN_POINT('Ctrl Pts',(15.4879929477942,11.7335606980522,-333.201013931531)) ;
#30768=CARTESIAN_POINT('Ctrl Pts',(15.1976861145089,12.107217305967,-333.194946031525)) ;
#30769=CARTESIAN_POINT('Ctrl Pts',(14.7583180814734,12.6319976359357,-333.186307815645)) ;
#30770=CARTESIAN_POINT('Ctrl Pts',(14.6199694614354,12.7918649944131,-333.18365902057)) ;
#30771=CARTESIAN_POINT('Ctrl Pts',(14.3908860959917,13.0480078332665,-333.179388674162)) ;
#30772=CARTESIAN_POINT('Ctrl Pts',(14.3017291188879,13.1456705919147,-333.177753975643)) ;
#30773=CARTESIAN_POINT('Ctrl Pts',(14.1253409408252,13.3349680079283,-333.174572372322)) ;
#30774=CARTESIAN_POINT('Ctrl Pts',(14.0381979334757,13.4266759585693,-333.173024806631)) ;
#30775=CARTESIAN_POINT('Ctrl Pts',(13.8419523826118,13.6292025028445,-333.169592290601)) ;
#30776=CARTESIAN_POINT('Ctrl Pts',(13.7324023107616,13.7395754478356,-333.167711465801)) ;
#30777=CARTESIAN_POINT('Ctrl Pts',(13.2333692518717,14.230425622525,-333.159294352496)) ;
#30778=CARTESIAN_POINT('Ctrl Pts',(12.8293183219051,14.5957414397109,-333.152892147122)) ;
#30779=CARTESIAN_POINT('Ctrl Pts',(11.9950124408525,15.2886210585865,-333.140213387796)) ;
#30780=CARTESIAN_POINT('Ctrl Pts',(11.5653628260783,15.6161658991078,-333.133941007662)) ;
#30781=CARTESIAN_POINT('Ctrl Pts',(10.9887083838154,16.018913677342,-333.125567869635)) ;
#30782=CARTESIAN_POINT('Ctrl Pts',(10.8536155118191,16.110752233322,-333.123608789363)) ;
#30783=CARTESIAN_POINT('Ctrl Pts',(10.6520543157837,16.2440912011431,-333.120678513776)) ;
#30784=CARTESIAN_POINT('Ctrl Pts',(10.5864672598366,16.2869110341224,-333.119723883043)) ;
#30785=CARTESIAN_POINT('Ctrl Pts',(10.4645500408342,16.3654595645565,-333.117945661744)) ;
#30786=CARTESIAN_POINT('Ctrl Pts',(10.40829148202,16.4012969824107,-333.117123515636)) ;
#30787=CARTESIAN_POINT('Ctrl Pts',(10.2670895262562,16.4902253317346,-333.115056802837)) ;
#30788=CARTESIAN_POINT('Ctrl Pts',(10.1819179910304,16.5429503056695,-333.113807403652)) ;
#30789=CARTESIAN_POINT('Ctrl Pts',(9.79143710092742,16.7805173730125,-333.10807359189)) ;
#30790=CARTESIAN_POINT('Ctrl Pts',(9.48147752154305,16.9575819899353,-333.103507420401)) ;
#30791=CARTESIAN_POINT('Ctrl Pts',(9.05011184033831,17.1884735491353,-333.097212351778)) ;
#30792=CARTESIAN_POINT('Ctrl Pts',(8.93277116644243,17.2497462748253,-333.095505690404)) ;
#30793=CARTESIAN_POINT('Ctrl Pts',(8.39656519742377,17.5228026665727,-333.087743567385)) ;
#30794=CARTESIAN_POINT('Ctrl Pts',(7.97073415744361,17.7205620325568,-333.081684402296)) ;
#30795=CARTESIAN_POINT('Ctrl Pts',(7.34124518317848,17.9856163017766,-333.072982606548)) ;
#30796=CARTESIAN_POINT('Ctrl Pts',(7.14297669632664,18.0652749415487,-333.070276864771)) ;
#30797=CARTESIAN_POINT('Ctrl Pts',(6.77343519647141,18.2067112280152,-333.065303854228)) ;
#30798=CARTESIAN_POINT('Ctrl Pts',(6.60252975588462,18.2693831058139,-333.063031185004)) ;
#30799=CARTESIAN_POINT('Ctrl Pts',(6.31076977857024,18.371744118536,-333.05919829711)) ;
#30800=CARTESIAN_POINT('Ctrl Pts',(6.19036035022939,18.412665096058,-333.057629841057)) ;
#30801=CARTESIAN_POINT('Ctrl Pts',(5.95798393448758,18.4891007902471,-333.054628162201)) ;
#30802=CARTESIAN_POINT('Ctrl Pts',(5.84607953364291,18.5247881154073,-333.053193821013)) ;
#30803=CARTESIAN_POINT('Ctrl Pts',(5.54137466680489,18.6189252659338,-333.049317416442)) ;
#30804=CARTESIAN_POINT('Ctrl Pts',(5.34797741724409,18.6753942121836,-333.046888667499)) ;
#30805=CARTESIAN_POINT('Ctrl Pts',(4.84618034748603,18.8134769387792,-333.040659276442)) ;
#30806=CARTESIAN_POINT('Ctrl Pts',(4.53658575028656,18.8905206043487,-333.03688640497)) ;
#30807=CARTESIAN_POINT('Ctrl Pts',(3.67056456854031,19.0835143101628,-333.026462374713)) ;
#30808=CARTESIAN_POINT('Ctrl Pts',(3.11073880895119,19.1827230887492,-333.019877242723)) ;
#30809=CARTESIAN_POINT('Ctrl Pts',(2.41727197784791,19.2744557206303,-333.011635316856)) ;
#30810=CARTESIAN_POINT('Ctrl Pts',(2.28700117345289,19.2903466201257,-333.010082926058)) ;
#30811=CARTESIAN_POINT('Ctrl Pts',(2.07729245154048,19.3137734778656,-333.007571641244)) ;
#30812=CARTESIAN_POINT('Ctrl Pts',(1.99795165563897,19.3221421962073,-333.00661870617)) ;
#30813=CARTESIAN_POINT('Ctrl Pts',(1.80226361975563,19.3415648101887,-333.004259342461)) ;
#30814=CARTESIAN_POINT('Ctrl Pts',(1.68586394131653,19.3520579312369,-333.002848097146)) ;
#30815=CARTESIAN_POINT('Ctrl Pts',(1.50003123457104,19.3671208934029,-333.000578089761)) ;
#30816=CARTESIAN_POINT('Ctrl Pts',(1.43065596303526,19.3723692128409,-332.999726879193)) ;
#30817=CARTESIAN_POINT('Ctrl Pts',(1.29826167994031,19.3816699287012,-332.998094109423)) ;
#30818=CARTESIAN_POINT('Ctrl Pts',(1.23524819987431,19.3857879511827,-332.997313438438)) ;
#30819=CARTESIAN_POINT('Ctrl Pts',(1.05330017153295,19.3967877846189,-332.995050180763)) ;
#30820=CARTESIAN_POINT('Ctrl Pts',(0.934321034145954,19.4028828207357,-332.993558974389)) ;
#30821=CARTESIAN_POINT('Ctrl Pts',(0.344803090013214,19.4276475084637,-332.986127106287)) ;
#30822=CARTESIAN_POINT('Ctrl Pts',(-0.126249964269435,19.4302968777024,
-332.980056226613)) ;
#30823=CARTESIAN_POINT('Ctrl Pts',(-0.613677451346516,19.4153111143555,
-332.973764851327)) ;
#30824=CARTESIAN_POINT('Ctrl Pts',(-0.630422417915108,19.4147746125597,
-332.973548702031)) ;
#30825=CARTESIAN_POINT('Ctrl Pts',(-1.09323222780011,19.3993469962056,-332.967574260517)) ;
#30826=CARTESIAN_POINT('Ctrl Pts',(-1.53865354229193,19.3691085770876,-332.961819045718)) ;
#30827=CARTESIAN_POINT('Ctrl Pts',(-2.12266817744188,19.3091874467497,-332.954344620164)) ;
#30828=CARTESIAN_POINT('Ctrl Pts',(-2.26253874258408,19.2932982804835,-332.95255960314)) ;
#30829=CARTESIAN_POINT('Ctrl Pts',(-2.61193680723005,19.2497551538605,-332.948115738213)) ;
#30830=CARTESIAN_POINT('Ctrl Pts',(-2.82120903691092,19.2201994567889,-332.945467837388)) ;
#30831=CARTESIAN_POINT('Ctrl Pts',(-3.16056135704347,19.1666105411561,-332.941198535374)) ;
#30832=CARTESIAN_POINT('Ctrl Pts',(-3.2909513116916,19.144653228733,-332.93956399948)) ;
#30833=CARTESIAN_POINT('Ctrl Pts',(-3.5456423729203,19.0990850743006,-332.93638246423)) ;
#30834=CARTESIAN_POINT('Ctrl Pts',(-3.66995717124761,19.0755876691145,-332.934834806657)) ;
#30835=CARTESIAN_POINT('Ctrl Pts',(-3.94657833863177,19.0204978175994,-332.931401770917)) ;
#30836=CARTESIAN_POINT('Ctrl Pts',(-4.09875276839955,18.9882870117658,-332.929520522777)) ;
#30837=CARTESIAN_POINT('Ctrl Pts',(-4.78169548142166,18.8351359186851,-332.921104345019)) ;
#30838=CARTESIAN_POINT('Ctrl Pts',(-5.30762564895109,18.6937440965461,-332.914703423215)) ;
#30839=CARTESIAN_POINT('Ctrl Pts',(-6.34208945927371,18.3684557387305,-332.902025849827)) ;
#30840=CARTESIAN_POINT('Ctrl Pts',(-6.85027615390731,18.1850482239758,-332.895753390762)) ;
#30841=CARTESIAN_POINT('Ctrl Pts',(-7.50136367455804,17.9188964974645,-332.887380125592)) ;
#30842=CARTESIAN_POINT('Ctrl Pts',(-7.65178360874278,17.8551817723879,-332.885420997911)) ;
#30843=CARTESIAN_POINT('Ctrl Pts',(-7.87311477003433,17.7581199462056,-332.882490665805)) ;
#30844=CARTESIAN_POINT('Ctrl Pts',(-7.94465681822003,17.7262288213319,-332.881536026868)) ;
#30845=CARTESIAN_POINT('Ctrl Pts',(-8.076762594974,17.6663799425577,-332.879757799825)) ;
#30846=CARTESIAN_POINT('Ctrl Pts',(-8.13737885336472,17.6385413130128,-332.878935656299)) ;
#30847=CARTESIAN_POINT('Ctrl Pts',(-8.28866081048154,17.5681177284296,-332.876868963693)) ;
#30848=CARTESIAN_POINT('Ctrl Pts',(-8.37914272793705,17.5251426714995,-332.875619582335)) ;
#30849=CARTESIAN_POINT('Ctrl Pts',(-8.79015125641648,17.3260204187595,-332.869890381904)) ;
#30850=CARTESIAN_POINT('Ctrl Pts',(-9.10667336779391,17.1617668660758,-332.865328981874)) ;
#30851=CARTESIAN_POINT('Ctrl Pts',(-9.49909402530684,16.944212304047,-332.859556101753)) ;
#30852=CARTESIAN_POINT('Ctrl Pts',(-9.57937449631672,16.8989556529289,-332.858368672963)) ;
#30853=CARTESIAN_POINT('Ctrl Pts',(-9.69243588238736,16.8341547964933,-332.856688416188)) ;
#30854=CARTESIAN_POINT('Ctrl Pts',(-9.72548593257093,16.815082646887,-332.856196273777)) ;
#30855=CARTESIAN_POINT('Ctrl Pts',(-10.1656923120821,16.5593213256834,-332.849628992767)) ;
#30856=CARTESIAN_POINT('Ctrl Pts',(-10.5641669132355,16.3079980912009,-332.843548740347)) ;
#30857=CARTESIAN_POINT('Ctrl Pts',(-11.1298541913737,15.9217703062943,-332.834821740233)) ;
#30858=CARTESIAN_POINT('Ctrl Pts',(-11.3045891844606,15.7981862118039,-332.832111456035)) ;
#30859=CARTESIAN_POINT('Ctrl Pts',(-11.6242732331865,15.5640646243421,-332.827131203072)) ;
#30860=CARTESIAN_POINT('Ctrl Pts',(-11.769777477771,15.4543254171097,-332.824855804296)) ;
#30861=CARTESIAN_POINT('Ctrl Pts',(-12.0141859922302,15.2645386657135,-332.821019772923)) ;
#30862=CARTESIAN_POINT('Ctrl Pts',(-12.1138871596305,15.1855373190068,-332.819450869595)) ;
#30863=CARTESIAN_POINT('Ctrl Pts',(-12.3166206303322,15.021627870495,-332.816251814469)) ;
#30864=CARTESIAN_POINT('Ctrl Pts',(-12.4195680638307,14.9366253483159,-332.814622564063)) ;
#30865=CARTESIAN_POINT('Ctrl Pts',(-12.6886292837425,14.709759595904,-332.810350125)) ;
#30866=CARTESIAN_POINT('Ctrl Pts',(-12.8532405659061,14.5661438839606,-332.807721776794)) ;
#30867=CARTESIAN_POINT('Ctrl Pts',(-13.2211306525875,14.2340837596221,-332.801803677417)) ;
#30868=CARTESIAN_POINT('Ctrl Pts',(-13.4228689011077,14.0440032395445,-332.798526908168)) ;
#30869=CARTESIAN_POINT('Ctrl Pts',(-14.0308187103431,13.4461144793822,-332.788505310189)) ;
#30870=CARTESIAN_POINT('Ctrl Pts',(-14.4230275582335,13.0245208219857,-332.781837196636)) ;
#30871=CARTESIAN_POINT('Ctrl Pts',(-14.8814798855379,12.4855761398134,-332.773501312507)) ;
#30872=CARTESIAN_POINT('Ctrl Pts',(-14.9659948553096,12.3841452295847,-332.77193975059)) ;
#30873=CARTESIAN_POINT('Ctrl Pts',(-15.1001252726387,12.2197897119688,-332.769415276397)) ;
#30874=CARTESIAN_POINT('Ctrl Pts',(-15.1503968620899,12.1574059223313,-332.768458391324)) ;
#30875=CARTESIAN_POINT('Ctrl Pts',(-15.2732690360566,12.002983772505,-332.766090895236)) ;
#30876=CARTESIAN_POINT('Ctrl Pts',(-15.3454251302086,11.9105958710813,-332.764675456101)) ;
#30877=CARTESIAN_POINT('Ctrl Pts',(-15.459108180474,11.7622892844271,-332.762400392098)) ;
#30878=CARTESIAN_POINT('Ctrl Pts',(-15.5011783715631,11.7067905096707,-332.761548377623)) ;
#30879=CARTESIAN_POINT('Ctrl Pts',(-15.5807867785326,11.6005899825796,-332.75991560678)) ;
#30880=CARTESIAN_POINT('Ctrl Pts',(-15.6183782225291,11.5499292754922,-332.75913575286)) ;
#30881=CARTESIAN_POINT('Ctrl Pts',(-15.7260335864455,11.4033591557038,-332.756877824472)) ;
#30882=CARTESIAN_POINT('Ctrl Pts',(-15.7954654458562,11.3069891519533,-332.75539119039)) ;
#30883=CARTESIAN_POINT('Ctrl Pts',(-16.1173902631968,10.8514116843935,-332.748365342679)) ;
#30884=CARTESIAN_POINT('Ctrl Pts',(-16.3585409384819,10.4843474655009,-332.742713310106)) ;
#30885=CARTESIAN_POINT('Ctrl Pts',(-16.8360655268671,9.70084898028878,-332.730878625599)) ;
#30886=CARTESIAN_POINT('Ctrl Pts',(-17.0699045422516,9.28320708008778,-332.724698969283)) ;
#30887=CARTESIAN_POINT('Ctrl Pts',(-17.354916199073,8.72691190692555,-332.716733552557)) ;
#30888=CARTESIAN_POINT('Ctrl Pts',(-17.4202701927891,8.59571370979229,-332.714873279382)) ;
#30889=CARTESIAN_POINT('Ctrl Pts',(-17.5788073100672,8.26821449266512,-332.71027760955)) ;
#30890=CARTESIAN_POINT('Ctrl Pts',(-17.6701934479759,8.0710656725557,-332.707553453045)) ;
#30891=CARTESIAN_POINT('Ctrl Pts',(-17.8122731492108,7.75056884177899,-332.703195100815)) ;
#30892=CARTESIAN_POINT('Ctrl Pts',(-17.8650376699087,7.62815975342177,-332.701546691436)) ;
#30893=CARTESIAN_POINT('Ctrl Pts',(-17.9651731074605,7.38911532081692,-332.698358711702)) ;
#30894=CARTESIAN_POINT('Ctrl Pts',(-18.0126783998465,7.27254335959728,-332.696818261432)) ;
#30895=CARTESIAN_POINT('Ctrl Pts',(-18.1260197636965,6.98649319462234,-332.693071763595)) ;
#30896=CARTESIAN_POINT('Ctrl Pts',(-18.1906159799789,6.81653651325428,-332.690874347761)) ;
#30897=CARTESIAN_POINT('Ctrl Pts',(-18.4917111519331,5.98956016241263,-332.680308407736)) ;
#30898=CARTESIAN_POINT('Ctrl Pts',(-18.69505245603,5.32101745546163,-332.672169990785)) ;
#30899=CARTESIAN_POINT('Ctrl Pts',(-18.965211654889,4.22350506080342,-332.658963549937)) ;
#30900=CARTESIAN_POINT('Ctrl Pts',(-19.0544461727274,3.80070091297439,-332.653906380235)) ;
#30901=CARTESIAN_POINT('Ctrl Pts',(-19.1507426307205,3.25493685063842,-332.647264359849)) ;
#30902=CARTESIAN_POINT('Ctrl Pts',(-19.1708395548099,3.13440072529529,-332.645790136637)) ;
#30903=CARTESIAN_POINT('Ctrl Pts',(-19.2007539260998,2.94391927657953,-332.64344396133)) ;
#30904=CARTESIAN_POINT('Ctrl Pts',(-19.2113295496236,2.87409619899446,-332.642580457603)) ;
#30905=CARTESIAN_POINT('Ctrl Pts',(-19.2305162936662,2.74258053620003,-332.640946234512)) ;
#30906=CARTESIAN_POINT('Ctrl Pts',(-19.239211882411,2.6809011640435,-332.640176605136)) ;
#30907=CARTESIAN_POINT('Ctrl Pts',(-19.2630127144438,2.50599567505363,-332.637986163198)) ;
#30908=CARTESIAN_POINT('Ctrl Pts',(-19.2774160923569,2.39267672415011,-332.636557541114)) ;
#30909=CARTESIAN_POINT('Ctrl Pts',(-19.3556851459913,1.73022966808652,-332.628163658032)) ;
#30910=CARTESIAN_POINT('Ctrl Pts',(-19.3970848131271,1.17870348039104,-332.621013138847)) ;
#30911=CARTESIAN_POINT('Ctrl Pts',(-19.4189239420216,0.501558483573225,
-332.612273500629)) ;
#30912=CARTESIAN_POINT('Ctrl Pts',(-19.4217430305178,0.376915967196436,
-332.61066603836)) ;
#30913=CARTESIAN_POINT('Ctrl Pts',(-19.4277516205274,-0.0857390490145371,
-332.604709669678)) ;
#30914=CARTESIAN_POINT('Ctrl Pts',(-19.423318112687,-0.423790456247844,
-332.600378949753)) ;
#30915=CARTESIAN_POINT('Ctrl Pts',(-19.4002828798608,-1.0108996640172,-332.592930403635)) ;
#30916=CARTESIAN_POINT('Ctrl Pts',(-19.3856959856753,-1.2600339100366,-332.589792231301)) ;
#30917=CARTESIAN_POINT('Ctrl Pts',(-19.3555143204028,-1.64742822420008,
-332.584952291665)) ;
#30918=CARTESIAN_POINT('Ctrl Pts',(-19.3432274914321,-1.78591843074365,
-332.583229919181)) ;
#30919=CARTESIAN_POINT('Ctrl Pts',(-19.317062796762,-2.04874569984758,-332.579975981516)) ;
#30920=CARTESIAN_POINT('Ctrl Pts',(-19.3034684240235,-2.17310397516719,
-332.578442664486)) ;
#30921=CARTESIAN_POINT('Ctrl Pts',(-19.269232337167,-2.46055545674489,-332.574912190885)) ;
#30922=CARTESIAN_POINT('Ctrl Pts',(-19.247719616884,-2.62353533827136,-332.57292078095)) ;
#30923=CARTESIAN_POINT('Ctrl Pts',(-19.158438627005,-3.23954867857116,-332.565426998394)) ;
#30924=CARTESIAN_POINT('Ctrl Pts',(-19.0767220977745,-3.69040940486956,
-332.560013957573)) ;
#30925=CARTESIAN_POINT('Ctrl Pts',(-18.9649286932409,-4.20316046581644,
-332.55386231649)) ;
#30926=CARTESIAN_POINT('Ctrl Pts',(-18.9503772606234,-4.2682877039268,-332.553080961274)) ;
#30927=CARTESIAN_POINT('Ctrl Pts',(-18.8307665069412,-4.7909535890797,-332.546807934775)) ;
#30928=CARTESIAN_POINT('Ctrl Pts',(-18.7094882783897,-5.24462112942083,
-332.541352269244)) ;
#30929=CARTESIAN_POINT('Ctrl Pts',(-18.5230373785132,-5.85281963444294,
-332.533843442027)) ;
#30930=CARTESIAN_POINT('Ctrl Pts',(-18.4721306018671,-6.01155573116635,
-332.531864900236)) ;
#30931=CARTESIAN_POINT('Ctrl Pts',(-18.3792129446722,-6.28895833144694,
-332.528361140513)) ;
#30932=CARTESIAN_POINT('Ctrl Pts',(-18.3380798814535,-6.4079085160051,-332.526843669243)) ;
#30933=CARTESIAN_POINT('Ctrl Pts',(-18.2718215176671,-6.59365257124561,
-332.524444998102)) ;
#30934=CARTESIAN_POINT('Ctrl Pts',(-18.2474791858175,-6.66072211932476,
-332.523572879237)) ;
#30935=CARTESIAN_POINT('Ctrl Pts',(-18.2013629439761,-6.78563420988526,
-332.521936181542)) ;
#30936=CARTESIAN_POINT('Ctrl Pts',(-18.1796814251312,-6.84350991195361,
-332.521172819736)) ;
#30937=CARTESIAN_POINT('Ctrl Pts',(-18.1181597730131,-7.00537742165052,
-332.519024754052)) ;
#30938=CARTESIAN_POINT('Ctrl Pts',(-18.077701063549,-7.10913149298922,-332.517632702517)) ;
#30939=CARTESIAN_POINT('Ctrl Pts',(-17.7803149815643,-7.85280380534435,
-332.507560122073)) ;
#30940=CARTESIAN_POINT('Ctrl Pts',(-17.4903657112314,-8.47898793077572,
-332.498590331982)) ;
#30941=CARTESIAN_POINT('Ctrl Pts',(-17.0112787635502,-9.3839673760511,-332.485410776379)) ;
#30942=CARTESIAN_POINT('Ctrl Pts',(-16.8472160760208,-9.67542040438931,
-332.481127569767)) ;
#30943=CARTESIAN_POINT('Ctrl Pts',(-16.6156281858173,-10.0630636209073,
-332.47540424251)) ;
#30944=CARTESIAN_POINT('Ctrl Pts',(-16.5546361838925,-10.163088620157,-332.473924858382)) ;
#30945=CARTESIAN_POINT('Ctrl Pts',(-16.3944887207595,-10.4204583249398,
-332.470112734989)) ;
#30946=CARTESIAN_POINT('Ctrl Pts',(-16.2939717182453,-10.5769418034851,
-332.467789520545)) ;
#30947=CARTESIAN_POINT('Ctrl Pts',(-16.1206128116088,-10.8384870647885,
-332.463898298816)) ;
#30948=CARTESIAN_POINT('Ctrl Pts',(-16.0489528599848,-10.9443168550778,
-332.462321431671)) ;
#30949=CARTESIAN_POINT('Ctrl Pts',(-15.9008859070986,-11.1584052570647,
-332.459126296506)) ;
#30950=CARTESIAN_POINT('Ctrl Pts',(-15.8244051026833,-11.2666047997321,
-332.457508719485)) ;
#30951=CARTESIAN_POINT('Ctrl Pts',(-15.6221841714602,-11.5465708177693,
-332.453314506119)) ;
#30952=CARTESIAN_POINT('Ctrl Pts',(-15.4947170122384,-11.7170679291378,
-332.450751668014)) ;
#30953=CARTESIAN_POINT('Ctrl Pts',(-15.1866665206812,-12.1152892190306,
-332.444735104618)) ;
#30954=CARTESIAN_POINT('Ctrl Pts',(-15.0037239967095,-12.3411239143907,
-332.441298887799)) ;
#30955=CARTESIAN_POINT('Ctrl Pts',(-14.4450966118055,-12.9999358605913,
-332.431148299937)) ;
#30956=CARTESIAN_POINT('Ctrl Pts',(-14.055242733301,-13.4204805629253,-332.4245072442)) ;
#30957=CARTESIAN_POINT('Ctrl Pts',(-13.5535984731228,-13.9157448947969,
-332.416201980336)) ;
#30958=CARTESIAN_POINT('Ctrl Pts',(-13.4588912874011,-14.0073635210805,
-332.414643392202)) ;
#30959=CARTESIAN_POINT('Ctrl Pts',(-13.2429961554026,-14.2120067553671,
-332.411103372992)) ;
#30960=CARTESIAN_POINT('Ctrl Pts',(-13.121279367638,-14.324458481653,-332.409116592753)) ;
#30961=CARTESIAN_POINT('Ctrl Pts',(-12.9396326178462,-14.4880202591157,
-332.406153316191)) ;
#30962=CARTESIAN_POINT('Ctrl Pts',(-12.8808066171937,-14.5403453942164,
-332.405193916987)) ;
#30963=CARTESIAN_POINT('Ctrl Pts',(-12.7716375520807,-14.6362677641729,
-332.403412307077)) ;
#30964=CARTESIAN_POINT('Ctrl Pts',(-12.7213853650103,-14.6799664231755,
-332.402591610123)) ;
#30965=CARTESIAN_POINT('Ctrl Pts',(-12.5955901877638,-14.7882252954947,
-332.400536390685)) ;
#30966=CARTESIAN_POINT('Ctrl Pts',(-12.5197746705447,-14.8524658467341,
-332.39929715802)) ;
#30967=CARTESIAN_POINT('Ctrl Pts',(-12.1717865264776,-15.142767842328,-332.393613267457)) ;
#30968=CARTESIAN_POINT('Ctrl Pts',(-11.8939622737829,-15.3619486310123,
-332.389087928359)) ;
#30969=CARTESIAN_POINT('Ctrl Pts',(-11.5326942342993,-15.6312814798705,
-332.383291120064)) ;
#30970=CARTESIAN_POINT('Ctrl Pts',(-11.4546489307258,-15.6885631869735,
-332.382043785992)) ;
#30971=CARTESIAN_POINT('Ctrl Pts',(-10.973894048919,-16.0359155823469,-332.374396324313)) ;
#30972=CARTESIAN_POINT('Ctrl Pts',(-10.5606171535038,-16.3110485875344,
-332.367981417839)) ;
#30973=CARTESIAN_POINT('Ctrl Pts',(-10.009640622601,-16.6481260620061,-332.35974641017)) ;
#30974=CARTESIAN_POINT('Ctrl Pts',(-9.88112539612904,-16.7247232485876,
-332.357846756401)) ;
#30975=CARTESIAN_POINT('Ctrl Pts',(-9.5611658863874,-16.9104490365189,-332.353172232872)) ;
#30976=CARTESIAN_POINT('Ctrl Pts',(-9.36872500665138,-17.0178192410676,
-332.350408746948)) ;
#30977=CARTESIAN_POINT('Ctrl Pts',(-9.056522161754,-17.1851082658492,-332.346004484073)) ;
#30978=CARTESIAN_POINT('Ctrl Pts',(-8.93789510671079,-17.2471032609878,
-332.344348925304)) ;
#30979=CARTESIAN_POINT('Ctrl Pts',(-8.70673695856695,-17.364882054619,-332.341157168328)) ;
#30980=CARTESIAN_POINT('Ctrl Pts',(-8.59428682941758,-17.4208102905137,
-332.339619980433)) ;
#30981=CARTESIAN_POINT('Ctrl Pts',(-8.31943551522749,-17.5542014850658,
-332.33589927257)) ;
#30982=CARTESIAN_POINT('Ctrl Pts',(-8.15648508900026,-17.630506180893,-332.333724084194)) ;
#30983=CARTESIAN_POINT('Ctrl Pts',(-7.33356451188227,-18.0020036892799,
-332.322880931629)) ;
#30984=CARTESIAN_POINT('Ctrl Pts',(-6.65853711032058,-18.2624529937872,
-332.31446363226)) ;
#30985=CARTESIAN_POINT('Ctrl Pts',(-5.57574936940371,-18.6121946282473,
-332.301164450802)) ;
#30986=CARTESIAN_POINT('Ctrl Pts',(-5.17694700309865,-18.7270389564152,
-332.296302070594)) ;
#30987=CARTESIAN_POINT('Ctrl Pts',(-4.65811098238901,-18.8586084530582,
-332.289884674294)) ;
#30988=CARTESIAN_POINT('Ctrl Pts',(-4.54117471486675,-18.8871078478145,
-332.288432204837)) ;
#30989=CARTESIAN_POINT('Ctrl Pts',(-4.35557352657564,-18.9305187430926,
-332.286112390987)) ;
#30990=CARTESIAN_POINT('Ctrl Pts',(-4.28707947926307,-18.9461476337104,
-332.285253182086)) ;
#30991=CARTESIAN_POINT('Ctrl Pts',(-4.1574320401589,-18.9749913832687,-332.283619788843)) ;
#30992=CARTESIAN_POINT('Ctrl Pts',(-4.09629665022204,-18.9882830426053,
-332.282846627552)) ;
#30993=CARTESIAN_POINT('Ctrl Pts',(-3.9218102891493,-19.0253368425524,-332.280632682393)) ;
#30994=CARTESIAN_POINT('Ctrl Pts',(-3.80830964206489,-19.0483809161981,
-332.279183829931)) ;
#30995=CARTESIAN_POINT('Ctrl Pts',(-3.17972743981411,-19.1701594293648,
-332.271124448513)) ;
#30996=CARTESIAN_POINT('Ctrl Pts',(-2.6610169450038,-19.2490172959982,-332.264348663488)) ;
#30997=CARTESIAN_POINT('Ctrl Pts',(-1.71549596462045,-19.3538085133732,
-332.252075231236)) ;
#30998=CARTESIAN_POINT('Ctrl Pts',(-1.28980314857844,-19.3868315955085,
-332.246576467878)) ;
#30999=CARTESIAN_POINT('Ctrl Pts',(-0.575820481165384,-19.4185968412911,
-332.237483147593)) ;
#31000=CARTESIAN_POINT('Ctrl Pts',(-0.288023300897207,-19.4249971845775,
-332.233852058736)) ;
#31001=CARTESIAN_POINT('Ctrl Pts',(-0.00018994165136052,-19.4249999990714,
-332.23026054535)) ;
#31002=CARTESIAN_POINT('Ctrl Pts',(-0.000307707308464245,-19.4249999975628,
-332.019601838307)) ;
#31003=CARTESIAN_POINT('Ctrl Pts',(-0.951439775158993,-19.4249849308813,
-332.030960958138)) ;
#31004=CARTESIAN_POINT('Ctrl Pts',(-1.90128001069508,-19.3551129679746,
-332.041854748475)) ;
#31005=CARTESIAN_POINT('Ctrl Pts',(-2.97483821811274,-19.1963264387993,
-332.054729320748)) ;
#31006=CARTESIAN_POINT('Ctrl Pts',(-3.10730053904505,-19.1753303611542,
-332.056329149228)) ;
#31007=CARTESIAN_POINT('Ctrl Pts',(-3.31967132845602,-19.1394099407424,
-332.058918618489)) ;
#31008=CARTESIAN_POINT('Ctrl Pts',(-3.39972210395476,-19.1253528125581,
-332.059900316459)) ;
#31009=CARTESIAN_POINT('Ctrl Pts',(-3.54100130439389,-19.09962877773,-332.061644494685)) ;
#31010=CARTESIAN_POINT('Ctrl Pts',(-3.60226624863132,-19.0881687845743,
-332.062404717117)) ;
#31011=CARTESIAN_POINT('Ctrl Pts',(-3.72859414795776,-19.0639085075207,
-332.063981187286)) ;
#31012=CARTESIAN_POINT('Ctrl Pts',(-3.79364867445113,-19.0510695659084,
-332.064798046553)) ;
#31013=CARTESIAN_POINT('Ctrl Pts',(-3.95380799781003,-19.0186081794214,
-332.06682094192)) ;
#31014=CARTESIAN_POINT('Ctrl Pts',(-4.04883375871283,-18.9986052099552,
-332.068031342115)) ;
#31015=CARTESIAN_POINT('Ctrl Pts',(-4.4347662699367,-18.9143392250366,-332.072983066224)) ;
#31016=CARTESIAN_POINT('Ctrl Pts',(-4.72432617156596,-18.8441004511013,
-332.076780831277)) ;
#31017=CARTESIAN_POINT('Ctrl Pts',(-5.60018938653857,-18.6101840807685,
-332.088415359661)) ;
#31018=CARTESIAN_POINT('Ctrl Pts',(-6.18051791537393,-18.4255874638366,
-332.096317378858)) ;
#31019=CARTESIAN_POINT('Ctrl Pts',(-6.97572807306964,-18.1308348139672,
-332.107155093707)) ;
#31020=CARTESIAN_POINT('Ctrl Pts',(-7.19867741351687,-18.0434751910813,
-332.110196346514)) ;
#31021=CARTESIAN_POINT('Ctrl Pts',(-7.55712179396332,-17.895322409297,-332.115082258856)) ;
#31022=CARTESIAN_POINT('Ctrl Pts',(-7.69363442015092,-17.8370581494356,
-332.116942252803)) ;
#31023=CARTESIAN_POINT('Ctrl Pts',(-7.89351260812988,-17.749027616591,-332.119663759718)) ;
#31024=CARTESIAN_POINT('Ctrl Pts',(-7.95740633862362,-17.7204742317892,
-332.120533453343)) ;
#31025=CARTESIAN_POINT('Ctrl Pts',(-8.12623069554891,-17.643931331889,-332.122830681574)) ;
#31026=CARTESIAN_POINT('Ctrl Pts',(-8.23089046721392,-17.5953510995359,
-332.124254041529)) ;
#31027=CARTESIAN_POINT('Ctrl Pts',(-8.43988527275577,-17.4960686010512,
-332.12709509048)) ;
#31028=CARTESIAN_POINT('Ctrl Pts',(-8.54421142404382,-17.4453584396755,
-332.12851265188)) ;
#31029=CARTESIAN_POINT('Ctrl Pts',(-8.82016514828314,-17.3081554988732,
-332.132261505826)) ;
#31030=CARTESIAN_POINT('Ctrl Pts',(-8.99097401522743,-17.2200449021287,
-332.134581100717)) ;
#31031=CARTESIAN_POINT('Ctrl Pts',(-9.69381805701577,-16.8441788132686,
-332.144134165511)) ;
#31032=CARTESIAN_POINT('Ctrl Pts',(-10.2135758742315,-16.5341869339315,
-332.151207780682)) ;
#31033=CARTESIAN_POINT('Ctrl Pts',(-11.0248944697991,-15.9974284287092,
-332.162569420456)) ;
#31034=CARTESIAN_POINT('Ctrl Pts',(-11.3259363983318,-15.785727047809,-332.166864059495)) ;
#31035=CARTESIAN_POINT('Ctrl Pts',(-11.7390432636421,-15.4773146486361,
-332.172966141708)) ;
#31036=CARTESIAN_POINT('Ctrl Pts',(-11.8562933575024,-15.3876805663342,
-332.174722745356)) ;
#31037=CARTESIAN_POINT('Ctrl Pts',(-12.0570342057736,-15.2305637441514,
-332.177782219564)) ;
#31038=CARTESIAN_POINT('Ctrl Pts',(-12.1410080832767,-15.1637089288877,
-332.179078145417)) ;
#31039=CARTESIAN_POINT('Ctrl Pts',(-12.2255574507256,-15.0952433616759,
-332.180401551843)) ;
#31040=CARTESIAN_POINT('Ctrl Pts',(-12.2266913522466,-15.0943249503285,
-332.180419303618)) ;
#31041=CARTESIAN_POINT('Ctrl Pts',(-12.228994943295,-15.0924587110059,-332.180455374399)) ;
#31042=CARTESIAN_POINT('Ctrl Pts',(-12.2301646261241,-15.0915108748082,
-332.18047369352)) ;
#31043=CARTESIAN_POINT('Ctrl Pts',(-12.2325396076684,-15.0895858841255,
-332.180510896976)) ;
#31044=CARTESIAN_POINT('Ctrl Pts',(-12.2337448995204,-15.0886087211854,
-332.18052978143)) ;
#31045=CARTESIAN_POINT('Ctrl Pts',(-12.2361908825572,-15.0866252103536,
-332.180568112855)) ;
#31046=CARTESIAN_POINT('Ctrl Pts',(-12.2374315667093,-15.0856188538011,
-332.180587559949)) ;
#31047=CARTESIAN_POINT('Ctrl Pts',(-12.2399480783119,-15.0835771201652,
-332.180627013358)) ;
#31048=CARTESIAN_POINT('Ctrl Pts',(-12.2412238985732,-15.0825417342284,
-332.180647019799)) ;
#31049=CARTESIAN_POINT('Ctrl Pts',(-12.2438103920022,-15.080442133277,-332.180687588083)) ;
#31050=CARTESIAN_POINT('Ctrl Pts',(-12.2451210577871,-15.0793779092692,
-332.180708150054)) ;
#31051=CARTESIAN_POINT('Ctrl Pts',(-12.2477769226022,-15.0772208466292,
-332.180749825136)) ;
#31052=CARTESIAN_POINT('Ctrl Pts',(-12.2491221141719,-15.076127998792,-332.180770938378)) ;
#31053=CARTESIAN_POINT('Ctrl Pts',(-12.2510140309455,-15.0745905652572,
-332.180800639532)) ;
#31054=CARTESIAN_POINT('Ctrl Pts',(-12.2515608783424,-15.0741461297426,
-332.180809225283)) ;
#31055=CARTESIAN_POINT('Ctrl Pts',(-12.2527455125578,-15.0731832430996,
-332.180827826327)) ;
#31056=CARTESIAN_POINT('Ctrl Pts',(-12.2533832906134,-15.0726647812813,
-332.180837841773)) ;
#31057=CARTESIAN_POINT('Ctrl Pts',(-12.2547627292948,-15.071543264126,-332.180859506384)) ;
#31058=CARTESIAN_POINT('Ctrl Pts',(-12.2555043782651,-15.0709401945619,
-332.180871155752)) ;
#31059=CARTESIAN_POINT('Ctrl Pts',(-12.2571056448104,-15.0696379332673,
-332.180896310687)) ;
#31060=CARTESIAN_POINT('Ctrl Pts',(-12.2579652472085,-15.0689387226188,
-332.180909816528)) ;
#31061=CARTESIAN_POINT('Ctrl Pts',(-12.3060966463666,-15.0297812356691,
-332.181666156376)) ;
#31062=CARTESIAN_POINT('Ctrl Pts',(-12.3531872611223,-14.9911007985688,
-332.182412210617)) ;
#31063=CARTESIAN_POINT('Ctrl Pts',(-12.4486230672338,-14.9119543775599,
-332.183937416464)) ;
#31064=CARTESIAN_POINT('Ctrl Pts',(-12.4969548139917,-14.8714733632677,
-332.184716766015)) ;
#31065=CARTESIAN_POINT('Ctrl Pts',(-12.6356024881665,-14.7541936275622,
-332.186971400356)) ;
#31066=CARTESIAN_POINT('Ctrl Pts',(-12.7254134726544,-14.6768025034912,
-332.188455207695)) ;
#31067=CARTESIAN_POINT('Ctrl Pts',(-13.115198781367,-14.3346525834505,-332.194987196964)) ;
#31068=CARTESIAN_POINT('Ctrl Pts',(-13.4076605370497,-14.061484337325,-332.200128175233)) ;
#31069=CARTESIAN_POINT('Ctrl Pts',(-13.9510611975513,-13.5215541457519,
-332.21000327909)) ;
#31070=CARTESIAN_POINT('Ctrl Pts',(-14.2033054706494,-13.2563437306619,
-332.214732895086)) ;
#31071=CARTESIAN_POINT('Ctrl Pts',(-14.639493158379,-12.7709834122329,-332.223107656365)) ;
#31072=CARTESIAN_POINT('Ctrl Pts',(-14.8263370842533,-12.5535853980457,
-332.226765010315)) ;
#31073=CARTESIAN_POINT('Ctrl Pts',(-15.1503124976644,-12.1593047735721,
-332.233215559331)) ;
#31074=CARTESIAN_POINT('Ctrl Pts',(-15.2893271087701,-11.984036806253,-332.23602183866)) ;
#31075=CARTESIAN_POINT('Ctrl Pts',(-15.5069999323951,-11.6996433312443,
-332.240476032222)) ;
#31076=CARTESIAN_POINT('Ctrl Pts',(-15.5876054753994,-11.5920341866365,
-332.242139355618)) ;
#31077=CARTESIAN_POINT('Ctrl Pts',(-15.7419976289247,-11.381396752822,-332.245352930139)) ;
#31078=CARTESIAN_POINT('Ctrl Pts',(-15.8159060672609,-11.2784660621457,
-332.246904107956)) ;
#31079=CARTESIAN_POINT('Ctrl Pts',(-15.9918278283731,-11.0283335164022,
-332.250628687595)) ;
#31080=CARTESIAN_POINT('Ctrl Pts',(-16.0928228896023,-10.8804296337474,
-332.25279404405)) ;
#31081=CARTESIAN_POINT('Ctrl Pts',(-16.5954006564032,-10.1221122501266,
-332.263721035737)) ;
#31082=CARTESIAN_POINT('Ctrl Pts',(-16.9643593381631,-9.49078458366264,
-332.272225256033)) ;
#31083=CARTESIAN_POINT('Ctrl Pts',(-17.4835040906425,-8.47501530310121,
-332.285559362289)) ;
#31084=CARTESIAN_POINT('Ctrl Pts',(-17.6585226967641,-8.10403444756312,
-332.29036685726)) ;
#31085=CARTESIAN_POINT('Ctrl Pts',(-17.8693367872057,-7.6178596528184,-332.296720849966)) ;
#31086=CARTESIAN_POINT('Ctrl Pts',(-17.915987951277,-7.50748683455282,-332.298167030131)) ;
#31087=CARTESIAN_POINT('Ctrl Pts',(-17.9883263876698,-7.33182512590009,
-332.3004792319)) ;
#31088=CARTESIAN_POINT('Ctrl Pts',(-18.0146863553376,-7.26681645687894,
-332.301337207854)) ;
#31089=CARTESIAN_POINT('Ctrl Pts',(-18.0639193856539,-7.14348416703496,
-332.302970422312)) ;
#31090=CARTESIAN_POINT('Ctrl Pts',(-18.0868635660893,-7.085189901955,-332.303744657638)) ;
#31091=CARTESIAN_POINT('Ctrl Pts',(-18.1515929910921,-6.91836836933145,
-332.305965705484)) ;
#31092=CARTESIAN_POINT('Ctrl Pts',(-18.1926861617147,-6.80957554994537,
-332.307420665331)) ;
#31093=CARTESIAN_POINT('Ctrl Pts',(-18.3545756949256,-6.36905103519003,
-332.313328893853)) ;
#31094=CARTESIAN_POINT('Ctrl Pts',(-18.4672950971057,-6.03442383918995,
-332.317853922846)) ;
#31095=CARTESIAN_POINT('Ctrl Pts',(-18.6016568407138,-5.59643050870255,
-332.323753268223)) ;
#31096=CARTESIAN_POINT('Ctrl Pts',(-18.6316651657819,-5.49570057430084,
-332.325108519062)) ;
#31097=CARTESIAN_POINT('Ctrl Pts',(-18.7910735249853,-4.94429298854793,
-332.332512834497)) ;
#31098=CARTESIAN_POINT('Ctrl Pts',(-18.9049409099176,-4.48928590308809,
-332.338565768473)) ;
#31099=CARTESIAN_POINT('Ctrl Pts',(-19.0322950044249,-3.8888767709539,-332.346385218203)) ;
#31100=CARTESIAN_POINT('Ctrl Pts',(-19.0607707745075,-3.74681641094796,
-332.348223595899)) ;
#31101=CARTESIAN_POINT('Ctrl Pts',(-19.1276543112821,-3.39262933653316,
-332.352775250304)) ;
#31102=CARTESIAN_POINT('Ctrl Pts',(-19.1641252752612,-3.18015658956369,
-332.355477369648)) ;
#31103=CARTESIAN_POINT('Ctrl Pts',(-19.2173652942855,-2.83569758372706,
-332.359809990587)) ;
#31104=CARTESIAN_POINT('Ctrl Pts',(-19.2363281062274,-2.70406928300005,
-332.361454390973)) ;
#31105=CARTESIAN_POINT('Ctrl Pts',(-19.2706293561641,-2.44731645927699,
-332.364640382477)) ;
#31106=CARTESIAN_POINT('Ctrl Pts',(-19.2861044002777,-2.32221677378434,
-332.366182790691)) ;
#31107=CARTESIAN_POINT('Ctrl Pts',(-19.317716192861,-2.04450813738184,-332.369585730242)) ;
#31108=CARTESIAN_POINT('Ctrl Pts',(-19.3332643806804,-1.89184061186663,
-332.371442391225)) ;
#31109=CARTESIAN_POINT('Ctrl Pts',(-19.3892511202734,-1.26896965949256,
-332.378965628)) ;
#31110=CARTESIAN_POINT('Ctrl Pts',(-19.4143569974093,-0.797550452465386,
-332.384535355409)) ;
#31111=CARTESIAN_POINT('Ctrl Pts',(-19.4252749986705,-0.146454517787673,
-332.392162686992)) ;
#31112=CARTESIAN_POINT('Ctrl Pts',(-19.4257993727771,0.0328092926956076,
-332.394256452771)) ;
#31113=CARTESIAN_POINT('Ctrl Pts',(-19.4198018815971,0.582169251885124,
-332.400672972894)) ;
#31114=CARTESIAN_POINT('Ctrl Pts',(-19.4051834745485,0.952092324516055,
-332.404992617901)) ;
#31115=CARTESIAN_POINT('Ctrl Pts',(-19.3699347202311,1.46907142367132,-332.411125563733)) ;
#31116=CARTESIAN_POINT('Ctrl Pts',(-19.3581759989151,1.61665204059852,-332.412887533737)) ;
#31117=CARTESIAN_POINT('Ctrl Pts',(-19.334241369452,1.87911634506717,-332.416050488706)) ;
#31118=CARTESIAN_POINT('Ctrl Pts',(-19.3227254735061,1.9940531057691,-332.417445658719)) ;
#31119=CARTESIAN_POINT('Ctrl Pts',(-19.3026602360087,2.17778258347615,-332.419696308407)) ;
#31120=CARTESIAN_POINT('Ctrl Pts',(-19.2947666182339,2.2466442345652,-332.42054446127)) ;
#31121=CARTESIAN_POINT('Ctrl Pts',(-19.2778310352548,2.38770816712964,-332.422292582599)) ;
#31122=CARTESIAN_POINT('Ctrl Pts',(-19.268751595483,2.45990480503155,-332.423192933375)) ;
#31123=CARTESIAN_POINT('Ctrl Pts',(-19.2419247586514,2.66395507253136,-332.425751941356)) ;
#31124=CARTESIAN_POINT('Ctrl Pts',(-19.2232281358396,2.79567970256964,-332.427420847213)) ;
#31125=CARTESIAN_POINT('Ctrl Pts',(-19.142664934783,3.32419458236349,-332.434171356912)) ;
#31126=CARTESIAN_POINT('Ctrl Pts',(-19.0698539343263,3.71921504313502,-332.439338386003)) ;
#31127=CARTESIAN_POINT('Ctrl Pts',(-18.9816921153021,4.12628310752134,-332.444709778016)) ;
#31128=CARTESIAN_POINT('Ctrl Pts',(-18.9785154974058,4.14086915492972,-332.444902311319)) ;
#31129=CARTESIAN_POINT('Ctrl Pts',(-18.873323934961,4.62121256983114,-332.451244822057)) ;
#31130=CARTESIAN_POINT('Ctrl Pts',(-18.7542116031314,5.08306113614125,-332.457402211653)) ;
#31131=CARTESIAN_POINT('Ctrl Pts',(-18.5765087687407,5.6802591136536,-332.465342018263)) ;
#31132=CARTESIAN_POINT('Ctrl Pts',(-18.5332081995949,5.81998415168714,-332.467198479046)) ;
#31133=CARTESIAN_POINT('Ctrl Pts',(-18.4217667368634,6.16572931278951,-332.471786494001)) ;
#31134=CARTESIAN_POINT('Ctrl Pts',(-18.3517440861384,6.37112210684672,-332.474506822288)) ;
#31135=CARTESIAN_POINT('Ctrl Pts',(-18.2331939049386,6.70067293632887,-332.478860705002)) ;
#31136=CARTESIAN_POINT('Ctrl Pts',(-18.1868039746501,6.8255797570648,-332.480508418207)) ;
#31137=CARTESIAN_POINT('Ctrl Pts',(-18.0940849993818,7.06757139849144,-332.483696046075)) ;
#31138=CARTESIAN_POINT('Ctrl Pts',(-18.0478953287191,7.18470261663132,-332.485236829812)) ;
#31139=CARTESIAN_POINT('Ctrl Pts',(-17.9321610439444,7.47003005996469,-332.488985931035)) ;
#31140=CARTESIAN_POINT('Ctrl Pts',(-17.8613850174887,7.63771393777761,-332.491185586413)) ;
#31141=CARTESIAN_POINT('Ctrl Pts',(-17.5060943264401,8.44751630380189,-332.501801973352)) ;
#31142=CARTESIAN_POINT('Ctrl Pts',(-17.1892537988264,9.07487878020027,-332.509985568648)) ;
#31143=CARTESIAN_POINT('Ctrl Pts',(-16.681154859224,9.95841987901278,-332.521895121165)) ;
#31144=CARTESIAN_POINT('Ctrl Pts',(-16.5164731476687,10.2292310654247,-332.525604710508)) ;
#31145=CARTESIAN_POINT('Ctrl Pts',(-16.2717131248583,10.6103955832704,-332.530976731591)) ;
#31146=CARTESIAN_POINT('Ctrl Pts',(-16.1969846593275,10.7241237555622,-332.532599465547)) ;
#31147=CARTESIAN_POINT('Ctrl Pts',(-16.0604812899361,10.927184419568,-332.535540293521)) ;
#31148=CARTESIAN_POINT('Ctrl Pts',(-15.9991404240994,11.0168019064017,-332.536853685179)) ;
#31149=CARTESIAN_POINT('Ctrl Pts',(-15.8981493742989,11.1617248321356,-332.539006630466)) ;
#31150=CARTESIAN_POINT('Ctrl Pts',(-15.858954338678,11.2173446968817,-332.539839976194)) ;
#31151=CARTESIAN_POINT('Ctrl Pts',(-15.7760317342591,11.3337129830864,-332.541599483263)) ;
#31152=CARTESIAN_POINT('Ctrl Pts',(-15.7322437134957,11.3944168338817,-332.542526432763)) ;
#31153=CARTESIAN_POINT('Ctrl Pts',(-15.6032171233982,11.5711262614762,-332.545249604931)) ;
#31154=CARTESIAN_POINT('Ctrl Pts',(-15.5170386270037,11.6864391370296,-332.547058134858)) ;
#31155=CARTESIAN_POINT('Ctrl Pts',(-15.0588465204583,12.2855277381321,-332.556597945434)) ;
#31156=CARTESIAN_POINT('Ctrl Pts',(-14.6654691378138,12.7525317234778,-332.564520907751)) ;
#31157=CARTESIAN_POINT('Ctrl Pts',(-14.0150958320654,13.454664007329,-332.576846162247)) ;
#31158=CARTESIAN_POINT('Ctrl Pts',(-13.7726572702083,13.7027299153684,-332.581292063254)) ;
#31159=CARTESIAN_POINT('Ctrl Pts',(-13.3416103969075,14.1207792413035,-332.588907541145)) ;
#31160=CARTESIAN_POINT('Ctrl Pts',(-13.1560707461509,14.2938020574615,-332.592098857732)) ;
#31161=CARTESIAN_POINT('Ctrl Pts',(-12.8631468947255,14.5564283219298,-332.597000238133)) ;
#31162=CARTESIAN_POINT('Ctrl Pts',(-12.758094556452,14.6485895867739,-332.598731794467)) ;
#31163=CARTESIAN_POINT('Ctrl Pts',(-12.5572621011422,14.8209783917265,-332.601993000319)) ;
#31164=CARTESIAN_POINT('Ctrl Pts',(-12.4616845566394,14.9014311400923,-332.603524521271)) ;
#31165=CARTESIAN_POINT('Ctrl Pts',(-12.239634706448,15.0847119185599,-332.607036561693)) ;
#31166=CARTESIAN_POINT('Ctrl Pts',(-12.1126308864883,15.1868813296355,-332.609011539671)) ;
#31167=CARTESIAN_POINT('Ctrl Pts',(-11.6807329638849,15.525461132819,-332.615620354055)) ;
#31168=CARTESIAN_POINT('Ctrl Pts',(-11.3700858147713,15.7543840066875,-332.620195103011)) ;
#31169=CARTESIAN_POINT('Ctrl Pts',(-10.5751372633674,16.3044329621867,-332.631559884871)) ;
#31170=CARTESIAN_POINT('Ctrl Pts',(-10.0828617378029,16.6133669017344,-332.638289209997)) ;
#31171=CARTESIAN_POINT('Ctrl Pts',(-9.46212466471949,16.9651526365882,-332.646694305598)) ;
#31172=CARTESIAN_POINT('Ctrl Pts',(-9.34609816972103,17.0293469077564,-332.648262536072)) ;
#31173=CARTESIAN_POINT('Ctrl Pts',(-9.15871136320605,17.1305309116395,-332.650796593944)) ;
#31174=CARTESIAN_POINT('Ctrl Pts',(-9.0877628722214,17.168274494321,-332.651756344326)) ;
#31175=CARTESIAN_POINT('Ctrl Pts',(-8.91252410717003,17.2601083670129,-332.654129735758)) ;
#31176=CARTESIAN_POINT('Ctrl Pts',(-8.80797349649241,17.3136948577398,-332.655548213167)) ;
#31177=CARTESIAN_POINT('Ctrl Pts',(-8.64063794099014,17.3975532145856,-332.657826942176)) ;
#31178=CARTESIAN_POINT('Ctrl Pts',(-8.57816495760147,17.4284413485401,-332.658679540645)) ;
#31179=CARTESIAN_POINT('Ctrl Pts',(-8.45886878010149,17.4866273995058,-332.660312321856)) ;
#31180=CARTESIAN_POINT('Ctrl Pts',(-8.40207629998039,17.5139862020692,-332.661091591915)) ;
#31181=CARTESIAN_POINT('Ctrl Pts',(-8.23812798589591,17.5919845056805,-332.663345706882)) ;
#31182=CARTESIAN_POINT('Ctrl Pts',(-8.13064064003027,17.6419203682814,-332.664829068499)) ;
#31183=CARTESIAN_POINT('Ctrl Pts',(-7.65866279998202,17.8559594888764,-332.671355872311)) ;
#31184=CARTESIAN_POINT('Ctrl Pts',(-7.28961378087681,18.0097733234336,-332.676491945733)) ;
#31185=CARTESIAN_POINT('Ctrl Pts',(-6.57506149291105,18.2820231290669,-332.686349256319)) ;
#31186=CARTESIAN_POINT('Ctrl Pts',(-6.23044537861813,18.4023192573496,-332.69106594326)) ;
#31187=CARTESIAN_POINT('Ctrl Pts',(-5.60878618085292,18.5998579120733,-332.699437691383)) ;
#31188=CARTESIAN_POINT('Ctrl Pts',(-5.33302918488979,18.6807921919778,-332.703104605044)) ;
#31189=CARTESIAN_POINT('Ctrl Pts',(-4.83922451433934,18.8138975493996,-332.709569592744)) ;
#31190=CARTESIAN_POINT('Ctrl Pts',(-4.6218777917697,18.868467898529,-332.712380843555)) ;
#31191=CARTESIAN_POINT('Ctrl Pts',(-4.27262091889825,18.9497606903381,-332.71684083581)) ;
#31192=CARTESIAN_POINT('Ctrl Pts',(-4.14129308742704,18.978893839237,-332.718505059916)) ;
#31193=CARTESIAN_POINT('Ctrl Pts',(-3.88572102613006,19.0328096983907,-332.72171914528)) ;
#31194=CARTESIAN_POINT('Ctrl Pts',(-3.76151597773658,19.0577456826991,-332.723269946789)) ;
#31195=CARTESIAN_POINT('Ctrl Pts',(-3.46137128063637,19.1149555993557,-332.726991524299)) ;
#31196=CARTESIAN_POINT('Ctrl Pts',(-3.28521240182119,19.1460178186432,-332.729154289542)) ;
#31197=CARTESIAN_POINT('Ctrl Pts',(-2.38620068584094,19.2917682442597,-332.740093801473)) ;
#31198=CARTESIAN_POINT('Ctrl Pts',(-1.65770878656152,19.3679704069865,-332.74861199613)) ;
#31199=CARTESIAN_POINT('Ctrl Pts',(-0.517637276200755,19.4224189521836,
-332.761953595217)) ;
#31200=CARTESIAN_POINT('Ctrl Pts',(-0.108099806806295,19.4290148804684,
-332.766754223067)) ;
#31201=CARTESIAN_POINT('Ctrl Pts',(0.421081211273075,19.4208047584362,-332.773100279281)) ;
#31202=CARTESIAN_POINT('Ctrl Pts',(0.540804409498887,19.4178396681817,-332.774545667479)) ;
#31203=CARTESIAN_POINT('Ctrl Pts',(0.730587800434719,19.4113828853774,-332.776856911019)) ;
#31204=CARTESIAN_POINT('Ctrl Pts',(0.800669779955762,19.4086184967789,-332.777714732002)) ;
#31205=CARTESIAN_POINT('Ctrl Pts',(0.933329644431869,19.4026659695296,-332.779347925939)) ;
#31206=CARTESIAN_POINT('Ctrl Pts',(0.995910069984909,19.3995544812717,-332.780122298234)) ;
#31207=CARTESIAN_POINT('Ctrl Pts',(1.17465513176301,19.3898001151477,-332.782344250563)) ;
#31208=CARTESIAN_POINT('Ctrl Pts',(1.2907765404271,19.3824162334728,-332.783799987968)) ;
#31209=CARTESIAN_POINT('Ctrl Pts',(1.7597563838488,19.3483616931963,-332.789719431497)) ;
#31210=CARTESIAN_POINT('Ctrl Pts',(2.11192170133388,19.3130947471029,-332.794255238131)) ;
#31211=CARTESIAN_POINT('Ctrl Pts',(2.9985047355511,19.1997688963305,-332.805764730046)) ;
#31212=CARTESIAN_POINT('Ctrl Pts',(3.53099754033945,19.1090087269549,-332.812756511182)) ;
#31213=CARTESIAN_POINT('Ctrl Pts',(4.37803642169187,18.9280173990274,-332.823810937845)) ;
#31214=CARTESIAN_POINT('Ctrl Pts',(4.69528922442561,18.8518249892294,-332.827937604129)) ;
#31215=CARTESIAN_POINT('Ctrl Pts',(5.15639586540763,18.7287217355113,-332.833900871855)) ;
#31216=CARTESIAN_POINT('Ctrl Pts',(5.3018595103528,18.6880636231466,-332.835777165975)) ;
#31217=CARTESIAN_POINT('Ctrl Pts',(5.56578347683712,18.6109654665928,-332.839172417575)) ;
#31218=CARTESIAN_POINT('Ctrl Pts',(5.68439749280751,18.5750802555426,-332.840694989585)) ;
#31219=CARTESIAN_POINT('Ctrl Pts',(5.94602210090458,18.4931882740085,-332.844046528912)) ;
#31220=CARTESIAN_POINT('Ctrl Pts',(6.08885885420201,18.4466525227567,-332.845871813009)) ;
#31221=CARTESIAN_POINT('Ctrl Pts',(6.53459891640948,18.2956905004917,-332.851556916245)) ;
#31222=CARTESIAN_POINT('Ctrl Pts',(6.83546749279926,18.1854243461246,-332.855377578623)) ;
#31223=CARTESIAN_POINT('Ctrl Pts',(7.75515833716328,17.8223142726826,-332.86706352596)) ;
#31224=CARTESIAN_POINT('Ctrl Pts',(8.36376086390613,17.5449385488919,-332.87479309188)) ;
#31225=CARTESIAN_POINT('Ctrl Pts',(9.20570521869414,17.107433071553,-332.885958357462)) ;
#31226=CARTESIAN_POINT('Ctrl Pts',(9.4517284328849,16.9727459150251,-332.889283622524)) ;
#31227=CARTESIAN_POINT('Ctrl Pts',(9.77574235800309,16.786131847062,-332.893794817613)) ;
#31228=CARTESIAN_POINT('Ctrl Pts',(9.8563984009187,16.7388999509152,-332.894928942998)) ;
#31229=CARTESIAN_POINT('Ctrl Pts',(9.99336662489437,16.65735861703,-332.896876483446)) ;
#31230=CARTESIAN_POINT('Ctrl Pts',(10.0498506987496,16.6233412264064,-332.897686042666)) ;
#31231=CARTESIAN_POINT('Ctrl Pts',(10.1764089524122,16.5462410276427,-332.89951489572)) ;
#31232=CARTESIAN_POINT('Ctrl Pts',(10.2463847022609,16.5029994795317,-332.900536254257)) ;
#31233=CARTESIAN_POINT('Ctrl Pts',(10.4750458545714,16.3596832119398,-332.903904447575)) ;
#31234=CARTESIAN_POINT('Ctrl Pts',(10.6325562092451,16.2577541100572,-332.906273341475)) ;
#31235=CARTESIAN_POINT('Ctrl Pts',(11.512525695155,15.6700441407369,-332.919733147003)) ;
#31236=CARTESIAN_POINT('Ctrl Pts',(12.2031638722667,15.138405944195,-332.93111674204)) ;
#31237=CARTESIAN_POINT('Ctrl Pts',(13.0556329510556,14.3858305828786,-332.945556867364)) ;
#31238=CARTESIAN_POINT('Ctrl Pts',(13.2518033584738,14.2053293340077,-332.948913822778)) ;
#31239=CARTESIAN_POINT('Ctrl Pts',(13.5466390717352,13.9226196533746,-332.954006002188)) ;
#31240=CARTESIAN_POINT('Ctrl Pts',(13.6480012761273,13.8232712983814,-332.955765583982)) ;
#31241=CARTESIAN_POINT('Ctrl Pts',(13.8362298720489,13.6346936907985,-332.95905017065)) ;
#31242=CARTESIAN_POINT('Ctrl Pts',(13.9233447226969,13.5457226050846,-332.960577402193)) ;
#31243=CARTESIAN_POINT('Ctrl Pts',(14.11985368302,13.3411277824146,-332.964039509232)) ;
#31244=CARTESIAN_POINT('Ctrl Pts',(14.2286942265889,13.2249846591956,-332.965969403081)) ;
#31245=CARTESIAN_POINT('Ctrl Pts',(14.6002130666653,12.8186430556208,-332.972604926997)) ;
#31246=CARTESIAN_POINT('Ctrl Pts',(14.8555396680625,12.5218518400703,-332.977248349292)) ;
#31247=CARTESIAN_POINT('Ctrl Pts',(15.4694125434608,11.7630630501135,-332.988724987734)) ;
#31248=CARTESIAN_POINT('Ctrl Pts',(15.8163948939545,11.292210924903,-332.995496618422)) ;
#31249=CARTESIAN_POINT('Ctrl Pts',(16.2155983937038,10.6959188602019,-333.003949500851)) ;
#31250=CARTESIAN_POINT('Ctrl Pts',(16.2884462982189,10.5846506162908,-333.005522292819)) ;
#31251=CARTESIAN_POINT('Ctrl Pts',(16.403561993799,10.4048192664751,-333.008062902962)) ;
#31252=CARTESIAN_POINT('Ctrl Pts',(16.4465560073873,10.336726054856,-333.00902460996)) ;
#31253=CARTESIAN_POINT('Ctrl Pts',(16.5513203752515,10.168493588557,-333.011402025205)) ;
#31254=CARTESIAN_POINT('Ctrl Pts',(16.612606688774,10.0680567622816,-333.012822575403)) ;
#31255=CARTESIAN_POINT('Ctrl Pts',(16.708753103041,9.90722243438955,-333.015103805458)) ;
#31256=CARTESIAN_POINT('Ctrl Pts',(16.7442070469886,9.84718320068299,-333.015956802993)) ;
#31257=CARTESIAN_POINT('Ctrl Pts',(16.8110823292512,9.73252823750605,-333.01758959551)) ;
#31258=CARTESIAN_POINT('Ctrl Pts',(16.8425626827219,9.67794798715886,-333.018368470866)) ;
#31259=CARTESIAN_POINT('Ctrl Pts',(16.9324052968254,9.52041392657122,-333.020620005819)) ;
#31260=CARTESIAN_POINT('Ctrl Pts',(16.9900929482566,9.41707874115112,-333.022101153134)) ;
#31261=CARTESIAN_POINT('Ctrl Pts',(17.3571183864579,8.74527895506652,-333.031741881167)) ;
#31262=CARTESIAN_POINT('Ctrl Pts',(17.6388271783303,8.16218343631383,-333.040148176756)) ;
#31263=CARTESIAN_POINT('Ctrl Pts',(18.0275342779838,7.24304337877152,-333.053002058919)) ;
#31264=CARTESIAN_POINT('Ctrl Pts',(18.1553873651541,6.91632704941147,-333.057500179498)) ;
#31265=CARTESIAN_POINT('Ctrl Pts',(18.3609612707661,6.34594487241042,-333.065190985208)) ;
#31266=CARTESIAN_POINT('Ctrl Pts',(18.4428474099819,6.10387540020582,-333.068406056403)) ;
#31267=CARTESIAN_POINT('Ctrl Pts',(18.562189085288,5.72672494866377,-333.073334865681)) ;
#31268=CARTESIAN_POINT('Ctrl Pts',(18.6029983375919,5.59273593100718,-333.075070497916)) ;
#31269=CARTESIAN_POINT('Ctrl Pts',(18.6774395802552,5.33848905934159,-333.078334996046)) ;
#31270=CARTESIAN_POINT('Ctrl Pts',(18.711368072532,5.2183253647359,-333.079865785902)) ;
#31271=CARTESIAN_POINT('Ctrl Pts',(18.7867547087438,4.94113805520366,-333.083369996614)) ;
#31272=CARTESIAN_POINT('Ctrl Pts',(18.8274069419168,4.78390485994989,-333.085337963309)) ;
#31273=CARTESIAN_POINT('Ctrl Pts',(18.9674860778513,4.21264640956687,-333.092421980478)) ;
#31274=CARTESIAN_POINT('Ctrl Pts',(19.0552654038366,3.79588980486646,-333.097462568134)) ;
#31275=CARTESIAN_POINT('Ctrl Pts',(19.2249088583184,2.83481333668933,-333.108917883733)) ;
#31276=CARTESIAN_POINT('Ctrl Pts',(19.29748011242,2.28922411432976,-333.115295851395)) ;
#31277=CARTESIAN_POINT('Ctrl Pts',(19.3583782397329,1.61260980982352,-333.12330253624)) ;
#31278=CARTESIAN_POINT('Ctrl Pts',(19.368676077332,1.48381448806581,-333.124831359226)) ;
#31279=CARTESIAN_POINT('Ctrl Pts',(19.3890957028787,1.19178001904634,-333.128316197844)) ;
#31280=CARTESIAN_POINT('Ctrl Pts',(19.3984423736851,1.02849653318006,-333.130277594457)) ;
#31281=CARTESIAN_POINT('Ctrl Pts',(19.409215878971,0.786831851089578,-333.133210631411)) ;
#31282=CARTESIAN_POINT('Ctrl Pts',(19.4122320366345,0.708528569487368,-333.134165662925)) ;
#31283=CARTESIAN_POINT('Ctrl Pts',(19.4169380638603,0.563550603007795,-333.13594416531)) ;
#31284=CARTESIAN_POINT('Ctrl Pts',(19.4187585037866,0.496881468035375,-333.13676618588)) ;
#31285=CARTESIAN_POINT('Ctrl Pts',(19.422452487332,0.330128079846534,-333.13883191478)) ;
#31286=CARTESIAN_POINT('Ctrl Pts',(19.4238958101808,0.230036274229013,-333.140080445144)) ;
#31287=CARTESIAN_POINT('Ctrl Pts',(19.4270698777963,-0.244458714760322,
-333.14603287715)) ;
#31288=CARTESIAN_POINT('Ctrl Pts',(19.4187494218004,-0.618848962459257,
-333.150827319851)) ;
#31289=CARTESIAN_POINT('Ctrl Pts',(19.3780453184075,-1.41424887511556,-333.161079880492)) ;
#31290=CARTESIAN_POINT('Ctrl Pts',(19.3427456569787,-1.83491993450364,-333.166541354533)) ;
#31291=CARTESIAN_POINT('Ctrl Pts',(19.2601708873612,-2.54170945163216,-333.175675757334)) ;
#31292=CARTESIAN_POINT('Ctrl Pts',(19.2201434189485,-2.82852557794944,-333.179371529156)) ;
#31293=CARTESIAN_POINT('Ctrl Pts',(19.1376070818677,-3.33666811908569,-333.185880055281)) ;
#31294=CARTESIAN_POINT('Ctrl Pts',(19.0976305425937,-3.55835170827102,-333.188706267461)) ;
#31295=CARTESIAN_POINT('Ctrl Pts',(19.0275956722537,-3.91144208003365,-333.193183707811)) ;
#31296=CARTESIAN_POINT('Ctrl Pts',(19.0000093963871,-4.04331784664598,-333.194850640627)) ;
#31297=CARTESIAN_POINT('Ctrl Pts',(18.9438480090212,-4.29851957321614,-333.198066286175)) ;
#31298=CARTESIAN_POINT('Ctrl Pts',(18.9154348509784,-4.42187430369103,-333.199615979712)) ;
#31299=CARTESIAN_POINT('Ctrl Pts',(18.8441201687388,-4.71821162476563,-333.203328665025)) ;
#31300=CARTESIAN_POINT('Ctrl Pts',(18.8000397681945,-4.89089876322019,-333.205483748462)) ;
#31301=CARTESIAN_POINT('Ctrl Pts',(18.5618979501145,-5.77299505741351,-333.216459641285)) ;
#31302=CARTESIAN_POINT('Ctrl Pts',(18.3300361759063,-6.47157643830683,-333.225018562004)) ;
#31303=CARTESIAN_POINT('Ctrl Pts',(17.9089230325428,-7.53441237786723,-333.238382301947)) ;
#31304=CARTESIAN_POINT('Ctrl Pts',(17.7468226703079,-7.90867736604197,-333.243163215145)) ;
#31305=CARTESIAN_POINT('Ctrl Pts',(17.522114550048,-8.38572730206592,-333.249486482239)) ;
#31306=CARTESIAN_POINT('Ctrl Pts',(17.4701670450243,-8.49342004410461,-333.250929590514)) ;
#31307=CARTESIAN_POINT('Ctrl Pts',(17.3861919973148,-8.66347889543662,-333.253238075894)) ;
#31308=CARTESIAN_POINT('Ctrl Pts',(17.3548153459296,-8.72616313401462,-333.25409545113)) ;
#31309=CARTESIAN_POINT('Ctrl Pts',(17.2947373336564,-8.8445811305174,-333.255728588559)) ;
#31310=CARTESIAN_POINT('Ctrl Pts',(17.2661041365587,-8.90034846222215,-333.256503357367)) ;
#31311=CARTESIAN_POINT('Ctrl Pts',(17.1834748891403,-9.05938159961081,-333.258727926446)) ;
#31312=CARTESIAN_POINT('Ctrl Pts',(17.1288189211743,-9.16230137789719,-333.260185913156)) ;
#31313=CARTESIAN_POINT('Ctrl Pts',(16.90332863112,-9.57783996479055,-333.266137820814)) ;
#31314=CARTESIAN_POINT('Ctrl Pts',(16.7248356904525,-9.88622311924342,-333.27070483042)) ;
#31315=CARTESIAN_POINT('Ctrl Pts',(16.484558840113,-10.2762011549869,-333.27660368282)) ;
#31316=CARTESIAN_POINT('Ctrl Pts',(16.4304729180761,-10.3624586857424,-333.27791649911)) ;
#31317=CARTESIAN_POINT('Ctrl Pts',(16.1236353937982,-10.8433684022128,-333.285275320516)) ;
#31318=CARTESIAN_POINT('Ctrl Pts',(15.8573438776645,-11.2291986851869,-333.291325147242)) ;
#31319=CARTESIAN_POINT('Ctrl Pts',(15.4908284405833,-11.7211704948601,-333.299141011212)) ;
#31320=CARTESIAN_POINT('Ctrl Pts',(15.4030008387464,-11.8363494696315,-333.300978845954)) ;
#31321=CARTESIAN_POINT('Ctrl Pts',(15.1813009182394,-12.120444598585,-333.305529407308)) ;
#31322=CARTESIAN_POINT('Ctrl Pts',(15.0458898880883,-12.2881354381344,-333.308230978633)) ;
#31323=CARTESIAN_POINT('Ctrl Pts',(14.8224643107209,-12.5555907606716,-333.312562959636)) ;
#31324=CARTESIAN_POINT('Ctrl Pts',(14.7361665580548,-12.65676510103,-333.314207260307)) ;
#31325=CARTESIAN_POINT('Ctrl Pts',(14.5660524821867,-12.8521060465932,-333.317393203597)) ;
#31326=CARTESIAN_POINT('Ctrl Pts',(14.4823448536997,-12.9463586515116,-333.318935661738)) ;
#31327=CARTESIAN_POINT('Ctrl Pts',(14.2947016590603,-13.1535426070349,-333.322338891705)) ;
#31328=CARTESIAN_POINT('Ctrl Pts',(14.1903330704038,-13.2660704833762,-333.324195790675)) ;
#31329=CARTESIAN_POINT('Ctrl Pts',(13.7594534229826,-13.7197317547138,-333.331722487689)) ;
#31330=CARTESIAN_POINT('Ctrl Pts',(13.421888348565,-14.0501427902272,-333.337295314231)) ;
#31331=CARTESIAN_POINT('Ctrl Pts',(12.7015345834842,-14.7055548048673,-333.348702412302)) ;
#31332=CARTESIAN_POINT('Ctrl Pts',(12.317509887149,-15.0286816392346,-333.354526683944)) ;
#31333=CARTESIAN_POINT('Ctrl Pts',(11.8240181317288,-15.4122819906828,-333.361899701347)) ;
#31334=CARTESIAN_POINT('Ctrl Pts',(11.7259087475863,-15.487056044977,-333.363360570929)) ;
#31335=CARTESIAN_POINT('Ctrl Pts',(11.5001026505558,-15.6557783104405,-333.366718420019)) ;
#31336=CARTESIAN_POINT('Ctrl Pts',(11.3719547499849,-15.7491079274222,-333.368620831042)) ;
#31337=CARTESIAN_POINT('Ctrl Pts',(11.1794869001049,-15.8857074864134,-333.371483458221)) ;
#31338=CARTESIAN_POINT('Ctrl Pts',(11.116027001697,-15.9301780709183,-333.372428175945)) ;
#31339=CARTESIAN_POINT('Ctrl Pts',(10.9972409608892,-16.0123639533652,-333.374199691141)) ;
#31340=CARTESIAN_POINT('Ctrl Pts',(10.9419827254241,-16.0501751431529,-333.375025190049)) ;
#31341=CARTESIAN_POINT('Ctrl Pts',(10.8021120515768,-16.1448254862809,-333.37711742042)) ;
#31342=CARTESIAN_POINT('Ctrl Pts',(10.7172456875459,-16.2012857387479,-333.378389255005)) ;
#31343=CARTESIAN_POINT('Ctrl Pts',(10.3246394516554,-16.4580456695274,-333.384276581815)) ;
#31344=CARTESIAN_POINT('Ctrl Pts',(10.0117038658228,-16.6502622160299,-333.388977930046)) ;
#31345=CARTESIAN_POINT('Ctrl Pts',(9.21641465754357,-17.108226793826,-333.400790599979)) ;
#31346=CARTESIAN_POINT('Ctrl Pts',(8.72785441120039,-17.3625540304771,-333.407922750224)) ;
#31347=CARTESIAN_POINT('Ctrl Pts',(8.02100651293836,-17.6931308867377,-333.417883994498)) ;
#31348=CARTESIAN_POINT('Ctrl Pts',(7.81114898600246,-17.7867753631974,-333.420799568417)) ;
#31349=CARTESIAN_POINT('Ctrl Pts',(7.42322370461186,-17.9516890171919,-333.42610525806)) ;
#31350=CARTESIAN_POINT('Ctrl Pts',(7.24566690246012,-18.0240866632313,-333.42850221011)) ;
#31351=CARTESIAN_POINT('Ctrl Pts',(6.94712249236005,-18.1406917051086,-333.432478913702)) ;
#31352=CARTESIAN_POINT('Ctrl Pts',(6.82671479110414,-18.1863457482993,-333.434068452753)) ;
#31353=CARTESIAN_POINT('Ctrl Pts',(6.5972197469767,-18.2707612514217,-333.437071326147)) ;
#31354=CARTESIAN_POINT('Ctrl Pts',(6.48822241123192,-18.3097513657635,-333.438486180836)) ;
#31355=CARTESIAN_POINT('Ctrl Pts',(6.19881025011907,-18.4103699602981,-333.442213941053)) ;
#31356=CARTESIAN_POINT('Ctrl Pts',(6.0178254491308,-18.4703207229875,-333.444515410412)) ;
#31357=CARTESIAN_POINT('Ctrl Pts',(5.25501892101676,-18.7105963011268,-333.454103335524)) ;
#31358=CARTESIAN_POINT('Ctrl Pts',(4.6657639393848,-18.8661677606078,-333.461226575795)) ;
#31359=CARTESIAN_POINT('Ctrl Pts',(3.71107003857639,-19.0707488819094,-333.472629833237)) ;
#31360=CARTESIAN_POINT('Ctrl Pts',(3.34985446408966,-19.1375018783846,-333.47691651829)) ;
#31361=CARTESIAN_POINT('Ctrl Pts',(2.84128348302247,-19.2166456540221,-333.483008777668)) ;
#31362=CARTESIAN_POINT('Ctrl Pts',(2.69534889049852,-19.2376572454649,-333.484763668503)) ;
#31363=CARTESIAN_POINT('Ctrl Pts',(2.43502184707032,-19.2721186238964,-333.487915387629)) ;
#31364=CARTESIAN_POINT('Ctrl Pts',(2.32072221776043,-19.2862162172956,-333.489306460008)) ;
#31365=CARTESIAN_POINT('Ctrl Pts',(2.13750616189181,-19.3071615580235,-333.491552181983)) ;
#31366=CARTESIAN_POINT('Ctrl Pts',(2.0686666245353,-19.3146586409899,-333.492399561775)) ;
#31367=CARTESIAN_POINT('Ctrl Pts',(1.93665750548425,-19.3283214718026,-333.494032544694)) ;
#31368=CARTESIAN_POINT('Ctrl Pts',(1.8734949467549,-19.3345460221858,-333.494817329822)) ;
#31369=CARTESIAN_POINT('Ctrl Pts',(1.68990157678104,-19.3517307026508,-333.497107314673)) ;
#31370=CARTESIAN_POINT('Ctrl Pts',(1.56939759749294,-19.3618759329444,-333.498621437269)) ;
#31371=CARTESIAN_POINT('Ctrl Pts',(0.966876196038792,-19.4069403018975,
-333.506234317399)) ;
#31372=CARTESIAN_POINT('Ctrl Pts',(0.483768668098201,-19.42498772913,-333.512469026684)) ;
#31373=CARTESIAN_POINT('Ctrl Pts',(0.000492969417159733,-19.4249999937447,
-333.518704187163)) ;
#31374=CARTESIAN_POINT('Origin',(0.,0.,-328.125)) ;
#31375=CARTESIAN_POINT('',(-0.000504255346276296,-19.424999993455,-335.231156847152)) ;
#31376=CARTESIAN_POINT('',(-0.000488271649964467,-19.425000024638,-335.01863418612)) ;
#31377=CARTESIAN_POINT('',(-2.37887640734373E-15,-19.425,-328.125)) ;
#31378=CARTESIAN_POINT('Ctrl Pts',(-0.000504255346276296,-19.424999993455,
-335.231156847152)) ;
#31379=CARTESIAN_POINT('Ctrl Pts',(0.401697001557673,-19.4250104342341,
-335.226213897056)) ;
#31380=CARTESIAN_POINT('Ctrl Pts',(0.803933718099742,-19.4125249605364,
-335.22127094696)) ;
#31381=CARTESIAN_POINT('Ctrl Pts',(1.20541431535202,-19.3875630580108,-335.216327996863)) ;
#31382=CARTESIAN_POINT('Ctrl Pts',(1.60686285129883,-19.3626031488845,-335.2113854415)) ;
#31383=CARTESIAN_POINT('Ctrl Pts',(2.00755514881831,-19.3251688159696,-335.206442886136)) ;
#31384=CARTESIAN_POINT('Ctrl Pts',(2.40670260443344,-19.2753315814233,-335.201500330772)) ;
#31385=CARTESIAN_POINT('Ctrl Pts',(2.80884240561074,-19.2251207249848,-335.19652072185)) ;
#31386=CARTESIAN_POINT('Ctrl Pts',(3.209413862284,-19.1623202687843,-335.191541112928)) ;
#31387=CARTESIAN_POINT('Ctrl Pts',(3.60761705354232,-19.0870564570599,-335.186561504006)) ;
#31388=CARTESIAN_POINT('Ctrl Pts',(4.00289111256762,-19.0123462764005,-335.181618524456)) ;
#31389=CARTESIAN_POINT('Ctrl Pts',(4.39583139329134,-18.9253555340871,-335.176675544907)) ;
#31390=CARTESIAN_POINT('Ctrl Pts',(4.78566548879298,-18.8262590768686,-335.171732565357)) ;
#31391=CARTESIAN_POINT('Ctrl Pts',(5.1798328143229,-18.7260611055724,-335.166734641749)) ;
#31392=CARTESIAN_POINT('Ctrl Pts',(5.5708242503035,-18.6134867699796,-335.16173671814)) ;
#31393=CARTESIAN_POINT('Ctrl Pts',(5.95785535789883,-18.4887691460074,-335.156738794532)) ;
#31394=CARTESIAN_POINT('Ctrl Pts',(6.34488646549424,-18.3640515220352,-335.151740870923)) ;
#31395=CARTESIAN_POINT('Ctrl Pts',(6.72795700563771,-18.2271906946848,-335.146742947315)) ;
#31396=CARTESIAN_POINT('Ctrl Pts',(7.10630024801675,-18.0784712236693,-335.141745023707)) ;
#31397=CARTESIAN_POINT('Ctrl Pts',(7.48194286066495,-17.9308133183961,-335.136782775484)) ;
#31398=CARTESIAN_POINT('Ctrl Pts',(7.85303165451542,-17.7714238280823,-335.131820527261)) ;
#31399=CARTESIAN_POINT('Ctrl Pts',(8.21883012953624,-17.600609543474,-335.126858279038)) ;
#31400=CARTESIAN_POINT('Ctrl Pts',(8.58435151182593,-17.4299246508666,-335.121899789724)) ;
#31401=CARTESIAN_POINT('Ctrl Pts',(8.94459037186042,-17.2478323664877,-335.116941300409)) ;
#31402=CARTESIAN_POINT('Ctrl Pts',(9.29883308421554,-17.0546864020391,-335.111982811095)) ;
#31403=CARTESIAN_POINT('Ctrl Pts',(9.65303778078999,-16.8615611651719,-335.107024853904)) ;
#31404=CARTESIAN_POINT('Ctrl Pts',(10.0012474066032,-16.6573847311153,-335.102066896713)) ;
#31405=CARTESIAN_POINT('Ctrl Pts',(10.3427729638405,-16.4425567482205,-335.097108939522)) ;
#31406=CARTESIAN_POINT('Ctrl Pts',(10.6842777656993,-16.2277418209696,-335.092151283638)) ;
#31407=CARTESIAN_POINT('Ctrl Pts',(11.0190991096253,-16.0022767644142,-335.087193627755)) ;
#31408=CARTESIAN_POINT('Ctrl Pts',(11.346575608599,-15.7666054354876,-335.082235971871)) ;
#31409=CARTESIAN_POINT('Ctrl Pts',(11.6745642237066,-15.5305655577025,-335.077270563079)) ;
#31410=CARTESIAN_POINT('Ctrl Pts',(11.9951848021529,-15.2842875892346,-335.072305154286)) ;
#31411=CARTESIAN_POINT('Ctrl Pts',(12.3078034626076,-15.0282600099221,-335.067339745493)) ;
#31412=CARTESIAN_POINT('Ctrl Pts',(12.6199660245349,-14.7726059649396,-335.06238158104)) ;
#31413=CARTESIAN_POINT('Ctrl Pts',(12.9241498258517,-14.5072308991849,-335.057423416587)) ;
#31414=CARTESIAN_POINT('Ctrl Pts',(13.2197570537452,-14.2326613266793,-335.052465252133)) ;
#31415=CARTESIAN_POINT('Ctrl Pts',(13.5160121461063,-13.957489996662,-335.047496221171)) ;
#31416=CARTESIAN_POINT('Ctrl Pts',(13.8036528449718,-13.6730839657378,-335.042527190209)) ;
#31417=CARTESIAN_POINT('Ctrl Pts',(14.0821136007754,-13.380011268114,-335.037558159247)) ;
#31418=CARTESIAN_POINT('Ctrl Pts',(14.3605743565788,-13.0869385704903,-335.032589128284)) ;
#31419=CARTESIAN_POINT('Ctrl Pts',(14.6298550090504,-12.7851993845068,-335.027620097322)) ;
#31420=CARTESIAN_POINT('Ctrl Pts',(14.8894287474079,-12.4753972512247,-335.02265106636)) ;
#31421=CARTESIAN_POINT('Ctrl Pts',(15.148648166975,-12.1660179986153,-335.017688818137)) ;
#31422=CARTESIAN_POINT('Ctrl Pts',(15.3982560705094,-11.8485155623468,-335.012726569915)) ;
#31423=CARTESIAN_POINT('Ctrl Pts',(15.6377524923644,-11.5235117037972,-335.007764321692)) ;
#31424=CARTESIAN_POINT('Ctrl Pts',(15.8770674954108,-11.1987540360355,-335.002805832378)) ;
#31425=CARTESIAN_POINT('Ctrl Pts',(16.1062861889675,-10.8665064975775,-334.997847343064)) ;
#31426=CARTESIAN_POINT('Ctrl Pts',(16.3249511423696,-10.5274211086688,-334.992888853749)) ;
#31427=CARTESIAN_POINT('Ctrl Pts',(16.5435926296039,-10.1883721089232,-334.987930896559)) ;
#31428=CARTESIAN_POINT('Ctrl Pts',(16.7516825102272,-9.84248692379159,-334.982972939368)) ;
#31429=CARTESIAN_POINT('Ctrl Pts',(16.9488069570013,-9.49044612936103,-334.978014982177)) ;
#31430=CARTESIAN_POINT('Ctrl Pts',(17.1459194240202,-9.13842672934713,-334.973057326295)) ;
#31431=CARTESIAN_POINT('Ctrl Pts',(17.3320676725531,-8.78025267442093,-334.968099670412)) ;
#31432=CARTESIAN_POINT('Ctrl Pts',(17.5068832716601,-8.41663015181654,-334.963142014529)) ;
#31433=CARTESIAN_POINT('Ctrl Pts',(17.681972251898,-8.0524389869573,-334.958176605736)) ;
#31434=CARTESIAN_POINT('Ctrl Pts',(17.8456929947439,-7.68278250932546,-334.953211196943)) ;
#31435=CARTESIAN_POINT('Ctrl Pts',(17.9977225714819,-7.30839293141586,-334.94824578815)) ;
#31436=CARTESIAN_POINT('Ctrl Pts',(18.1495303429329,-6.93454957345618,-334.943287623697)) ;
#31437=CARTESIAN_POINT('Ctrl Pts',(18.2896809616296,-6.555987141927,-334.938329459244)) ;
#31438=CARTESIAN_POINT('Ctrl Pts',(18.4179013681401,-6.17345399217179,-334.933371294792)) ;
#31439=CARTESIAN_POINT('Ctrl Pts',(18.5464027875771,-5.79008246759955,-334.928402263829)) ;
#31440=CARTESIAN_POINT('Ctrl Pts',(18.6629215540654,-5.40272302320347,-334.923433232866)) ;
#31441=CARTESIAN_POINT('Ctrl Pts',(18.7672328037281,-5.0121450388703,-334.918464201903)) ;
#31442=CARTESIAN_POINT('Ctrl Pts',(18.8715440533908,-4.62156705453713,-334.913495170941)) ;
#31443=CARTESIAN_POINT('Ctrl Pts',(18.9636477308124,-4.22777076354923,-334.908526139978)) ;
#31444=CARTESIAN_POINT('Ctrl Pts',(19.0433699771015,-3.83153819180081,-334.903557109015)) ;
#31445=CARTESIAN_POINT('Ctrl Pts',(19.1229834023199,-3.43584647852945,-334.898594860793)) ;
#31446=CARTESIAN_POINT('Ctrl Pts',(19.1902703496577,-3.03761994844676,-334.89363261257)) ;
#31447=CARTESIAN_POINT('Ctrl Pts',(19.2450892507532,-2.63764378386144,-334.888670364347)) ;
#31448=CARTESIAN_POINT('Ctrl Pts',(19.2998666264733,-2.23797060164256,-334.883711875033)) ;
#31449=CARTESIAN_POINT('Ctrl Pts',(19.3421948056454,-1.83655066995297,-334.878753385718)) ;
#31450=CARTESIAN_POINT('Ctrl Pts',(19.3719840476789,-1.43417539250789,-334.873794896404)) ;
#31451=CARTESIAN_POINT('Ctrl Pts',(19.4017700928612,-1.03184329621813,-334.868836939213)) ;
#31452=CARTESIAN_POINT('Ctrl Pts',(19.4190198710382,-0.628556295574683,
-334.863878982022)) ;
#31453=CARTESIAN_POINT('Ctrl Pts',(19.4236955928532,-0.225110009052542,
-334.858921024831)) ;
#31454=CARTESIAN_POINT('Ctrl Pts',(19.4283710305126,0.178311759007074,-334.853963368947)) ;
#31455=CARTESIAN_POINT('Ctrl Pts',(19.4204739356573,0.5818925563304,-334.849005713064)) ;
#31456=CARTESIAN_POINT('Ctrl Pts',(19.4000186357227,0.984835993256649,-334.84404805718)) ;
#31457=CARTESIAN_POINT('Ctrl Pts',(19.3795313472662,1.38840956344723,-334.839082648388)) ;
#31458=CARTESIAN_POINT('Ctrl Pts',(19.3464465438132,1.79134353924963,-334.834117239595)) ;
#31459=CARTESIAN_POINT('Ctrl Pts',(19.3008309607296,2.19284044685003,-334.829151830803)) ;
#31460=CARTESIAN_POINT('Ctrl Pts',(19.2552819290164,2.59375158599994,-334.824193666349)) ;
#31461=CARTESIAN_POINT('Ctrl Pts',(19.1972386964926,2.99322961251154,-334.819235501896)) ;
#31462=CARTESIAN_POINT('Ctrl Pts',(19.1268195133082,3.39048673575542,-334.814277337443)) ;
#31463=CARTESIAN_POINT('Ctrl Pts',(19.0562459966626,3.78861450338956,-334.80930830648)) ;
#31464=CARTESIAN_POINT('Ctrl Pts',(18.9732422499562,4.18451138403192,-334.804339275518)) ;
#31465=CARTESIAN_POINT('Ctrl Pts',(18.8779789038953,4.57739418272927,-334.799370244556)) ;
#31466=CARTESIAN_POINT('Ctrl Pts',(18.7827155578344,4.97027698142663,-334.794401213594)) ;
#31467=CARTESIAN_POINT('Ctrl Pts',(18.6751926753652,5.36014546681486,-334.789432182632)) ;
#31468=CARTESIAN_POINT('Ctrl Pts',(18.5556317262961,5.74622974114971,-334.784463151669)) ;
#31469=CARTESIAN_POINT('Ctrl Pts',(18.4362339782159,6.13178700950241,-334.779500903447)) ;
#31470=CARTESIAN_POINT('Ctrl Pts',(18.304799277508,6.51367288511617,-334.774538655224)) ;
#31471=CARTESIAN_POINT('Ctrl Pts',(18.1615789593283,6.89113014708642,-334.769576407001)) ;
#31472=CARTESIAN_POINT('Ctrl Pts',(18.0184671306969,7.26830148476646,-334.764617917687)) ;
#31473=CARTESIAN_POINT('Ctrl Pts',(17.8635876173225,7.64105069352826,-334.759659428373)) ;
#31474=CARTESIAN_POINT('Ctrl Pts',(17.6972402422889,8.00863988494365,-334.754700939059)) ;
#31475=CARTESIAN_POINT('Ctrl Pts',(17.5309107189271,8.3761896282968,-334.749742981868)) ;
#31476=CARTESIAN_POINT('Ctrl Pts',(17.3531158898041,8.73858024415288,-334.744785024677)) ;
#31477=CARTESIAN_POINT('Ctrl Pts',(17.1642032143184,9.09509499772164,-334.739827067486)) ;
#31478=CARTESIAN_POINT('Ctrl Pts',(16.9753020195385,9.45158808497829,-334.734869411603)) ;
#31479=CARTESIAN_POINT('Ctrl Pts',(16.7752844393008,9.80220581365237,-334.72991175572)) ;
#31480=CARTESIAN_POINT('Ctrl Pts',(16.5645440672102,10.1462557057,-334.724954099837)) ;
#31481=CARTESIAN_POINT('Ctrl Pts',(16.3534741339166,10.4908436317998,-334.719988691044)) ;
#31482=CARTESIAN_POINT('Ctrl Pts',(16.1316479583973,10.8288429527156,-334.715023282251)) ;
#31483=CARTESIAN_POINT('Ctrl Pts',(15.899505673852,11.1595853116121,-334.710057873459)) ;
#31484=CARTESIAN_POINT('Ctrl Pts',(15.6677020759331,11.4898451301822,-334.705099709006)) ;
#31485=CARTESIAN_POINT('Ctrl Pts',(15.4256125974639,11.8128689604294,-334.700141544553)) ;
#31486=CARTESIAN_POINT('Ctrl Pts',(15.173717975584,12.1280215945322,-334.6951833801)) ;
#31487=CARTESIAN_POINT('Ctrl Pts',(14.9212712914812,12.4438649296211,-334.690214349137)) ;
#31488=CARTESIAN_POINT('Ctrl Pts',(14.6589765761222,12.7518023329777,-334.685245318175)) ;
#31489=CARTESIAN_POINT('Ctrl Pts',(14.3873583648343,13.0512276925136,-334.680276287212)) ;
#31490=CARTESIAN_POINT('Ctrl Pts',(14.1157401535463,13.3506530520495,-334.67530725625)) ;
#31491=CARTESIAN_POINT('Ctrl Pts',(13.8347986122943,13.6415661947121,-334.670338225287)) ;
#31492=CARTESIAN_POINT('Ctrl Pts',(13.5450965579716,13.9233970077429,-334.665369194325)) ;
#31493=CARTESIAN_POINT('Ctrl Pts',(13.255789947683,14.2048431210039,-334.660406946102)) ;
#31494=CARTESIAN_POINT('Ctrl Pts',(12.9576698274976,14.4773065065886,-334.655444697879)) ;
#31495=CARTESIAN_POINT('Ctrl Pts',(12.6513191750186,14.7402424719476,-334.650482449656)) ;
#31496=CARTESIAN_POINT('Ctrl Pts',(12.3452005834881,15.0029792630302,-334.645523960342)) ;
#31497=CARTESIAN_POINT('Ctrl Pts',(12.0308641044568,15.2562029077659,-334.640565471028)) ;
#31498=CARTESIAN_POINT('Ctrl Pts',(11.7089260450411,15.4994088878176,-334.635606981713)) ;
#31499=CARTESIAN_POINT('Ctrl Pts',(11.3870225346129,15.7425887680648,-334.630649024522)) ;
#31500=CARTESIAN_POINT('Ctrl Pts',(11.0575192624823,15.9757529878346,-334.625691067331)) ;
#31501=CARTESIAN_POINT('Ctrl Pts',(10.7210642461646,16.198438394784,-334.62073311014)) ;
#31502=CARTESIAN_POINT('Ctrl Pts',(10.3846296770743,16.4211102685745,-334.615775454257)) ;
#31503=CARTESIAN_POINT('Ctrl Pts',(10.0412444056747,16.6333044707947,-334.610817798374)) ;
#31504=CARTESIAN_POINT('Ctrl Pts',(9.69158535623311,16.8346012213788,-334.60586014249)) ;
#31505=CARTESIAN_POINT('Ctrl Pts',(9.34137950100503,17.0362127649825,-334.600894733698)) ;
#31506=CARTESIAN_POINT('Ctrl Pts',(8.98488043018721,17.2268926160082,-334.595929324905)) ;
#31507=CARTESIAN_POINT('Ctrl Pts',(8.62279439562653,17.4062644415955,-334.590963916112)) ;
#31508=CARTESIAN_POINT('Ctrl Pts',(8.261236630593,17.5853745706233,-334.586005751659)) ;
#31509=CARTESIAN_POINT('Ctrl Pts',(7.8941084119804,17.7532095538587,-334.581047587206)) ;
#31510=CARTESIAN_POINT('Ctrl Pts',(7.52213578782325,17.9094415934598,-334.576089422753)) ;
#31511=CARTESIAN_POINT('Ctrl Pts',(7.14934793375844,18.066016037375,-334.57112039179)) ;
#31512=CARTESIAN_POINT('Ctrl Pts',(6.77169463145451,18.2109365167461,-334.566151360828)) ;
#31513=CARTESIAN_POINT('Ctrl Pts',(6.38992646928316,18.3439217376534,-334.561182329866)) ;
#31514=CARTESIAN_POINT('Ctrl Pts',(6.0081583071118,18.4769069585608,-334.556213298903)) ;
#31515=CARTESIAN_POINT('Ctrl Pts',(5.62227551360419,18.5979568484436,-334.551244267941)) ;
#31516=CARTESIAN_POINT('Ctrl Pts',(5.23304507031604,18.7068400402644,-334.546275236979)) ;
#31517=CARTESIAN_POINT('Ctrl Pts',(4.84434592755306,18.8155746062571,-334.541312988756)) ;
#31518=CARTESIAN_POINT('Ctrl Pts',(4.45220494496474,18.9122045825489,-334.536350740533)) ;
#31519=CARTESIAN_POINT('Ctrl Pts',(4.057394646156,18.9965305696947,-334.53138849231)) ;
#31520=CARTESIAN_POINT('Ctrl Pts',(3.66288341657788,19.0807926798135,-334.526430002996)) ;
#31521=CARTESIAN_POINT('Ctrl Pts',(3.26570714556296,19.1527693846673,-334.521471513682)) ;
#31522=CARTESIAN_POINT('Ctrl Pts',(2.86664840399438,19.212312508594,-334.516513024367)) ;
#31523=CARTESIAN_POINT('Ctrl Pts',(2.46763248766517,19.2718492426129,-334.511555067177)) ;
#31524=CARTESIAN_POINT('Ctrl Pts',(2.06673473895779,19.3189550257579,-334.506597109986)) ;
#31525=CARTESIAN_POINT('Ctrl Pts',(1.66474578406556,19.3535331780643,-334.501639152795)) ;
#31526=CARTESIAN_POINT('Ctrl Pts',(1.26278125907246,19.3881092289677,-334.496681496912)) ;
#31527=CARTESIAN_POINT('Ctrl Pts',(0.85972589679546,19.4101591496573,-334.491723841029)) ;
#31528=CARTESIAN_POINT('Ctrl Pts',(0.456374956919836,19.4196381763074,-334.486766185145)) ;
#31529=CARTESIAN_POINT('Ctrl Pts',(0.052393246489807,19.4291320265028,-334.481800776353)) ;
#31530=CARTESIAN_POINT('Ctrl Pts',(-0.351884728504625,19.4260156153053,
-334.47683536756)) ;
#31531=CARTESIAN_POINT('Ctrl Pts',(-0.755658741192586,19.4102963621594,
-334.471869958768)) ;
#31532=CARTESIAN_POINT('Ctrl Pts',(-1.15884366319998,19.3946000427964,-334.466911794314)) ;
#31533=CARTESIAN_POINT('Ctrl Pts',(-1.5615258552778,19.3663376529126,-334.461953629861)) ;
#31534=CARTESIAN_POINT('Ctrl Pts',(-1.96291092729285,19.325568702926,-334.456995465408)) ;
#31535=CARTESIAN_POINT('Ctrl Pts',(-2.36517569070632,19.2847104020963,-334.452026434446)) ;
#31536=CARTESIAN_POINT('Ctrl Pts',(-2.76613740260173,19.2312906708978,-334.447057403483)) ;
#31537=CARTESIAN_POINT('Ctrl Pts',(-3.16500237188338,19.1654215968753,-334.442088372521)) ;
#31538=CARTESIAN_POINT('Ctrl Pts',(-3.56386734116495,19.0995525228527,-334.437119341558)) ;
#31539=CARTESIAN_POINT('Ctrl Pts',(-3.96063533243817,19.0212341516236,-334.432150310596)) ;
#31540=CARTESIAN_POINT('Ctrl Pts',(-4.35452214552194,18.930630255862,-334.427181279634)) ;
#31541=CARTESIAN_POINT('Ctrl Pts',(-4.74787130211817,18.8401500346454,-334.422219031411)) ;
#31542=CARTESIAN_POINT('Ctrl Pts',(-5.13845170566674,18.7373937652141,-334.417256783188)) ;
#31543=CARTESIAN_POINT('Ctrl Pts',(-5.52548958343109,18.6225559433552,-334.412294534965)) ;
#31544=CARTESIAN_POINT('Ctrl Pts',(-5.9122342795839,18.5078051112707,-334.407336045651)) ;
#31545=CARTESIAN_POINT('Ctrl Pts',(-6.29544158712495,18.3809910909594,-334.402377556337)) ;
#31546=CARTESIAN_POINT('Ctrl Pts',(-6.67435341722363,18.2423581661471,-334.397419067022)) ;
#31547=CARTESIAN_POINT('Ctrl Pts',(-7.05322458416268,18.1037401188138,-334.392461109831)) ;
#31548=CARTESIAN_POINT('Ctrl Pts',(-7.42780097154076,17.9533057818234,-334.38750315264)) ;
#31549=CARTESIAN_POINT('Ctrl Pts',(-7.79734205372781,17.7913485126105,-334.382545195449)) ;
#31550=CARTESIAN_POINT('Ctrl Pts',(-8.16686067795821,17.6294010859551,-334.377587539566)) ;
#31551=CARTESIAN_POINT('Ctrl Pts',(-8.53134439099051,17.4559322213099,-334.372629883683)) ;
#31552=CARTESIAN_POINT('Ctrl Pts',(-8.89007343634173,17.2712830819384,-334.3676722278)) ;
#31553=CARTESIAN_POINT('Ctrl Pts',(-9.24936347137597,17.0863451835062,-334.362706819007)) ;
#31554=CARTESIAN_POINT('Ctrl Pts',(-9.60288060766997,16.8901921120831,-334.357741410214)) ;
#31555=CARTESIAN_POINT('Ctrl Pts',(-9.94992569266374,16.6832132309837,-334.352776001422)) ;
#31556=CARTESIAN_POINT('Ctrl Pts',(-10.2964644522903,16.476536324073,-334.347817836968)) ;
#31557=CARTESIAN_POINT('Ctrl Pts',(-10.6365498351517,16.2590653079337,-334.342859672515)) ;
#31558=CARTESIAN_POINT('Ctrl Pts',(-10.9695127356894,16.0312324960231,-334.337901508062)) ;
#31559=CARTESIAN_POINT('Ctrl Pts',(-11.3032053708883,15.8029003567114,-334.3329324771)) ;
#31560=CARTESIAN_POINT('Ctrl Pts',(-11.6297440639063,15.5641610762247,-334.327963446137)) ;
#31561=CARTESIAN_POINT('Ctrl Pts',(-11.948485477212,15.3154928030688,-334.322994415175)) ;
#31562=CARTESIAN_POINT('Ctrl Pts',(-12.2672268905179,15.0668245299129,-334.318025384212)) ;
#31563=CARTESIAN_POINT('Ctrl Pts',(-12.5781708392292,14.8082274167643,-334.31305635325)) ;
#31564=CARTESIAN_POINT('Ctrl Pts',(-12.8807070474881,14.5402204576406,-334.308087322288)) ;
#31565=CARTESIAN_POINT('Ctrl Pts',(-13.182830293066,14.2725793286865,-334.303125074065)) ;
#31566=CARTESIAN_POINT('Ctrl Pts',(-13.47664905564,13.9954828882491,-334.298162825842)) ;
#31567=CARTESIAN_POINT('Ctrl Pts',(-13.7615769146786,13.7094721204496,-334.293200577619)) ;
#31568=CARTESIAN_POINT('Ctrl Pts',(-14.0462889405564,13.4236780061156,-334.288242088305)) ;
#31569=CARTESIAN_POINT('Ctrl Pts',(-14.3221233598798,13.1289832328028,-334.283283598991)) ;
#31570=CARTESIAN_POINT('Ctrl Pts',(-14.5885313443723,12.8259650012881,-334.278325109676)) ;
#31571=CARTESIAN_POINT('Ctrl Pts',(-14.854910739124,12.5229792883659,-334.273367152485)) ;
#31572=CARTESIAN_POINT('Ctrl Pts',(-15.1118655628799,12.2116720795278,-334.268409195295)) ;
#31573=CARTESIAN_POINT('Ctrl Pts',(-15.3588858881755,11.8926552659196,-334.263451238104)) ;
#31574=CARTESIAN_POINT('Ctrl Pts',(-15.6058912014136,11.5736578397797,-334.25849358222)) ;
#31575=CARTESIAN_POINT('Ctrl Pts',(-15.8429630770454,11.2469519325026,-334.253535926337)) ;
#31576=CARTESIAN_POINT('Ctrl Pts',(-16.0696326970679,10.9131814784382,-334.248578270454)) ;
#31577=CARTESIAN_POINT('Ctrl Pts',(-16.2966567888581,10.5788890655738,-334.243612861662)) ;
#31578=CARTESIAN_POINT('Ctrl Pts',(-16.5132459196395,10.2375101829376,-334.238647452869)) ;
#31579=CARTESIAN_POINT('Ctrl Pts',(-16.7189724243879,9.88972123330872,-334.233682044076)) ;
#31580=CARTESIAN_POINT('Ctrl Pts',(-16.924398782118,9.54243969431409,-334.228723879623)) ;
#31581=CARTESIAN_POINT('Ctrl Pts',(-17.1189940787293,9.18876699104686,-334.22376571517)) ;
#31582=CARTESIAN_POINT('Ctrl Pts',(-17.3023775827306,8.82940286682075,-334.218807550717)) ;
#31583=CARTESIAN_POINT('Ctrl Pts',(-17.4861629972697,8.46925114597181,-334.213838519754)) ;
#31584=CARTESIAN_POINT('Ctrl Pts',(-17.6586872990454,8.10338323622678,-334.208869488792)) ;
#31585=CARTESIAN_POINT('Ctrl Pts',(-17.8196143128186,7.73252680191873,-334.20390045783)) ;
#31586=CARTESIAN_POINT('Ctrl Pts',(-17.9805413265917,7.36167036761077,-334.198931426867)) ;
#31587=CARTESIAN_POINT('Ctrl Pts',(-18.1298709630558,6.98582563126151,-334.193962395905)) ;
#31588=CARTESIAN_POINT('Ctrl Pts',(-18.2673156208678,6.60574030730857,-334.188993364943)) ;
#31589=CARTESIAN_POINT('Ctrl Pts',(-18.4045726663784,6.22617380077244,-334.18403111672)) ;
#31590=CARTESIAN_POINT('Ctrl Pts',(-18.5300136547585,5.84227738117756,-334.179068868497)) ;
#31591=CARTESIAN_POINT('Ctrl Pts',(-18.6433824533151,5.45480666013219,-334.174106620274)) ;
#31592=CARTESIAN_POINT('Ctrl Pts',(-18.7566653748843,5.06762944857674,-334.16914813096)) ;
#31593=CARTESIAN_POINT('Ctrl Pts',(-18.8578943223797,4.67688357657028,-334.164189641646)) ;
#31594=CARTESIAN_POINT('Ctrl Pts',(-18.9468635008799,4.28333847355357,-334.159231152331)) ;
#31595=CARTESIAN_POINT('Ctrl Pts',(-19.0358231315961,3.88983560408043,-334.15427319514)) ;
#31596=CARTESIAN_POINT('Ctrl Pts',(-19.1125255688101,3.49353433503265,-334.149315237949)) ;
#31597=CARTESIAN_POINT('Ctrl Pts',(-19.1768157742415,3.09521594736152,-334.144357280758)) ;
#31598=CARTESIAN_POINT('Ctrl Pts',(-19.2411020725932,2.69692176651476,-334.139399624875)) ;
#31599=CARTESIAN_POINT('Ctrl Pts',(-19.2929776083019,2.29661094620041,-334.134441968992)) ;
#31600=CARTESIAN_POINT('Ctrl Pts',(-19.3323387727382,1.89507323765717,-334.129484313109)) ;
#31601=CARTESIAN_POINT('Ctrl Pts',(-19.3717614911733,1.49290759414245,-334.124518904316)) ;
#31602=CARTESIAN_POINT('Ctrl Pts',(-19.3986306302936,1.08951145825837,-334.119553495523)) ;
#31603=CARTESIAN_POINT('Ctrl Pts',(-19.4128942527724,0.685683404113655,
-334.114588086731)) ;
#31604=CARTESIAN_POINT('Ctrl Pts',(-19.4271370651773,0.282444519490505,
-334.109629922277)) ;
#31605=CARTESIAN_POINT('Ctrl Pts',(-19.4288111225219,-0.121224785798165,
-334.104671757824)) ;
#31606=CARTESIAN_POINT('Ctrl Pts',(-19.4179168678447,-0.524527895798856,
-334.099713593371)) ;
#31607=CARTESIAN_POINT('Ctrl Pts',(-19.4069987368883,-0.928714900840813,
-334.094744562408)) ;
#31608=CARTESIAN_POINT('Ctrl Pts',(-19.3834571348805,-1.33253386406551,
-334.089775531446)) ;
#31609=CARTESIAN_POINT('Ctrl Pts',(-19.3473449890827,-1.73518496807009,
-334.084806500484)) ;
#31610=CARTESIAN_POINT('Ctrl Pts',(-19.3112328432849,-2.13783607207458,
-334.079837469521)) ;
#31611=CARTESIAN_POINT('Ctrl Pts',(-19.2625501817346,-2.53931907872982,
-334.074868438559)) ;
#31612=CARTESIAN_POINT('Ctrl Pts',(-19.2014021782866,-2.93883980299876,
-334.069899407596)) ;
#31613=CARTESIAN_POINT('Ctrl Pts',(-19.1403376420162,-3.33781518048016,
-334.064937159373)) ;
#31614=CARTESIAN_POINT('Ctrl Pts',(-19.066825550336,-3.73493968856343,-334.059974911151)) ;
#31615=CARTESIAN_POINT('Ctrl Pts',(-18.9810024888263,-4.12942726285024,
-334.055012662928)) ;
#31616=CARTESIAN_POINT('Ctrl Pts',(-18.8952444383777,-4.5236160123761,-334.050054173613)) ;
#31617=CARTESIAN_POINT('Ctrl Pts',(-18.7971941126643,-4.91517158944148,
-334.045095684299)) ;
#31618=CARTESIAN_POINT('Ctrl Pts',(-18.6870389110983,-5.30331987863233,
-334.040137194985)) ;
#31619=CARTESIAN_POINT('Ctrl Pts',(-18.5768955309073,-5.69142651344479,
-334.035179237794)) ;
#31620=CARTESIAN_POINT('Ctrl Pts',(-18.4546499342569,-6.07612636245392,
-334.030221280603)) ;
#31621=CARTESIAN_POINT('Ctrl Pts',(-18.3205397614761,-6.456659186311,-334.025263323412)) ;
#31622=CARTESIAN_POINT('Ctrl Pts',(-18.1864377389124,-6.83716888421797,
-334.020305667528)) ;
#31623=CARTESIAN_POINT('Ctrl Pts',(-18.0404726595519,-7.21351183908467,
-334.015348011645)) ;
#31624=CARTESIAN_POINT('Ctrl Pts',(-17.8829313779694,-7.58494497876132,
-334.010390355762)) ;
#31625=CARTESIAN_POINT('Ctrl Pts',(-17.7251437292923,-7.9569589751034,-334.005424946969)) ;
#31626=CARTESIAN_POINT('Ctrl Pts',(-17.5557437243768,-8.32404756306942,
-334.000459538177)) ;
#31627=CARTESIAN_POINT('Ctrl Pts',(-17.37506781293,-8.68548464370782,-333.995494129384)) ;
#31628=CARTESIAN_POINT('Ctrl Pts',(-17.1946555006545,-9.04639440161577,
-333.990535964931)) ;
#31629=CARTESIAN_POINT('Ctrl Pts',(-17.0030002797343,-9.40166892475343,
-333.985577800478)) ;
#31630=CARTESIAN_POINT('Ctrl Pts',(-16.8004836597507,-9.75060889372814,
-333.980619636025)) ;
#31631=CARTESIAN_POINT('Ctrl Pts',(-16.5975231963353,-10.1003136133358,
-333.975650605062)) ;
#31632=CARTESIAN_POINT('Ctrl Pts',(-16.3836537805527,-10.4436557678626,
-333.9706815741)) ;
#31633=CARTESIAN_POINT('Ctrl Pts',(-16.1593045415395,-10.7799583363657,
-333.965712543137)) ;
#31634=CARTESIAN_POINT('Ctrl Pts',(-15.9349553025264,-11.1162609048688,
-333.960743512175)) ;
#31635=CARTESIAN_POINT('Ctrl Pts',(-15.7001263788299,-11.4455236916539,
-333.955774481213)) ;
#31636=CARTESIAN_POINT('Ctrl Pts',(-15.4552900841601,-11.7670996177675,
-333.95080545025)) ;
#31637=CARTESIAN_POINT('Ctrl Pts',(-15.2107879916426,-12.0882365919404,
-333.945843202028)) ;
#31638=CARTESIAN_POINT('Ctrl Pts',(-14.9562408442818,-12.4017930498775,
-333.940880953805)) ;
#31639=CARTESIAN_POINT('Ctrl Pts',(-14.6921446542139,-12.7071440717281,
-333.935918705582)) ;
#31640=CARTESIAN_POINT('Ctrl Pts',(-14.4282485172965,-13.0122637898483,
-333.930960216268)) ;
#31641=CARTESIAN_POINT('Ctrl Pts',(-14.1548179543914,-13.309190318756,-333.926001726953)) ;
#31642=CARTESIAN_POINT('Ctrl Pts',(-13.8723878820347,-13.5973335419257,
-333.921043237639)) ;
#31643=CARTESIAN_POINT('Ctrl Pts',(-13.5899881188345,-13.8854458428286,
-333.916085280448)) ;
#31644=CARTESIAN_POINT('Ctrl Pts',(-13.2985909412687,-14.164776551195,-333.911127323257)) ;
#31645=CARTESIAN_POINT('Ctrl Pts',(-12.9987687452168,-14.4347717719532,
-333.906169366066)) ;
#31646=CARTESIAN_POINT('Ctrl Pts',(-12.6989647701228,-14.7047505844146,
-333.901211710183)) ;
#31647=CARTESIAN_POINT('Ctrl Pts',(-12.3907369757437,-14.9653948838844,
-333.8962540543)) ;
#31648=CARTESIAN_POINT('Ctrl Pts',(-12.0746927611949,-15.2161893955993,
-333.891296398416)) ;
#31649=CARTESIAN_POINT('Ctrl Pts',(-11.7581543086052,-15.4673761061978,
-333.886330989624)) ;
#31650=CARTESIAN_POINT('Ctrl Pts',(-11.4337751481267,-15.708682039252,-333.881365580831)) ;
#31651=CARTESIAN_POINT('Ctrl Pts',(-11.1021981093919,-15.9396305521745,
-333.876400172039)) ;
#31652=CARTESIAN_POINT('Ctrl Pts',(-10.7711048287413,-16.1702421201428,
-333.871442007586)) ;
#31653=CARTESIAN_POINT('Ctrl Pts',(-10.4328348610376,-16.3905263443745,
-333.866483843132)) ;
#31654=CARTESIAN_POINT('Ctrl Pts',(-10.0880577922883,-16.6000516559272,
-333.861525678679)) ;
#31655=CARTESIAN_POINT('Ctrl Pts',(-9.74252509648156,-16.810036171438,-333.856556647717)) ;
#31656=CARTESIAN_POINT('Ctrl Pts',(-9.39045694281454,-17.0092144264153,
-333.851587616755)) ;
#31657=CARTESIAN_POINT('Ctrl Pts',(-9.03255406527089,-17.1971972151848,
-333.846618585792)) ;
#31658=CARTESIAN_POINT('Ctrl Pts',(-8.67465118772716,-17.3851800039543,
-333.84164955483)) ;
#31659=CARTESIAN_POINT('Ctrl Pts',(-8.31091380159397,-17.5619672209556,
-333.836680523868)) ;
#31660=CARTESIAN_POINT('Ctrl Pts',(-7.94206623749012,-17.7272166139899,
-333.831711492905)) ;
#31661=CARTESIAN_POINT('Ctrl Pts',(-7.57542016948373,-17.8914797028453,
-333.82677212)) ;
#31662=CARTESIAN_POINT('Ctrl Pts',(-7.20362005613073,-18.0443891674317,
-333.821832747096)) ;
#31663=CARTESIAN_POINT('Ctrl Pts',(-6.82739290416258,-18.1856352963593,
-333.816893374191)) ;
#31664=CARTESIAN_POINT('Ctrl Pts',(-6.45122839700186,-18.3268579066852,
-333.811954823731)) ;
#31665=CARTESIAN_POINT('Ctrl Pts',(-6.07063854896628,-18.4564209748887,
-333.807016273271)) ;
#31666=CARTESIAN_POINT('Ctrl Pts',(-5.68636928654813,-18.5740633501935,
-333.802077722811)) ;
#31667=CARTESIAN_POINT('Ctrl Pts',(-5.30214293324897,-18.6916925890569,
-333.79713972381)) ;
#31668=CARTESIAN_POINT('Ctrl Pts',(-4.91423821668825,-18.7974037230299,
-333.792201724809)) ;
#31669=CARTESIAN_POINT('Ctrl Pts',(-4.52341669546291,-18.8909853210257,
-333.787263725808)) ;
#31670=CARTESIAN_POINT('Ctrl Pts',(-4.13258414277082,-18.9845695604888,
-333.782325587426)) ;
#31671=CARTESIAN_POINT('Ctrl Pts',(-3.73883485478379,-19.0660235209341,
-333.777387449043)) ;
#31672=CARTESIAN_POINT('Ctrl Pts',(-3.342942861601,-19.1351863859245,-333.772449310661)) ;
#31673=CARTESIAN_POINT('Ctrl Pts',(-2.94705968997046,-19.2043477097778,
-333.767511282313)) ;
#31674=CARTESIAN_POINT('Ctrl Pts',(-2.54903414638424,-19.2612184453507,
-333.762573253966)) ;
#31675=CARTESIAN_POINT('Ctrl Pts',(-2.14964907568037,-19.3056891576402,
-333.757635225619)) ;
#31676=CARTESIAN_POINT('Ctrl Pts',(-1.75019814895231,-19.3501672028635,
-333.752696383022)) ;
#31677=CARTESIAN_POINT('Ctrl Pts',(-1.34938748670992,-19.3822411103973,
-333.747757540426)) ;
#31678=CARTESIAN_POINT('Ctrl Pts',(-0.948005606204455,-19.4018532715461,
-333.742818697829)) ;
#31679=CARTESIAN_POINT('Ctrl Pts',(-0.632084577866105,-19.4172896786661,
-333.738931416645)) ;
#31680=CARTESIAN_POINT('Ctrl Pts',(-0.315809823623688,-19.4250070501413,
-333.73504413546)) ;
#31681=CARTESIAN_POINT('Ctrl Pts',(0.000433346557224641,-19.4249999951663,
-333.731156854276)) ;
#31682=CARTESIAN_POINT('Ctrl Pts',(0.00049296941716015,-19.4249999937447,
-333.518704187163)) ;
#31683=CARTESIAN_POINT('Ctrl Pts',(-0.634377794024984,-19.4250161055527,
-333.526895207536)) ;
#31684=CARTESIAN_POINT('Ctrl Pts',(-1.26886984962391,-19.3939078124572,
-333.535071304866)) ;
#31685=CARTESIAN_POINT('Ctrl Pts',(-2.08814708294686,-19.3133566103983,
-333.545427955287)) ;
#31686=CARTESIAN_POINT('Ctrl Pts',(-2.27531831103279,-19.2922012363027,
-333.54778157939)) ;
#31687=CARTESIAN_POINT('Ctrl Pts',(-2.5880520073918,-19.2522393847525,-333.551692190441)) ;
#31688=CARTESIAN_POINT('Ctrl Pts',(-2.71379097667053,-19.2349180685968,
-333.553258578115)) ;
#31689=CARTESIAN_POINT('Ctrl Pts',(-2.96955422421659,-19.1971272757905,
-333.556433013483)) ;
#31690=CARTESIAN_POINT('Ctrl Pts',(-3.09955840904494,-19.1765660548772,
-333.558040375671)) ;
#31691=CARTESIAN_POINT('Ctrl Pts',(-3.43440878247859,-19.120112663677,-333.562165822838)) ;
#31692=CARTESIAN_POINT('Ctrl Pts',(-3.63890566184248,-19.0822492840032,
-333.56467100356)) ;
#31693=CARTESIAN_POINT('Ctrl Pts',(-3.97755774036059,-19.0139046811789,
-333.56880235924)) ;
#31694=CARTESIAN_POINT('Ctrl Pts',(-4.11206753742703,-18.9852689582846,
-333.570438778873)) ;
#31695=CARTESIAN_POINT('Ctrl Pts',(-4.8889902194043,-18.8112261640848,-333.579873963237)) ;
#31696=CARTESIAN_POINT('Ctrl Pts',(-5.52397797503081,-18.6346484022811,
-333.587502859057)) ;
#31697=CARTESIAN_POINT('Ctrl Pts',(-6.45655009296665,-18.3234512419332,
-333.599039042833)) ;
#31698=CARTESIAN_POINT('Ctrl Pts',(-6.76171162596236,-18.2130491550333,
-333.602872010311)) ;
#31699=CARTESIAN_POINT('Ctrl Pts',(-7.15629336903421,-18.0590119933025,
-333.607974761023)) ;
#31700=CARTESIAN_POINT('Ctrl Pts',(-7.24834591687685,-18.0222620774717,
-333.609175844674)) ;
#31701=CARTESIAN_POINT('Ctrl Pts',(-7.40173864602791,-17.9596581345363,
-333.611198027685)) ;
#31702=CARTESIAN_POINT('Ctrl Pts',(-7.46323449639608,-17.9341904237043,
-333.612014402899)) ;
#31703=CARTESIAN_POINT('Ctrl Pts',(-7.59730253902076,-17.8778588825336,
-333.613807380551)) ;
#31704=CARTESIAN_POINT('Ctrl Pts',(-7.6698199724682,-17.84686823121,-333.614785485383)) ;
#31705=CARTESIAN_POINT('Ctrl Pts',(-7.89483493865592,-17.7490823127808,
-333.617843951232)) ;
#31706=CARTESIAN_POINT('Ctrl Pts',(-8.04666373334751,-17.6807676379174,
-333.619941350387)) ;
#31707=CARTESIAN_POINT('Ctrl Pts',(-8.31789712404011,-17.5545099886051,
-333.623737369494)) ;
#31708=CARTESIAN_POINT('Ctrl Pts',(-8.43762187156459,-17.4972789486582,
-333.625430452278)) ;
#31709=CARTESIAN_POINT('Ctrl Pts',(-9.07908498771921,-17.1825306939237,
-333.634580265556)) ;
#31710=CARTESIAN_POINT('Ctrl Pts',(-9.58964074187833,-16.9028973008236,
-333.64213509543)) ;
#31711=CARTESIAN_POINT('Ctrl Pts',(-10.4242964122772,-16.3957481446031,
-333.654655823424)) ;
#31712=CARTESIAN_POINT('Ctrl Pts',(-10.7553897361116,-16.1804853398693,
-333.659672961205)) ;
#31713=CARTESIAN_POINT('Ctrl Pts',(-11.21043332849,-15.8644932222774,-333.666609681646)) ;
#31714=CARTESIAN_POINT('Ctrl Pts',(-11.3400527938041,-15.7721007904114,
-333.668590815108)) ;
#31715=CARTESIAN_POINT('Ctrl Pts',(-11.5690204990481,-15.6046113045006,
-333.672099507132)) ;
#31716=CARTESIAN_POINT('Ctrl Pts',(-11.6688097120516,-15.5301322989524,
-333.673631839425)) ;
#31717=CARTESIAN_POINT('Ctrl Pts',(-11.880790810823,-15.3687207248924,-333.676894311884)) ;
#31718=CARTESIAN_POINT('Ctrl Pts',(-11.9927600583853,-15.2815075584804,
-333.678622052446)) ;
#31719=CARTESIAN_POINT('Ctrl Pts',(-12.3122233639389,-15.027002904733,-333.683566892419)) ;
#31720=CARTESIAN_POINT('Ctrl Pts',(-12.5172433336689,-14.8566577724609,
-333.686758958099)) ;
#31721=CARTESIAN_POINT('Ctrl Pts',(-13.3784181426972,-14.1106485051642,
-333.700290106059)) ;
#31722=CARTESIAN_POINT('Ctrl Pts',(-13.9988696326359,-13.495336643232,-333.710306358222)) ;
#31723=CARTESIAN_POINT('Ctrl Pts',(-14.6873365459008,-12.7138201991444,
-333.722668430197)) ;
#31724=CARTESIAN_POINT('Ctrl Pts',(-14.797186343034,-12.5857997381955,-333.724684708977)) ;
#31725=CARTESIAN_POINT('Ctrl Pts',(-14.9567467823962,-12.3948688424859,
-333.727690860287)) ;
#31726=CARTESIAN_POINT('Ctrl Pts',(-15.0077578550807,-12.3330552612761,
-333.728663964886)) ;
#31727=CARTESIAN_POINT('Ctrl Pts',(-15.1001491280674,-12.2196764387105,
-333.730450272513)) ;
#31728=CARTESIAN_POINT('Ctrl Pts',(-15.1416513777497,-12.1682122563362,
-333.731261710531)) ;
#31729=CARTESIAN_POINT('Ctrl Pts',(-15.2334276378244,-12.0532100187903,
-333.733076894494)) ;
#31730=CARTESIAN_POINT('Ctrl Pts',(-15.2835683696731,-11.9895674326024,
-333.734082503568)) ;
#31731=CARTESIAN_POINT('Ctrl Pts',(-15.443606743269,-11.7837987324861,-333.737334675666)) ;
#31732=CARTESIAN_POINT('Ctrl Pts',(-15.5519312085663,-11.6404612154855,
-333.739601342375)) ;
#31733=CARTESIAN_POINT('Ctrl Pts',(-15.8248690241512,-11.2686917240223,
-333.745462468966)) ;
#31734=CARTESIAN_POINT('Ctrl Pts',(-15.9865325735823,-11.0381460746716,
-333.749079907081)) ;
#31735=CARTESIAN_POINT('Ctrl Pts',(-16.5745066961902,-10.1596202300234,
-333.76270219977)) ;
#31736=CARTESIAN_POINT('Ctrl Pts',(-16.9668986651267,-9.48981112800607,
-333.772735206145)) ;
#31737=CARTESIAN_POINT('Ctrl Pts',(-17.389210438649,-8.65855465042104,-333.784437923188)) ;
#31738=CARTESIAN_POINT('Ctrl Pts',(-17.4585320656547,-8.51791444651106,
-333.786394586159)) ;
#31739=CARTESIAN_POINT('Ctrl Pts',(-17.5808205479466,-8.26204884621995,
-333.789911880438)) ;
#31740=CARTESIAN_POINT('Ctrl Pts',(-17.6343762150223,-8.14711469375784,
-333.791476594318)) ;
#31741=CARTESIAN_POINT('Ctrl Pts',(-17.7412973315182,-7.91166004604576,
-333.794651497065)) ;
#31742=CARTESIAN_POINT('Ctrl Pts',(-17.7945691683645,-7.79110414875335,
-333.796260960422)) ;
#31743=CARTESIAN_POINT('Ctrl Pts',(-17.9291227409596,-7.47802457544677,
-333.800400587902)) ;
#31744=CARTESIAN_POINT('Ctrl Pts',(-18.0085320546082,-7.28471463050536,
-333.802917665049)) ;
#31745=CARTESIAN_POINT('Ctrl Pts',(-18.1353558997643,-6.96122623787912,
-333.807072133883)) ;
#31746=CARTESIAN_POINT('Ctrl Pts',(-18.1845245625784,-6.83175459364493,
-333.808719814951)) ;
#31747=CARTESIAN_POINT('Ctrl Pts',(-18.3821408107369,-6.29413533803565,
-333.815506504031)) ;
#31748=CARTESIAN_POINT('Ctrl Pts',(-18.5182644386963,-5.88159188289777,
-333.820580729743)) ;
#31749=CARTESIAN_POINT('Ctrl Pts',(-18.6796300960854,-5.331176608105,-333.827279740326)) ;
#31750=CARTESIAN_POINT('Ctrl Pts',(-18.7173756970051,-5.19710222717293,
-333.828906361971)) ;
#31751=CARTESIAN_POINT('Ctrl Pts',(-18.7726314959133,-4.99241639642702,
-333.831386999337)) ;
#31752=CARTESIAN_POINT('Ctrl Pts',(-18.7911924004187,-4.92209334769814,
-333.832238793075)) ;
#31753=CARTESIAN_POINT('Ctrl Pts',(-18.8927928610358,-4.52820004483407,
-333.837010193975)) ;
#31754=CARTESIAN_POINT('Ctrl Pts',(-18.9678696745375,-4.20263450562384,
-333.840954228702)) ;
#31755=CARTESIAN_POINT('Ctrl Pts',(-19.0542615433035,-3.77829863155859,
-333.846171093305)) ;
#31756=CARTESIAN_POINT('Ctrl Pts',(-19.0732678405119,-3.68115163446636,
-333.847370654727)) ;
#31757=CARTESIAN_POINT('Ctrl Pts',(-19.1038078518183,-3.51846253403099,
-333.849391106166)) ;
#31758=CARTESIAN_POINT('Ctrl Pts',(-19.1157488118805,-3.45299875643084,
-333.850207291852)) ;
#31759=CARTESIAN_POINT('Ctrl Pts',(-19.1411172677412,-3.30975594454825,
-333.8520009225)) ;
#31760=CARTESIAN_POINT('Ctrl Pts',(-19.1544075363511,-3.23195398795656,
-333.85297988125)) ;
#31761=CARTESIAN_POINT('Ctrl Pts',(-19.1943198331489,-2.98940797272952,
-333.85604420457)) ;
#31762=CARTESIAN_POINT('Ctrl Pts',(-19.2192933105096,-2.82440053416878,
-333.85814669636)) ;
#31763=CARTESIAN_POINT('Ctrl Pts',(-19.2603674821564,-2.52717319999682,
-333.861953973039)) ;
#31764=CARTESIAN_POINT('Ctrl Pts',(-19.2772404053223,-2.39507040272328,
-333.863653225687)) ;
#31765=CARTESIAN_POINT('Ctrl Pts',(-19.3610532645679,-1.68047897078858,
-333.872867192125)) ;
#31766=CARTESIAN_POINT('Ctrl Pts',(-19.4029529317605,-1.09535937448209,
-333.880480907722)) ;
#31767=CARTESIAN_POINT('Ctrl Pts',(-19.4224441328253,-0.352124682352392,
-333.890010289483)) ;
#31768=CARTESIAN_POINT('Ctrl Pts',(-19.424657459709,-0.194962874678155,
-333.892018032003)) ;
#31769=CARTESIAN_POINT('Ctrl Pts',(-19.4255111694189,0.243847458051502,
-333.897598177308)) ;
#31770=CARTESIAN_POINT('Ctrl Pts',(-19.4199338945183,0.525465325456291,
-333.901149453673)) ;
#31771=CARTESIAN_POINT('Ctrl Pts',(-19.4022376525988,0.951129909222373,
-333.90646402678)) ;
#31772=CARTESIAN_POINT('Ctrl Pts',(-19.3946316050709,1.09532598287024,-333.908255236887)) ;
#31773=CARTESIAN_POINT('Ctrl Pts',(-19.3774938025193,1.36337266285042,-333.911568008291)) ;
#31774=CARTESIAN_POINT('Ctrl Pts',(-19.3683804326872,1.4872425981483,-333.913092183635)) ;
#31775=CARTESIAN_POINT('Ctrl Pts',(-19.344969578548,1.7685489203768,-333.916539000137)) ;
#31776=CARTESIAN_POINT('Ctrl Pts',(-19.3299369724226,1.9259153700103,-333.918456787977)) ;
#31777=CARTESIAN_POINT('Ctrl Pts',(-19.2718928924541,2.46406271261185,-333.924983894577)) ;
#31778=CARTESIAN_POINT('Ctrl Pts',(-19.219536221626,2.84374560318721,-333.929533760456)) ;
#31779=CARTESIAN_POINT('Ctrl Pts',(-19.02760865851,3.98495661289765,-333.943151099483)) ;
#31780=CARTESIAN_POINT('Ctrl Pts',(-18.8537237035872,4.73992233222652,-333.952057623934)) ;
#31781=CARTESIAN_POINT('Ctrl Pts',(-18.595520069256,5.61756917537427,-333.962985451683)) ;
#31782=CARTESIAN_POINT('Ctrl Pts',(-18.5543129387541,5.7522101282501,-333.964679219269)) ;
#31783=CARTESIAN_POINT('Ctrl Pts',(-18.4891439782415,5.9571548415608,-333.96729126482)) ;
#31784=CARTESIAN_POINT('Ctrl Pts',(-18.4662366996387,6.02778906313,-333.968197700335)) ;
#31785=CARTESIAN_POINT('Ctrl Pts',(-18.4214640392247,6.16319403724513,-333.969948670654)) ;
#31786=CARTESIAN_POINT('Ctrl Pts',(-18.3996606681789,6.22798405172113,-333.970792500178)) ;
#31787=CARTESIAN_POINT('Ctrl Pts',(-18.3417566032372,6.39709112056289,-333.973009519479)) ;
#31788=CARTESIAN_POINT('Ctrl Pts',(-18.3051079115303,6.50121791613505,-333.974389132721)) ;
#31789=CARTESIAN_POINT('Ctrl Pts',(-18.0976765588818,7.07491243554616,-333.982059551711)) ;
#31790=CARTESIAN_POINT('Ctrl Pts',(-17.9097129459894,7.53806764257432,-333.988504886171)) ;
#31791=CARTESIAN_POINT('Ctrl Pts',(-17.441099631996,8.57596357037019,-334.003197205166)) ;
#31792=CARTESIAN_POINT('Ctrl Pts',(-17.1495075145107,9.14513557604694,-334.011429167314)) ;
#31793=CARTESIAN_POINT('Ctrl Pts',(-16.7365603605633,9.86171826123412,-334.021833258483)) ;
#31794=CARTESIAN_POINT('Ctrl Pts',(-16.6403729353542,10.0231695833263,-334.024181372581)) ;
#31795=CARTESIAN_POINT('Ctrl Pts',(-16.4753577366656,10.2912246138698,-334.028085613267)) ;
#31796=CARTESIAN_POINT('Ctrl Pts',(-16.4078009288665,10.3985953538322,-334.02965107128)) ;
#31797=CARTESIAN_POINT('Ctrl Pts',(-16.2679630988419,10.6160892467489,-334.032825758557)) ;
#31798=CARTESIAN_POINT('Ctrl Pts',(-16.1956038888716,10.7261544371592,-334.034434280181)) ;
#31799=CARTESIAN_POINT('Ctrl Pts',(-16.0058174326016,11.0085381814168,-334.03856755477)) ;
#31800=CARTESIAN_POINT('Ctrl Pts',(-15.886724897396,11.1797172061345,-334.041079302723)) ;
#31801=CARTESIAN_POINT('Ctrl Pts',(-15.6136749186512,11.5590128266572,-334.046667662037)) ;
#31802=CARTESIAN_POINT('Ctrl Pts',(-15.4582666947986,11.7660364210973,-334.049733608004)) ;
#31803=CARTESIAN_POINT('Ctrl Pts',(-14.8267557090714,12.573173142812,-334.061798558308)) ;
#31804=CARTESIAN_POINT('Ctrl Pts',(-14.3194752461305,13.1480031934642,-334.070615137339)) ;
#31805=CARTESIAN_POINT('Ctrl Pts',(-13.6723612371942,13.7992863954528,-334.081562388432)) ;
#31806=CARTESIAN_POINT('Ctrl Pts',(-13.5638751844945,13.9059360232863,-334.083389500396)) ;
#31807=CARTESIAN_POINT('Ctrl Pts',(-13.3990762927668,14.0641817690922,-334.086161963129)) ;
#31808=CARTESIAN_POINT('Ctrl Pts',(-13.3436935429148,14.1167381836986,-334.087093183689)) ;
#31809=CARTESIAN_POINT('Ctrl Pts',(-13.2388643695025,14.2150495386456,-334.088856388651)) ;
#31810=CARTESIAN_POINT('Ctrl Pts',(-13.1894870589464,14.2608763497804,-334.089687277657)) ;
#31811=CARTESIAN_POINT('Ctrl Pts',(-13.0628509588499,14.3771863180403,-334.091818229695)) ;
#31812=CARTESIAN_POINT('Ctrl Pts',(-12.9852595440676,14.4473041127236,-334.093123805156)) ;
#31813=CARTESIAN_POINT('Ctrl Pts',(-12.8559948557357,14.5622353610732,-334.095295896157)) ;
#31814=CARTESIAN_POINT('Ctrl Pts',(-12.8046443065917,14.6074086207401,-334.096158005758)) ;
#31815=CARTESIAN_POINT('Ctrl Pts',(-12.6028574243775,14.783039597545,-334.099541042289)) ;
#31816=CARTESIAN_POINT('Ctrl Pts',(-12.450657432261,14.9114521202667,-334.10208246997)) ;
#31817=CARTESIAN_POINT('Ctrl Pts',(-11.7312234350435,15.4997498138426,-334.114001191108)) ;
#31818=CARTESIAN_POINT('Ctrl Pts',(-11.1403181042868,15.9297572552004,-334.123498200318)) ;
#31819=CARTESIAN_POINT('Ctrl Pts',(-10.2979503832235,16.4729131206968,-334.136232765216)) ;
#31820=CARTESIAN_POINT('Ctrl Pts',(-10.0662176184587,16.6155322541338,-334.139660829656)) ;
#31821=CARTESIAN_POINT('Ctrl Pts',(-9.70837105736396,16.8255329776774,-334.144834577377)) ;
#31822=CARTESIAN_POINT('Ctrl Pts',(-9.58438292326255,16.8964680516786,-334.146605895128)) ;
#31823=CARTESIAN_POINT('Ctrl Pts',(-9.36185898784423,17.020539078971,-334.149747255704)) ;
#31824=CARTESIAN_POINT('Ctrl Pts',(-9.26362498593705,17.0742029506824,-334.151121145487)) ;
#31825=CARTESIAN_POINT('Ctrl Pts',(-9.02955205330633,17.1994590255382,-334.154365026376)) ;
#31826=CARTESIAN_POINT('Ctrl Pts',(-8.89331722638138,17.2702955924288,-334.156229438772)) ;
#31827=CARTESIAN_POINT('Ctrl Pts',(-8.44821656927212,17.4950664046412,-334.162248417962)) ;
#31828=CARTESIAN_POINT('Ctrl Pts',(-8.13608545504577,17.6423871938157,-334.166356350361)) ;
#31829=CARTESIAN_POINT('Ctrl Pts',(-7.26145445614535,18.0270485847878,-334.177627740218)) ;
#31830=CARTESIAN_POINT('Ctrl Pts',(-6.69144257907105,18.2463091121516,-334.184697804073)) ;
#31831=CARTESIAN_POINT('Ctrl Pts',(-5.83097877883014,18.53154060576,-334.195351718606)) ;
#31832=CARTESIAN_POINT('Ctrl Pts',(-5.54780808086928,18.6182742365684,-334.198857161506)) ;
#31833=CARTESIAN_POINT('Ctrl Pts',(-5.16952436517516,18.7247436726624,-334.203594046749)) ;
#31834=CARTESIAN_POINT('Ctrl Pts',(-5.07608752347006,18.7502891494303,-334.204768451229)) ;
#31835=CARTESIAN_POINT('Ctrl Pts',(-4.91840038492085,18.7921354768562,-334.2067604979)) ;
#31836=CARTESIAN_POINT('Ctrl Pts',(-4.85425063662515,18.8088082793602,-334.207573762549)) ;
#31837=CARTESIAN_POINT('Ctrl Pts',(-4.71239121114863,18.8449040834322,-334.209379186949)) ;
#31838=CARTESIAN_POINT('Ctrl Pts',(-4.6346443741653,18.8641753687738,-334.210373057371)) ;
#31839=CARTESIAN_POINT('Ctrl Pts',(-4.38770282220305,18.9237665649291,-334.21354124599)) ;
#31840=CARTESIAN_POINT('Ctrl Pts',(-4.21808483359718,18.9622951466243,-334.215734308373)) ;
#31841=CARTESIAN_POINT('Ctrl Pts',(-3.78625431788715,19.0543042198343,-334.221341561554)) ;
#31842=CARTESIAN_POINT('Ctrl Pts',(-3.52341190293161,19.1046538658482,-334.224776523735)) ;
#31843=CARTESIAN_POINT('Ctrl Pts',(-2.45960639989161,19.2857335125215,-334.238674905473)) ;
#31844=CARTESIAN_POINT('Ctrl Pts',(-1.65184645812952,19.3716441231337,-334.249182942896)) ;
#31845=CARTESIAN_POINT('Ctrl Pts',(-0.689503890939881,19.4133518377827,
-334.261261090429)) ;
#31846=CARTESIAN_POINT('Ctrl Pts',(-0.537850230463686,19.4181451844941,
-334.263152901883)) ;
#31847=CARTESIAN_POINT('Ctrl Pts',(-0.260502263392738,19.4236597643566,
-334.266591167595)) ;
#31848=CARTESIAN_POINT('Ctrl Pts',(-0.134827284795461,19.4249386542778,
-334.268141087538)) ;
#31849=CARTESIAN_POINT('Ctrl Pts',(0.124518842200064,19.4250607994973,-334.271323305699)) ;
#31850=CARTESIAN_POINT('Ctrl Pts',(0.2581835305543,19.4237440605022,-334.272954489055)) ;
#31851=CARTESIAN_POINT('Ctrl Pts',(0.61113973312722,19.416623088611,-334.27723986224)) ;
#31852=CARTESIAN_POINT('Ctrl Pts',(0.830364918795019,19.4084836673696,-334.279879036645)) ;
#31853=CARTESIAN_POINT('Ctrl Pts',(1.32753338176573,19.3815856349554,-334.285823989006)) ;
#31854=CARTESIAN_POINT('Ctrl Pts',(1.60530578702086,19.3605578498618,-334.289116639316)) ;
#31855=CARTESIAN_POINT('Ctrl Pts',(2.25685442342576,19.2971158559699,-334.29680947418)) ;
#31856=CARTESIAN_POINT('Ctrl Pts',(2.63004145476046,19.2498040050695,-334.301191236327)) ;
#31857=CARTESIAN_POINT('Ctrl Pts',(3.23823228134206,19.1546817263087,-334.308387622607)) ;
#31858=CARTESIAN_POINT('Ctrl Pts',(3.47414076295643,19.1133023341043,-334.311193211085)) ;
#31859=CARTESIAN_POINT('Ctrl Pts',(3.93147985578674,19.0243359513042,-334.316697805706)) ;
#31860=CARTESIAN_POINT('Ctrl Pts',(4.15296303474062,18.9772176552967,-334.319393892073)) ;
#31861=CARTESIAN_POINT('Ctrl Pts',(4.45229957401473,18.9080454469311,-334.323104769871)) ;
#31862=CARTESIAN_POINT('Ctrl Pts',(4.53091348121899,18.8893614800622,-334.324085692013)) ;
#31863=CARTESIAN_POINT('Ctrl Pts',(4.67372734080227,18.8544764314364,-334.325880952515)) ;
#31864=CARTESIAN_POINT('Ctrl Pts',(4.73796539112706,18.8384365783743,-334.326693441782)) ;
#31865=CARTESIAN_POINT('Ctrl Pts',(4.88008928481094,18.8021761623923,-334.328502711755)) ;
#31866=CARTESIAN_POINT('Ctrl Pts',(4.95793384102203,18.7817994844825,-334.329501264188)) ;
#31867=CARTESIAN_POINT('Ctrl Pts',(5.20582194639987,18.7152634994681,-334.332702706351)) ;
#31868=CARTESIAN_POINT('Ctrl Pts',(5.37536487826349,18.6672740978224,-334.334924872975)) ;
#31869=CARTESIAN_POINT('Ctrl Pts',(5.80592576708458,18.5390509134454,-334.340631766853)) ;
#31870=CARTESIAN_POINT('Ctrl Pts',(6.06594783206197,18.4556078031719,-334.344138120188)) ;
#31871=CARTESIAN_POINT('Ctrl Pts',(7.08209615220398,18.1057221974789,-334.357982670507)) ;
#31872=CARTESIAN_POINT('Ctrl Pts',(7.82319024184046,17.7980607967928,-334.368358698966)) ;
#31873=CARTESIAN_POINT('Ctrl Pts',(8.67977105247503,17.3785885647298,-334.380319051033)) ;
#31874=CARTESIAN_POINT('Ctrl Pts',(8.81560029398608,17.3100825407098,-334.382215952489)) ;
#31875=CARTESIAN_POINT('Ctrl Pts',(9.06222758245143,17.1820392440777,-334.385660385211)) ;
#31876=CARTESIAN_POINT('Ctrl Pts',(9.17327890013426,17.1230077851434,-334.387211430201)) ;
#31877=CARTESIAN_POINT('Ctrl Pts',(9.40102028807281,16.9990960422778,-334.390392855248)) ;
#31878=CARTESIAN_POINT('Ctrl Pts',(9.51763054201109,16.9340827219558,-334.392022152738)) ;
#31879=CARTESIAN_POINT('Ctrl Pts',(9.82326402869296,16.7595296492867,-334.396294905916)) ;
#31880=CARTESIAN_POINT('Ctrl Pts',(10.0111256431434,16.6479942883146,-334.398923516916)) ;
#31881=CARTESIAN_POINT('Ctrl Pts',(10.3228053863565,16.4557630767802,-334.403296424333)) ;
#31882=CARTESIAN_POINT('Ctrl Pts',(10.4476559343108,16.3767803618156,-334.40505140074)) ;
#31883=CARTESIAN_POINT('Ctrl Pts',(10.9786591694058,16.0323142947773,-334.412538912018)) ;
#31884=CARTESIAN_POINT('Ctrl Pts',(11.3756880836951,15.7530879412827,-334.418192080288)) ;
#31885=CARTESIAN_POINT('Ctrl Pts',(11.864769683699,15.3809814757215,-334.425373483521)) ;
#31886=CARTESIAN_POINT('Ctrl Pts',(11.9669103162139,15.3016472404185,-334.426886135509)) ;
#31887=CARTESIAN_POINT('Ctrl Pts',(12.3149650574973,15.0256910292463,-334.432095155414)) ;
#31888=CARTESIAN_POINT('Ctrl Pts',(12.5568864500716,14.8241140441618,-334.435809919664)) ;
#31889=CARTESIAN_POINT('Ctrl Pts',(12.8770812712878,14.5438527268276,-334.440922023936)) ;
#31890=CARTESIAN_POINT('Ctrl Pts',(12.9597372553524,14.4702482503935,-334.442260007276)) ;
#31891=CARTESIAN_POINT('Ctrl Pts',(13.0874778812556,14.3545237920577,-334.444360258854)) ;
#31892=CARTESIAN_POINT('Ctrl Pts',(13.1329985978956,14.3128885418513,-334.44511521892)) ;
#31893=CARTESIAN_POINT('Ctrl Pts',(13.2308768379954,14.2225047265733,-334.44675361316)) ;
#31894=CARTESIAN_POINT('Ctrl Pts',(13.2831649466434,14.173682357935,-334.447638273811)) ;
#31895=CARTESIAN_POINT('Ctrl Pts',(13.4273839481385,14.0375234280768,-334.450102943273)) ;
#31896=CARTESIAN_POINT('Ctrl Pts',(13.5187311184769,13.9495739202564,-334.451692091572)) ;
#31897=CARTESIAN_POINT('Ctrl Pts',(13.7294001720252,13.7427278049008,-334.455416038119)) ;
#31898=CARTESIAN_POINT('Ctrl Pts',(13.8480497449699,13.6231609674283,-334.457558474823)) ;
#31899=CARTESIAN_POINT('Ctrl Pts',(14.2988121341239,13.1569393685709,-334.465849427585)) ;
#31900=CARTESIAN_POINT('Ctrl Pts',(14.6195865231154,12.7995613987023,-334.472069508058)) ;
#31901=CARTESIAN_POINT('Ctrl Pts',(15.2455699376987,12.047878240723,-334.484664107277)) ;
#31902=CARTESIAN_POINT('Ctrl Pts',(15.5495062383087,11.652966621828,-334.491030249142)) ;
#31903=CARTESIAN_POINT('Ctrl Pts',(15.9272817524453,11.1209774255067,-334.499215896157)) ;
#31904=CARTESIAN_POINT('Ctrl Pts',(16.0151343417675,10.994085456421,-334.501141069363)) ;
#31905=CARTESIAN_POINT('Ctrl Pts',(16.17208476471,10.7615164683546,-334.504619873024)) ;
#31906=CARTESIAN_POINT('Ctrl Pts',(16.2416822384837,10.6561869563588,-334.506177285148)) ;
#31907=CARTESIAN_POINT('Ctrl Pts',(16.3822961557718,10.4388023738032,-334.50935501507)) ;
#31908=CARTESIAN_POINT('Ctrl Pts',(16.453201442586,10.3266831403083,-334.51097442404)) ;
#31909=CARTESIAN_POINT('Ctrl Pts',(16.6353392518003,10.0320385648566,-334.515180930944)) ;
#31910=CARTESIAN_POINT('Ctrl Pts',(16.7447174510192,9.84838806535011,-334.517754068654)) ;
#31911=CARTESIAN_POINT('Ctrl Pts',(16.922227487327,9.53883217616622,-334.522017931058)) ;
#31912=CARTESIAN_POINT('Ctrl Pts',(16.9920384034922,9.4139116930759,-334.523719148186)) ;
#31913=CARTESIAN_POINT('Ctrl Pts',(17.2799231723973,8.88512992007277,-334.530846968818)) ;
#31914=CARTESIAN_POINT('Ctrl Pts',(17.4850282774572,8.47437697204201,-334.536201904592)) ;
#31915=CARTESIAN_POINT('Ctrl Pts',(17.8696485059172,7.63057312607779,-334.547033824975)) ;
#31916=CARTESIAN_POINT('Ctrl Pts',(18.0484281152728,7.19751514768427,-334.552507699877)) ;
#31917=CARTESIAN_POINT('Ctrl Pts',(18.2527768518267,6.64687286975248,-334.55955143004)) ;
#31918=CARTESIAN_POINT('Ctrl Pts',(18.2931477771119,6.53494652555024,-334.560987653462)) ;
#31919=CARTESIAN_POINT('Ctrl Pts',(18.3533579661568,6.36308577665903,-334.563204274281)) ;
#31920=CARTESIAN_POINT('Ctrl Pts',(18.3739376464864,6.30341372487098,-334.563975990038)) ;
#31921=CARTESIAN_POINT('Ctrl Pts',(18.4165977216969,6.17773403193171,-334.565606685783)) ;
#31922=CARTESIAN_POINT('Ctrl Pts',(18.4386149160791,6.11170592877813,-334.566466537116)) ;
#31923=CARTESIAN_POINT('Ctrl Pts',(18.4966957532922,5.93435459209416,-334.568783110975)) ;
#31924=CARTESIAN_POINT('Ctrl Pts',(18.5321091190621,5.82282145989313,-334.570247325835)) ;
#31925=CARTESIAN_POINT('Ctrl Pts',(18.7398594809636,5.14742023960839,-334.579144123232)) ;
#31926=CARTESIAN_POINT('Ctrl Pts',(18.8874578434867,4.57626528498771,-334.58678395247)) ;
#31927=CARTESIAN_POINT('Ctrl Pts',(19.0621695167566,3.74584977088118,-334.597725919259)) ;
#31928=CARTESIAN_POINT('Ctrl Pts',(19.1104161528741,3.49137392110125,-334.601058634067)) ;
#31929=CARTESIAN_POINT('Ctrl Pts',(19.2118003405683,2.89129282172694,-334.608842610779)) ;
#31930=CARTESIAN_POINT('Ctrl Pts',(19.2607239090064,2.54506619183486,-334.613275146882)) ;
#31931=CARTESIAN_POINT('Ctrl Pts',(19.3181680777768,2.04059127631761,-334.619629037976)) ;
#31932=CARTESIAN_POINT('Ctrl Pts',(19.3341396084398,1.88326215243514,-334.621596152364)) ;
#31933=CARTESIAN_POINT('Ctrl Pts',(19.3592230421088,1.60204096113557,-334.625086341218)) ;
#31934=CARTESIAN_POINT('Ctrl Pts',(19.3690709023552,1.47822341394301,-334.626614070654)) ;
#31935=CARTESIAN_POINT('Ctrl Pts',(19.3877949863084,1.21031753268275,-334.629900872155)) ;
#31936=CARTESIAN_POINT('Ctrl Pts',(19.3962538865434,1.06620739104831,-334.6316571584)) ;
#31937=CARTESIAN_POINT('Ctrl Pts',(19.4164624701931,0.640933667484384,-334.636808043619)) ;
#31938=CARTESIAN_POINT('Ctrl Pts',(19.4237098311887,0.359593733983076,-334.640174001494)) ;
#31939=CARTESIAN_POINT('Ctrl Pts',(19.4264955186439,-0.332409683582954,
-334.648380355026)) ;
#31940=CARTESIAN_POINT('Ctrl Pts',(19.4151288650228,-0.742964319775833,
-334.653184693709)) ;
#31941=CARTESIAN_POINT('Ctrl Pts',(19.3578940572392,-1.70564529116212,-334.664449441326)) ;
#31942=CARTESIAN_POINT('Ctrl Pts',(19.301404710087,-2.25678104368422,-334.670894887691)) ;
#31943=CARTESIAN_POINT('Ctrl Pts',(19.2049678140431,-2.91768092711522,-334.678912798869)) ;
#31944=CARTESIAN_POINT('Ctrl Pts',(19.1874937363946,-3.03046775120494,-334.680291650034)) ;
#31945=CARTESIAN_POINT('Ctrl Pts',(19.1589506884336,-3.20454541803918,-334.682440136039)) ;
#31946=CARTESIAN_POINT('Ctrl Pts',(19.1485792102026,-3.26594810704615,-334.683201900217)) ;
#31947=CARTESIAN_POINT('Ctrl Pts',(19.1258123312159,-3.39689829664632,-334.684835799605)) ;
#31948=CARTESIAN_POINT('Ctrl Pts',(19.1133324431301,-3.46643019059573,-334.685709006972)) ;
#31949=CARTESIAN_POINT('Ctrl Pts',(19.0782086967679,-3.65616452493381,-334.688105686054)) ;
#31950=CARTESIAN_POINT('Ctrl Pts',(19.054808361097,-3.77622355869785,-334.689637530054)) ;
#31951=CARTESIAN_POINT('Ctrl Pts',(18.9981436465971,-4.05300239806385,-334.69319815189)) ;
#31952=CARTESIAN_POINT('Ctrl Pts',(18.9640712454272,-4.2095477366355,-334.695233716727)) ;
#31953=CARTESIAN_POINT('Ctrl Pts',(18.8309354854158,-4.78678148261534,-334.702799672112)) ;
#31954=CARTESIAN_POINT('Ctrl Pts',(18.7197773055192,-5.20455047700074,-334.708391575344)) ;
#31955=CARTESIAN_POINT('Ctrl Pts',(18.5684397585047,-5.70543268815176,-334.715137184554)) ;
#31956=CARTESIAN_POINT('Ctrl Pts',(18.5414894993282,-5.79241610868852,-334.71631028718)) ;
#31957=CARTESIAN_POINT('Ctrl Pts',(18.3697224867553,-6.3333193812925,-334.723612021278)) ;
#31958=CARTESIAN_POINT('Ctrl Pts',(18.2088570919137,-6.78197347736084,-334.729693862465)) ;
#31959=CARTESIAN_POINT('Ctrl Pts',(17.9749958220313,-7.36568822842079,-334.737579636723)) ;
#31960=CARTESIAN_POINT('Ctrl Pts',(17.9166711744184,-7.50644602941054,-334.739479558734)) ;
#31961=CARTESIAN_POINT('Ctrl Pts',(17.807171071639,-7.76215900802771,-334.742927654322)) ;
#31962=CARTESIAN_POINT('Ctrl Pts',(17.7565230416508,-7.87733099218671,-334.744479370161)) ;
#31963=CARTESIAN_POINT('Ctrl Pts',(17.6498706987718,-8.11359893735732,-334.7476603437)) ;
#31964=CARTESIAN_POINT('Ctrl Pts',(17.593730467232,-8.23462638514033,-334.749288537846)) ;
#31965=CARTESIAN_POINT('Ctrl Pts',(17.4426099123047,-8.55181150737795,-334.753553906259)) ;
#31966=CARTESIAN_POINT('Ctrl Pts',(17.3455674619773,-8.74696577419348,-334.756176335411)) ;
#31967=CARTESIAN_POINT('Ctrl Pts',(17.1775069612165,-9.07113834075854,-334.760537050718)) ;
#31968=CARTESIAN_POINT('Ctrl Pts',(17.108268710975,-9.20105635074467,-334.762285996648)) ;
#31969=CARTESIAN_POINT('Ctrl Pts',(16.8059554315782,-9.75310181943261,-334.769732223868)) ;
#31970=CARTESIAN_POINT('Ctrl Pts',(16.558683069537,-10.1672586446759,-334.775351045869)) ;
#31971=CARTESIAN_POINT('Ctrl Pts',(16.1822448993713,-10.7475328032465,-334.783433351497)) ;
#31972=CARTESIAN_POINT('Ctrl Pts',(16.0653969918523,-10.9214253069532,-334.785884418162)) ;
#31973=CARTESIAN_POINT('Ctrl Pts',(15.7902093765532,-11.3169828494484,-334.791556433841)) ;
#31974=CARTESIAN_POINT('Ctrl Pts',(15.6299740795108,-11.5372753581351,-334.794786836622)) ;
#31975=CARTESIAN_POINT('Ctrl Pts',(15.4134379894353,-11.8221766417319,-334.79910280901)) ;
#31976=CARTESIAN_POINT('Ctrl Pts',(15.3612674408727,-11.8898861974324,-334.800139098917)) ;
#31977=CARTESIAN_POINT('Ctrl Pts',(15.2677723592363,-12.0095862745577,-334.801991920674)) ;
#31978=CARTESIAN_POINT('Ctrl Pts',(15.2266248676298,-12.0617134126996,-334.802805937522)) ;
#31979=CARTESIAN_POINT('Ctrl Pts',(15.1372936228876,-12.1736958606878,-334.804571030093)) ;
#31980=CARTESIAN_POINT('Ctrl Pts',(15.0890204863635,-12.2334782411454,-334.805523357729)) ;
#31981=CARTESIAN_POINT('Ctrl Pts',(14.9424018823832,-12.4128654115637,-334.808409244295)) ;
#31982=CARTESIAN_POINT('Ctrl Pts',(14.842979855528,-12.5315821277078,-334.810357316582)) ;
#31983=CARTESIAN_POINT('Ctrl Pts',(14.6645607892344,-12.7395242798043,-334.813828429465)) ;
#31984=CARTESIAN_POINT('Ctrl Pts',(14.5861420288576,-12.8292354678863,-334.815345872513)) ;
#31985=CARTESIAN_POINT('Ctrl Pts',(14.1944166568483,-13.2691352533951,-334.822875088162)) ;
#31986=CARTESIAN_POINT('Ctrl Pts',(13.8693005980717,-13.6085971192817,-334.828961637716)) ;
#31987=CARTESIAN_POINT('Ctrl Pts',(13.4868948813232,-13.9799241303449,-334.8358266719)) ;
#31988=CARTESIAN_POINT('Ctrl Pts',(13.4413793458772,-14.023691864575,-334.836639339529)) ;
#31989=CARTESIAN_POINT('Ctrl Pts',(13.0619152649048,-14.3850399041647,-334.843376442844)) ;
#31990=CARTESIAN_POINT('Ctrl Pts',(12.7169748762829,-14.690866395463,-334.849252819499)) ;
#31991=CARTESIAN_POINT('Ctrl Pts',(12.2346115849936,-15.088802343119,-334.857090671779)) ;
#31992=CARTESIAN_POINT('Ctrl Pts',(12.1064144226376,-15.1918533010078,-334.859139626251)) ;
#31993=CARTESIAN_POINT('Ctrl Pts',(11.8784274358333,-15.3704013742308,-334.862723697414)) ;
#31994=CARTESIAN_POINT('Ctrl Pts',(11.7791879937148,-15.4465856100895,-334.86426435134)) ;
#31995=CARTESIAN_POINT('Ctrl Pts',(11.5763506343292,-15.5992084459143,-334.867374646476)) ;
#31996=CARTESIAN_POINT('Ctrl Pts',(11.4727148317295,-15.6755865149792,-334.868943753308)) ;
#31997=CARTESIAN_POINT('Ctrl Pts',(11.1812381850836,-15.8859615339028,-334.873302931403)) ;
#31998=CARTESIAN_POINT('Ctrl Pts',(10.9917577893027,-16.0176503323075,-334.876074902452)) ;
#31999=CARTESIAN_POINT('Ctrl Pts',(10.5475633085915,-16.3147709755197,-334.882445318473)) ;
#32000=CARTESIAN_POINT('Ctrl Pts',(10.2912255975046,-16.4776673049456,-334.886026786228)) ;
#32001=CARTESIAN_POINT('Ctrl Pts',(9.73819263880107,-16.8111654154795,-334.89360137547)) ;
#32002=CARTESIAN_POINT('Ctrl Pts',(9.44059423175864,-16.9800724097364,-334.897587649871)) ;
#32003=CARTESIAN_POINT('Ctrl Pts',(9.0159245438828,-17.2064838124149,-334.903215431777)) ;
#32004=CARTESIAN_POINT('Ctrl Pts',(8.89245874074754,-17.2706154517907,-334.904844765602)) ;
#32005=CARTESIAN_POINT('Ctrl Pts',(8.50494782159208,-17.4666424705805,-334.90994895841)) ;
#32006=CARTESIAN_POINT('Ctrl Pts',(8.23857914032455,-17.5938497693262,-334.91344319999)) ;
#32007=CARTESIAN_POINT('Ctrl Pts',(7.88120251882413,-17.7546227337772,-334.918166919395)) ;
#32008=CARTESIAN_POINT('Ctrl Pts',(7.79269356099606,-17.793647984327,-334.919339719362)) ;
#32009=CARTESIAN_POINT('Ctrl Pts',(7.6430660818716,-17.8582909855102,-334.921329968823)) ;
#32010=CARTESIAN_POINT('Ctrl Pts',(7.58210126016342,-17.8842600221946,-334.922143061582)) ;
#32011=CARTESIAN_POINT('Ctrl Pts',(7.46899527689833,-17.931757207155,-334.923656138937)) ;
#32012=CARTESIAN_POINT('Ctrl Pts',(7.41689106658348,-17.9533711007519,-334.924354843448)) ;
#32013=CARTESIAN_POINT('Ctrl Pts',(7.35876822609363,-17.9771854359115,-334.925135815056)) ;
#32014=CARTESIAN_POINT('Ctrl Pts',(7.35284176862584,-17.9796102273674,-334.925215464332)) ;
#32015=CARTESIAN_POINT('Ctrl Pts',(7.34059571155037,-17.9846135956811,-334.925380082952)) ;
#32016=CARTESIAN_POINT('Ctrl Pts',(7.33427594971204,-17.9871917730326,-334.925465056875)) ;
#32017=CARTESIAN_POINT('Ctrl Pts',(7.32110337465282,-17.9925574921708,-334.925642212687)) ;
#32018=CARTESIAN_POINT('Ctrl Pts',(7.31425032521435,-17.9953444510382,-334.925734401166)) ;
#32019=CARTESIAN_POINT('Ctrl Pts',(7.29984921075362,-18.0011914282705,-334.9259281745)) ;
#32020=CARTESIAN_POINT('Ctrl Pts',(7.29230081000141,-18.0042506157132,-334.926029768605)) ;
#32021=CARTESIAN_POINT('Ctrl Pts',(7.28313043062368,-18.0079604393346,-334.926153224825)) ;
#32022=CARTESIAN_POINT('Ctrl Pts',(7.28151028477896,-18.0086156055032,-334.926175037244)) ;
#32023=CARTESIAN_POINT('Ctrl Pts',(7.27777929594972,-18.0101237836594,-334.926225271219)) ;
#32024=CARTESIAN_POINT('Ctrl Pts',(7.27566839139559,-18.0109766431955,-334.926253694441)) ;
#32025=CARTESIAN_POINT('Ctrl Pts',(7.27077911679054,-18.0129510356304,-334.926319532947)) ;
#32026=CARTESIAN_POINT('Ctrl Pts',(7.26800063717667,-18.0140722968232,-334.926356951185)) ;
#32027=CARTESIAN_POINT('Ctrl Pts',(7.26151933851884,-18.0166860946971,-334.926444243946)) ;
#32028=CARTESIAN_POINT('Ctrl Pts',(7.25781631861398,-18.0181781327578,-334.926494123855)) ;
#32029=CARTESIAN_POINT('Ctrl Pts',(7.24910376199596,-18.0216855150923,-334.926611496741)) ;
#32030=CARTESIAN_POINT('Ctrl Pts',(7.24409384452291,-18.0236999123046,-334.926678999855)) ;
#32031=CARTESIAN_POINT('Ctrl Pts',(7.23218566214197,-18.028482209982,-334.926839475173)) ;
#32032=CARTESIAN_POINT('Ctrl Pts',(7.22528664743942,-18.0312482404754,-334.926932467153)) ;
#32033=CARTESIAN_POINT('Ctrl Pts',(7.00269667854131,-18.1203432502996,-334.929933403537)) ;
#32034=CARTESIAN_POINT('Ctrl Pts',(6.78547612516215,-18.2027996114837,-334.932881126412)) ;
#32035=CARTESIAN_POINT('Ctrl Pts',(6.13301935114675,-18.4371682293537,-334.941741166967)) ;
#32036=CARTESIAN_POINT('Ctrl Pts',(5.6938002848191,-18.5775062096151,-334.947710492633)) ;
#32037=CARTESIAN_POINT('Ctrl Pts',(5.0463101262993,-18.7592681318011,-334.956374340118)) ;
#32038=CARTESIAN_POINT('Ctrl Pts',(4.84169341590354,-18.8131175437422,-334.959093465878)) ;
#32039=CARTESIAN_POINT('Ctrl Pts',(4.29992491791702,-18.9462716498603,-334.966227774864)) ;
#32040=CARTESIAN_POINT('Ctrl Pts',(3.96146110807376,-19.0199208859464,-334.970618015183)) ;
#32041=CARTESIAN_POINT('Ctrl Pts',(3.4660359946238,-19.1139259467775,-334.976928232904)) ;
#32042=CARTESIAN_POINT('Ctrl Pts',(3.31050942772025,-19.141475858428,-334.97889291829)) ;
#32043=CARTESIAN_POINT('Ctrl Pts',(3.03212029015865,-19.1872951536998,-334.982380503251)) ;
#32044=CARTESIAN_POINT('Ctrl Pts',(2.9093858334737,-19.2062886286724,-334.983908030054)) ;
#32045=CARTESIAN_POINT('Ctrl Pts',(2.67064164709251,-19.2408938998855,-334.986860391166)) ;
#32046=CARTESIAN_POINT('Ctrl Pts',(2.55465623886165,-19.256636684872,-334.988286018659)) ;
#32047=CARTESIAN_POINT('Ctrl Pts',(2.29624680491736,-19.2893350293378,-334.991443954951)) ;
#32048=CARTESIAN_POINT('Ctrl Pts',(2.15376290812911,-19.3057634053631,-334.993172865671)) ;
#32049=CARTESIAN_POINT('Ctrl Pts',(1.34283424036464,-19.3901741251841,-335.002949862918)) ;
#32050=CARTESIAN_POINT('Ctrl Pts',(0.671398683770775,-19.4250168820751,
-335.010784597034)) ;
#32051=CARTESIAN_POINT('Ctrl Pts',(-0.000488257005959863,-19.4249999938637,
-335.018634132644)) ;
#32052=CARTESIAN_POINT('Origin',(0.,0.,-328.125)) ;
#32053=CARTESIAN_POINT('',(0.000403208488304671,-19.4249999958153,-336.731156847152)) ;
#32054=CARTESIAN_POINT('',(2.0594453916303E-9,-19.425,-336.519643262718)) ;
#32055=CARTESIAN_POINT('',(-2.37887640734373E-15,-19.425,-328.125)) ;
#32056=CARTESIAN_POINT('Ctrl Pts',(0.000397956517500714,-19.4247394275783,
-336.730705552561)) ;
#32057=CARTESIAN_POINT('Ctrl Pts',(0.417181488622901,-19.4248114247665,
-336.725723703886)) ;
#32058=CARTESIAN_POINT('Ctrl Pts',(0.833910655153896,-19.4114928611389,
-336.720789889741)) ;
#32059=CARTESIAN_POINT('Ctrl Pts',(1.24973803346114,-19.3847950115984,-336.715859644829)) ;
#32060=CARTESIAN_POINT('Ctrl Pts',(1.66569352250536,-19.3580889368151,-336.710927880977)) ;
#32061=CARTESIAN_POINT('Ctrl Pts',(2.08074675907296,-19.3179951449265,-336.705999533908)) ;
#32062=CARTESIAN_POINT('Ctrl Pts',(2.49404451930397,-19.2645639374455,-336.701006302343)) ;
#32063=CARTESIAN_POINT('Ctrl Pts',(2.77527427666225,-19.2282065047151,-336.697608642262)) ;
#32064=CARTESIAN_POINT('Ctrl Pts',(3.05569110924822,-19.1856744275963,-336.694180437861)) ;
#32065=CARTESIAN_POINT('Ctrl Pts',(3.33502460600275,-19.1369946814523,-336.69069454568)) ;
#32066=CARTESIAN_POINT('Ctrl Pts',(3.73266187925462,-19.0676980101108,-336.685732302778)) ;
#32067=CARTESIAN_POINT('Ctrl Pts',(4.12817743095628,-18.9859283585497,-336.680653272706)) ;
#32068=CARTESIAN_POINT('Ctrl Pts',(4.52078979820639,-18.8918837491355,-336.675533912964)) ;
#32069=CARTESIAN_POINT('Ctrl Pts',(4.91310476537855,-18.7979103776049,-336.670418431087)) ;
#32070=CARTESIAN_POINT('Ctrl Pts',(5.30252101598689,-18.691680818477,-336.665262846928)) ;
#32071=CARTESIAN_POINT('Ctrl Pts',(5.68827676331055,-18.5734305685259,-336.660123589436)) ;
#32072=CARTESIAN_POINT('Ctrl Pts',(6.07399111223989,-18.455193008912,-336.654984883478)) ;
#32073=CARTESIAN_POINT('Ctrl Pts',(6.45604581295528,-18.3249374404889,-336.649862604335)) ;
#32074=CARTESIAN_POINT('Ctrl Pts',(6.83369616006065,-18.1829351066735,-336.644791285714)) ;
#32075=CARTESIAN_POINT('Ctrl Pts',(7.21132355562628,-18.0409414029897,-336.639720275299)) ;
#32076=CARTESIAN_POINT('Ctrl Pts',(7.58454718817121,-17.8872023967985,-336.634700265376)) ;
#32077=CARTESIAN_POINT('Ctrl Pts',(7.95263837668096,-17.7220240807298,-336.629742789312)) ;
#32078=CARTESIAN_POINT('Ctrl Pts',(8.32130519074602,-17.5565874567666,-336.624777560686)) ;
#32079=CARTESIAN_POINT('Ctrl Pts',(8.68482352257974,-17.3796756825354,-336.61987506014)) ;
#32080=CARTESIAN_POINT('Ctrl Pts',(9.04247658715762,-17.1916311113474,-336.615023464694)) ;
#32081=CARTESIAN_POINT('Ctrl Pts',(9.39960785268114,-17.0038608883733,-336.610178947498)) ;
#32082=CARTESIAN_POINT('Ctrl Pts',(9.75089095264054,-16.8049902574347,-336.605385119696)) ;
#32083=CARTESIAN_POINT('Ctrl Pts',(10.0956272775635,-16.5953956451601,-336.600607418064)) ;
#32084=CARTESIAN_POINT('Ctrl Pts',(10.4411191359784,-16.3853416796412,-336.595819245492)) ;
#32085=CARTESIAN_POINT('Ctrl Pts',(10.7800354361742,-16.1645165305077,-336.591047157463)) ;
#32086=CARTESIAN_POINT('Ctrl Pts',(11.1116885036331,-15.9333365194949,-336.586234776286)) ;
#32087=CARTESIAN_POINT('Ctrl Pts',(11.443341571092,-15.7021565084822,-336.581422395109)) ;
#32088=CARTESIAN_POINT('Ctrl Pts',(11.7677312947932,-15.4606214608348,-336.576569535009)) ;
#32089=CARTESIAN_POINT('Ctrl Pts',(12.0841867469861,-15.2091874595654,-336.571600497178)) ;
#32090=CARTESIAN_POINT('Ctrl Pts',(12.4002102400622,-14.9580966636614,-336.566638242043)) ;
#32091=CARTESIAN_POINT('Ctrl Pts',(12.7084032091301,-14.6970680724526,-336.561559204438)) ;
#32092=CARTESIAN_POINT('Ctrl Pts',(13.0081741684115,-14.4266494454657,-336.556439840925)) ;
#32093=CARTESIAN_POINT('Ctrl Pts',(13.3077181659163,-14.156435557097,-336.55132435337)) ;
#32094=CARTESIAN_POINT('Ctrl Pts',(13.5988530508822,-13.8768459710949,-336.546168767258)) ;
#32095=CARTESIAN_POINT('Ctrl Pts',(13.8810225436247,-13.5884519413831,-336.541029510624)) ;
#32096=CARTESIAN_POINT('Ctrl Pts',(14.1631617563221,-13.3000888596811,-336.535890805491)) ;
#32097=CARTESIAN_POINT('Ctrl Pts',(14.4363376106901,-13.0029232802281,-336.530768529981)) ;
#32098=CARTESIAN_POINT('Ctrl Pts',(14.7000259285989,-12.6975496750222,-336.525697216853)) ;
#32099=CARTESIAN_POINT('Ctrl Pts',(14.9636982223526,-12.3921946271573,-336.520626211905)) ;
#32100=CARTESIAN_POINT('Ctrl Pts',(15.2178841980396,-12.0786325555002,-336.515606209307)) ;
#32101=CARTESIAN_POINT('Ctrl Pts',(15.4620903737834,-11.7574807799444,-336.510648741478)) ;
#32102=CARTESIAN_POINT('Ctrl Pts',(15.7066782786258,-11.4358269983383,-336.50568352442)) ;
#32103=CARTESIAN_POINT('Ctrl Pts',(15.9412551663695,-11.106559723592,-336.500781036268)) ;
#32104=CARTESIAN_POINT('Ctrl Pts',(16.1653553980525,-10.7703225124114,-336.495929453147)) ;
#32105=CARTESIAN_POINT('Ctrl Pts',(16.3891288296542,-10.4345756280238,-336.491084944975)) ;
#32106=CARTESIAN_POINT('Ctrl Pts',(16.6024561041871,-10.0918790576013,-336.486291126198)) ;
#32107=CARTESIAN_POINT('Ctrl Pts',(16.8049038436912,-9.74289758437938,-336.481513432745)) ;
#32108=CARTESIAN_POINT('Ctrl Pts',(17.0077950670615,-9.39315162915654,-336.476725273233)) ;
#32109=CARTESIAN_POINT('Ctrl Pts',(17.1997589195039,-9.03709310484679,-336.471953197376)) ;
#32110=CARTESIAN_POINT('Ctrl Pts',(17.3803907133679,-8.67541659417091,-336.467140826901)) ;
#32111=CARTESIAN_POINT('Ctrl Pts',(17.5610225072322,-8.31374008349453,-336.462328456426)) ;
#32112=CARTESIAN_POINT('Ctrl Pts',(17.7303220614185,-7.9464454861091,-336.457475605556)) ;
#32113=CARTESIAN_POINT('Ctrl Pts',(17.8879184167642,-7.57425428821266,-336.452506575107)) ;
#32114=CARTESIAN_POINT('Ctrl Pts',(18.0452997522663,-7.20257089706718,-336.447544324257)) ;
#32115=CARTESIAN_POINT('Ctrl Pts',(18.1910503965086,-6.82590715285856,-336.442465288938)) ;
#32116=CARTESIAN_POINT('Ctrl Pts',(18.3249130098465,-6.44502704079927,-336.43734592625)) ;
#32117=CARTESIAN_POINT('Ctrl Pts',(18.4586741782345,-6.06443557067592,-336.432230443162)) ;
#32118=CARTESIAN_POINT('Ctrl Pts',(18.5805655177904,-5.67963415908177,-336.427074860113)) ;
#32119=CARTESIAN_POINT('Ctrl Pts',(18.6903718452331,-5.29139057726848,-336.421935605528)) ;
#32120=CARTESIAN_POINT('Ctrl Pts',(18.8001663884123,-4.90318866122054,-336.416796902482)) ;
#32121=CARTESIAN_POINT('Ctrl Pts',(18.8978786366604,-4.51154531074026,-336.411674628045)) ;
#32122=CARTESIAN_POINT('Ctrl Pts',(18.9833327041114,-4.11723332735543,-336.406603315378)) ;
#32123=CARTESIAN_POINT('Ctrl Pts',(19.0687815781059,-3.72294530821419,-336.401532310919)) ;
#32124=CARTESIAN_POINT('Ctrl Pts',(19.1419738207046,-3.32598895314096,-336.396512308198)) ;
#32125=CARTESIAN_POINT('Ctrl Pts',(19.2027714323094,-2.9271424411949,-336.391554840038)) ;
#32126=CARTESIAN_POINT('Ctrl Pts',(19.2636641561563,-2.52767197075691,-336.386589616378)) ;
#32127=CARTESIAN_POINT('Ctrl Pts',(19.3121234236185,-2.12630538368973,-336.38168712158)) ;
#32128=CARTESIAN_POINT('Ctrl Pts',(19.3480482367358,-1.72383058058084,-336.376835532106)) ;
#32129=CARTESIAN_POINT('Ctrl Pts',(19.3839206160168,-1.32194320705312,-336.37199102374)) ;
#32130=CARTESIAN_POINT('Ctrl Pts',(19.4072950430532,-0.918950811292931,
-336.36719720493)) ;
#32131=CARTESIAN_POINT('Ctrl Pts',(19.4181090048869,-0.515644496032888,
-336.362419511952)) ;
#32132=CARTESIAN_POINT('Ctrl Pts',(19.4289466765016,-0.111453925347685,
-336.357631343808)) ;
#32133=CARTESIAN_POINT('Ctrl Pts',(19.4271685926751,0.293051974743328,-336.352859259899)) ;
#32134=CARTESIAN_POINT('Ctrl Pts',(19.4127516909178,0.697069655333783,-336.348046881928)) ;
#32135=CARTESIAN_POINT('Ctrl Pts',(19.3983347891605,1.10108733592369,-336.343234503957)) ;
#32136=CARTESIAN_POINT('Ctrl Pts',(19.3712788624363,1.50461679848425,-336.338381646147)) ;
#32137=CARTESIAN_POINT('Ctrl Pts',(19.3316033377714,1.9068470059226,-336.333412609093)) ;
#32138=CARTESIAN_POINT('Ctrl Pts',(19.2919819916405,2.30852795174019,-336.32845035746)) ;
#32139=CARTESIAN_POINT('Ctrl Pts',(19.2397646789853,2.70901787938607,-336.323371321958)) ;
#32140=CARTESIAN_POINT('Ctrl Pts',(19.1750909318642,3.1075227944095,-336.318251959449)) ;
#32141=CARTESIAN_POINT('Ctrl Pts',(19.1104661629915,3.5057259166096,-336.313136473897)) ;
#32142=CARTESIAN_POINT('Ctrl Pts',(19.0334040050997,3.90194708926831,-336.307980888707)) ;
#32143=CARTESIAN_POINT('Ctrl Pts',(18.9440828204927,4.29540916073728,-336.302841632186)) ;
#32144=CARTESIAN_POINT('Ctrl Pts',(18.8547712213034,4.68882900819909,-336.297702927179)) ;
#32145=CARTESIAN_POINT('Ctrl Pts',(18.7532033333435,5.07949040829823,-336.292580650987)) ;
#32146=CARTESIAN_POINT('Ctrl Pts',(18.6395944337072,5.46663059300599,-336.287509336649)) ;
#32147=CARTESIAN_POINT('Ctrl Pts',(18.5259924382392,5.85374725067457,-336.282438330503)) ;
#32148=CARTESIAN_POINT('Ctrl Pts',(18.4003509336652,6.23734317341979,-336.277418326181)) ;
#32149=CARTESIAN_POINT('Ctrl Pts',(18.2629210388392,6.61666899676879,-336.272460856384)) ;
#32150=CARTESIAN_POINT('Ctrl Pts',(18.1252762735369,6.99658789282885,-336.267495635625)) ;
#32151=CARTESIAN_POINT('Ctrl Pts',(17.9758061945978,7.37222335572817,-336.262593143574)) ;
#32152=CARTESIAN_POINT('Ctrl Pts',(17.8147990632875,7.74283518875109,-336.257741556614)) ;
#32153=CARTESIAN_POINT('Ctrl Pts',(17.6540267813688,8.1129064372497,-336.252897046311)) ;
#32154=CARTESIAN_POINT('Ctrl Pts',(17.4817510074677,8.47796870558782,-336.248103225427)) ;
#32155=CARTESIAN_POINT('Ctrl Pts',(17.2982953304001,8.83729739527294,-336.243325530142)) ;
#32156=CARTESIAN_POINT('Ctrl Pts',(17.1144376768194,9.19741342332789,-336.238537366272)) ;
#32157=CARTESIAN_POINT('Ctrl Pts',(16.9193509244493,9.55177067442556,-336.233765286353)) ;
#32158=CARTESIAN_POINT('Ctrl Pts',(16.7133992577366,9.89965249773097,-336.228952912242)) ;
#32159=CARTESIAN_POINT('Ctrl Pts',(16.5074475910245,10.2475343210354,-336.224140538132)) ;
#32160=CARTESIAN_POINT('Ctrl Pts',(16.2906308274627,10.5889406187893,-336.219287684055)) ;
#32161=CARTESIAN_POINT('Ctrl Pts',(16.0633540450927,10.9231684924966,-336.214318650879)) ;
#32162=CARTESIAN_POINT('Ctrl Pts',(15.836387425919,11.2569402475256,-336.209356398912)) ;
#32163=CARTESIAN_POINT('Ctrl Pts',(15.5989297383643,11.5836399182122,-336.204277363033)) ;
#32164=CARTESIAN_POINT('Ctrl Pts',(15.3514833758824,11.902637030503,-336.19915800018)) ;
#32165=CARTESIAN_POINT('Ctrl Pts',(15.1042244749132,12.2213924755467,-336.194042515676)) ;
#32166=CARTESIAN_POINT('Ctrl Pts',(14.8469921633439,12.532457167964,-336.188886931587)) ;
#32167=CARTESIAN_POINT('Ctrl Pts',(14.5803148741814,12.835234001684,-336.18374767623)) ;
#32168=CARTESIAN_POINT('Ctrl Pts',(14.313666203832,13.1379783425222,-336.178608972399)) ;
#32169=CARTESIAN_POINT('Ctrl Pts',(14.0375746473913,13.4324367087426,-336.173486697444)) ;
#32170=CARTESIAN_POINT('Ctrl Pts',(13.7525941723335,13.7180422858725,-336.168415384415)) ;
#32171=CARTESIAN_POINT('Ctrl Pts',(13.4676310163982,14.0036305058906,-336.163344379585)) ;
#32172=CARTESIAN_POINT('Ctrl Pts',(13.173780031458,14.2803670776265,-336.158324376649)) ;
#32173=CARTESIAN_POINT('Ctrl Pts',(12.871620246085,14.5477141042196,-336.153366908317)) ;
#32174=CARTESIAN_POINT('Ctrl Pts',(12.568987890871,14.815479254428,-336.148401686636)) ;
#32175=CARTESIAN_POINT('Ctrl Pts',(12.2580206829302,15.0738254766371,-336.143499193805)) ;
#32176=CARTESIAN_POINT('Ctrl Pts',(11.9393258814595,15.3222406935615,-336.138647606194)) ;
#32177=CARTESIAN_POINT('Ctrl Pts',(11.6210960903992,15.5702934456405,-336.133803097577)) ;
#32178=CARTESIAN_POINT('Ctrl Pts',(11.2951611748144,15.8084441224461,-336.129009278458)) ;
#32179=CARTESIAN_POINT('Ctrl Pts',(10.9621519526002,16.0362112462496,-336.124231585018)) ;
#32180=CARTESIAN_POINT('Ctrl Pts',(10.6284128203053,16.2644776040341,-336.119443419536)) ;
#32181=CARTESIAN_POINT('Ctrl Pts',(10.2875682265132,16.4823147300163,-336.11467133811)) ;
#32182=CARTESIAN_POINT('Ctrl Pts',(9.94028083639845,16.6892675465024,-336.109858962474)) ;
#32183=CARTESIAN_POINT('Ctrl Pts',(9.59299344628393,16.8962203629883,-336.105046586837)) ;
#32184=CARTESIAN_POINT('Ctrl Pts',(9.23926314635195,17.0922886968174,-336.100193731212)) ;
#32185=CARTESIAN_POINT('Ctrl Pts',(8.87978193223753,17.2770491112091,-336.095224696288)) ;
#32186=CARTESIAN_POINT('Ctrl Pts',(8.52079145992081,17.4615573019675,-336.090262444786)) ;
#32187=CARTESIAN_POINT('Ctrl Pts',(8.155971937366,17.6348361085319,-336.085183409269)) ;
#32188=CARTESIAN_POINT('Ctrl Pts',(7.78606616485268,17.7965722509237,-336.080064046666)) ;
#32189=CARTESIAN_POINT('Ctrl Pts',(7.41644058646154,17.9581858823417,-336.074948561848)) ;
#32190=CARTESIAN_POINT('Ctrl Pts',(7.04173651286741,18.1082745168596,-336.069792977324)) ;
#32191=CARTESIAN_POINT('Ctrl Pts',(6.66270364660427,18.2465666337444,-336.064653721431)) ;
#32192=CARTESIAN_POINT('Ctrl Pts',(6.28371145642438,18.3848439097482,-336.05951501706)) ;
#32193=CARTESIAN_POINT('Ctrl Pts',(5.90039140878735,18.5113273231904,-336.054392741465)) ;
#32194=CARTESIAN_POINT('Ctrl Pts',(5.51350113652929,18.6257841695783,-336.049321427717)) ;
#32195=CARTESIAN_POINT('Ctrl Pts',(5.12663437653233,18.7402340601459,-336.044250422164)) ;
#32196=CARTESIAN_POINT('Ctrl Pts',(4.73619780293921,18.8426589067191,-336.039230418426)) ;
#32197=CARTESIAN_POINT('Ctrl Pts',(4.34295722055786,18.932863388036,-336.034272949234)) ;
#32198=CARTESIAN_POINT('Ctrl Pts',(3.94910169708311,19.0232089291642,-336.029307727659)) ;
#32199=CARTESIAN_POINT('Ctrl Pts',(3.55243334612323,19.1012958438172,-336.024405234849)) ;
#32200=CARTESIAN_POINT('Ctrl Pts',(3.15373040943338,19.1669649899548,-336.019553647204)) ;
#32201=CARTESIAN_POINT('Ctrl Pts',(2.7556091460887,19.2325383304475,-336.014709137609)) ;
#32202=CARTESIAN_POINT('Ctrl Pts',(2.35545918607513,19.2857300515833,-336.009915317477)) ;
#32203=CARTESIAN_POINT('Ctrl Pts',(1.95406481959108,19.3264191526301,-336.005137623011)) ;
#32204=CARTESIAN_POINT('Ctrl Pts',(1.55179076985886,19.3671974266288,-336.0003494579)) ;
#32205=CARTESIAN_POINT('Ctrl Pts',(1.14826681025661,19.3954180707545,-335.995577376822)) ;
#32206=CARTESIAN_POINT('Ctrl Pts',(0.744292565869232,19.410998503486,-335.99076500158)) ;
#32207=CARTESIAN_POINT('Ctrl Pts',(0.340318321481302,19.4265789362175,-335.985952626338)) ;
#32208=CARTESIAN_POINT('Ctrl Pts',(-0.0641062245104881,19.4295189511988,
-335.981099771155)) ;
#32209=CARTESIAN_POINT('Ctrl Pts',(-0.468170828899835,19.4197777840626,
-335.97613073681)) ;
#32210=CARTESIAN_POINT('Ctrl Pts',(-0.87168390175727,19.4100499132182,-335.971168484991)) ;
#32211=CARTESIAN_POINT('Ctrl Pts',(-1.27494321941302,19.3876724375374,-335.966089449256)) ;
#32212=CARTESIAN_POINT('Ctrl Pts',(-1.67714662679196,19.3527256306513,-335.96097008652)) ;
#32213=CARTESIAN_POINT('Ctrl Pts',(-2.07904536333704,19.3178052961238,-335.955854601725)) ;
#32214=CARTESIAN_POINT('Ctrl Pts',(-2.47988983244948,19.2703348553497,-335.950699017313)) ;
#32215=CARTESIAN_POINT('Ctrl Pts',(-2.87889179669617,19.210434554152,-335.945559761603)) ;
#32216=CARTESIAN_POINT('Ctrl Pts',(-3.27785094179539,19.150540681193,-335.940421057416)) ;
#32217=CARTESIAN_POINT('Ctrl Pts',(-3.6749680310441,19.0782197267368,-335.935298782076)) ;
#32218=CARTESIAN_POINT('Ctrl Pts',(-4.0694664338171,18.9936298163128,-335.930227468632)) ;
#32219=CARTESIAN_POINT('Ctrl Pts',(-4.46394086191889,18.9090450466327,-335.925156463386)) ;
#32220=CARTESIAN_POINT('Ctrl Pts',(-4.85579697128176,18.8121928550736,-335.920136460004)) ;
#32221=CARTESIAN_POINT('Ctrl Pts',(-5.24426884028382,18.7032681041243,-335.9151789912)) ;
#32222=CARTESIAN_POINT('Ctrl Pts',(-5.63334821378748,18.5941730132306,-335.91021376975)) ;
#32223=CARTESIAN_POINT('Ctrl Pts',(-6.01903278542061,18.4729675443096,-335.905311277103)) ;
#32224=CARTESIAN_POINT('Ctrl Pts',(-6.40056302122172,18.339884280041,-335.900459689639)) ;
#32225=CARTESIAN_POINT('Ctrl Pts',(-6.78153661699106,18.2069951798661,-335.895615180481)) ;
#32226=CARTESIAN_POINT('Ctrl Pts',(-7.1583680006544,18.0622628466857,-335.890821360796)) ;
#32227=CARTESIAN_POINT('Ctrl Pts',(-7.53031057479022,17.9059562498481,-335.88604366677)) ;
#32228=CARTESIAN_POINT('Ctrl Pts',(-7.90306831615217,17.7493070839586,-335.88125550172)) ;
#32229=CARTESIAN_POINT('Ctrl Pts',(-8.27091576187639,17.5810327139357,-335.876483420698)) ;
#32230=CARTESIAN_POINT('Ctrl Pts',(-8.63311122904986,17.4014431828012,-335.871671045477)) ;
#32231=CARTESIAN_POINT('Ctrl Pts',(-8.99530669622332,17.2218536516666,-335.866858670257)) ;
#32232=CARTESIAN_POINT('Ctrl Pts',(-9.35185010088917,17.030948770167,-335.862005815059)) ;
#32233=CARTESIAN_POINT('Ctrl Pts',(-9.70201044240801,16.8290803821525,-335.85703678063)) ;
#32234=CARTESIAN_POINT('Ctrl Pts',(-10.0516928123364,16.6274875460583,-335.852074528972)) ;
#32235=CARTESIAN_POINT('Ctrl Pts',(-10.3951004725014,16.4149081312252,-335.846995493338)) ;
#32236=CARTESIAN_POINT('Ctrl Pts',(-10.7315674323518,16.1917963988285,-335.841876130656)) ;
#32237=CARTESIAN_POINT('Ctrl Pts',(-11.0677795169522,15.9688536745822,-335.836760645915)) ;
#32238=CARTESIAN_POINT('Ctrl Pts',(-11.3970615415595,15.7353947287877,-335.831605061509)) ;
#32239=CARTESIAN_POINT('Ctrl Pts',(-11.7187788607783,15.4919022648105,-335.826465805769)) ;
#32240=CARTESIAN_POINT('Ctrl Pts',(-12.0404616546875,15.2484359313901,-335.821327101552)) ;
#32241=CARTESIAN_POINT('Ctrl Pts',(-12.3545814670092,14.9949383052232,-335.816204826145)) ;
#32242=CARTESIAN_POINT('Ctrl Pts',(-12.6605319671979,14.7319197999514,-335.81113351261)) ;
#32243=CARTESIAN_POINT('Ctrl Pts',(-12.9664638739843,14.4689172789937,-335.806062507272)) ;
#32244=CARTESIAN_POINT('Ctrl Pts',(-13.264227525505,14.1963950501257,-335.801042503775)) ;
#32245=CARTESIAN_POINT('Ctrl Pts',(-13.553243570959,13.9148906633192,-335.796085034843)) ;
#32246=CARTESIAN_POINT('Ctrl Pts',(-13.8427115888996,13.6329460509969,-335.791119813262)) ;
#32247=CARTESIAN_POINT('Ctrl Pts',(-14.1234046330415,13.3419911239812,-335.786217320472)) ;
#32248=CARTESIAN_POINT('Ctrl Pts',(-14.3947670080328,13.0425934994147,-335.781365732863)) ;
#32249=CARTESIAN_POINT('Ctrl Pts',(-14.6657334741274,12.7436326862641,-335.776521223562)) ;
#32250=CARTESIAN_POINT('Ctrl Pts',(-14.9273964527425,12.4362537254702,-335.771727403734)) ;
#32251=CARTESIAN_POINT('Ctrl Pts',(-15.179229016747,12.121049997195,-335.766949709574)) ;
#32252=CARTESIAN_POINT('Ctrl Pts',(-15.4316135093015,11.8051554530303,-335.762161544386)) ;
#32253=CARTESIAN_POINT('Ctrl Pts',(-15.6741243484905,11.4814016885572,-335.757389463236)) ;
#32254=CARTESIAN_POINT('Ctrl Pts',(-15.9062585734021,11.1504158006893,-335.752577087905)) ;
#32255=CARTESIAN_POINT('Ctrl Pts',(-16.1383927983141,10.819429912821,-335.747764712574)) ;
#32256=CARTESIAN_POINT('Ctrl Pts',(-16.3601502446802,10.4812117755364,-335.742911857287)) ;
#32257=CARTESIAN_POINT('Ctrl Pts',(-16.5710573305373,10.1364200815959,-335.737942822794)) ;
#32258=CARTESIAN_POINT('Ctrl Pts',(-16.7816765264918,9.79209903114648,-335.732980571073)) ;
#32259=CARTESIAN_POINT('Ctrl Pts',(-16.9815294718259,9.44113232479675,-335.727901535404)) ;
#32260=CARTESIAN_POINT('Ctrl Pts',(-17.1702486707563,9.08423748848073,-335.722782172708)) ;
#32261=CARTESIAN_POINT('Ctrl Pts',(-17.358824915386,8.72761299907167,-335.717666687915)) ;
#32262=CARTESIAN_POINT('Ctrl Pts',(-17.5362844577517,8.36506942339514,-335.712511103478)) ;
#32263=CARTESIAN_POINT('Ctrl Pts',(-17.7023009345826,7.99733426701588,-335.707371847721)) ;
#32264=CARTESIAN_POINT('Ctrl Pts',(-17.8682995952563,7.62963857435403,-335.702233143487)) ;
#32265=CARTESIAN_POINT('Ctrl Pts',(-18.0228577688157,7.25675243049972,-335.697110868077)) ;
#32266=CARTESIAN_POINT('Ctrl Pts',(-18.1656872133452,6.87941412769221,-335.692039554548)) ;
#32267=CARTESIAN_POINT('Ctrl Pts',(-18.308507977769,6.50209875668508,-335.686968549216)) ;
#32268=CARTESIAN_POINT('Ctrl Pts',(-18.4396015015549,6.12033174955262,-335.681948545734)) ;
#32269=CARTESIAN_POINT('Ctrl Pts',(-18.5587162171598,5.73486231995589,-335.67699107682)) ;
#32270=CARTESIAN_POINT('Ctrl Pts',(-18.6780172066311,5.34879008590577,-335.672025855321)) ;
#32271=CARTESIAN_POINT('Ctrl Pts',(-18.7853018849544,4.95900379762273,-335.667123362615)) ;
#32272=CARTESIAN_POINT('Ctrl Pts',(-18.8803538419933,4.56626775423995,-335.662271775086)) ;
#32273=CARTESIAN_POINT('Ctrl Pts',(-18.9752671225249,4.17410469498566,-335.657427265805)) ;
#32274=CARTESIAN_POINT('Ctrl Pts',(-19.0579832957413,3.77900043415976,-335.652633445994)) ;
#32275=CARTESIAN_POINT('Ctrl Pts',(-19.1283235393561,3.38172813075498,-335.647855751845)) ;
#32276=CARTESIAN_POINT('Ctrl Pts',(-19.1988179427352,2.98358515358625,-335.64306758676)) ;
#32277=CARTESIAN_POINT('Ctrl Pts',(-19.2568819647207,2.58326456638056,-335.638295505705)) ;
#32278=CARTESIAN_POINT('Ctrl Pts',(-19.3023739593782,2.18155766970835,-335.633483130463)) ;
#32279=CARTESIAN_POINT('Ctrl Pts',(-19.3478659540356,1.77985077303668,-335.62867075522)) ;
#32280=CARTESIAN_POINT('Ctrl Pts',(-19.3807857168242,1.37675753482452,-335.623817900012)) ;
#32281=CARTESIAN_POINT('Ctrl Pts',(-19.4010325165295,0.973082945256434,
-335.618848865593)) ;
#32282=CARTESIAN_POINT('Ctrl Pts',(-19.4212516794254,0.569959370063551,
-335.613886613888)) ;
#32283=CARTESIAN_POINT('Ctrl Pts',(-19.4288372442096,0.166150890841973,
-335.608807578225)) ;
#32284=CARTESIAN_POINT('Ctrl Pts',(-19.4238097842129,-0.237536593306288,
-335.603688215528)) ;
#32285=CARTESIAN_POINT('Ctrl Pts',(-19.4187861325342,-0.640918282809963,
-335.598572730766)) ;
#32286=CARTESIAN_POINT('Ctrl Pts',(-19.4011687499022,-1.04417919004252,
-335.593417146355)) ;
#32287=CARTESIAN_POINT('Ctrl Pts',(-19.3710191037869,-1.44652433131471,
-335.588277890619)) ;
#32288=CARTESIAN_POINT('Ctrl Pts',(-19.3408726932006,-1.84882629465552,
-335.583139186406)) ;
#32289=CARTESIAN_POINT('Ctrl Pts',(-19.298196823703,-2.25021273376001,-335.578016911014)) ;
#32290=CARTESIAN_POINT('Ctrl Pts',(-19.2430915988317,-2.64989743103697,
-335.572945597502)) ;
#32291=CARTESIAN_POINT('Ctrl Pts',(-19.1879897228463,-3.04955783844967,
-335.567874592186)) ;
#32292=CARTESIAN_POINT('Ctrl Pts',(-19.1204600486215,-3.44751675700766,
-335.562854588718)) ;
#32293=CARTESIAN_POINT('Ctrl Pts',(-19.0406401095888,-3.84299592462276,
-335.557897119818)) ;
#32294=CARTESIAN_POINT('Ctrl Pts',(-18.9606953457586,-4.23909355433633,
-335.552931898281)) ;
#32295=CARTESIAN_POINT('Ctrl Pts',(-18.8684218195035,-4.63270370490894,
-335.548029405537)) ;
#32296=CARTESIAN_POINT('Ctrl Pts',(-18.763995154248,-5.02305168740151,-335.543177817974)) ;
#32297=CARTESIAN_POINT('Ctrl Pts',(-18.6597208438918,-5.41283016566436,
-335.538333308709)) ;
#32298=CARTESIAN_POINT('Ctrl Pts',(-18.5433287606616,-5.79935600341102,
-335.533539488917)) ;
#32299=CARTESIAN_POINT('Ctrl Pts',(-18.4150317737214,-6.18186471457878,
-335.52876179479)) ;
#32300=CARTESIAN_POINT('Ctrl Pts',(-18.2864536052352,-6.56521174933737,
-335.52397362965)) ;
#32301=CARTESIAN_POINT('Ctrl Pts',(-18.1459181396667,-6.9445240077796,-335.519201548544)) ;
#32302=CARTESIAN_POINT('Ctrl Pts',(-17.993679571189,-7.31903885923887,-335.514389173252)) ;
#32303=CARTESIAN_POINT('Ctrl Pts',(-17.8414410027114,-7.69355371069813,
-335.50957679796)) ;
#32304=CARTESIAN_POINT('Ctrl Pts',(-17.6774991363662,-8.0632710854823,-335.504723942706)) ;
#32305=CARTESIAN_POINT('Ctrl Pts',(-17.5021506441656,-8.42743590628459,
-335.499754908239)) ;
#32306=CARTESIAN_POINT('Ctrl Pts',(-17.3270415037638,-8.79110363980762,
-335.494792656536)) ;
#32307=CARTESIAN_POINT('Ctrl Pts',(-17.1405107631171,-9.14932858519802,
-335.489713620875)) ;
#32308=CARTESIAN_POINT('Ctrl Pts',(-16.9429620500801,-9.50141290208948,
-335.484594258182)) ;
#32309=CARTESIAN_POINT('Ctrl Pts',(-16.7455629801875,-9.85323051512083,
-335.479478773406)) ;
#32310=CARTESIAN_POINT('Ctrl Pts',(-16.5371627784836,-10.1989169171179,
-335.47432318898)) ;
#32311=CARTESIAN_POINT('Ctrl Pts',(-16.3181957609453,-10.5378034176016,
-335.469183933231)) ;
#32312=CARTESIAN_POINT('Ctrl Pts',(-16.0992522419896,-10.8766535502684,
-335.464045229003)) ;
#32313=CARTESIAN_POINT('Ctrl Pts',(-15.8697442543277,-11.2087053354623,
-335.458922953597)) ;
#32314=CARTESIAN_POINT('Ctrl Pts',(-15.630135847461,-11.5333162649052,-335.453851640069)) ;
#32315=CARTESIAN_POINT('Ctrl Pts',(-15.3905420022053,-11.857907466918,-335.448780634739)) ;
#32316=CARTESIAN_POINT('Ctrl Pts',(-15.1408489840806,-12.1750587802935,
-335.443760631255)) ;
#32317=CARTESIAN_POINT('Ctrl Pts',(-14.8815499047474,-12.4841525900853,
-335.438803162339)) ;
#32318=CARTESIAN_POINT('Ctrl Pts',(-14.6218453273732,-12.7937297680969,
-335.433837940815)) ;
#32319=CARTESIAN_POINT('Ctrl Pts',(-14.3525045804028,-13.095224238069,-335.428935448083)) ;
#32320=CARTESIAN_POINT('Ctrl Pts',(-14.0740525139215,-13.3880397459356,
-335.424083860531)) ;
#32321=CARTESIAN_POINT('Ctrl Pts',(-13.7960066976958,-13.6804280478692,
-335.419239351247)) ;
#32322=CARTESIAN_POINT('Ctrl Pts',(-13.5088760596408,-13.9641626740379,
-335.414445531436)) ;
#32323=CARTESIAN_POINT('Ctrl Pts',(-13.2132132751,-14.2386741490737,-335.409667837287)) ;
#32324=CARTESIAN_POINT('Ctrl Pts',(-12.9169025051837,-14.5137872535012,
-335.40487967217)) ;
#32325=CARTESIAN_POINT('Ctrl Pts',(-12.6120220248791,-14.7796366419539,
-335.400107591085)) ;
#32326=CARTESIAN_POINT('Ctrl Pts',(-12.2991599105236,-15.0356742392506,
-335.395295215814)) ;
#32327=CARTESIAN_POINT('Ctrl Pts',(-11.9862977961685,-15.291711836547,-335.390482840544)) ;
#32328=CARTESIAN_POINT('Ctrl Pts',(-11.6654539099066,-15.5379374882154,
-335.38562998531)) ;
#32329=CARTESIAN_POINT('Ctrl Pts',(-11.3372500153741,-15.7738300743316,
-335.380660950867)) ;
#32330=CARTESIAN_POINT('Ctrl Pts',(-11.0094941193816,-16.0094006669069,
-335.375698699158)) ;
#32331=CARTESIAN_POINT('Ctrl Pts',(-10.6743125509312,-16.2347274182438,
-335.370619663494)) ;
#32332=CARTESIAN_POINT('Ctrl Pts',(-10.3323936111183,-16.4493906400966,
-335.365500300798)) ;
#32333=CARTESIAN_POINT('Ctrl Pts',(-9.99073367541036,-16.6638912542399,
-335.360384816027)) ;
#32334=CARTESIAN_POINT('Ctrl Pts',(-9.64234665101162,-16.8677446656216,
-335.355229231607)) ;
#32335=CARTESIAN_POINT('Ctrl Pts',(-9.28793384112007,-17.0605714652986,
-335.350089975865)) ;
#32336=CARTESIAN_POINT('Ctrl Pts',(-8.93355906526314,-17.2533775716457,
-335.344951271644)) ;
#32337=CARTESIAN_POINT('Ctrl Pts',(-8.57315982150312,-17.4351595538585,
-335.339828996246)) ;
#32338=CARTESIAN_POINT('Ctrl Pts',(-8.20745099669403,-17.6055752195817,
-335.334757682728)) ;
#32339=CARTESIAN_POINT('Ctrl Pts',(-7.84176439694247,-17.7759805287106,
-335.329686677406)) ;
#32340=CARTESIAN_POINT('Ctrl Pts',(-7.47076884789392,-17.9350209668775,
-335.324666673932)) ;
#32341=CARTESIAN_POINT('Ctrl Pts',(-7.0951928471428,-18.0823901053232,-335.319709205027)) ;
#32342=CARTESIAN_POINT('Ctrl Pts',(-6.71902951074151,-18.2299897035123,
-335.3147439835)) ;
#32343=CARTESIAN_POINT('Ctrl Pts',(-6.33827134199943,-18.3658814645726,
-335.309841490767)) ;
#32344=CARTESIAN_POINT('Ctrl Pts',(-5.95366448937237,-18.4897929017834,
-335.304989903213)) ;
#32345=CARTESIAN_POINT('Ctrl Pts',(-5.56961876354971,-18.613523556909,-335.300145393942)) ;
#32346=CARTESIAN_POINT('Ctrl Pts',(-5.18173552463438,-18.725308770049,-335.295351574143)) ;
#32347=CARTESIAN_POINT('Ctrl Pts',(-4.79077254364982,-18.8249128819126,
-335.290573880007)) ;
#32348=CARTESIAN_POINT('Ctrl Pts',(-4.39895271232139,-18.9247352901921,
-335.285785714883)) ;
#32349=CARTESIAN_POINT('Ctrl Pts',(-4.00403956016823,-19.0123230044549,
-335.281013633792)) ;
#32350=CARTESIAN_POINT('Ctrl Pts',(-3.60681170648216,-19.0874760942272,
-335.276201258515)) ;
#32351=CARTESIAN_POINT('Ctrl Pts',(-3.20958385279609,-19.1626291839994,
-335.271388883238)) ;
#32352=CARTESIAN_POINT('Ctrl Pts',(-2.81004125042442,-19.2253474476804,
-335.266536027998)) ;
#32353=CARTESIAN_POINT('Ctrl Pts',(-2.40897920439023,-19.2754707418096,
-335.261566993546)) ;
#32354=CARTESIAN_POINT('Ctrl Pts',(-1.98818862475481,-19.3280596372146,
-335.256353528677)) ;
#32355=CARTESIAN_POINT('Ctrl Pts',(-1.5656546785899,-19.3667931000231,-335.251011760576)) ;
#32356=CARTESIAN_POINT('Ctrl Pts',(-1.14226732751046,-19.3916351229619,
-335.24562939536)) ;
#32357=CARTESIAN_POINT('Ctrl Pts',(-0.762155209100447,-19.4139379951208,
-335.240797172009)) ;
#32358=CARTESIAN_POINT('Ctrl Pts',(-0.381355021190701,-19.4250447171769,
-335.235932049976)) ;
#32359=CARTESIAN_POINT('Ctrl Pts',(-0.000505252659192643,-19.4249560735629,
-335.231080776623)) ;
#32360=CARTESIAN_POINT('Ctrl Pts',(-0.000488272271658846,-19.4249999938633,
-335.018634132822)) ;
#32361=CARTESIAN_POINT('Ctrl Pts',(-0.468717606056336,-19.4249882243189,
-335.024104372837)) ;
#32362=CARTESIAN_POINT('Ctrl Pts',(-0.936792336862977,-19.4080468254062,
-335.029582516708)) ;
#32363=CARTESIAN_POINT('Ctrl Pts',(-1.48555256655971,-19.3682853646297,
-335.036195527655)) ;
#32364=CARTESIAN_POINT('Ctrl Pts',(-1.5672717674808,-19.3618440129123,-335.037185408023)) ;
#32365=CARTESIAN_POINT('Ctrl Pts',(-1.71125369797793,-19.3495774113658,
-335.038940172386)) ;
#32366=CARTESIAN_POINT('Ctrl Pts',(-1.77353368560344,-19.343968400327,-335.039702732533)) ;
#32367=CARTESIAN_POINT('Ctrl Pts',(-1.90166063482093,-19.3318051530813,
-335.041279704335)) ;
#32368=CARTESIAN_POINT('Ctrl Pts',(-1.96750318988438,-19.325215000439,-335.042094685323)) ;
#32369=CARTESIAN_POINT('Ctrl Pts',(-2.12867204830871,-19.3082514698797,
-335.044100366175)) ;
#32370=CARTESIAN_POINT('Ctrl Pts',(-2.22395759981224,-19.2975084420849,
-335.045295244128)) ;
#32371=CARTESIAN_POINT('Ctrl Pts',(-2.60634702361314,-19.2515258990493,
-335.050121609932)) ;
#32372=CARTESIAN_POINT('Ctrl Pts',(-2.89272684723886,-19.2105810705904,
-335.053806452374)) ;
#32373=CARTESIAN_POINT('Ctrl Pts',(-3.35022309201495,-19.1347086954307,
-335.059754882247)) ;
#32374=CARTESIAN_POINT('Ctrl Pts',(-3.52196899990878,-19.1038427008835,
-335.062002161339)) ;
#32375=CARTESIAN_POINT('Ctrl Pts',(-4.17682254465237,-18.9770220388341,
-335.070603310764)) ;
#32376=CARTESIAN_POINT('Ctrl Pts',(-4.65663385048137,-18.8650198705459,
-335.076968430991)) ;
#32377=CARTESIAN_POINT('Ctrl Pts',(-5.42240760696615,-18.6552671305497,
-335.087090322891)) ;
#32378=CARTESIAN_POINT('Ctrl Pts',(-5.71125364216025,-18.5688739131451,
-335.090900874196)) ;
#32379=CARTESIAN_POINT('Ctrl Pts',(-6.08250417820151,-18.4483513254985,
-335.095779205614)) ;
#32380=CARTESIAN_POINT('Ctrl Pts',(-6.16684668136298,-18.420329142885,-335.096886244625)) ;
#32381=CARTESIAN_POINT('Ctrl Pts',(-6.36106680269313,-18.3543174701958,
-335.099432528422)) ;
#32382=CARTESIAN_POINT('Ctrl Pts',(-6.47080165456166,-18.3159183949568,
-335.100868981337)) ;
#32383=CARTESIAN_POINT('Ctrl Pts',(-6.69896362834188,-18.2337721932833,
-335.103851292836)) ;
#32384=CARTESIAN_POINT('Ctrl Pts',(-6.81732237804154,-18.1898509541121,
-335.105395876785)) ;
#32385=CARTESIAN_POINT('Ctrl Pts',(-7.07939981786079,-18.0896804776572,
-335.108811394339)) ;
#32386=CARTESIAN_POINT('Ctrl Pts',(-7.22289336033244,-18.0328659162564,
-335.110678349121)) ;
#32387=CARTESIAN_POINT('Ctrl Pts',(-7.81827949264123,-17.7888830666712,
-335.118417418889)) ;
#32388=CARTESIAN_POINT('Ctrl Pts',(-8.26369844989171,-17.5863908843134,
-335.124184558792)) ;
#32389=CARTESIAN_POINT('Ctrl Pts',(-8.8406215197942,-17.2973530790208,-335.131738439332)) ;
#32390=CARTESIAN_POINT('Ctrl Pts',(-8.97939500145368,-17.2257214019571,
-335.133562562827)) ;
#32391=CARTESIAN_POINT('Ctrl Pts',(-9.44631434337654,-16.9775326429109,
-335.139738403987)) ;
#32392=CARTESIAN_POINT('Ctrl Pts',(-9.77023828626849,-16.7932103081035,
-335.144086463682)) ;
#32393=CARTESIAN_POINT('Ctrl Pts',(-10.2651110727269,-16.4924454046484,
-335.150939897255)) ;
#32394=CARTESIAN_POINT('Ctrl Pts',(-10.4398413964372,-16.3823982406034,
-335.153402423781)) ;
#32395=CARTESIAN_POINT('Ctrl Pts',(-10.6836412791606,-16.2233655941138,
-335.156919690524)) ;
#32396=CARTESIAN_POINT('Ctrl Pts',(-10.7541961257338,-16.1766822261781,
-335.15794737896)) ;
#32397=CARTESIAN_POINT('Ctrl Pts',(-10.8268721074768,-16.1279097815406,
-335.15901726738)) ;
#32398=CARTESIAN_POINT('Ctrl Pts',(-10.8293001636972,-16.1262795311789,
-335.15905302476)) ;
#32399=CARTESIAN_POINT('Ctrl Pts',(-10.8327514110086,-16.1239611568537,
-335.159103869138)) ;
#32400=CARTESIAN_POINT('Ctrl Pts',(-10.8337749049054,-16.1232734837029,
-335.159118949769)) ;
#32401=CARTESIAN_POINT('Ctrl Pts',(-10.8367519506596,-16.1212728312673,
-335.159162821756)) ;
#32402=CARTESIAN_POINT('Ctrl Pts',(-10.8387053293361,-16.1199595943694,
-335.159191616757)) ;
#32403=CARTESIAN_POINT('Ctrl Pts',(-10.8443435223978,-16.1161676055536,
-335.159274754806)) ;
#32404=CARTESIAN_POINT('Ctrl Pts',(-10.8480277253574,-16.1136879450963,
-335.159329110773)) ;
#32405=CARTESIAN_POINT('Ctrl Pts',(-10.8548335498523,-16.1091038788023,
-335.159429579171)) ;
#32406=CARTESIAN_POINT('Ctrl Pts',(-10.8579554106576,-16.1069998284352,
-335.159475686502)) ;
#32407=CARTESIAN_POINT('Ctrl Pts',(-10.898833902465,-16.0794315371296,-335.160079718477)) ;
#32408=CARTESIAN_POINT('Ctrl Pts',(-10.9365013771734,-16.0538355732736,
-335.160639585098)) ;
#32409=CARTESIAN_POINT('Ctrl Pts',(-11.0408883486838,-15.9823642010369,
-335.162200311732)) ;
#32410=CARTESIAN_POINT('Ctrl Pts',(-11.1074114268968,-15.9362038250601,
-335.163205262736)) ;
#32411=CARTESIAN_POINT('Ctrl Pts',(-11.3203373948191,-15.7864735229052,
-335.166452672252)) ;
#32412=CARTESIAN_POINT('Ctrl Pts',(-11.4655951856702,-15.6812917796276,
-335.168715156102)) ;
#32413=CARTESIAN_POINT('Ctrl Pts',(-12.1000046014807,-15.2083854496675,
-335.178770583222)) ;
#32414=CARTESIAN_POINT('Ctrl Pts',(-12.5730774465558,-14.8196769065436,
-335.186721695118)) ;
#32415=CARTESIAN_POINT('Ctrl Pts',(-13.2616118452136,-14.1971933068906,
-335.198657295305)) ;
#32416=CARTESIAN_POINT('Ctrl Pts',(-13.4909975254565,-13.9794003034446,
-335.20270268335)) ;
#32417=CARTESIAN_POINT('Ctrl Pts',(-13.8378959456707,-13.6335393509121,
-335.208905543823)) ;
#32418=CARTESIAN_POINT('Ctrl Pts',(-13.9591798504278,-13.5093322357607,
-335.211091352377)) ;
#32419=CARTESIAN_POINT('Ctrl Pts',(-14.0857776466956,-13.3761577503329,
-335.213390126188)) ;
#32420=CARTESIAN_POINT('Ctrl Pts',(-14.0927668114792,-13.3687939497635,
-335.213517092702)) ;
#32421=CARTESIAN_POINT('Ctrl Pts',(-14.1059375361512,-13.3548954372635,
-335.21375646134)) ;
#32422=CARTESIAN_POINT('Ctrl Pts',(-14.1121203362033,-13.3483619043902,
-335.213868873829)) ;
#32423=CARTESIAN_POINT('Ctrl Pts',(-14.1238252084541,-13.3359758258083,
-335.21408176994)) ;
#32424=CARTESIAN_POINT('Ctrl Pts',(-14.1293481867567,-13.3301241390663,
-335.214182261163)) ;
#32425=CARTESIAN_POINT('Ctrl Pts',(-14.1398512429717,-13.3189821163414,
-335.214373433112)) ;
#32426=CARTESIAN_POINT('Ctrl Pts',(-14.1448319917629,-13.3136924147134,
-335.214464119482)) ;
#32427=CARTESIAN_POINT('Ctrl Pts',(-14.1543459035586,-13.3035769956617,
-335.21463739826)) ;
#32428=CARTESIAN_POINT('Ctrl Pts',(-14.1588795693581,-13.2987517526085,
-335.214719994908)) ;
#32429=CARTESIAN_POINT('Ctrl Pts',(-14.1675771576496,-13.2894853002144,
-335.214878498247)) ;
#32430=CARTESIAN_POINT('Ctrl Pts',(-14.1717414610177,-13.2850444494795,
-335.214954408157)) ;
#32431=CARTESIAN_POINT('Ctrl Pts',(-14.1797645855679,-13.276480451863,-335.215100698681)) ;
#32432=CARTESIAN_POINT('Ctrl Pts',(-14.1836236977655,-13.2723575784792,
-335.215171081759)) ;
#32433=CARTESIAN_POINT('Ctrl Pts',(-14.1910901372963,-13.2643738500591,
-335.215307289755)) ;
#32434=CARTESIAN_POINT('Ctrl Pts',(-14.194697688281,-13.2605132048995,-335.215373116568)) ;
#32435=CARTESIAN_POINT('Ctrl Pts',(-14.2017064989729,-13.2530065411227,
-335.215501035847)) ;
#32436=CARTESIAN_POINT('Ctrl Pts',(-14.2051079309394,-13.2493606839114,
-335.215563129774)) ;
#32437=CARTESIAN_POINT('Ctrl Pts',(-14.2117436624687,-13.2422426193297,
-335.215684293282)) ;
#32438=CARTESIAN_POINT('Ctrl Pts',(-14.2149780942441,-13.2387705357059,
-335.215743363987)) ;
#32439=CARTESIAN_POINT('Ctrl Pts',(-14.2213141558534,-13.2319639290496,
-335.215859104308)) ;
#32440=CARTESIAN_POINT('Ctrl Pts',(-14.2244158859593,-13.2286294997788,
-335.215915774778)) ;
#32441=CARTESIAN_POINT('Ctrl Pts',(-14.2305172902006,-13.2220657266557,
-335.216027273568)) ;
#32442=CARTESIAN_POINT('Ctrl Pts',(-14.2335170383797,-13.2188364520051,
-335.216082102518)) ;
#32443=CARTESIAN_POINT('Ctrl Pts',(-14.2394427023473,-13.2124530287226,
-335.21619043207)) ;
#32444=CARTESIAN_POINT('Ctrl Pts',(-14.2423686698649,-13.2092989284551,
-335.216243933112)) ;
#32445=CARTESIAN_POINT('Ctrl Pts',(-14.2481734218118,-13.2030374189185,
-335.216350092709)) ;
#32446=CARTESIAN_POINT('Ctrl Pts',(-14.2510522381442,-13.1999300395523,
-335.216402751533)) ;
#32447=CARTESIAN_POINT('Ctrl Pts',(-14.256788659448,-13.1937341122544,-335.216507700916)) ;
#32448=CARTESIAN_POINT('Ctrl Pts',(-14.2596462762036,-13.1906455786874,
-335.216559991557)) ;
#32449=CARTESIAN_POINT('Ctrl Pts',(-14.3441951202398,-13.0992049719767,
-335.218107413801)) ;
#32450=CARTESIAN_POINT('Ctrl Pts',(-14.4250646849292,-13.0100965954714,
-335.21959547102)) ;
#32451=CARTESIAN_POINT('Ctrl Pts',(-14.5892261258045,-12.8257983287526,
-335.222632888508)) ;
#32452=CARTESIAN_POINT('Ctrl Pts',(-14.6724267779877,-12.7305347182748,
-335.224181422136)) ;
#32453=CARTESIAN_POINT('Ctrl Pts',(-14.8701579558119,-12.4996217037103,
-335.227884708995)) ;
#32454=CARTESIAN_POINT('Ctrl Pts',(-14.9837708873418,-12.3632014659998,
-335.230031661985)) ;
#32455=CARTESIAN_POINT('Ctrl Pts',(-15.5607946918287,-11.6507034236138,
-335.241046953763)) ;
#32456=CARTESIAN_POINT('Ctrl Pts',(-15.9929117975076,-11.0500676134274,
-335.249649783577)) ;
#32457=CARTESIAN_POINT('Ctrl Pts',(-16.6075928916345,-10.083809877613,-335.263037228399)) ;
#32458=CARTESIAN_POINT('Ctrl Pts',(-16.8146593927414,-9.7346079187652,-335.267796674189)) ;
#32459=CARTESIAN_POINT('Ctrl Pts',(-17.068262448583,-9.27465833767664,-335.274095118541)) ;
#32460=CARTESIAN_POINT('Ctrl Pts',(-17.1249266482483,-9.16961054373564,
-335.275535733547)) ;
#32461=CARTESIAN_POINT('Ctrl Pts',(-17.2133087105605,-9.00208510118727,
-335.277841203368)) ;
#32462=CARTESIAN_POINT('Ctrl Pts',(-17.245662926587,-8.93994648477509,-335.278698091801)) ;
#32463=CARTESIAN_POINT('Ctrl Pts',(-17.3063456584251,-8.82184555696794,
-335.280331171837)) ;
#32464=CARTESIAN_POINT('Ctrl Pts',(-17.3347406502135,-8.76591841501513,
-335.281106378047)) ;
#32465=CARTESIAN_POINT('Ctrl Pts',(-17.4152014752633,-8.60552189644457,
-335.283333830865)) ;
#32466=CARTESIAN_POINT('Ctrl Pts',(-17.466597188511,-8.50071950654463,-335.284794295983)) ;
#32467=CARTESIAN_POINT('Ctrl Pts',(-17.6721569060288,-8.07182118795383,
-335.290782144169)) ;
#32468=CARTESIAN_POINT('Ctrl Pts',(-17.8182695260716,-7.74394584960671,
-335.295383716441)) ;
#32469=CARTESIAN_POINT('Ctrl Pts',(-18.159707420861,-6.91685259050838,-335.306907810768)) ;
#32470=CARTESIAN_POINT('Ctrl Pts',(-18.3436135433347,-6.41324156320669,
-335.313846308809)) ;
#32471=CARTESIAN_POINT('Ctrl Pts',(-18.5538387942488,-5.75412902052858,
-335.322675024848)) ;
#32472=CARTESIAN_POINT('Ctrl Pts',(-18.599426835328,-5.60502062960723,-335.324656587289)) ;
#32473=CARTESIAN_POINT('Ctrl Pts',(-18.7068627434282,-5.23786913791506,
-335.329493847755)) ;
#32474=CARTESIAN_POINT('Ctrl Pts',(-18.7666993003637,-5.01926134466978,
-335.332337884868)) ;
#32475=CARTESIAN_POINT('Ctrl Pts',(-18.8560478070511,-4.66886545578968,
-335.336836107212)) ;
#32476=CARTESIAN_POINT('Ctrl Pts',(-18.8880344876731,-4.53773035761718,
-335.338506263097)) ;
#32477=CARTESIAN_POINT('Ctrl Pts',(-18.9473392464463,-4.28310105391946,
-335.341723810595)) ;
#32478=CARTESIAN_POINT('Ctrl Pts',(-18.9748230942038,-4.15965235934368,
-335.343272230829)) ;
#32479=CARTESIAN_POINT('Ctrl Pts',(-19.0379699798092,-3.86235877558695,
-335.346974593721)) ;
#32480=CARTESIAN_POINT('Ctrl Pts',(-19.0724600988067,-3.68827631412663,
-335.349120746758)) ;
#32481=CARTESIAN_POINT('Ctrl Pts',(-19.2383650879695,-2.78623552285682,
-335.360140046453)) ;
#32482=CARTESIAN_POINT('Ctrl Pts',(-19.3305051179945,-2.0516753747047,-335.368747317222)) ;
#32483=CARTESIAN_POINT('Ctrl Pts',(-19.4079650940754,-0.908898808793932,
-335.3821371249)) ;
#32484=CARTESIAN_POINT('Ctrl Pts',(-19.4227137908521,-0.503382222379939,
-335.38689436078)) ;
#32485=CARTESIAN_POINT('Ctrl Pts',(-19.4253544977313,0.021627213401816,
-335.393190249366)) ;
#32486=CARTESIAN_POINT('Ctrl Pts',(-19.4248550878299,0.140960466288975,
-335.394630607076)) ;
#32487=CARTESIAN_POINT('Ctrl Pts',(-19.4223174750438,0.330327465152303,
-335.396935765745)) ;
#32488=CARTESIAN_POINT('Ctrl Pts',(-19.4209999186418,0.400367943033998,
-335.397792603982)) ;
#32489=CARTESIAN_POINT('Ctrl Pts',(-19.4177845371009,0.533107112279973,
-335.39942567836)) ;
#32490=CARTESIAN_POINT('Ctrl Pts',(-19.4159618319896,0.595806722133799,
-335.400200929935)) ;
#32491=CARTESIAN_POINT('Ctrl Pts',(-19.4098779021935,0.775173564898709,
-335.402428681672)) ;
#32492=CARTESIAN_POINT('Ctrl Pts',(-19.4048685757636,0.891812610105692,
-335.403889403669)) ;
#32493=CARTESIAN_POINT('Ctrl Pts',(-19.3801629671762,1.36708007932384,-335.409880992972)) ;
#32494=CARTESIAN_POINT('Ctrl Pts',(-19.3515735088423,1.72517434836294,-335.414486164467)) ;
#32495=CARTESIAN_POINT('Ctrl Pts',(-19.2556494408886,2.61487141692982,-335.426011064085)) ;
#32496=CARTESIAN_POINT('Ctrl Pts',(-19.1762188862869,3.14487184893335,-335.432946655477)) ;
#32497=CARTESIAN_POINT('Ctrl Pts',(-19.0455262681809,3.82398398899898,-335.441772099194)) ;
#32498=CARTESIAN_POINT('Ctrl Pts',(-19.0142262467662,3.97669771167166,-335.443753228237)) ;
#32499=CARTESIAN_POINT('Ctrl Pts',(-18.932925213169,4.35043845825549,-335.44858963212)) ;
#32500=CARTESIAN_POINT('Ctrl Pts',(-18.8808881900747,4.57099916093684,-335.451433247436)) ;
#32501=CARTESIAN_POINT('Ctrl Pts',(-18.7917178537821,4.92140041614273,-335.455930978082)) ;
#32502=CARTESIAN_POINT('Ctrl Pts',(-18.7570690824531,5.05185128919522,-335.457601057752)) ;
#32503=CARTESIAN_POINT('Ctrl Pts',(-18.6873254822222,5.30381807260058,-335.460818559719)) ;
#32504=CARTESIAN_POINT('Ctrl Pts',(-18.6523978254009,5.42537328095011,-335.462367009511)) ;
#32505=CARTESIAN_POINT('Ctrl Pts',(-18.5656095485827,5.71666551737828,-335.466069613333)) ;
#32506=CARTESIAN_POINT('Ctrl Pts',(-18.5126048808818,5.88604988075187,-335.468215974972)) ;
#32507=CARTESIAN_POINT('Ctrl Pts',(-18.2267532672315,6.75744876962215,-335.479234226507)) ;
#32508=CARTESIAN_POINT('Ctrl Pts',(-17.9562710382641,7.44647428341406,-335.487840336432)) ;
#32509=CARTESIAN_POINT('Ctrl Pts',(-17.4775899549772,8.48699573708209,-335.501229527281)) ;
#32510=CARTESIAN_POINT('Ctrl Pts',(-17.2965115328921,8.85019404269283,-335.505987341714)) ;
#32511=CARTESIAN_POINT('Ctrl Pts',(-17.0476270811357,9.31253334822059,-335.512283899406)) ;
#32512=CARTESIAN_POINT('Ctrl Pts',(-16.9900939650053,9.41708943659527,-335.513724324487)) ;
#32513=CARTESIAN_POINT('Ctrl Pts',(-16.8972645931346,9.58216999233022,-335.516029564628)) ;
#32514=CARTESIAN_POINT('Ctrl Pts',(-16.8625980185336,9.64304519079513,-335.516886416007)) ;
#32515=CARTESIAN_POINT('Ctrl Pts',(-16.7962688043851,9.75806915620797,-335.518519491861)) ;
#32516=CARTESIAN_POINT('Ctrl Pts',(-16.7646717087004,9.81225467948012,-335.519294731551)) ;
#32517=CARTESIAN_POINT('Ctrl Pts',(-16.6735190100144,9.96684588149034,-335.521522404988)) ;
#32518=CARTESIAN_POINT('Ctrl Pts',(-16.6133200368016,10.0668689421253,-335.522983059698)) ;
#32519=CARTESIAN_POINT('Ctrl Pts',(-16.3642868687349,10.4723296390465,-335.528973668722)) ;
#32520=CARTESIAN_POINT('Ctrl Pts',(-16.1679021706417,10.7730455960562,-335.533577897087)) ;
#32521=CARTESIAN_POINT('Ctrl Pts',(-15.6580332516087,11.5084162372768,-335.545102585639)) ;
#32522=CARTESIAN_POINT('Ctrl Pts',(-15.3346865724285,11.9358719467092,-335.552038938598)) ;
#32523=CARTESIAN_POINT('Ctrl Pts',(-14.8949776330543,12.4697461248486,-335.560865239719)) ;
#32524=CARTESIAN_POINT('Ctrl Pts',(-14.7944249329524,12.5888807319695,-335.562846482339)) ;
#32525=CARTESIAN_POINT('Ctrl Pts',(-14.5442147919297,12.8781905521565,-335.567683110706)) ;
#32526=CARTESIAN_POINT('Ctrl Pts',(-14.3929925006144,13.0469821398511,-335.570526836563)) ;
#32527=CARTESIAN_POINT('Ctrl Pts',(-14.1470423158832,13.3120259946588,-335.57502469607)) ;
#32528=CARTESIAN_POINT('Ctrl Pts',(-14.0542043784957,13.4100030468764,-335.576694795714)) ;
#32529=CARTESIAN_POINT('Ctrl Pts',(-13.8724130162241,13.5978960415927,-335.579912309609)) ;
#32530=CARTESIAN_POINT('Ctrl Pts',(-13.7835876218738,13.687926503664,-335.58146075165)) ;
#32531=CARTESIAN_POINT('Ctrl Pts',(-13.5680190044615,13.9021933951095,-335.585163292311)) ;
#32532=CARTESIAN_POINT('Ctrl Pts',(-13.4404399625115,14.0255728810238,-335.587309599264)) ;
#32533=CARTESIAN_POINT('Ctrl Pts',(-12.7725118632409,14.6540311459201,-335.598328125349)) ;
#32534=CARTESIAN_POINT('Ctrl Pts',(-12.2053262599333,15.129695942914,-335.606934539384)) ;
#32535=CARTESIAN_POINT('Ctrl Pts',(-11.2871592626856,15.8144007879201,-335.620323891879)) ;
#32536=CARTESIAN_POINT('Ctrl Pts',(-10.9543967132614,16.0466952259967,-335.625081554806)) ;
#32537=CARTESIAN_POINT('Ctrl Pts',(-10.5146619542784,16.3336079936501,-335.63137793728)) ;
#32538=CARTESIAN_POINT('Ctrl Pts',(-10.4141195227223,16.3978956151936,-335.632818344719)) ;
#32539=CARTESIAN_POINT('Ctrl Pts',(-10.2536263069596,16.4984447754482,-335.635123563526)) ;
#32540=CARTESIAN_POINT('Ctrl Pts',(-10.19406065239,16.5353155355663,-335.635980411464)) ;
#32541=CARTESIAN_POINT('Ctrl Pts',(-10.0807848215183,16.6045878244281,-335.637613486936)) ;
#32542=CARTESIAN_POINT('Ctrl Pts',(-10.0271146131637,16.6370529830363,-335.638388729742)) ;
#32543=CARTESIAN_POINT('Ctrl Pts',(-9.87310919136187,16.7291950858579,-335.640616423696)) ;
#32544=CARTESIAN_POINT('Ctrl Pts',(-9.77239205851055,16.7882282186189,-335.642077096036)) ;
#32545=CARTESIAN_POINT('Ctrl Pts',(-9.35970890294749,17.0251412801353,-335.648067961863)) ;
#32546=CARTESIAN_POINT('Ctrl Pts',(-9.04337103664606,17.1952617273774,-335.652672437296)) ;
#32547=CARTESIAN_POINT('Ctrl Pts',(-8.2438164806741,17.5970771228733,-335.664197181086)) ;
#32548=CARTESIAN_POINT('Ctrl Pts',(-7.75538450843575,17.8177340412732,-335.671133334483)) ;
#32549=CARTESIAN_POINT('Ctrl Pts',(-7.11386087053336,18.0761696691357,-335.679959410929)) ;
#32550=CARTESIAN_POINT('Ctrl Pts',(-6.96856784008059,18.1326773732957,-335.681940623787)) ;
#32551=CARTESIAN_POINT('Ctrl Pts',(-6.61044241615653,18.2670201688964,-335.686777193329)) ;
#32552=CARTESIAN_POINT('Ctrl Pts',(-6.39689785167203,18.3428916186177,-335.68962089022)) ;
#32553=CARTESIAN_POINT('Ctrl Pts',(-6.05412096514747,18.4579647198664,-335.694118715964)) ;
#32554=CARTESIAN_POINT('Ctrl Pts',(-5.9257230647847,18.4995850893973,-335.695788810376)) ;
#32555=CARTESIAN_POINT('Ctrl Pts',(-5.67619444389009,18.5776057750132,-335.699006321153)) ;
#32556=CARTESIAN_POINT('Ctrl Pts',(-5.55512135805032,18.6141678955278,-335.70055476523)) ;
#32557=CARTESIAN_POINT('Ctrl Pts',(-5.2633124822417,18.6991888339239,-335.704257322457)) ;
#32558=CARTESIAN_POINT('Ctrl Pts',(-5.0922527103062,18.7464952402663,-335.706403643753)) ;
#32559=CARTESIAN_POINT('Ctrl Pts',(-4.0807826751397,19.0113501298913,-335.718965577428)) ;
#32560=CARTESIAN_POINT('Ctrl Pts',(-3.22720415501608,19.1747065159298,-335.728993928958)) ;
#32561=CARTESIAN_POINT('Ctrl Pts',(-2.14653114354692,19.3072972921911,-335.741774078026)) ;
#32562=CARTESIAN_POINT('Ctrl Pts',(-1.92705175389449,19.3304370356936,-335.744377046707)) ;
#32563=CARTESIAN_POINT('Ctrl Pts',(-1.55469452571458,19.3632899309323,-335.748833489649)) ;
#32564=CARTESIAN_POINT('Ctrl Pts',(-1.40200925360456,19.3749436631064,-335.750672366312)) ;
#32565=CARTESIAN_POINT('Ctrl Pts',(-1.17283058990149,19.3897124859085,-335.753458936906)) ;
#32566=CARTESIAN_POINT('Ctrl Pts',(-1.09643039862242,19.3941826907074,-335.754392290496)) ;
#32567=CARTESIAN_POINT('Ctrl Pts',(-0.953578611560748,19.4016941943485,
-335.756147210947)) ;
#32568=CARTESIAN_POINT('Ctrl Pts',(-0.887134055795053,19.4048458615229,
-335.75696754852)) ;
#32569=CARTESIAN_POINT('Ctrl Pts',(-0.717372114571747,19.4120244373768,
-335.759072973522)) ;
#32570=CARTESIAN_POINT('Ctrl Pts',(-0.614036384668021,19.4155678460163,
-335.760363470728)) ;
#32571=CARTESIAN_POINT('Ctrl Pts',(-0.145464010118424,19.4278907322384,
-335.766248073594)) ;
#32572=CARTESIAN_POINT('Ctrl Pts',(0.219947175243785,19.4271902351739,-335.770926314856)) ;
#32573=CARTESIAN_POINT('Ctrl Pts',(1.00693950659581,19.4034736899051,-335.78106120025)) ;
#32574=CARTESIAN_POINT('Ctrl Pts',(1.42823334259071,19.3770190790373,-335.786522476523)) ;
#32575=CARTESIAN_POINT('Ctrl Pts',(2.13771006504435,19.3092031544045,-335.795671930856)) ;
#32576=CARTESIAN_POINT('Ctrl Pts',(2.42643280787893,19.2750500662543,-335.799382610356)) ;
#32577=CARTESIAN_POINT('Ctrl Pts',(2.93790715458167,19.2028729964967,-335.805913599525)) ;
#32578=CARTESIAN_POINT('Ctrl Pts',(3.16096675878464,19.167418166897,-335.808747513376)) ;
#32579=CARTESIAN_POINT('Ctrl Pts',(3.51613095889253,19.1045970483289,-335.81323393383)) ;
#32580=CARTESIAN_POINT('Ctrl Pts',(3.64865628121196,19.0797304147725,-335.81490225981)) ;
#32581=CARTESIAN_POINT('Ctrl Pts',(3.90502407913752,19.0288576192373,-335.818118721493)) ;
#32582=CARTESIAN_POINT('Ctrl Pts',(4.02889258391949,19.0030171275002,-335.819667858727)) ;
#32583=CARTESIAN_POINT('Ctrl Pts',(4.32627361890008,18.9379414122439,-335.823376048315)) ;
#32584=CARTESIAN_POINT('Ctrl Pts',(4.49951697778285,18.8975293478571,-335.825527244058)) ;
#32585=CARTESIAN_POINT('Ctrl Pts',(5.05450323104763,18.7600044742503,-335.832396258865)) ;
#32586=CARTESIAN_POINT('Ctrl Pts',(5.43385589438791,18.653658670498,-335.837055457851)) ;
#32587=CARTESIAN_POINT('Ctrl Pts',(6.33344971196237,18.3716979848589,-335.848120535167)) ;
#32588=CARTESIAN_POINT('Ctrl Pts',(6.84999272707859,18.185419165304,-335.854483788144)) ;
#32589=CARTESIAN_POINT('Ctrl Pts',(7.4773912529085,17.9286335358407,-335.862473726898)) ;
#32590=CARTESIAN_POINT('Ctrl Pts',(7.59634010366043,17.8785597125019,-335.86400083869)) ;
#32591=CARTESIAN_POINT('Ctrl Pts',(7.86475938980588,17.7624010395596,-335.867482496846)) ;
#32592=CARTESIAN_POINT('Ctrl Pts',(8.01391258620065,17.6956078128295,-335.869442425844)) ;
#32593=CARTESIAN_POINT('Ctrl Pts',(8.23329279274307,17.5940231848689,-335.872373713308)) ;
#32594=CARTESIAN_POINT('Ctrl Pts',(8.30418081290992,17.5606760418493,-335.873328490985)) ;
#32595=CARTESIAN_POINT('Ctrl Pts',(8.43504732675797,17.498144200191,-335.875106815385)) ;
#32596=CARTESIAN_POINT('Ctrl Pts',(8.49508084183715,17.469077689153,-335.875928915506)) ;
#32597=CARTESIAN_POINT('Ctrl Pts',(8.64487238338976,17.3955981586829,-335.877995267685)) ;
#32598=CARTESIAN_POINT('Ctrl Pts',(8.7344388651488,17.3507991601208,-335.879244348401)) ;
#32599=CARTESIAN_POINT('Ctrl Pts',(9.15923585859752,17.1342030911272,-335.885225994469)) ;
#32600=CARTESIAN_POINT('Ctrl Pts',(9.48976834250732,16.9533717272254,-335.890050243089)) ;
#32601=CARTESIAN_POINT('Ctrl Pts',(10.1790623279319,16.5497872254017,-335.90033326609)) ;
#32602=CARTESIAN_POINT('Ctrl Pts',(10.5362449572835,16.3247146916703,-335.90579499952)) ;
#32603=CARTESIAN_POINT('Ctrl Pts',(11.1246149894576,15.9266036031314,-335.914913253124)) ;
#32604=CARTESIAN_POINT('Ctrl Pts',(11.3597914538405,15.7597239683559,-335.918592986358)) ;
#32605=CARTESIAN_POINT('Ctrl Pts',(11.7713929167244,15.4536525284395,-335.925077323906)) ;
#32606=CARTESIAN_POINT('Ctrl Pts',(11.9492819863367,15.3165181403209,-335.927895229523)) ;
#32607=CARTESIAN_POINT('Ctrl Pts',(12.2299210674897,15.0923084892762,-335.932362983197)) ;
#32608=CARTESIAN_POINT('Ctrl Pts',(12.3342127994981,15.0071962580834,-335.934028412512)) ;
#32609=CARTESIAN_POINT('Ctrl Pts',(12.5348849984341,14.8399231725124,-335.937243187685)) ;
#32610=CARTESIAN_POINT('Ctrl Pts',(12.6313633170866,14.7578901774911,-335.938793491881)) ;
#32611=CARTESIAN_POINT('Ctrl Pts',(12.8405959111588,14.5764302356289,-335.942166946575)) ;
#32612=CARTESIAN_POINT('Ctrl Pts',(12.9530121778428,14.4766258971537,-335.943986766317)) ;
#32613=CARTESIAN_POINT('Ctrl Pts',(13.4061798029301,14.0647940922574,-335.951357962422)) ;
#32614=CARTESIAN_POINT('Ctrl Pts',(13.7369062771369,13.7419611781387,-335.956816230053)) ;
#32615=CARTESIAN_POINT('Ctrl Pts',(14.1323392970849,13.3274117999146,-335.963530527086)) ;
#32616=CARTESIAN_POINT('Ctrl Pts',(14.208182975782,13.2465261796419,-335.964827616629)) ;
#32617=CARTESIAN_POINT('Ctrl Pts',(14.576358653743,12.8470748738478,-335.971177050621)) ;
#32618=CARTESIAN_POINT('Ctrl Pts',(14.8586907523923,12.519459757042,-335.976208764485)) ;
#32619=CARTESIAN_POINT('Ctrl Pts',(15.2303499169125,12.0578912903062,-335.983209849402)) ;
#32620=CARTESIAN_POINT('Ctrl Pts',(15.3292969887696,11.9318462395133,-335.985113483242)) ;
#32621=CARTESIAN_POINT('Ctrl Pts',(15.5010153825124,11.7074383465584,-335.988500001492)) ;
#32622=CARTESIAN_POINT('Ctrl Pts',(15.5744381709813,11.6095850967504,-335.989975834619)) ;
#32623=CARTESIAN_POINT('Ctrl Pts',(15.6887957362159,11.4541391740718,-335.992323962761)) ;
#32624=CARTESIAN_POINT('Ctrl Pts',(15.7303490777553,11.3970054729745,-335.993187786119)) ;
#32625=CARTESIAN_POINT('Ctrl Pts',(15.8079406133976,11.2890883627189,-335.994822083267)) ;
#32626=CARTESIAN_POINT('Ctrl Pts',(15.8440480979892,11.2383558564305,-335.995591462222)) ;
#32627=CARTESIAN_POINT('Ctrl Pts',(15.9456335041618,11.0941615034446,-335.997780228086)) ;
#32628=CARTESIAN_POINT('Ctrl Pts',(16.0105326151956,11.0002951158325,-335.999207406125)) ;
#32629=CARTESIAN_POINT('Ctrl Pts',(16.3855850565694,10.447489843194,-336.007613311568)) ;
#32630=CARTESIAN_POINT('Ctrl Pts',(16.6768208230405,9.97602565532701,-336.014778137021)) ;
#32631=CARTESIAN_POINT('Ctrl Pts',(17.1481353942045,9.13458374899171,-336.027219344601)) ;
#32632=CARTESIAN_POINT('Ctrl Pts',(17.3373560548407,8.77013419506925,-336.032503228553)) ;
#32633=CARTESIAN_POINT('Ctrl Pts',(17.6365602947772,8.14625903012451,-336.041301732381)) ;
#32634=CARTESIAN_POINT('Ctrl Pts',(17.7527075687761,7.88994104496799,-336.044849563252)) ;
#32635=CARTESIAN_POINT('Ctrl Pts',(17.9199542184514,7.49844667179827,-336.050160207248)) ;
#32636=CARTESIAN_POINT('Ctrl Pts',(17.9751810094003,7.36507497812842,-336.051950868857)) ;
#32637=CARTESIAN_POINT('Ctrl Pts',(18.0751527732988,7.11582070932191,-336.055263137615)) ;
#32638=CARTESIAN_POINT('Ctrl Pts',(18.1202826986435,7.00010050735837,-336.056787352189)) ;
#32639=CARTESIAN_POINT('Ctrl Pts',(18.2203416760889,6.736080600315,-336.060234938578)) ;
#32640=CARTESIAN_POINT('Ctrl Pts',(18.2745758429249,6.5875268880064,-336.062153447982)) ;
#32641=CARTESIAN_POINT('Ctrl Pts',(18.442947427211,6.10824955982248,-336.068279194138)) ;
#32642=CARTESIAN_POINT('Ctrl Pts',(18.5499664591244,5.77509892452837,-336.072439164663)) ;
#32643=CARTESIAN_POINT('Ctrl Pts',(18.7203733115832,5.19087480740729,-336.0796116639)) ;
#32644=CARTESIAN_POINT('Ctrl Pts',(18.7878475444258,4.94108722586867,-336.08264044136)) ;
#32645=CARTESIAN_POINT('Ctrl Pts',(18.9926711719856,4.11785321353048,-336.092553859892)) ;
#32646=CARTESIAN_POINT('Ctrl Pts',(19.1089044987125,3.53949682372526,-336.099402211662)) ;
#32647=CARTESIAN_POINT('Ctrl Pts',(19.2164633242485,2.84110104341549,-336.107879963591)) ;
#32648=CARTESIAN_POINT('Ctrl Pts',(19.2332294135482,2.72528972725188,-336.109292946476)) ;
#32649=CARTESIAN_POINT('Ctrl Pts',(19.2582974932836,2.54036355951316,-336.111565048673)) ;
#32650=CARTESIAN_POINT('Ctrl Pts',(19.2672761955969,2.47134322898719,-336.112416592098)) ;
#32651=CARTESIAN_POINT('Ctrl Pts',(19.2836898911206,2.33963959939585,-336.114049360738)) ;
#32652=CARTESIAN_POINT('Ctrl Pts',(19.2911906764554,2.27696542472912,-336.114829691825)) ;
#32653=CARTESIAN_POINT('Ctrl Pts',(19.3119488024704,2.09604761226497,-336.117090733073)) ;
#32654=CARTESIAN_POINT('Ctrl Pts',(19.3244253751792,1.9777173707613,-336.118580037919)) ;
#32655=CARTESIAN_POINT('Ctrl Pts',(19.3806467667172,1.3930360476835,-336.125978195184)) ;
#32656=CARTESIAN_POINT('Ctrl Pts',(19.408601031983,0.925323421021146,-336.132015947265)) ;
#32657=CARTESIAN_POINT('Ctrl Pts',(19.4304207575132,-0.00175656256659662,
-336.143979551693)) ;
#32658=CARTESIAN_POINT('Ctrl Pts',(19.4249557886001,-0.460812106955017,
-336.149901328882)) ;
#32659=CARTESIAN_POINT('Ctrl Pts',(19.3964656964208,-1.06217678930648,-336.157569146231)) ;
#32660=CARTESIAN_POINT('Ctrl Pts',(19.3881148957429,-1.20503190508095,-336.159384351076)) ;
#32661=CARTESIAN_POINT('Ctrl Pts',(19.3633566612534,-1.56100175775195,-336.163889286857)) ;
#32662=CARTESIAN_POINT('Ctrl Pts',(19.3450087715052,-1.77396266488482,-336.166567950269)) ;
#32663=CARTESIAN_POINT('Ctrl Pts',(19.3095838071213,-2.11853612078625,-336.17087317959)) ;
#32664=CARTESIAN_POINT('Ctrl Pts',(19.2946660155655,-2.2503523066438,-336.172513311891)) ;
#32665=CARTESIAN_POINT('Ctrl Pts',(19.2629184547589,-2.50729636778672,-336.175697296077)) ;
#32666=CARTESIAN_POINT('Ctrl Pts',(19.24621667837,-2.63243349173348,-336.177241897102)) ;
#32667=CARTESIAN_POINT('Ctrl Pts',(19.2063885002707,-2.91016914352994,-336.180657512761)) ;
#32668=CARTESIAN_POINT('Ctrl Pts',(19.1826608814919,-3.06267289414458,-336.182524547727)) ;
#32669=CARTESIAN_POINT('Ctrl Pts',(19.0655550987178,-3.76049392732415,-336.191035074715)) ;
#32670=CARTESIAN_POINT('Ctrl Pts',(18.9507238557215,-4.30194988497588,-336.197539000283)) ;
#32671=CARTESIAN_POINT('Ctrl Pts',(18.6791969513373,-5.35785465170593,-336.210283752651)) ;
#32672=CARTESIAN_POINT('Ctrl Pts',(18.5239461474595,-5.87217350887204,-336.216522294436)) ;
#32673=CARTESIAN_POINT('Ctrl Pts',(18.2945098342491,-6.53204827840809,-336.22484090314)) ;
#32674=CARTESIAN_POINT('Ctrl Pts',(18.2395302320901,-6.68403183406783,-336.226779640034)) ;
#32675=CARTESIAN_POINT('Ctrl Pts',(18.1552036921936,-6.9083494659383,-336.229685651692)) ;
#32676=CARTESIAN_POINT('Ctrl Pts',(18.1273070387683,-6.98122145118926,-336.230636748208)) ;
#32677=CARTESIAN_POINT('Ctrl Pts',(18.074718553917,-7.11615310254565,-336.232412524771)) ;
#32678=CARTESIAN_POINT('Ctrl Pts',(18.0501443023728,-7.17825719857534,-336.233235812079)) ;
#32679=CARTESIAN_POINT('Ctrl Pts',(17.9876865531158,-7.33375171384866,-336.2353113631)) ;
#32680=CARTESIAN_POINT('Ctrl Pts',(17.9493956519603,-7.42697633109431,-336.236568553163)) ;
#32681=CARTESIAN_POINT('Ctrl Pts',(17.7685866806301,-7.85761479207375,-336.242428491236)) ;
#32682=CARTESIAN_POINT('Ctrl Pts',(17.6172689575329,-8.1912524325871,-336.247117288097)) ;
#32683=CARTESIAN_POINT('Ctrl Pts',(17.2583880445812,-8.92652727186592,-336.25764767693)) ;
#32684=CARTESIAN_POINT('Ctrl Pts',(17.0460545886829,-9.32560296489143,-336.263497832938)) ;
#32685=CARTESIAN_POINT('Ctrl Pts',(16.7209311660354,-9.88839251163785,-336.271833471019)) ;
#32686=CARTESIAN_POINT('Ctrl Pts',(16.6192486144482,-10.0583508164693,-336.274363010264)) ;
#32687=CARTESIAN_POINT('Ctrl Pts',(16.3752969091566,-10.4523047834956,-336.280246521599)) ;
#32688=CARTESIAN_POINT('Ctrl Pts',(16.2310015222702,-10.6749994920816,-336.283587770418)) ;
#32689=CARTESIAN_POINT('Ctrl Pts',(16.002703164668,-11.0120026223252,-336.28866190468)) ;
#32690=CARTESIAN_POINT('Ctrl Pts',(15.9219350634168,-11.1284632468303,-336.290418869715)) ;
#32691=CARTESIAN_POINT('Ctrl Pts',(15.7678058116543,-11.3455910879825,-336.293701204069)) ;
#32692=CARTESIAN_POINT('Ctrl Pts',(15.694736780256,-11.4464568620659,-336.295228767429)) ;
#32693=CARTESIAN_POINT('Ctrl Pts',(15.5258939742687,-11.6748739117895,-336.298695174043)) ;
#32694=CARTESIAN_POINT('Ctrl Pts',(15.4295090456217,-11.8019623478959,-336.300628987119)) ;
#32695=CARTESIAN_POINT('Ctrl Pts',(15.0891799257369,-12.2394074793645,-336.307308146187)) ;
#32696=CARTESIAN_POINT('Ctrl Pts',(14.8373491696948,-12.5435049673477,-336.311990059341)) ;
#32697=CARTESIAN_POINT('Ctrl Pts',(14.1922744002128,-13.275833017342,-336.323463519854)) ;
#32698=CARTESIAN_POINT('Ctrl Pts',(13.788742799292,-13.6944866733356,-336.33019611587)) ;
#32699=CARTESIAN_POINT('Ctrl Pts',(13.2708181332957,-14.185682969699,-336.338604907545)) ;
#32700=CARTESIAN_POINT('Ctrl Pts',(13.1736534573154,-14.2759612558908,-336.340173492077)) ;
#32701=CARTESIAN_POINT('Ctrl Pts',(12.9524962889447,-14.4772636366326,-336.343731983731)) ;
#32702=CARTESIAN_POINT('Ctrl Pts',(12.8279861534573,-14.5877035072095,-336.345727228018)) ;
#32703=CARTESIAN_POINT('Ctrl Pts',(12.6424151263889,-14.7480908029304,-336.348700579874)) ;
#32704=CARTESIAN_POINT('Ctrl Pts',(12.5824444545552,-14.799288296626,-336.349661426106)) ;
#32705=CARTESIAN_POINT('Ctrl Pts',(12.4712773116559,-14.8930284985256,-336.351444083941)) ;
#32706=CARTESIAN_POINT('Ctrl Pts',(12.4201708051575,-14.9356758393262,-336.352264360868)) ;
#32707=CARTESIAN_POINT('Ctrl Pts',(12.2924063434799,-15.0411834289602,-336.354316186417)) ;
#32708=CARTESIAN_POINT('Ctrl Pts',(12.2154845131321,-15.1037210887828,-336.35555240904)) ;
#32709=CARTESIAN_POINT('Ctrl Pts',(11.8812327865812,-15.371244874611,-336.360921790152)) ;
#32710=CARTESIAN_POINT('Ctrl Pts',(11.619197284578,-15.5702638142426,-336.365124064473)) ;
#32711=CARTESIAN_POINT('Ctrl Pts',(11.2130320402589,-15.8627855616346,-336.371557307521)) ;
#32712=CARTESIAN_POINT('Ctrl Pts',(11.072507449104,-15.9611914363373,-336.373769151282)) ;
#32713=CARTESIAN_POINT('Ctrl Pts',(10.5476251998511,-16.3184855137077,-336.381960337636)) ;
#32714=CARTESIAN_POINT('Ctrl Pts',(10.1553433565598,-16.5654571154243,-336.387940941636)) ;
#32715=CARTESIAN_POINT('Ctrl Pts',(9.63016404898978,-16.8704259850824,-336.395676840117)) ;
#32716=CARTESIAN_POINT('Ctrl Pts',(9.50492342080253,-16.9413034726601,-336.3975025033)) ;
#32717=CARTESIAN_POINT('Ctrl Pts',(9.19101110953334,-17.1143792398034,-336.402028541279)) ;
#32718=CARTESIAN_POINT('Ctrl Pts',(9.00141174488035,-17.2148554687064,-336.404717807719)) ;
#32719=CARTESIAN_POINT('Ctrl Pts',(8.69182841190599,-17.3724028416349,-336.409035419336)) ;
#32720=CARTESIAN_POINT('Ctrl Pts',(8.57285555503001,-17.4314201751824,-336.410677480818)) ;
#32721=CARTESIAN_POINT('Ctrl Pts',(8.33970372192579,-17.5441124569692,-336.413862357455)) ;
#32722=CARTESIAN_POINT('Ctrl Pts',(8.22558847166244,-17.5979042620308,-336.415405952612)) ;
#32723=CARTESIAN_POINT('Ctrl Pts',(7.97108788755957,-17.7148547123622,-336.41881577427)) ;
#32724=CARTESIAN_POINT('Ctrl Pts',(7.8304593726415,-17.7774639835853,-336.420678071071)) ;
#32725=CARTESIAN_POINT('Ctrl Pts',(7.180939864233,-18.0574343139087,-336.429185815075)) ;
#32726=CARTESIAN_POINT('Ctrl Pts',(6.66365011223411,-18.2546596843894,-336.435691474728)) ;
#32727=CARTESIAN_POINT('Ctrl Pts',(5.63817601070086,-18.5962323345682,-336.448326642071)) ;
#32728=CARTESIAN_POINT('Ctrl Pts',(5.13112309516517,-18.7424774018071,-336.454455553875)) ;
#32729=CARTESIAN_POINT('Ctrl Pts',(4.45499673814361,-18.9079890758856,-336.462736015455)) ;
#32730=CARTESIAN_POINT('Ctrl Pts',(4.29072926475043,-18.9459412289238,-336.464756649918)) ;
#32731=CARTESIAN_POINT('Ctrl Pts',(4.04858103134329,-18.9985760444933,-336.467760200872)) ;
#32732=CARTESIAN_POINT('Ctrl Pts',(3.97107103327412,-19.0149282121542,-336.468725359217)) ;
#32733=CARTESIAN_POINT('Ctrl Pts',(3.82833856802639,-19.0441294774557,-336.470511192693)) ;
#32734=CARTESIAN_POINT('Ctrl Pts',(3.76314614256492,-19.057118743938,-336.471330271087)) ;
#32735=CARTESIAN_POINT('Ctrl Pts',(3.61698586669218,-19.0854612092665,-336.473173676975)) ;
#32736=CARTESIAN_POINT('Ctrl Pts',(3.53598441859183,-19.1006342957284,-336.474200022203)) ;
#32737=CARTESIAN_POINT('Ctrl Pts',(3.22171914446849,-19.1574344562094,-336.47819705375)) ;
#32738=CARTESIAN_POINT('Ctrl Pts',(2.98779808049232,-19.1953075375904,-336.481204102568)) ;
#32739=CARTESIAN_POINT('Ctrl Pts',(2.09464684482769,-19.3231912820163,-336.492737977661)) ;
#32740=CARTESIAN_POINT('Ctrl Pts',(1.4316402263817,-19.3835929583719,-336.50139268135)) ;
#32741=CARTESIAN_POINT('Ctrl Pts',(0.511344704047695,-19.4199519322021,
-336.513172303539)) ;
#32742=CARTESIAN_POINT('Ctrl Pts',(0.255680463055959,-19.4249999999729,
-336.516422120054)) ;
#32743=CARTESIAN_POINT('Ctrl Pts',(2.0594771027449E-9,-19.425,-336.519643262718)) ;
#32744=CARTESIAN_POINT('Origin',(0.,0.,-10.)) ;
#32745=CARTESIAN_POINT('',(-8.95436071499832E-8,-22.12975,-1.02655085110559)) ;
#32746=CARTESIAN_POINT('',(1.7916049440271E-8,-22.12975,-0.560977995021738)) ;
#32747=CARTESIAN_POINT('',(-2.71011275034311E-15,-22.12975,-10.)) ;
#32748=CARTESIAN_POINT('',(19.8223774287336,9.83980908931111,-0.000330426971074296)) ;
#32749=CARTESIAN_POINT('Ctrl Pts',(-8.95436062103849E-8,-22.12975,-1.02655085110559)) ;
#32750=CARTESIAN_POINT('Ctrl Pts',(0.362609696220858,-22.1297500014672,
-1.01848600551515)) ;
#32751=CARTESIAN_POINT('Ctrl Pts',(0.72522705394756,-22.1208376234837,-1.01042986688896)) ;
#32752=CARTESIAN_POINT('Ctrl Pts',(1.53612769302464,-22.0809392872267,-0.992319112084816)) ;
#32753=CARTESIAN_POINT('Ctrl Pts',(1.98395382077021,-22.0452146938743,-0.982252578822297)) ;
#32754=CARTESIAN_POINT('Ctrl Pts',(2.77376933583332,-21.9579460610462,-0.964168476362566)) ;
#32755=CARTESIAN_POINT('Ctrl Pts',(3.11622005686572,-21.9119683960168,-0.956204436732142)) ;
#32756=CARTESIAN_POINT('Ctrl Pts',(3.9444882237055,-21.7809547225949,-0.936731115874486)) ;
#32757=CARTESIAN_POINT('Ctrl Pts',(4.42881434833868,-21.6876595690219,-0.925172598567827)) ;
#32758=CARTESIAN_POINT('Ctrl Pts',(5.77387688743604,-21.3816227828005,-0.892846020575418)) ;
#32759=CARTESIAN_POINT('Ctrl Pts',(6.62554836549475,-21.1332339814427,-0.872142020144239)) ;
#32760=CARTESIAN_POINT('Ctrl Pts',(7.98459866969752,-20.6466092522381,-0.83899701975258)) ;
#32761=CARTESIAN_POINT('Ctrl Pts',(8.50189076450104,-20.4390349407229,-0.82634521033463)) ;
#32762=CARTESIAN_POINT('Ctrl Pts',(9.71611455548687,-19.8977208160516,-0.796431441609054)) ;
#32763=CARTESIAN_POINT('Ctrl Pts',(10.4044875617115,-19.5465807129507,-0.779305327577847)) ;
#32764=CARTESIAN_POINT('Ctrl Pts',(11.5569027476881,-18.8805741829163,-0.749688324724039)) ;
#32765=CARTESIAN_POINT('Ctrl Pts',(12.0299437418324,-18.5827481545256,-0.737229280268692)) ;
#32766=CARTESIAN_POINT('Ctrl Pts',(12.7567649357998,-18.0857480739021,-0.717247463297029)) ;
#32767=CARTESIAN_POINT('Ctrl Pts',(13.0183335205635,-17.8983888437069,-0.709861462377852)) ;
#32768=CARTESIAN_POINT('Ctrl Pts',(13.9712906261952,-17.1838499002227,-0.682284087339741)) ;
#32769=CARTESIAN_POINT('Ctrl Pts',(14.6355198505277,-16.6217694411575,-0.661791940043313)) ;
#32770=CARTESIAN_POINT('Ctrl Pts',(15.7608075048988,-15.54965683489,-0.625490019299988)) ;
#32771=CARTESIAN_POINT('Ctrl Pts',(16.2344618515354,-15.054472452485,-0.609621715797516)) ;
#32772=CARTESIAN_POINT('Ctrl Pts',(17.0783717573338,-14.0859755606526,-0.58024669556295)) ;
#32773=CARTESIAN_POINT('Ctrl Pts',(17.4538110284374,-13.6180019539252,-0.566701247149113)) ;
#32774=CARTESIAN_POINT('Ctrl Pts',(18.2720246233815,-12.5086140739283,-0.535824299528097)) ;
#32775=CARTESIAN_POINT('Ctrl Pts',(18.7008625973473,-11.8579107081509,-0.518599680720284)) ;
#32776=CARTESIAN_POINT('Ctrl Pts',(19.3207214504822,-10.7998076192541,-0.491241644673661)) ;
#32777=CARTESIAN_POINT('Ctrl Pts',(19.5351702612548,-10.4068842802415,-0.481209390700184)) ;
#32778=CARTESIAN_POINT('Ctrl Pts',(19.8943100646021,-9.69857774783108,-0.463132144181344)) ;
#32779=CARTESIAN_POINT('Ctrl Pts',(20.0437768095907,-9.38578656101391,-0.455139564468137)) ;
#32780=CARTESIAN_POINT('Ctrl Pts',(20.3897033426949,-8.61587365703672,-0.435534276632124)) ;
#32781=CARTESIAN_POINT('Ctrl Pts',(20.5782156949307,-8.15538584256677,-0.423871110867056)) ;
#32782=CARTESIAN_POINT('Ctrl Pts',(21.0560121038169,-6.86590010377982,-0.391641309174787)) ;
#32783=CARTESIAN_POINT('Ctrl Pts',(21.3117412612872,-6.02544075174472,-0.371139443495109)) ;
#32784=CARTESIAN_POINT('Ctrl Pts',(21.6467235625728,-4.63183043577311,-0.338224605979193)) ;
#32785=CARTESIAN_POINT('Ctrl Pts',(21.7561801925713,-4.08694554924959,-0.32560717830562)) ;
#32786=CARTESIAN_POINT('Ctrl Pts',(21.9694215327346,-2.77050134494014,-0.295594424331887)) ;
#32787=CARTESIAN_POINT('Ctrl Pts',(22.0532381496147,-1.99645952212054,-0.27834037997748)) ;
#32788=CARTESIAN_POINT('Ctrl Pts',(22.126963222074,-0.660759385464442,-0.248573501066504)) ;
#32789=CARTESIAN_POINT('Ctrl Pts',(22.1365965856442,-0.100939272688503,
-0.236093430574614)) ;
#32790=CARTESIAN_POINT('Ctrl Pts',(22.1182742535962,0.782940635789909,-0.216027390570924)) ;
#32791=CARTESIAN_POINT('Ctrl Pts',(22.1044223123916,1.10705099321042,-0.208578216171669)) ;
#32792=CARTESIAN_POINT('Ctrl Pts',(21.9965322016293,2.77233645091229,-0.16993458549348)) ;
#32793=CARTESIAN_POINT('Ctrl Pts',(21.7875385940238,4.10323198088417,-0.138092596463536)) ;
#32794=CARTESIAN_POINT('Ctrl Pts',(21.3339118596575,5.90359022006686,-0.0953269285021801)) ;
#32795=CARTESIAN_POINT('Ctrl Pts',(21.1915639711943,6.39576377758073,-0.0836435870746683)) ;
#32796=CARTESIAN_POINT('Ctrl Pts',(20.7006088227332,7.89606379120685,-0.0479604109604452)) ;
#32797=CARTESIAN_POINT('Ctrl Pts',(20.2961277010017,8.88426843257487,-0.0244196869317178)) ;
#32798=CARTESIAN_POINT('Ctrl Pts',(19.8219829119648,9.8394526524738,-0.000629142560504862)) ;
#32799=CARTESIAN_POINT('',(19.8220328557589,-9.83935203800096,1.66533453693773E-15)) ;
#32800=CARTESIAN_POINT('Origin',(0.,0.,1.11022302462516E-15)) ;
#32801=CARTESIAN_POINT('Ctrl Pts',(19.8220328557589,-9.83935203800097,-5.87962838138889E-14)) ;
#32802=CARTESIAN_POINT('Ctrl Pts',(19.7227624021928,-10.0393390071218,-0.00509820586393841)) ;
#32803=CARTESIAN_POINT('Ctrl Pts',(19.6204713487578,-10.2378116787129,-0.0102333105362058)) ;
#32804=CARTESIAN_POINT('Ctrl Pts',(19.2629858100134,-10.9063885188397,-0.0277523314883718)) ;
#32805=CARTESIAN_POINT('Ctrl Pts',(18.9937589249579,-11.3687753322354,-0.0402408666751295)) ;
#32806=CARTESIAN_POINT('Ctrl Pts',(18.3810236588299,-12.3385009151472,-0.0670033576910186)) ;
#32807=CARTESIAN_POINT('Ctrl Pts',(18.0326653279391,-12.8422592393881,-0.0812604592177863)) ;
#32808=CARTESIAN_POINT('Ctrl Pts',(17.3294415863396,-13.7740513635541,-0.108181886905778)) ;
#32809=CARTESIAN_POINT('Ctrl Pts',(16.9784569708648,-14.2044374063232,-0.12086245142339)) ;
#32810=CARTESIAN_POINT('Ctrl Pts',(16.0958552164432,-15.2071942202832,-0.151062922909145)) ;
#32811=CARTESIAN_POINT('Ctrl Pts',(15.5494020885818,-15.7655134967636,-0.168423762842354)) ;
#32812=CARTESIAN_POINT('Ctrl Pts',(14.4039919245186,-16.8181873391972,-0.202885386509353)) ;
#32813=CARTESIAN_POINT('Ctrl Pts',(13.8062473940792,-17.3122478815185,-0.219965866429256)) ;
#32814=CARTESIAN_POINT('Ctrl Pts',(12.9446389381245,-17.9513466049824,-0.244141957214301)) ;
#32815=CARTESIAN_POINT('Ctrl Pts',(12.7018989674816,-18.1239146914682,-0.250916992724896)) ;
#32816=CARTESIAN_POINT('Ctrl Pts',(11.8950105963065,-18.67337101296,-0.273365355048762)) ;
#32817=CARTESIAN_POINT('Ctrl Pts',(11.3170132879896,-19.0292213673286,-0.289270604881214)) ;
#32818=CARTESIAN_POINT('Ctrl Pts',(10.1719036387582,-19.6635695184228,-0.319947037687785)) ;
#32819=CARTESIAN_POINT('Ctrl Pts',(9.6074046478026,-19.9454599331646,-0.334706087224686)) ;
#32820=CARTESIAN_POINT('Ctrl Pts',(8.52106232577095,-20.4311065996851,-0.362271338155627)) ;
#32821=CARTESIAN_POINT('Ctrl Pts',(8.0020163974881,-20.6399215203552,-0.375101142193199)) ;
#32822=CARTESIAN_POINT('Ctrl Pts',(6.61815770165498,-21.1365977990698,-0.408479285520121)) ;
#32823=CARTESIAN_POINT('Ctrl Pts',(5.74251417470133,-21.3911037495927,-0.428748456364493)) ;
#32824=CARTESIAN_POINT('Ctrl Pts',(4.38808097926699,-21.6955828842006,-0.459624145952587)) ;
#32825=CARTESIAN_POINT('Ctrl Pts',(3.91922099362602,-21.7851618163998,-0.47023673397663)) ;
#32826=CARTESIAN_POINT('Ctrl Pts',(3.11104135450716,-21.9126335258969,-0.488623482855503)) ;
#32827=CARTESIAN_POINT('Ctrl Pts',(2.77306623558891,-21.9579641625977,-0.496344205641062)) ;
#32828=CARTESIAN_POINT('Ctrl Pts',(1.74610825411354,-22.0716148026216,-0.520044881800077)) ;
#32829=CARTESIAN_POINT('Ctrl Pts',(1.05484652816179,-22.1154327344403,-0.536261600369375)) ;
#32830=CARTESIAN_POINT('Ctrl Pts',(0.241784244200346,-22.1287594266641,
-0.555313852831496)) ;
#32831=CARTESIAN_POINT('Ctrl Pts',(0.120888776504814,-22.1297499999021,
-0.558146584989623)) ;
#32832=CARTESIAN_POINT('Ctrl Pts',(1.79160461119543E-8,-22.12975,-0.560977995021737)) ;
#32833=CARTESIAN_POINT('Origin',(0.,0.,-10.)) ;
#32834=CARTESIAN_POINT('',(-1.88975816071502E-8,-22.12975,-4.20243196305312)) ;
#32835=CARTESIAN_POINT('',(-0.000296723799801057,-22.1297499979164,-3.73504651729724)) ;
#32836=CARTESIAN_POINT('',(-2.71011275034311E-15,-22.12975,-10.)) ;
#32837=CARTESIAN_POINT('Ctrl Pts',(-1.88975821102666E-8,-22.12975,-4.20243196305312)) ;
#32838=CARTESIAN_POINT('Ctrl Pts',(0.78300485118741,-22.1297500006686,-4.18423521862199)) ;
#32839=CARTESIAN_POINT('Ctrl Pts',(1.56551886118347,-22.0881930893127,-4.16579715593098)) ;
#32840=CARTESIAN_POINT('Ctrl Pts',(3.02567666389269,-21.9326410176014,-4.13149793264282)) ;
#32841=CARTESIAN_POINT('Ctrl Pts',(3.70337738557218,-21.8284325774216,-4.11561883254211)) ;
#32842=CARTESIAN_POINT('Ctrl Pts',(4.9623028889739,-21.57452559444,-4.08624955504827)) ;
#32843=CARTESIAN_POINT('Ctrl Pts',(5.54440609758268,-21.4323160869635,-4.07271992113879)) ;
#32844=CARTESIAN_POINT('Ctrl Pts',(6.86618024283472,-21.0519419155049,-4.04190991419865)) ;
#32845=CARTESIAN_POINT('Ctrl Pts',(7.60051623168367,-20.7980970534689,-4.02473541276586)) ;
#32846=CARTESIAN_POINT('Ctrl Pts',(8.73589994440261,-20.337437042036,-3.99740218876045)) ;
#32847=CARTESIAN_POINT('Ctrl Pts',(9.14657913863443,-20.1560754837298,-3.98734203485526)) ;
#32848=CARTESIAN_POINT('Ctrl Pts',(9.86376618477889,-19.8129205153953,-3.96924708911815)) ;
#32849=CARTESIAN_POINT('Ctrl Pts',(10.1725230076371,-19.6561815526484,-3.96126537294436)) ;
#32850=CARTESIAN_POINT('Ctrl Pts',(10.9138762948244,-19.2576897257486,-3.94171893335661)) ;
#32851=CARTESIAN_POINT('Ctrl Pts',(11.3422787689048,-19.0085249251094,-3.93010441909909)) ;
#32852=CARTESIAN_POINT('Ctrl Pts',(12.5084906178322,-18.2767676092257,-3.89784067067216)) ;
#32853=CARTESIAN_POINT('Ctrl Pts',(13.2263820873722,-17.7641608524847,-3.87725589537778)) ;
#32854=CARTESIAN_POINT('Ctrl Pts',(14.3449480049318,-16.8599681317877,-3.84423021760251)) ;
#32855=CARTESIAN_POINT('Ctrl Pts',(14.7647325830739,-16.493596841325,-3.83158274933754)) ;
#32856=CARTESIAN_POINT('Ctrl Pts',(15.733125214267,-15.5817944163126,-3.80165297156323)) ;
#32857=CARTESIAN_POINT('Ctrl Pts',(16.2678412400112,-15.0226792186925,-3.78450734009598)) ;
#32858=CARTESIAN_POINT('Ctrl Pts',(17.1366560616442,-14.0133137923059,-3.75487365330684)) ;
#32859=CARTESIAN_POINT('Ctrl Pts',(17.4849461579156,-13.5762511426536,-3.7424175187845)) ;
#32860=CARTESIAN_POINT('Ctrl Pts',(18.0068635981934,-12.8678626249446,-3.72244984900015)) ;
#32861=CARTESIAN_POINT('Ctrl Pts',(18.1917492710008,-12.6051290949033,-3.71507520463808)) ;
#32862=CARTESIAN_POINT('Ctrl Pts',(18.8494782161314,-11.6258307576775,-3.68776265657516)) ;
#32863=CARTESIAN_POINT('Ctrl Pts',(19.2862352510792,-10.885949687718,-3.66753074198687)) ;
#32864=CARTESIAN_POINT('Ctrl Pts',(19.9955580434754,-9.50698232095388,-3.63130141047985)) ;
#32865=CARTESIAN_POINT('Ctrl Pts',(20.2831517821455,-8.87686994284161,-3.61525579695924)) ;
#32866=CARTESIAN_POINT('Ctrl Pts',(20.7625767009978,-7.68093014452203,-3.58578552089687)) ;
#32867=CARTESIAN_POINT('Ctrl Pts',(20.961962437541,-7.11880728035882,-3.57231532063576)) ;
#32868=CARTESIAN_POINT('Ctrl Pts',(21.3650867628127,-5.81769368693727,-3.54179649387805)) ;
#32869=CARTESIAN_POINT('Ctrl Pts',(21.5536293318583,-5.07479594928609,-3.52484904812858)) ;
#32870=CARTESIAN_POINT('Ctrl Pts',(21.7954011197627,-3.86117466366818,-3.49725501933999)) ;
#32871=CARTESIAN_POINT('Ctrl Pts',(21.8727230561259,-3.39590352541369,-3.4866923328178)) ;
#32872=CARTESIAN_POINT('Ctrl Pts',(21.9814386856978,-2.58160504952151,-3.46798920868275)) ;
#32873=CARTESIAN_POINT('Ctrl Pts',(22.019517880678,-2.23364242468428,-3.45991686684113)) ;
#32874=CARTESIAN_POINT('Ctrl Pts',(22.0925718415895,-1.37907841379411,-3.43999185570009)) ;
#32875=CARTESIAN_POINT('Ctrl Pts',(22.1183948259315,-0.87189240776236,-3.42808647880888)) ;
#32876=CARTESIAN_POINT('Ctrl Pts',(22.1408557271778,0.492446247477333,-3.39611120558737)) ;
#32877=CARTESIAN_POINT('Ctrl Pts',(22.1051917487505,1.34926413969942,-3.37610701003947)) ;
#32878=CARTESIAN_POINT('Ctrl Pts',(21.964606013123,2.75520954571649,-3.34365897132579)) ;
#32879=CARTESIAN_POINT('Ctrl Pts',(21.8884352135779,3.30628298570175,-3.33102890509898)) ;
#32880=CARTESIAN_POINT('Ctrl Pts',(21.6560422697815,4.62033004379686,-3.30099688488503)) ;
#32881=CARTESIAN_POINT('Ctrl Pts',(21.4801585306618,5.37907142113982,-3.28373621250674)) ;
#32882=CARTESIAN_POINT('Ctrl Pts',(21.1099059788529,6.66409497016883,-3.25397972806693)) ;
#32883=CARTESIAN_POINT('Ctrl Pts',(20.9348493009641,7.19516294096022,-3.24151647728626)) ;
#32884=CARTESIAN_POINT('Ctrl Pts',(20.6277345573049,8.02033433692923,-3.22153479730581)) ;
#32885=CARTESIAN_POINT('Ctrl Pts',(20.5090426254401,8.31915634344553,-3.21415356247645)) ;
#32886=CARTESIAN_POINT('Ctrl Pts',(20.0454777454888,9.41595734257507,-3.18658348578997)) ;
#32887=CARTESIAN_POINT('Ctrl Pts',(19.6601908849865,10.1959956136134,-3.16609350199875)) ;
#32888=CARTESIAN_POINT('Ctrl Pts',(18.8908864215178,11.5468563991095,-3.12978223140487)) ;
#32889=CARTESIAN_POINT('Ctrl Pts',(18.524266906083,12.1262949679955,-3.1139027623445)) ;
#32890=CARTESIAN_POINT('Ctrl Pts',(17.7879394254013,13.1785359453817,-3.08453323347962)) ;
#32891=CARTESIAN_POINT('Ctrl Pts',(17.4247452710093,13.6551403561135,-3.07100370448131)) ;
#32892=CARTESIAN_POINT('Ctrl Pts',(16.5473917018921,14.7143632602694,-3.0401942464351)) ;
#32893=CARTESIAN_POINT('Ctrl Pts',(16.0209968529366,15.2858207703453,-3.02302017978602)) ;
#32894=CARTESIAN_POINT('Ctrl Pts',(15.1446172460368,16.1421148353708,-2.99568718783662)) ;
#32895=CARTESIAN_POINT('Ctrl Pts',(14.8141058538501,16.4459589627924,-2.98562680814571)) ;
#32896=CARTESIAN_POINT('Ctrl Pts',(14.2127121157218,16.965980751191,-2.96753211413899)) ;
#32897=CARTESIAN_POINT('Ctrl Pts',(13.9455635588588,17.1862427666548,-2.95955088865832)) ;
#32898=CARTESIAN_POINT('Ctrl Pts',(13.2838481960133,17.7062311402656,-2.94000648848942)) ;
#32899=CARTESIAN_POINT('Ctrl Pts',(12.8841681615987,17.9991514527427,-2.92839353878091)) ;
#32900=CARTESIAN_POINT('Ctrl Pts',(11.7469408061356,18.7753079532402,-2.89612819949671)) ;
#32901=CARTESIAN_POINT('Ctrl Pts',(10.9898416888136,19.2282658823658,-2.87554025816708)) ;
#32902=CARTESIAN_POINT('Ctrl Pts',(9.7135581298685,19.8917784829508,-2.84251145681018)) ;
#32903=CARTESIAN_POINT('Ctrl Pts',(9.20984560148602,20.129948164333,-2.82986391701871)) ;
#32904=CARTESIAN_POINT('Ctrl Pts',(7.98680608592124,20.652710061993,-2.79993469071419)) ;
#32905=CARTESIAN_POINT('Ctrl Pts',(7.26049624586082,20.9190989743876,-2.78278965894124)) ;
#32906=CARTESIAN_POINT('Ctrl Pts',(5.98788325920292,21.3115742357783,-2.75315661800815)) ;
#32907=CARTESIAN_POINT('Ctrl Pts',(5.44798861120393,21.4559398592125,-2.74070052636858)) ;
#32908=CARTESIAN_POINT('Ctrl Pts',(4.589968180642,21.6508941231005,-2.72073293767643)) ;
#32909=CARTESIAN_POINT('Ctrl Pts',(4.27521349671628,21.7152381899526,-2.71335832994253)) ;
#32910=CARTESIAN_POINT('Ctrl Pts',(3.11457478013725,21.9262899467058,-2.68604586299899)) ;
#32911=CARTESIAN_POINT('Ctrl Pts',(2.26175726656313,22.0305974020626,-2.66581398965343)) ;
#32912=CARTESIAN_POINT('Ctrl Pts',(0.714175751691377,22.1290536445136,-2.62958455912763)) ;
#32913=CARTESIAN_POINT('Ctrl Pts',(0.0216245513053864,22.1405647277536,
-2.61353880990829)) ;
#32914=CARTESIAN_POINT('Ctrl Pts',(-1.26624617556435,22.1015361333412,-2.58406840570951)) ;
#32915=CARTESIAN_POINT('Ctrl Pts',(-1.86119259462364,22.0594027148098,-2.57059820929732)) ;
#32916=CARTESIAN_POINT('Ctrl Pts',(-3.21492331677136,21.9083718212019,-2.54007944873172)) ;
#32917=CARTESIAN_POINT('Ctrl Pts',(-3.97120944804521,21.7839845389495,-2.52313206377637)) ;
#32918=CARTESIAN_POINT('Ctrl Pts',(-5.18021211847231,21.5200740511633,-2.49553798236486)) ;
#32919=CARTESIAN_POINT('Ctrl Pts',(-5.63756937642704,21.4048123368308,-2.48497517833923)) ;
#32920=CARTESIAN_POINT('Ctrl Pts',(-6.42737165390238,21.1786974905219,-2.46627185364127)) ;
#32921=CARTESIAN_POINT('Ctrl Pts',(-6.76151536127838,21.0743977054054,-2.45819943051582)) ;
#32922=CARTESIAN_POINT('Ctrl Pts',(-7.57395918489904,20.7994889440321,-2.43827410429456)) ;
#32923=CARTESIAN_POINT('Ctrl Pts',(-8.04913386346131,20.6202580079614,-2.42636849172306)) ;
#32924=CARTESIAN_POINT('Ctrl Pts',(-9.30852046957356,20.0950591552303,-2.3943935393047)) ;
#32925=CARTESIAN_POINT('Ctrl Pts',(-10.0795049122872,19.719623648425,-2.37438990042575)) ;
#32926=CARTESIAN_POINT('Ctrl Pts',(-11.3117935185232,19.0283584423186,-2.34194238675986)) ;
#32927=CARTESIAN_POINT('Ctrl Pts',(-11.7863812637265,18.7380981065092,-2.3293123087284)) ;
#32928=CARTESIAN_POINT('Ctrl Pts',(-12.8977356618232,17.9994451284545,-2.29928037167604)) ;
#32929=CARTESIAN_POINT('Ctrl Pts',(-13.5227583816477,17.5347260953241,-2.28201979107091)) ;
#32930=CARTESIAN_POINT('Ctrl Pts',(-14.5523612059734,16.6813390151862,-2.25226348711761)) ;
#32931=CARTESIAN_POINT('Ctrl Pts',(-14.9690529600201,16.3084559135027,-2.23980032374567)) ;
#32932=CARTESIAN_POINT('Ctrl Pts',(-15.6024542784167,15.6968980650459,-2.21981900498933)) ;
#32933=CARTESIAN_POINT('Ctrl Pts',(-15.8288355106009,15.4685859272784,-2.21243804525713)) ;
#32934=CARTESIAN_POINT('Ctrl Pts',(-16.6485931966349,14.6049905149185,-2.18486861910694)) ;
#32935=CARTESIAN_POINT('Ctrl Pts',(-17.2093610350114,13.9398456805276,-2.16437899105456)) ;
#32936=CARTESIAN_POINT('Ctrl Pts',(-18.1396885637255,12.6943776160362,-2.12806730355967)) ;
#32937=CARTESIAN_POINT('Ctrl Pts',(-18.5241009163116,12.1265502537836,-2.11218709079074)) ;
#32938=CARTESIAN_POINT('Ctrl Pts',(-19.1939231797678,11.0307696365686,-2.08281744373015)) ;
#32939=CARTESIAN_POINT('Ctrl Pts',(-19.4854276896824,10.5072679986121,-2.06928850416174)) ;
#32940=CARTESIAN_POINT('Ctrl Pts',(-20.1051828605012,9.27955487831268,-2.03848164596858)) ;
#32941=CARTESIAN_POINT('Ctrl Pts',(-20.4183165844046,8.56859749036841,-2.02130954992691)) ;
#32942=CARTESIAN_POINT('Ctrl Pts',(-20.8525291489185,7.42289524805143,-1.99397761802501)) ;
#32943=CARTESIAN_POINT('Ctrl Pts',(-20.9988066582684,6.99838983381805,-1.98391622678796)) ;
#32944=CARTESIAN_POINT('Ctrl Pts',(-21.2348329910298,6.23919225199287,-1.96582176560169)) ;
#32945=CARTESIAN_POINT('Ctrl Pts',(-21.3298238849591,5.90628986974985,-1.95784182554096)) ;
#32946=CARTESIAN_POINT('Ctrl Pts',(-21.5416370124958,5.09204642411329,-1.93830305965728)) ;
#32947=CARTESIAN_POINT('Ctrl Pts',(-21.6501856686398,4.60874393128813,-1.92669450677504)) ;
#32948=CARTESIAN_POINT('Ctrl Pts',(-21.9066916395153,3.25581329932268,-1.89442487885326)) ;
#32949=CARTESIAN_POINT('Ctrl Pts',(-22.0190220773615,2.38036714803317,-1.87382822227687)) ;
#32950=CARTESIAN_POINT('Ctrl Pts',(-22.1165872472184,0.944815354558331,
-1.8407901513055)) ;
#32951=CARTESIAN_POINT('Ctrl Pts',(-22.133361451287,0.387846271600151,-1.82814176368577)) ;
#32952=CARTESIAN_POINT('Ctrl Pts',(-22.1231949989612,-0.942071459656081,
-1.79821539165576)) ;
#32953=CARTESIAN_POINT('Ctrl Pts',(-22.0767975374566,-1.71413808165435,
-1.78107391405708)) ;
#32954=CARTESIAN_POINT('Ctrl Pts',(-21.927440800533,-3.03731095775537,-1.75144495311507)) ;
#32955=CARTESIAN_POINT('Ctrl Pts',(-21.8437829605374,-3.58985469157925,
-1.73898936360242)) ;
#32956=CARTESIAN_POINT('Ctrl Pts',(-21.6792430329331,-4.45414533651674,
-1.71902358227166)) ;
#32957=CARTESIAN_POINT('Ctrl Pts',(-21.6123170743208,-4.76830532813321,
-1.71165027570279)) ;
#32958=CARTESIAN_POINT('Ctrl Pts',(-21.3415016515141,-5.91632722744004,
-1.68434114745722)) ;
#32959=CARTESIAN_POINT('Ctrl Pts',(-21.0959858458467,-6.73958475879623,
-1.66411122837106)) ;
#32960=CARTESIAN_POINT('Ctrl Pts',(-20.567158394392,-8.1973927173502,-1.62788027517404)) ;
#32961=CARTESIAN_POINT('Ctrl Pts',(-20.3006232293971,-8.83685239021096,
-1.61183118178125)) ;
#32962=CARTESIAN_POINT('Ctrl Pts',(-19.7496733585932,-10.0015755730293,
-1.58236064140842)) ;
#32963=CARTESIAN_POINT('Ctrl Pts',(-19.4731341546841,-10.5298701360726,
-1.56889347892619)) ;
#32964=CARTESIAN_POINT('Ctrl Pts',(-18.7935015006124,-11.7096586900459,
-1.53838759212057)) ;
#32965=CARTESIAN_POINT('Ctrl Pts',(-18.3772404828784,-12.3526854016887,
-1.52144985819985)) ;
#32966=CARTESIAN_POINT('Ctrl Pts',(-17.6517188554879,-13.3553576573114,
-1.49385264748403)) ;
#32967=CARTESIAN_POINT('Ctrl Pts',(-17.3627695643622,-13.7289105407336,
-1.48327654797979)) ;
#32968=CARTESIAN_POINT('Ctrl Pts',(-16.839231852533,-14.3627495768589,-1.46456053495045)) ;
#32969=CARTESIAN_POINT('Ctrl Pts',(-16.610001756091,-14.6272397022557,-1.45648915640155)) ;
#32970=CARTESIAN_POINT('Ctrl Pts',(-16.0331909849394,-15.2617238358109,
-1.43656888437737)) ;
#32971=CARTESIAN_POINT('Ctrl Pts',(-15.6789654724278,-15.6254109550156,
-1.42466732831652)) ;
#32972=CARTESIAN_POINT('Ctrl Pts',(-14.6937161027081,-16.5697097847477,
-1.39268799087216)) ;
#32973=CARTESIAN_POINT('Ctrl Pts',(-14.0409393043516,-17.1263720344066,
-1.37267590563707)) ;
#32974=CARTESIAN_POINT('Ctrl Pts',(-12.9140564481339,-17.9794982076989,
-1.34021798416833)) ;
#32975=CARTESIAN_POINT('Ctrl Pts',(-12.4580920903304,-18.2983922120309,
-1.32758571610207)) ;
#32976=CARTESIAN_POINT('Ctrl Pts',(-11.3366601677733,-19.0213386412986,
-1.29755783226305)) ;
#32977=CARTESIAN_POINT('Ctrl Pts',(-10.6609471716456,-19.4081270662132,
-1.28030321993197)) ;
#32978=CARTESIAN_POINT('Ctrl Pts',(-9.46720108948631,-20.0102567895931,
-1.25055321400253)) ;
#32979=CARTESIAN_POINT('Ctrl Pts',(-8.95877701813951,-20.2429884253592,
-1.23809034144233)) ;
#32980=CARTESIAN_POINT('Ctrl Pts',(-8.14495636055075,-20.5788446569233,
-1.21811032811782)) ;
#32981=CARTESIAN_POINT('Ctrl Pts',(-7.84518853795099,-20.6949794436523,
-1.21073036990084)) ;
#32982=CARTESIAN_POINT('Ctrl Pts',(-6.72591648848527,-21.1007883412187,
-1.18316442353116)) ;
#32983=CARTESIAN_POINT('Ctrl Pts',(-5.89209133134835,-21.3486412314298,
-1.16267723841777)) ;
#32984=CARTESIAN_POINT('Ctrl Pts',(-4.37851361886198,-21.703092443609,-1.12636644503436)) ;
#32985=CARTESIAN_POINT('Ctrl Pts',(-3.7042683138324,-21.8282846544745,-1.11048478203516)) ;
#32986=CARTESIAN_POINT('Ctrl Pts',(-2.43216842952851,-22.0038381908663,
-1.0811180233647)) ;
#32987=CARTESIAN_POINT('Ctrl Pts',(-1.83595857765317,-22.0615865643175,
-1.06759326658192)) ;
#32988=CARTESIAN_POINT('Ctrl Pts',(-0.825758939772332,-22.1181949647166,
-1.04492861924944)) ;
#32989=CARTESIAN_POINT('Ctrl Pts',(-0.412884428402931,-22.1297499983293,
-1.0357338587638)) ;
#32990=CARTESIAN_POINT('Ctrl Pts',(-8.95436081532752E-8,-22.12975,-1.02655085110559)) ;
#32991=CARTESIAN_POINT('Ctrl Pts',(1.79160500324294E-8,-22.12975,-0.560977995021737)) ;
#32992=CARTESIAN_POINT('Ctrl Pts',(-0.525934233726528,-22.1297500004258,
-0.573296224886261)) ;
#32993=CARTESIAN_POINT('Ctrl Pts',(-1.05174160701657,-22.1110010115208,
-0.585584835713953)) ;
#32994=CARTESIAN_POINT('Ctrl Pts',(-2.14236416750074,-22.0331123011704,
-0.610922730527558)) ;
#32995=CARTESIAN_POINT('Ctrl Pts',(-2.7065473814672,-21.9709437695922,-0.623944376031082)) ;
#32996=CARTESIAN_POINT('Ctrl Pts',(-4.23937387499394,-21.7420951240243,
-0.659141534859372)) ;
#32997=CARTESIAN_POINT('Ctrl Pts',(-5.20028927254187,-21.5324869269799,
-0.680968147911927)) ;
#32998=CARTESIAN_POINT('Ctrl Pts',(-6.57268083743359,-21.1358635940895,
-0.712756985953018)) ;
#32999=CARTESIAN_POINT('Ctrl Pts',(-6.99742249130262,-20.9990699599077,
-0.722693869659368)) ;
#33000=CARTESIAN_POINT('Ctrl Pts',(-7.73067864718106,-20.7381959459378,
-0.740209003861003)) ;
#33001=CARTESIAN_POINT('Ctrl Pts',(-8.04107334303412,-20.6198279101231,
-0.747743458136614)) ;
#33002=CARTESIAN_POINT('Ctrl Pts',(-8.81179954500836,-20.3058633897718,
-0.766857211105509)) ;
#33003=CARTESIAN_POINT('Ctrl Pts',(-9.26838307869553,-20.1015663545691,
-0.778518701035829)) ;
#33004=CARTESIAN_POINT('Ctrl Pts',(-10.3732984113895,-19.5615204702096,
-0.807302275381897)) ;
#33005=CARTESIAN_POINT('Ctrl Pts',(-11.0126962137024,-19.2088243304817,
-0.824444438292544)) ;
#33006=CARTESIAN_POINT('Ctrl Pts',(-12.1304611322545,-18.5180732519022,
-0.854979494902476)) ;
#33007=CARTESIAN_POINT('Ctrl Pts',(-12.6150703659842,-18.1914026816838,
-0.868430106089242)) ;
#33008=CARTESIAN_POINT('Ctrl Pts',(-13.6524660232289,-17.4306943543624,
-0.897719551719603)) ;
#33009=CARTESIAN_POINT('Ctrl Pts',(-14.1986607081937,-16.9887309063024,
-0.913470706192331)) ;
#33010=CARTESIAN_POINT('Ctrl Pts',(-15.363018668484,-15.9511313916318,-0.948224457860342)) ;
#33011=CARTESIAN_POINT('Ctrl Pts',(-15.9694235822837,-15.344003048714,-0.967138713186487)) ;
#33012=CARTESIAN_POINT('Ctrl Pts',(-16.748893478574,-14.4672089660127,-0.993584009925753)) ;
#33013=CARTESIAN_POINT('Ctrl Pts',(-16.9536383825249,-14.2267253122953,
-1.00076556794163)) ;
#33014=CARTESIAN_POINT('Ctrl Pts',(-17.5040650937794,-13.5514568881276,
-1.0208041086825)) ;
#33015=CARTESIAN_POINT('Ctrl Pts',(-17.8386303606473,-13.10791899846,-1.03378431894615)) ;
#33016=CARTESIAN_POINT('Ctrl Pts',(-18.5847678980595,-12.0372028709565,
-1.06435353693008)) ;
#33017=CARTESIAN_POINT('Ctrl Pts',(-18.9818526392715,-11.4007513249138,
-1.08193672320922)) ;
#33018=CARTESIAN_POINT('Ctrl Pts',(-19.6190852117209,-10.253484035639,-1.11234484795959)) ;
#33019=CARTESIAN_POINT('Ctrl Pts',(-19.8734409520661,-9.75134816160269,
-1.12525635915599)) ;
#33020=CARTESIAN_POINT('Ctrl Pts',(-20.5014056720916,-8.38476047681561,
-1.15940775539414)) ;
#33021=CARTESIAN_POINT('Ctrl Pts',(-20.8394579939037,-7.50525444662354,
-1.18033985803072)) ;
#33022=CARTESIAN_POINT('Ctrl Pts',(-21.2598581503898,-6.16134783804295,
-1.21166270583013)) ;
#33023=CARTESIAN_POINT('Ctrl Pts',(-21.3851008125506,-5.71150035202914,
-1.22205022015792)) ;
#33024=CARTESIAN_POINT('Ctrl Pts',(-21.5763229745779,-4.92974082849986,
-1.24014546081878)) ;
#33025=CARTESIAN_POINT('Ctrl Pts',(-21.6490931518115,-4.59965472559595,
-1.24780277003546)) ;
#33026=CARTESIAN_POINT('Ctrl Pts',(-21.7997270967248,-3.83328101800073,
-1.26572608417951)) ;
#33027=CARTESIAN_POINT('Ctrl Pts',(-21.8721029768026,-3.39606429648156,
-1.27603579643099)) ;
#33028=CARTESIAN_POINT('Ctrl Pts',(-22.0342274791183,-2.19361766733191,
-1.30439659115754)) ;
#33029=CARTESIAN_POINT('Ctrl Pts',(-22.0972252640812,-1.42540587648294,
-1.32250772317673)) ;
#33030=CARTESIAN_POINT('Ctrl Pts',(-22.1377192723276,-0.0588754101339896,
-1.35430243779505)) ;
#33031=CARTESIAN_POINT('Ctrl Pts',(-22.1312545947905,0.538199772947654,
-1.36805692004755)) ;
#33032=CARTESIAN_POINT('Ctrl Pts',(-22.065528057541,1.81882994007757,-1.39727310533383)) ;
#33033=CARTESIAN_POINT('Ctrl Pts',(-21.9986091500527,2.50137470790254,-1.41266615438963)) ;
#33034=CARTESIAN_POINT('Ctrl Pts',(-21.7762742344478,4.03269502775326,-1.44717668925988)) ;
#33035=CARTESIAN_POINT('Ctrl Pts',(-21.6027014919803,4.87770663822004,-1.46619325571305)) ;
#33036=CARTESIAN_POINT('Ctrl Pts',(-21.2968947637669,6.02267015428563,-1.49287984762274)) ;
#33037=CARTESIAN_POINT('Ctrl Pts',(-21.206670970756,6.33303944595073,-1.50021806156309)) ;
#33038=CARTESIAN_POINT('Ctrl Pts',(-20.9218571548879,7.23832996013415,-1.5220267101671)) ;
#33039=CARTESIAN_POINT('Ctrl Pts',(-20.7087926045076,7.82709588407729,-1.53667526987314)) ;
#33040=CARTESIAN_POINT('Ctrl Pts',(-20.2192948393412,9.01916079884334,-1.56687112516782)) ;
#33041=CARTESIAN_POINT('Ctrl Pts',(-19.9401075452378,9.62066852641224,-1.58240309376065)) ;
#33042=CARTESIAN_POINT('Ctrl Pts',(-19.3722193991147,10.7128810502313,-1.61095405981049)) ;
#33043=CARTESIAN_POINT('Ctrl Pts',(-19.0907730496586,11.2067433381483,-1.62400700481309)) ;
#33044=CARTESIAN_POINT('Ctrl Pts',(-18.2527961500009,12.5538053119113,-1.66006314438083)) ;
#33045=CARTESIAN_POINT('Ctrl Pts',(-17.6559336417536,13.3802321976155,-1.68267092765148)) ;
#33046=CARTESIAN_POINT('Ctrl Pts',(-16.722694425566,14.5007218651046,-1.71510917494069)) ;
#33047=CARTESIAN_POINT('Ctrl Pts',(-16.4310763896471,14.8303462408771,-1.72490818097374)) ;
#33048=CARTESIAN_POINT('Ctrl Pts',(-15.9041529901443,15.3913093400057,-1.74222597187494)) ;
#33049=CARTESIAN_POINT('Ctrl Pts',(-15.6731395383495,15.6264897734192,-1.74970248122091)) ;
#33050=CARTESIAN_POINT('Ctrl Pts',(-14.9006423455448,16.3785514108231,-1.77446062695326)) ;
#33051=CARTESIAN_POINT('Ctrl Pts',(-14.3381829911038,16.8731321797791,-1.79203078367609)) ;
#33052=CARTESIAN_POINT('Ctrl Pts',(-13.0839306877115,17.8679359134632,-1.82954223027897)) ;
#33053=CARTESIAN_POINT('Ctrl Pts',(-12.3860618412477,18.3585911314175,-1.84943309023077)) ;
#33054=CARTESIAN_POINT('Ctrl Pts',(-11.1867634180766,19.1022080556933,-1.88182551786269)) ;
#33055=CARTESIAN_POINT('Ctrl Pts',(-10.7009131383429,19.3785575509763,-1.89450877185929)) ;
#33056=CARTESIAN_POINT('Ctrl Pts',(-9.52789998562627,19.9881830934131,-1.9242466888764)) ;
#33057=CARTESIAN_POINT('Ctrl Pts',(-8.83292272725293,20.3048718476124,-1.9411733310623)) ;
#33058=CARTESIAN_POINT('Ctrl Pts',(-7.6039256579658,20.7898415854069,-1.97057144166248)) ;
#33059=CARTESIAN_POINT('Ctrl Pts',(-7.07731797239299,20.974955583818,-1.98301221226514)) ;
#33060=CARTESIAN_POINT('Ctrl Pts',(-6.23805127550414,21.2347666678504,-2.00294752040356)) ;
#33061=CARTESIAN_POINT('Ctrl Pts',(-5.92980142995826,21.3228996638014,-2.01030577323518)) ;
#33062=CARTESIAN_POINT('Ctrl Pts',(-4.79050821283295,21.6220236337416,-2.03757436514442)) ;
#33063=CARTESIAN_POINT('Ctrl Pts',(-3.94931768438597,21.7913690612007,-2.0577798501529)) ;
#33064=CARTESIAN_POINT('Ctrl Pts',(-2.4129879761375,22.008756446236,-2.09403330529205)) ;
#33065=CARTESIAN_POINT('Ctrl Pts',(-1.72134697110337,22.0736233514168,-2.11012757794793)) ;
#33066=CARTESIAN_POINT('Ctrl Pts',(-0.433185813950684,22.1335156406398,
-2.13962455197018)) ;
#33067=CARTESIAN_POINT('Ctrl Pts',(0.162303146382963,22.1371594702166,-2.15307465430135)) ;
#33068=CARTESIAN_POINT('Ctrl Pts',(1.51936022008785,22.0906976721499,-2.18349949427501)) ;
#33069=CARTESIAN_POINT('Ctrl Pts',(2.27964448276855,22.0252264327582,-2.20037451130819)) ;
#33070=CARTESIAN_POINT('Ctrl Pts',(3.50678570364562,21.8553222435539,-2.22799575024501)) ;
#33071=CARTESIAN_POINT('Ctrl Pts',(3.97630900291109,21.7747931750443,-2.23866200647971)) ;
#33072=CARTESIAN_POINT('Ctrl Pts',(4.78485058601815,21.6090931435798,-2.25745076839496)) ;
#33073=CARTESIAN_POINT('Ctrl Pts',(5.12512670229219,21.5309259615509,-2.2655014930802)) ;
#33074=CARTESIAN_POINT('Ctrl Pts',(5.9525599736799,21.3201234746012,-2.28533625510541)) ;
#33075=CARTESIAN_POINT('Ctrl Pts',(6.43730444714733,21.1788041412342,-2.29717231584179)) ;
#33076=CARTESIAN_POINT('Ctrl Pts',(7.73623135930551,20.751403406109,-2.32921619425072)) ;
#33077=CARTESIAN_POINT('Ctrl Pts',(8.53921126501607,20.434086979508,-2.34935847370628)) ;
#33078=CARTESIAN_POINT('Ctrl Pts',(9.82623942292865,19.8363410055606,-2.38194566386641)) ;
#33079=CARTESIAN_POINT('Ctrl Pts',(10.3218449881087,19.5830265296391,-2.39458150646353)) ;
#33080=CARTESIAN_POINT('Ctrl Pts',(11.4853755036592,18.9318682280159,-2.42458785176237)) ;
#33081=CARTESIAN_POINT('Ctrl Pts',(12.1429194254384,18.5169920943436,-2.44181832507531)) ;
#33082=CARTESIAN_POINT('Ctrl Pts',(13.233632050842,17.7456816838172,-2.47154335487439)) ;
#33083=CARTESIAN_POINT('Ctrl Pts',(13.6775906966312,17.4057961959282,-2.48400551785132)) ;
#33084=CARTESIAN_POINT('Ctrl Pts',(14.3558842376998,16.844517664891,-2.50398567886508)) ;
#33085=CARTESIAN_POINT('Ctrl Pts',(14.5990675051604,16.6341940420368,-2.51136656529882)) ;
#33086=CARTESIAN_POINT('Ctrl Pts',(15.4824518518825,15.8358770269977,-2.53893470792046)) ;
#33087=CARTESIAN_POINT('Ctrl Pts',(16.0924283562774,15.2156191992287,-2.55942312987066)) ;
#33088=CARTESIAN_POINT('Ctrl Pts',(17.1153048252688,14.0449957290865,-2.59573437156419)) ;
#33089=CARTESIAN_POINT('Ctrl Pts',(17.5420514525484,13.5082199677597,-2.61161529381933)) ;
#33090=CARTESIAN_POINT('Ctrl Pts',(18.2937098202633,12.4669420185057,-2.64098365630942)) ;
#33091=CARTESIAN_POINT('Ctrl Pts',(18.6243656518279,11.9673503159477,-2.65451067440508)) ;
#33092=CARTESIAN_POINT('Ctrl Pts',(19.3360586677326,10.7909651494682,-2.68530952231401)) ;
#33093=CARTESIAN_POINT('Ctrl Pts',(19.7025582832172,10.1062994845046,-2.70247564262063)) ;
#33094=CARTESIAN_POINT('Ctrl Pts',(20.2231451795239,8.99732542747596,-2.72980405391132)) ;
#33095=CARTESIAN_POINT('Ctrl Pts',(20.4015402034208,8.58513941034812,-2.73986820441059)) ;
#33096=CARTESIAN_POINT('Ctrl Pts',(20.6949003878055,7.84643286970198,-2.75795728854641)) ;
#33097=CARTESIAN_POINT('Ctrl Pts',(20.8149780378034,7.52210708541269,-2.76592888200795)) ;
#33098=CARTESIAN_POINT('Ctrl Pts',(21.0880550767143,6.72784565895061,-2.78543345294672)) ;
#33099=CARTESIAN_POINT('Ctrl Pts',(21.233010006295,6.25533838774175,-2.79701589963105)) ;
#33100=CARTESIAN_POINT('Ctrl Pts',(21.5928764928195,4.92495147678466,-2.82931303748762)) ;
#33101=CARTESIAN_POINT('Ctrl Pts',(21.7723781672084,4.05845211560372,-2.84996349285406)) ;
#33102=CARTESIAN_POINT('Ctrl Pts',(21.9797079555187,2.63223045739763,-2.88305511207917)) ;
#33103=CARTESIAN_POINT('Ctrl Pts',(22.0390051115066,2.07809023695964,-2.89570517479943)) ;
#33104=CARTESIAN_POINT('Ctrl Pts',(22.1304645660627,0.751690054509215,-2.92562200915772)) ;
#33105=CARTESIAN_POINT('Ctrl Pts',(22.1432169020043,-0.0211741976199246,
-2.94275270633856)) ;
#33106=CARTESIAN_POINT('Ctrl Pts',(22.0955115780757,-1.35139852307501,-2.97237069737913)) ;
#33107=CARTESIAN_POINT('Ctrl Pts',(22.0543580756396,-1.90871489643176,-2.98482615231563)) ;
#33108=CARTESIAN_POINT('Ctrl Pts',(21.9563973499803,-2.78309808608486,-3.00479286697957)) ;
#33109=CARTESIAN_POINT('Ctrl Pts',(21.9136873453836,-3.1015032382929,-3.01216727806539)) ;
#33110=CARTESIAN_POINT('Ctrl Pts',(21.7314428907408,-4.26697937008732,-3.03947891539823)) ;
#33111=CARTESIAN_POINT('Ctrl Pts',(21.549588235056,-5.10665946494792,-3.05971017258317)) ;
#33112=CARTESIAN_POINT('Ctrl Pts',(21.1337930212615,-6.60059902190559,-3.09593993820866)) ;
#33113=CARTESIAN_POINT('Ctrl Pts',(20.9169708439003,-7.25847487490876,-3.11198659951746)) ;
#33114=CARTESIAN_POINT('Ctrl Pts',(20.4567085292055,-8.46193351282878,-3.14145720880366)) ;
#33115=CARTESIAN_POINT('Ctrl Pts',(20.2213356776939,-9.00992970070769,-3.154926741026)) ;
#33116=CARTESIAN_POINT('Ctrl Pts',(19.6337100633174,-10.2386404994311,-3.18544255027454)) ;
#33117=CARTESIAN_POINT('Ctrl Pts',(19.2676571059666,-10.9119072056271,-3.20238769200689)) ;
#33118=CARTESIAN_POINT('Ctrl Pts',(18.6209405410612,-11.9669919833376,-3.22998262841657)) ;
#33119=CARTESIAN_POINT('Ctrl Pts',(18.3616471611248,-12.3611582053818,-3.24054865479097)) ;
#33120=CARTESIAN_POINT('Ctrl Pts',(17.8883871663665,-13.0328011158217,-3.25925418653295)) ;
#33121=CARTESIAN_POINT('Ctrl Pts',(17.6800607603497,-13.3140432139573,-3.26732546995719)) ;
#33122=CARTESIAN_POINT('Ctrl Pts',(17.1534578336099,-13.9907945288812,-3.28724616389628)) ;
#33123=CARTESIAN_POINT('Ctrl Pts',(16.8280722996134,-14.3805225244584,-3.29914825048019)) ;
#33124=CARTESIAN_POINT('Ctrl Pts',(15.9179591311133,-15.3973711363029,-3.33112665991972)) ;
#33125=CARTESIAN_POINT('Ctrl Pts',(15.3097173060681,-16.0022822486626,-3.35113728810968)) ;
#33126=CARTESIAN_POINT('Ctrl Pts',(14.2515089346783,-16.9389964188399,-3.38359171297152)) ;
#33127=CARTESIAN_POINT('Ctrl Pts',(13.8213458646886,-17.2917758315769,-3.39622195410535)) ;
#33128=CARTESIAN_POINT('Ctrl Pts',(12.7584059189391,-18.0984697061888,-3.42625283502378)) ;
#33129=CARTESIAN_POINT('Ctrl Pts',(12.1140750641772,-18.5359304052641,-3.44351224388142)) ;
#33130=CARTESIAN_POINT('Ctrl Pts',(10.9696712017121,-19.2277040358139,-3.47326739064209)) ;
#33131=CARTESIAN_POINT('Ctrl Pts',(10.480520705525,-19.4986401396969,-3.48573057414477)) ;
#33132=CARTESIAN_POINT('Ctrl Pts',(9.69470631030959,-19.8957750505562,-3.50571216183121)) ;
#33133=CARTESIAN_POINT('Ctrl Pts',(9.40464904100198,-20.0345144078224,-3.51309337529043)) ;
#33134=CARTESIAN_POINT('Ctrl Pts',(8.31952684369476,-20.524787457452,-3.54066337858747)) ;
#33135=CARTESIAN_POINT('Ctrl Pts',(7.50698066475757,-20.8357066076486,-3.56115331180284)) ;
#33136=CARTESIAN_POINT('Ctrl Pts',(6.02489615056135,-21.3048377995494,-3.59746461967355)) ;
#33137=CARTESIAN_POINT('Ctrl Pts',(5.36227712727311,-21.4811890468595,-3.61334417286704)) ;
#33138=CARTESIAN_POINT('Ctrl Pts',(4.1960747363392,-21.7342328013673,-3.64063391776006)) ;
#33139=CARTESIAN_POINT('Ctrl Pts',(3.69604415758763,-21.8248294584951,-3.65213300120995)) ;
#33140=CARTESIAN_POINT('Ctrl Pts',(2.13577037616094,-22.0523593330427,-3.68754652786183)) ;
#33141=CARTESIAN_POINT('Ctrl Pts',(1.06842946296467,-22.129765004344,-3.71104938457161)) ;
#33142=CARTESIAN_POINT('Ctrl Pts',(-0.000310730952457761,-22.1297499978185,
-3.73504649578496)) ;
#33143=CARTESIAN_POINT('Origin',(0.,0.,-10.)) ;
#33144=CARTESIAN_POINT('',(-4.10971426655051E-9,-22.12975,-7.37565036637909)) ;
#33145=CARTESIAN_POINT('',(-0.00028260616734981,-22.1297499981955,-6.91183148751772)) ;
#33146=CARTESIAN_POINT('',(-2.71011275034311E-15,-22.12975,-10.)) ;
#33147=CARTESIAN_POINT('Ctrl Pts',(-4.1097096559195E-9,-22.12975,-7.37565036637909)) ;
#33148=CARTESIAN_POINT('Ctrl Pts',(0.496307662068902,-22.1297500000922,
-7.36418082185928)) ;
#33149=CARTESIAN_POINT('Ctrl Pts',(0.992494088983844,-22.1130538540768,
-7.35281336153108)) ;
#33150=CARTESIAN_POINT('Ctrl Pts',(2.36728846219153,-22.0204209047268,-7.32154322916872)) ;
#33151=CARTESIAN_POINT('Ctrl Pts',(3.24253230519655,-21.9086509499698,-7.3019184235776)) ;
#33152=CARTESIAN_POINT('Ctrl Pts',(4.59550185240573,-21.6530034652559,-7.27130069620706)) ;
#33153=CARTESIAN_POINT('Ctrl Pts',(5.0790022644443,-21.544719292526,-7.26029312857459)) ;
#33154=CARTESIAN_POINT('Ctrl Pts',(5.89354108416853,-21.3333506313142,-7.241394104392)) ;
#33155=CARTESIAN_POINT('Ctrl Pts',(6.22653636982164,-21.2385479855221,-7.23356203120506)) ;
#33156=CARTESIAN_POINT('Ctrl Pts',(6.98587369482261,-21.0029731010004,-7.21533578284537)) ;
#33157=CARTESIAN_POINT('Ctrl Pts',(7.41042930664819,-20.8569615256471,-7.20489586716275)) ;
#33158=CARTESIAN_POINT('Ctrl Pts',(8.55641784940482,-20.4234262497798,-7.17626174148924)) ;
#33159=CARTESIAN_POINT('Ctrl Pts',(9.26763108493787,-20.1106849090278,-7.15800347887808)) ;
#33160=CARTESIAN_POINT('Ctrl Pts',(10.4957909943736,-19.491612650642,-7.12601334926235)) ;
#33161=CARTESIAN_POINT('Ctrl Pts',(11.0194841439878,-19.2004054548611,-7.11220861145816)) ;
#33162=CARTESIAN_POINT('Ctrl Pts',(12.1156566581831,-18.5312265814932,-7.08294433729836)) ;
#33163=CARTESIAN_POINT('Ctrl Pts',(12.6836913137425,-18.1471617251315,-7.06755216845237)) ;
#33164=CARTESIAN_POINT('Ctrl Pts',(13.9297080673345,-17.217568480866,-7.0328764797819)) ;
#33165=CARTESIAN_POINT('Ctrl Pts',(14.5951913428042,-16.6571847938103,-7.01369812697652)) ;
#33166=CARTESIAN_POINT('Ctrl Pts',(15.4592835098897,-15.8379211434953,-6.98687201777148)) ;
#33167=CARTESIAN_POINT('Ctrl Pts',(15.6877333883636,-15.6116691522672,-6.97956769369083)) ;
#33168=CARTESIAN_POINT('Ctrl Pts',(16.2996722163591,-14.9786172301129,-6.95932600226643)) ;
#33169=CARTESIAN_POINT('Ctrl Pts',(16.6728003485183,-14.5621431061368,-6.94626356423777)) ;
#33170=CARTESIAN_POINT('Ctrl Pts',(17.5267634254894,-13.5330748793806,-6.91494121500932)) ;
#33171=CARTESIAN_POINT('Ctrl Pts',(17.9918313774377,-12.9083525963353,-6.89668664815354)) ;
#33172=CARTESIAN_POINT('Ctrl Pts',(18.7311247176936,-11.7974603535927,-6.86579235779266)) ;
#33173=CARTESIAN_POINT('Ctrl Pts',(19.0216689555042,-11.3230393780551,-6.85304258236847)) ;
#33174=CARTESIAN_POINT('Ctrl Pts',(19.7137627574503,-10.0909795027729,-6.82097761216475)) ;
#33175=CARTESIAN_POINT('Ctrl Pts',(20.0897321840658,-9.32003114857441,-6.80188898968452)) ;
#33176=CARTESIAN_POINT('Ctrl Pts',(20.6156840630731,-8.06083537101872,-6.77154387662993)) ;
#33177=CARTESIAN_POINT('Ctrl Pts',(20.7951499715355,-7.585857294535,-6.76026821908286)) ;
#33178=CARTESIAN_POINT('Ctrl Pts',(21.070485255523,-6.77369620850567,-6.74101557182124)) ;
#33179=CARTESIAN_POINT('Ctrl Pts',(21.1749689073444,-6.43964291964075,-6.73310155986182)) ;
#33180=CARTESIAN_POINT('Ctrl Pts',(21.4015739580845,-5.64986301072583,-6.71427114495625)) ;
#33181=CARTESIAN_POINT('Ctrl Pts',(21.5171318797554,-5.19243212120798,-6.70329477168496)) ;
#33182=CARTESIAN_POINT('Ctrl Pts',(21.7817285490791,-3.98354462693207,-6.67436353817122)) ;
#33183=CARTESIAN_POINT('Ctrl Pts',(21.9065295868642,-3.22742855079625,-6.65635871501739)) ;
#33184=CARTESIAN_POINT('Ctrl Pts',(22.0583243522427,-1.87391891094637,-6.62468616832486)) ;
#33185=CARTESIAN_POINT('Ctrl Pts',(22.1007997555033,-1.27902442930549,-6.61094933754796)) ;
#33186=CARTESIAN_POINT('Ctrl Pts',(22.1405753799507,0.0088617248840879,
-6.58159446988023)) ;
#33187=CARTESIAN_POINT('Ctrl Pts',(22.1294618825395,0.70148611629901,-6.56605026013672)) ;
#33188=CARTESIAN_POINT('Ctrl Pts',(22.0318851110312,2.24916708245715,-6.53146751218405)) ;
#33189=CARTESIAN_POINT('Ctrl Pts',(21.9280696632736,3.10200898704139,-6.51252370818853)) ;
#33190=CARTESIAN_POINT('Ctrl Pts',(21.7176951362174,4.26271362501853,-6.48594668174259)) ;
#33191=CARTESIAN_POINT('Ctrl Pts',(21.6535369038551,4.57748280302964,-6.47864830219849)) ;
#33192=CARTESIAN_POINT('Ctrl Pts',(21.4590877363213,5.43557422771732,-6.45841988997357)) ;
#33193=CARTESIAN_POINT('Ctrl Pts',(21.3150409195593,5.97552835276067,-6.44536509524797)) ;
#33194=CARTESIAN_POINT('Ctrl Pts',(20.9234355198276,7.24794560222024,-6.41418160461128)) ;
#33195=CARTESIAN_POINT('Ctrl Pts',(20.6576290839189,7.97403542187047,-6.39605827537518)) ;
#33196=CARTESIAN_POINT('Ctrl Pts',(20.1357787940604,9.1970947982472,-6.36526698125948)) ;
#33197=CARTESIAN_POINT('Ctrl Pts',(19.8978977926689,9.70102110404991,-6.35249349192216)) ;
#33198=CARTESIAN_POINT('Ctrl Pts',(19.2343249103643,10.9793777858995,-6.31980670403162)) ;
#33199=CARTESIAN_POINT('Ctrl Pts',(18.7808252719957,11.7382538801348,-6.30014479502846)) ;
#33200=CARTESIAN_POINT('Ctrl Pts',(18.0045800719058,12.8765471936912,-6.26950781340728)) ;
#33201=CARTESIAN_POINT('Ctrl Pts',(17.7123583162599,13.2756442831883,-6.25851846716267)) ;
#33202=CARTESIAN_POINT('Ctrl Pts',(17.1934144354014,13.9367140277936,-6.2396434699741)) ;
#33203=CARTESIAN_POINT('Ctrl Pts',(16.973464371159,14.2037672860175,-6.23181695621271)) ;
#33204=CARTESIAN_POINT('Ctrl Pts',(16.4538468090212,14.8053490809352,-6.2135929915005)) ;
#33205=CARTESIAN_POINT('Ctrl Pts',(16.1500766897881,15.1361307924852,-6.20314963370124)) ;
#33206=CARTESIAN_POINT('Ctrl Pts',(15.2943390582676,16.0128511005082,-6.17451825355095)) ;
#33207=CARTESIAN_POINT('Ctrl Pts',(14.7233751830527,16.5393602674812,-6.15626645606375)) ;
#33208=CARTESIAN_POINT('Ctrl Pts',(13.6649254194284,17.4170697981906,-6.12428441983908)) ;
#33209=CARTESIAN_POINT('Ctrl Pts',(13.1885863196782,17.7804866657199,-6.11048140676089)) ;
#33210=CARTESIAN_POINT('Ctrl Pts',(12.1366814230179,18.5174699092258,-6.08121501655037)) ;
#33211=CARTESIAN_POINT('Ctrl Pts',(11.5572971722019,18.8845073810979,-6.06581916463472)) ;
#33212=CARTESIAN_POINT('Ctrl Pts',(10.2067746205897,19.6545929170521,-6.0311419360206)) ;
#33213=CARTESIAN_POINT('Ctrl Pts',(9.42703538156276,20.0402659451474,-6.01196556578956)) ;
#33214=CARTESIAN_POINT('Ctrl Pts',(8.33063323822664,20.5043826648788,-5.98514246771099)) ;
#33215=CARTESIAN_POINT('Ctrl Pts',(8.0319316418891,20.6232207114201,-5.97783925186562)) ;
#33216=CARTESIAN_POINT('Ctrl Pts',(7.20704314787377,20.9307608265602,-5.95760001351314)) ;
#33217=CARTESIAN_POINT('Ctrl Pts',(6.67613558175924,21.1060993134591,-5.94453897697726)) ;
#33218=CARTESIAN_POINT('Ctrl Pts',(5.39243676892041,21.4767677489006,-5.91324250950174)) ;
#33219=CARTESIAN_POINT('Ctrl Pts',(4.63486479183454,21.6528974215475,-5.89501242673719)) ;
#33220=CARTESIAN_POINT('Ctrl Pts',(3.32187853024127,21.8860781630063,-5.86413740758064)) ;
#33221=CARTESIAN_POINT('Ctrl Pts',(2.7706830842171,21.962664141789,-5.85138326708829)) ;
#33222=CARTESIAN_POINT('Ctrl Pts',(1.35935766125119,22.1047803025969,-5.81919659312306)) ;
#33223=CARTESIAN_POINT('Ctrl Pts',(0.497213970667352,22.1409564892583,-5.79999541863384)) ;
#33224=CARTESIAN_POINT('Ctrl Pts',(-0.869765365137659,22.1184167863385,
-5.76959400497232)) ;
#33225=CARTESIAN_POINT('Ctrl Pts',(-1.37425526351653,22.0928104228207,-5.75837541604237)) ;
#33226=CARTESIAN_POINT('Ctrl Pts',(-2.22532353515171,22.0203469842369,-5.73919805579457)) ;
#33227=CARTESIAN_POINT('Ctrl Pts',(-2.57247240361083,21.9824960327275,-5.73130150126133)) ;
#33228=CARTESIAN_POINT('Ctrl Pts',(-3.39048648996683,21.8736616525,-5.71238792003792)) ;
#33229=CARTESIAN_POINT('Ctrl Pts',(-3.86024194050749,21.7956647192008,-5.70130768513868)) ;
#33230=CARTESIAN_POINT('Ctrl Pts',(-5.07516058635754,21.553431296399,-5.67234246688728)) ;
#33231=CARTESIAN_POINT('Ctrl Pts',(-5.81500044892733,21.3657069296551,-5.65441091981165)) ;
#33232=CARTESIAN_POINT('Ctrl Pts',(-7.11239366019708,20.9641153432611,-5.62283031380103)) ;
#33233=CARTESIAN_POINT('Ctrl Pts',(-7.67378713261747,20.7651938283145,-5.60911322905975)) ;
#33234=CARTESIAN_POINT('Ctrl Pts',(-8.87121184191377,20.2857035967481,-5.57972901047383)) ;
#33235=CARTESIAN_POINT('Ctrl Pts',(-9.50343639164586,19.9973217219708,-5.56413768632299)) ;
#33236=CARTESIAN_POINT('Ctrl Pts',(-10.8834548708722,19.2875928238917,-5.52953331972418)) ;
#33237=CARTESIAN_POINT('Ctrl Pts',(-11.622421315353,18.8515287006678,-5.51061311864944)) ;
#33238=CARTESIAN_POINT('Ctrl Pts',(-12.6003643592225,18.1950379619678,-5.48407232833942)) ;
#33239=CARTESIAN_POINT('Ctrl Pts',(-12.862592167643,18.0106166160129,-5.47678759398956)) ;
#33240=CARTESIAN_POINT('Ctrl Pts',(-13.5699219315696,17.4898317486615,-5.45659083669298)) ;
#33241=CARTESIAN_POINT('Ctrl Pts',(-14.0064521933666,17.1422369503527,-5.4435548060097)) ;
#33242=CARTESIAN_POINT('Ctrl Pts',(-15.0056425929214,16.2829421350354,-5.41268607960386)) ;
#33243=CARTESIAN_POINT('Ctrl Pts',(-15.5559945043242,15.7579998521014,-5.39485881886433)) ;
#33244=CARTESIAN_POINT('Ctrl Pts',(-16.4625323791601,14.7994475512052,-5.36429728057912)) ;
#33245=CARTESIAN_POINT('Ctrl Pts',(-16.8312789717815,14.3786882247092,-5.35146753515695)) ;
#33246=CARTESIAN_POINT('Ctrl Pts',(-17.7736061901449,13.2174587601229,-5.31751744471359)) ;
#33247=CARTESIAN_POINT('Ctrl Pts',(-18.3167964616073,12.4538055017185,-5.29670184885839)) ;
#33248=CARTESIAN_POINT('Ctrl Pts',(-19.1658170571993,11.0839305286475,-5.2608621650526)) ;
#33249=CARTESIAN_POINT('Ctrl Pts',(-19.4951700657963,10.4938263225175,-5.24584525929691)) ;
#33250=CARTESIAN_POINT('Ctrl Pts',(-19.9462060966197,9.59094087082683,-5.22290208766585)) ;
#33251=CARTESIAN_POINT('Ctrl Pts',(-20.0886174380408,9.28895736846857,-5.21521891004722)) ;
#33252=CARTESIAN_POINT('Ctrl Pts',(-20.408764658061,8.56825437477137,-5.19692776974995)) ;
#33253=CARTESIAN_POINT('Ctrl Pts',(-20.5805318657076,8.14704634224766,-5.18628036926511)) ;
#33254=CARTESIAN_POINT('Ctrl Pts',(-21.0542000353278,6.87471208972843,-5.15446774294738)) ;
#33255=CARTESIAN_POINT('Ctrl Pts',(-21.317126839163,6.01008580146231,-5.13333791591706)) ;
#33256=CARTESIAN_POINT('Ctrl Pts',(-21.6537142677631,4.59819814478098,-5.09995067199544)) ;
#33257=CARTESIAN_POINT('Ctrl Pts',(-21.7610413984736,4.06003093786366,-5.08746704218324)) ;
#33258=CARTESIAN_POINT('Ctrl Pts',(-21.8955651861364,3.22468367392709,-5.06839162574475)) ;
#33259=CARTESIAN_POINT('Ctrl Pts',(-21.9369411081335,2.93001283100947,-5.06171867725492)) ;
#33260=CARTESIAN_POINT('Ctrl Pts',(-22.1041604726886,1.5354144236028,-5.030326132673)) ;
#33261=CARTESIAN_POINT('Ctrl Pts',(-22.1532900175718,0.427903943387989,
-5.00602798842732)) ;
#33262=CARTESIAN_POINT('Ctrl Pts',(-22.1093034917611,-1.00584028333761,
-4.97344579562935)) ;
#33263=CARTESIAN_POINT('Ctrl Pts',(-22.0920041376088,-1.332803124651,-4.96591970733462)) ;
#33264=CARTESIAN_POINT('Ctrl Pts',(-22.0350296168648,-2.09054069118996,
-4.94830950104404)) ;
#33265=CARTESIAN_POINT('Ctrl Pts',(-21.9899651334064,-2.52077807973778,
-4.93819215488364)) ;
#33266=CARTESIAN_POINT('Ctrl Pts',(-21.8000951345113,-3.93268105860742,
-4.90481740402699)) ;
#33267=CARTESIAN_POINT('Ctrl Pts',(-21.6018937209033,-4.90595017565772,
-4.88158485777349)) ;
#33268=CARTESIAN_POINT('Ctrl Pts',(-21.1915603818775,-6.39949874262833,
-4.8460189891286)) ;
#33269=CARTESIAN_POINT('Ctrl Pts',(-21.0238549325764,-6.93060933036597,
-4.83337592406703)) ;
#33270=CARTESIAN_POINT('Ctrl Pts',(-20.5754212068982,-8.18398417888593,
-4.80342069968414)) ;
#33271=CARTESIAN_POINT('Ctrl Pts',(-20.276450118227,-8.89893975599737,-4.78624636284093)) ;
#33272=CARTESIAN_POINT('Ctrl Pts',(-19.6983124091077,-10.1002237895192,
-4.75658201191927)) ;
#33273=CARTESIAN_POINT('Ctrl Pts',(-19.4370276470082,-10.5943372339023,
-4.74412407811697)) ;
#33274=CARTESIAN_POINT('Ctrl Pts',(-18.9964856135211,-11.356170213598,-4.72415289309478)) ;
#33275=CARTESIAN_POINT('Ctrl Pts',(-18.829609516084,-11.6307724984423,-4.71677660961995)) ;
#33276=CARTESIAN_POINT('Ctrl Pts',(-18.1950720849967,-12.6254627434472,
-4.68945967525079)) ;
#33277=CARTESIAN_POINT('Ctrl Pts',(-17.6915982245896,-13.321798334969,-4.66922513240996)) ;
#33278=CARTESIAN_POINT('Ctrl Pts',(-16.7115399382497,-14.5234014778031,
-4.63299849398948)) ;
#33279=CARTESIAN_POINT('Ctrl Pts',(-16.2492167693292,-15.0388737558885,
-4.61695800463579)) ;
#33280=CARTESIAN_POINT('Ctrl Pts',(-15.3450027077108,-15.95657444771,-4.58749093006662)) ;
#33281=CARTESIAN_POINT('Ctrl Pts',(-14.9095098421141,-16.3642262161272,
-4.5740189923709)) ;
#33282=CARTESIAN_POINT('Ctrl Pts',(-13.8779849385705,-17.2544051054192,
-4.54349167000361)) ;
#33283=CARTESIAN_POINT('Ctrl Pts',(-13.27227759947,-17.7245481716059,-4.52653760212552)) ;
#33284=CARTESIAN_POINT('Ctrl Pts',(-12.2567679246685,-18.4314787636057,
-4.49894613495367)) ;
#33285=CARTESIAN_POINT('Ctrl Pts',(-11.8616335650097,-18.6882158977968,
-4.48839300048637)) ;
#33286=CARTESIAN_POINT('Ctrl Pts',(-11.1591150946941,-19.1134125849576,
-4.46969774468818)) ;
#33287=CARTESIAN_POINT('Ctrl Pts',(-10.8553644412281,-19.2875464494945,
-4.46162338153668)) ;
#33288=CARTESIAN_POINT('Ctrl Pts',(-10.1010577457714,-19.696509781283,-4.44168992650591)) ;
#33289=CARTESIAN_POINT('Ctrl Pts',(-9.64629823566461,-19.9231722799568,
-4.42977806295117)) ;
#33290=CARTESIAN_POINT('Ctrl Pts',(-8.4050733846082,-20.4893586613698,-4.39780899839229)) ;
#33291=CARTESIAN_POINT('Ctrl Pts',(-7.60602734897138,-20.7992174182761,
-4.37781751014594)) ;
#33292=CARTESIAN_POINT('Ctrl Pts',(-6.26177191280288,-21.2326468107708,
-4.34538208168149)) ;
#33293=CARTESIAN_POINT('Ctrl Pts',(-5.72626080505905,-21.3832883719748,
-4.33275235569584)) ;
#33294=CARTESIAN_POINT('Ctrl Pts',(-4.42889046591634,-21.6960067771973,
-4.30271824734036)) ;
#33295=CARTESIAN_POINT('Ctrl Pts',(-3.66304172562807,-21.8383586724143,
-4.2854552403341)) ;
#33296=CARTESIAN_POINT('Ctrl Pts',(-2.33709354084746,-22.0130936651908,
-4.25569627073051)) ;
#33297=CARTESIAN_POINT('Ctrl Pts',(-1.78033510003659,-22.0651013742485,
-4.24323288237793)) ;
#33298=CARTESIAN_POINT('Ctrl Pts',(-0.901198406149303,-22.1137296775406,
-4.22325094299919)) ;
#33299=CARTESIAN_POINT('Ctrl Pts',(-0.57984253157056,-22.1244881814877,
-4.21586959248389)) ;
#33300=CARTESIAN_POINT('Ctrl Pts',(-0.172242706946389,-22.1292473028186,
-4.2064314930422)) ;
#33301=CARTESIAN_POINT('Ctrl Pts',(-0.0861183909271938,-22.1297499999265,
-4.20443332226111)) ;
#33302=CARTESIAN_POINT('Ctrl Pts',(-1.88975816071502E-8,-22.12975,-4.20243196305312)) ;
#33303=CARTESIAN_POINT('Ctrl Pts',(-0.000310769958409111,-22.1297499978179,
-3.73504649666078)) ;
#33304=CARTESIAN_POINT('Ctrl Pts',(-0.200541522835967,-22.1297471859604,
-3.73954240658829)) ;
#33305=CARTESIAN_POINT('Ctrl Pts',(-0.400762522146849,-22.1270268313811,
-3.74405692376472)) ;
#33306=CARTESIAN_POINT('Ctrl Pts',(-0.768716641826934,-22.1170316004905,
-3.75240859043868)) ;
#33307=CARTESIAN_POINT('Ctrl Pts',(-0.936456061890543,-22.1105644872954,
-3.75623821292539)) ;
#33308=CARTESIAN_POINT('Ctrl Pts',(-1.66817341771166,-22.0740118210972,
-3.77305255713291)) ;
#33309=CARTESIAN_POINT('Ctrl Pts',(-2.23095253771463,-22.0242513029601,
-3.78624144779857)) ;
#33310=CARTESIAN_POINT('Ctrl Pts',(-3.60621661434526,-21.8493939245641,
-3.81870716164814)) ;
#33311=CARTESIAN_POINT('Ctrl Pts',(-4.41482808983057,-21.7004635809194,
-3.83798398665093)) ;
#33312=CARTESIAN_POINT('Ctrl Pts',(-5.73102840938846,-21.3814161944027,
-3.86931673964317)) ;
#33313=CARTESIAN_POINT('Ctrl Pts',(-6.24407438572413,-21.2372593807404,
-3.88152544266926)) ;
#33314=CARTESIAN_POINT('Ctrl Pts',(-7.57468034409793,-20.8109915072469,
-3.9132304516488)) ;
#33315=CARTESIAN_POINT('Ctrl Pts',(-8.38178044918709,-20.4992418609031,
-3.93248203484719)) ;
#33316=CARTESIAN_POINT('Ctrl Pts',(-9.62712771118747,-19.9323378242688,
-3.96290880854848)) ;
#33317=CARTESIAN_POINT('Ctrl Pts',(-10.0784171780189,-19.7079979522517,
-3.97410195993235)) ;
#33318=CARTESIAN_POINT('Ctrl Pts',(-10.8285062145454,-19.3026150680927,
-3.99324575402595)) ;
#33319=CARTESIAN_POINT('Ctrl Pts',(-11.1313945415384,-19.1295465400972,
-4.00113451966606)) ;
#33320=CARTESIAN_POINT('Ctrl Pts',(-11.8394751691021,-18.7024400557531,
-4.02008756982268)) ;
#33321=CARTESIAN_POINT('Ctrl Pts',(-12.240772292093,-18.4422863452518,-4.03121658323939)) ;
#33322=CARTESIAN_POINT('Ctrl Pts',(-13.258423038794,-17.7347035692855,-4.06019809312191)) ;
#33323=CARTESIAN_POINT('Ctrl Pts',(-13.8606777930296,-17.2680951606565,
-4.07809559863234)) ;
#33324=CARTESIAN_POINT('Ctrl Pts',(-14.8885916697527,-16.3832128387353,
-4.10963347141587)) ;
#33325=CARTESIAN_POINT('Ctrl Pts',(-15.3236639289168,-15.9770196403791,
-4.12334136308469)) ;
#33326=CARTESIAN_POINT('Ctrl Pts',(-16.2306949339859,-15.059022136013,-4.15273972809553)) ;
#33327=CARTESIAN_POINT('Ctrl Pts',(-16.6959532686593,-14.5414840903016,
-4.16835345192879)) ;
#33328=CARTESIAN_POINT('Ctrl Pts',(-17.6782179986661,-13.3394357884123,
-4.2029682176775)) ;
#33329=CARTESIAN_POINT('Ctrl Pts',(-18.1813772124013,-12.6450561919917,
-4.22187730826934)) ;
#33330=CARTESIAN_POINT('Ctrl Pts',(-18.8155515565008,-11.653472146878,-4.24840115225942)) ;
#33331=CARTESIAN_POINT('Ctrl Pts',(-18.9822182306007,-11.3799729444245,
-4.25567957345567)) ;
#33332=CARTESIAN_POINT('Ctrl Pts',(-19.4225573565425,-10.6207724804839,
-4.27586109499909)) ;
#33333=CARTESIAN_POINT('Ctrl Pts',(-19.6839032677579,-10.1282026736812,
-4.28888783124412)) ;
#33334=CARTESIAN_POINT('Ctrl Pts',(-20.2673658974562,-8.92043861104602,
-4.32030592670864)) ;
#33335=CARTESIAN_POINT('Ctrl Pts',(-20.5706158135332,-8.19695809928377,
-4.33869147029722)) ;
#33336=CARTESIAN_POINT('Ctrl Pts',(-21.021834729172,-6.93657721917457,-4.36967795612505)) ;
#33337=CARTESIAN_POINT('Ctrl Pts',(-21.1891242913723,-6.40739082956183,
-4.38239397725943)) ;
#33338=CARTESIAN_POINT('Ctrl Pts',(-21.5505913360704,-5.09407958436841,
-4.41329471133959)) ;
#33339=CARTESIAN_POINT('Ctrl Pts',(-21.7220754018432,-4.30454222400385,
-4.43129698086119)) ;
#33340=CARTESIAN_POINT('Ctrl Pts',(-21.9346704254269,-2.98014012052194,
-4.46112880058563)) ;
#33341=CARTESIAN_POINT('Ctrl Pts',(-22.0001941963648,-2.44999059466151,
-4.47298184936933)) ;
#33342=CARTESIAN_POINT('Ctrl Pts',(-22.0775121595318,-1.56125497948422,
-4.49299584415311)) ;
#33343=CARTESIAN_POINT('Ctrl Pts',(-22.0998842892926,-1.20381656046676,
-4.50108622449457)) ;
#33344=CARTESIAN_POINT('Ctrl Pts',(-22.1317623476045,-0.37055021076278,
-4.52018548448845)) ;
#33345=CARTESIAN_POINT('Ctrl Pts',(-22.1346133513152,0.105353776105306,
-4.53125492860899)) ;
#33346=CARTESIAN_POINT('Ctrl Pts',(-22.1019459321339,1.34924782320897,-4.56034283612349)) ;
#33347=CARTESIAN_POINT('Ctrl Pts',(-22.0417613568237,2.11595065717036,-4.57841263321092)) ;
#33348=CARTESIAN_POINT('Ctrl Pts',(-21.8641885173178,3.469778717009,-4.61016664978308)) ;
#33349=CARTESIAN_POINT('Ctrl Pts',(-21.7626520881668,4.05821216683142,-4.62392093804273)) ;
#33350=CARTESIAN_POINT('Ctrl Pts',(-21.4926247252075,5.31692106606395,-4.65325094552115)) ;
#33351=CARTESIAN_POINT('Ctrl Pts',(-21.3162817870169,5.98487320121514,-4.66875455218612)) ;
#33352=CARTESIAN_POINT('Ctrl Pts',(-20.8510098801605,7.46322647123125,-4.70331895447133)) ;
#33353=CARTESIAN_POINT('Ctrl Pts',(-20.5454905604847,8.26723441600469,-4.72228336145066)) ;
#33354=CARTESIAN_POINT('Ctrl Pts',(-20.0623774469812,9.3450733381197,-4.74889227402707)) ;
#33355=CARTESIAN_POINT('Ctrl Pts',(-19.924372457776,9.63580647890616,-4.7562028171952)) ;
#33356=CARTESIAN_POINT('Ctrl Pts',(-19.5292677768152,10.4233567425039,-4.77645809541545)) ;
#33357=CARTESIAN_POINT('Ctrl Pts',(-19.2595988116131,10.913593088194,-4.78952821243563)) ;
#33358=CARTESIAN_POINT('Ctrl Pts',(-18.5679490044021,12.0653215252867,-4.82099568293175)) ;
#33359=CARTESIAN_POINT('Ctrl Pts',(-18.1288013307063,12.7156316242544,-4.83938771094345)) ;
#33360=CARTESIAN_POINT('Ctrl Pts',(-17.3213657906186,13.7842064524659,-4.87039066200427)) ;
#33361=CARTESIAN_POINT('Ctrl Pts',(-16.9701152389385,14.2144031090547,-4.88311642380444)) ;
#33362=CARTESIAN_POINT('Ctrl Pts',(-16.0580501673271,15.2494064568733,-4.91441356788873)) ;
#33363=CARTESIAN_POINT('Ctrl Pts',(-15.4789107718696,15.8369411127266,-4.93278781134249)) ;
#33364=CARTESIAN_POINT('Ctrl Pts',(-14.4797167438843,16.743325414955,-4.96278872713749)) ;
#33365=CARTESIAN_POINT('Ctrl Pts',(-14.0786761609113,17.0819207741667,-4.97443814105603)) ;
#33366=CARTESIAN_POINT('Ctrl Pts',(-13.3865805637117,17.625308040362,-4.99418376146878)) ;
#33367=CARTESIAN_POINT('Ctrl Pts',(-13.1019374029501,17.8379163231805,-5.00221205674375)) ;
#33368=CARTESIAN_POINT('Ctrl Pts',(-12.4262785704206,18.3176849515461,-5.0211959024732)) ;
#33369=CARTESIAN_POINT('Ctrl Pts',(-12.0315617059617,18.579329903176,-5.03221118505256)) ;
#33370=CARTESIAN_POINT('Ctrl Pts',(-10.975184780307,19.2317773622652,-5.06123625810335)) ;
#33371=CARTESIAN_POINT('Ctrl Pts',(-10.3010314096455,19.6011402879855,-5.07929759429781)) ;
#33372=CARTESIAN_POINT('Ctrl Pts',(-9.07144627497917,20.1938320888549,-5.11104100138105)) ;
#33373=CARTESIAN_POINT('Ctrl Pts',(-8.52358819327445,20.431114612194,-5.12479301574892)) ;
#33374=CARTESIAN_POINT('Ctrl Pts',(-7.32242041396754,20.8946179175482,-5.15412617223657)) ;
#33375=CARTESIAN_POINT('Ctrl Pts',(-6.66674359863551,21.1129684717986,-5.16963498145321)) ;
#33376=CARTESIAN_POINT('Ctrl Pts',(-5.17488102333366,21.5333405703672,-5.20420171504553)) ;
#33377=CARTESIAN_POINT('Ctrl Pts',(-4.33496867318201,21.7180151301816,-5.22316346411793)) ;
#33378=CARTESIAN_POINT('Ctrl Pts',(-3.16875812005566,21.904070574223,-5.24976824930907)) ;
#33379=CARTESIAN_POINT('Ctrl Pts',(-2.84999765764796,21.9478210514412,-5.25707720977021)) ;
#33380=CARTESIAN_POINT('Ctrl Pts',(-1.97483220502725,22.0485511818991,-5.27732906589829)) ;
#33381=CARTESIAN_POINT('Ctrl Pts',(-1.41704952437104,22.0914131940008,-5.29039726590137)) ;
#33382=CARTESIAN_POINT('Ctrl Pts',(-0.0761744825440683,22.1434547999542,
-5.32182810271876)) ;
#33383=CARTESIAN_POINT('Ctrl Pts',(0.706961598408949,22.1322978877363,-5.34018540968855)) ;
#33384=CARTESIAN_POINT('Ctrl Pts',(2.04201585686068,22.0423340601216,-5.37116083124624)) ;
#33385=CARTESIAN_POINT('Ctrl Pts',(2.5945730176349,21.9841423993488,-5.38389257137758)) ;
#33386=CARTESIAN_POINT('Ctrl Pts',(3.96929825990537,21.7868092126303,-5.41540176041185)) ;
#33387=CARTESIAN_POINT('Ctrl Pts',(4.78689211074122,21.6218884100961,-5.43397407139527)) ;
#33388=CARTESIAN_POINT('Ctrl Pts',(6.09621737926986,21.2798548727959,-5.46406798866477)) ;
#33389=CARTESIAN_POINT('Ctrl Pts',(6.59441139680776,21.130779089994,-5.47561162401545)) ;
#33390=CARTESIAN_POINT('Ctrl Pts',(7.42200204430552,20.8510156442929,-5.49521776033945)) ;
#33391=CARTESIAN_POINT('Ctrl Pts',(7.75434879016758,20.7297139969472,-5.50321373789683)) ;
#33392=CARTESIAN_POINT('Ctrl Pts',(8.52316269327929,20.4280310792644,-5.52213587572265)) ;
#33393=CARTESIAN_POINT('Ctrl Pts',(8.95704681294598,20.2415430278296,-5.53312128606359)) ;
#33394=CARTESIAN_POINT('Ctrl Pts',(10.0801606824826,19.715629156828,-5.56211215592589)) ;
#33395=CARTESIAN_POINT('Ctrl Pts',(10.7582680191723,19.3539491804508,-5.58016929236793)) ;
#33396=CARTESIAN_POINT('Ctrl Pts',(11.9274044668907,18.6499050700725,-5.61190743373268)) ;
#33397=CARTESIAN_POINT('Ctrl Pts',(12.4259531766966,18.3215073648659,-5.62565831993863)) ;
#33398=CARTESIAN_POINT('Ctrl Pts',(13.4716902267222,17.5703337037636,-5.65499305360478)) ;
#33399=CARTESIAN_POINT('Ctrl Pts',(14.0135813377178,17.1412546618382,-5.67050445835928)) ;
#33400=CARTESIAN_POINT('Ctrl Pts',(15.1824117125005,16.1232260543807,-5.70507235750584)) ;
#33401=CARTESIAN_POINT('Ctrl Pts',(15.7968900275897,15.521671756844,-5.72403278287323)) ;
#33402=CARTESIAN_POINT('Ctrl Pts',(16.5912136510912,14.6478988622716,-5.75063551409591)) ;
#33403=CARTESIAN_POINT('Ctrl Pts',(16.802376499957,14.4051884839352,-5.75794368786569)) ;
#33404=CARTESIAN_POINT('Ctrl Pts',(17.365926768366,13.7281867576746,-5.77819383399693)) ;
#33405=CARTESIAN_POINT('Ctrl Pts',(17.7072580479724,13.2850115320437,-5.79126107171641)) ;
#33406=CARTESIAN_POINT('Ctrl Pts',(18.4847424476353,12.1922735212756,-5.82267362763488)) ;
#33407=CARTESIAN_POINT('Ctrl Pts',(18.9039666108296,11.5315781560394,-5.84101361371161)) ;
#33408=CARTESIAN_POINT('Ctrl Pts',(19.5597153226286,10.3659049976172,-5.87197532144633)) ;
#33409=CARTESIAN_POINT('Ctrl Pts',(19.8137617581694,9.87164127779549,-5.88471006449852)) ;
#33410=CARTESIAN_POINT('Ctrl Pts',(20.4035568290975,8.60943617051446,-5.91631948121035)) ;
#33411=CARTESIAN_POINT('Ctrl Pts',(20.7147973820972,7.83100900801546,-5.93498520188137)) ;
#33412=CARTESIAN_POINT('Ctrl Pts',(21.1457489774053,6.54607143869715,-5.96512365156787)) ;
#33413=CARTESIAN_POINT('Ctrl Pts',(21.2930687282403,6.0497084329768,-5.97661799940822)) ;
#33414=CARTESIAN_POINT('Ctrl Pts',(21.5113686385928,5.20687011928226,-5.99615913005439)) ;
#33415=CARTESIAN_POINT('Ctrl Pts',(21.5916974680388,4.86303171155186,-6.00414003828569)) ;
#33416=CARTESIAN_POINT('Ctrl Pts',(21.7600197712438,4.05582412939803,-6.02303301427399)) ;
#33417=CARTESIAN_POINT('Ctrl Pts',(21.8414955137431,3.59127264945049,-6.03400409591986)) ;
#33418=CARTESIAN_POINT('Ctrl Pts',(22.0164919121313,2.36424057376675,-6.06297865359718)) ;
#33419=CARTESIAN_POINT('Ctrl Pts',(22.085270287227,1.59887246678189,-6.08103387237598)) ;
#33420=CARTESIAN_POINT('Ctrl Pts',(22.1365444622168,0.235181564788166,-6.11276960939535)) ;
#33421=CARTESIAN_POINT('Ctrl Pts',(22.1348375113695,-0.361783735674271,
-6.12651998052101)) ;
#33422=CARTESIAN_POINT('Ctrl Pts',(22.0790999003191,-1.64817696238934,-6.15585543692131)) ;
#33423=CARTESIAN_POINT('Ctrl Pts',(22.0168874746631,-2.33662468130006,-6.17136802927127)) ;
#33424=CARTESIAN_POINT('Ctrl Pts',(21.8052840313235,-3.87215491530582,-6.20593646212339)) ;
#33425=CARTESIAN_POINT('Ctrl Pts',(21.638530448543,-4.71571630429198,-6.22489628219893)) ;
#33426=CARTESIAN_POINT('Ctrl Pts',(21.3425265379606,-5.85882764679597,-6.25149807459006)) ;
#33427=CARTESIAN_POINT('Ctrl Pts',(21.2551151160185,-6.16841808170601,-6.2588058890153)) ;
#33428=CARTESIAN_POINT('Ctrl Pts',(20.9973520955256,-7.01068523466416,-6.27905525207966)) ;
#33429=CARTESIAN_POINT('Ctrl Pts',(20.8135128120323,-7.53897749788815,-6.29212204818657)) ;
#33430=CARTESIAN_POINT('Ctrl Pts',(20.3252082260409,-8.78764012677162,-6.32352623903764)) ;
#33431=CARTESIAN_POINT('Ctrl Pts',(20.0021882940404,-9.49995701454437,-6.34185830059628)) ;
#33432=CARTESIAN_POINT('Ctrl Pts',(19.3862409872981,-10.686822267341,-6.37281373851423)) ;
#33433=CARTESIAN_POINT('Ctrl Pts',(19.1118392659059,-11.1701439682956,-6.38554986009722)) ;
#33434=CARTESIAN_POINT('Ctrl Pts',(18.3778314702062,-12.3566189996006,-6.41720408757462)) ;
#33435=CARTESIAN_POINT('Ctrl Pts',(17.8958499836011,-13.0448950264439,-6.43591152766555)) ;
#33436=CARTESIAN_POINT('Ctrl Pts',(17.0560146186469,-14.1097512675814,-6.46607000174394)) ;
#33437=CARTESIAN_POINT('Ctrl Pts',(16.7219960302373,-14.5040532669279,-6.47754245598373)) ;
#33438=CARTESIAN_POINT('Ctrl Pts',(16.1372058629939,-15.147304920914,-6.49705470885759)) ;
#33439=CARTESIAN_POINT('Ctrl Pts',(15.8937185273065,-15.4025962308711,-6.50502892159334)) ;
#33440=CARTESIAN_POINT('Ctrl Pts',(15.3294933987821,-15.9665428946197,-6.52330751926019)) ;
#33441=CARTESIAN_POINT('Ctrl Pts',(15.0053374985415,-16.2715611622163,-6.53365313101545)) ;
#33442=CARTESIAN_POINT('Ctrl Pts',(14.0859161431552,-17.085846792298,-6.56234821794787)) ;
#33443=CARTESIAN_POINT('Ctrl Pts',(13.4724697939694,-17.5736097348172,-6.58076895856172)) ;
#33444=CARTESIAN_POINT('Ctrl Pts',(12.3450672819344,-18.3762358898492,-6.61296233748966)) ;
#33445=CARTESIAN_POINT('Ctrl Pts',(11.8416872239089,-18.7045765399974,-6.62681027876094)) ;
#33446=CARTESIAN_POINT('Ctrl Pts',(10.7403532416062,-19.3606471926614,-6.65602433380518)) ;
#33447=CARTESIAN_POINT('Ctrl Pts',(10.1393504172356,-19.6820585724023,-6.67132693531074)) ;
#33448=CARTESIAN_POINT('Ctrl Pts',(8.73780570539514,-20.3503350997291,-6.70596589931371)) ;
#33449=CARTESIAN_POINT('Ctrl Pts',(7.92966609128081,-20.6786306949514,-6.72519313103484)) ;
#33450=CARTESIAN_POINT('Ctrl Pts',(6.79854002410633,-21.0620489817465,-6.75209409975387)) ;
#33451=CARTESIAN_POINT('Ctrl Pts',(6.49057147896317,-21.1589823837779,-6.75942636518843)) ;
#33452=CARTESIAN_POINT('Ctrl Pts',(5.50761057293395,-21.4448892819535,-6.78295567123037)) ;
#33453=CARTESIAN_POINT('Ctrl Pts',(4.8257155288337,-21.6085518542192,-6.79939307837907)) ;
#33454=CARTESIAN_POINT('Ctrl Pts',(3.31406344596355,-21.8962309070508,-6.83545312907827)) ;
#33455=CARTESIAN_POINT('Ctrl Pts',(2.48267867047688,-22.0060053046048,-6.85502984038374)) ;
#33456=CARTESIAN_POINT('Ctrl Pts',(1.09890934430578,-22.1092828813567,-6.8869385881317)) ;
#33457=CARTESIAN_POINT('Ctrl Pts',(0.549410420858502,-22.1297570180054,
-6.89944285905113)) ;
#33458=CARTESIAN_POINT('Ctrl Pts',(-0.000282606165597638,-22.1297499981955,
-6.91183148751768)) ;
#33459=CARTESIAN_POINT('Origin',(0.,0.,-10.)) ;
#33460=CARTESIAN_POINT('',(0.000546534359808369,-22.1297499932512,-10.5515753459688)) ;
#33461=CARTESIAN_POINT('',(0.000544184811332343,-22.1297499933091,-10.0859246540312)) ;
#33462=CARTESIAN_POINT('',(-2.71011275034311E-15,-22.12975,-10.)) ;
#33463=CARTESIAN_POINT('Ctrl Pts',(0.000540719825256331,-22.129749993394,
-10.5513173733145)) ;
#33464=CARTESIAN_POINT('Ctrl Pts',(0.762095726907136,-22.1297313855069,
-10.5343591835597)) ;
#33465=CARTESIAN_POINT('Ctrl Pts',(1.52313896987673,-22.0904015410209,-10.5175178070212)) ;
#33466=CARTESIAN_POINT('Ctrl Pts',(2.46957986378866,-21.9923417204627,-10.4960849774183)) ;
#33467=CARTESIAN_POINT('Ctrl Pts',(2.65826587189515,-21.9703332061555,-10.4917864962238)) ;
#33468=CARTESIAN_POINT('Ctrl Pts',(3.20059935057029,-21.8999860919078,-10.4793296251818)) ;
#33469=CARTESIAN_POINT('Ctrl Pts',(3.55338801608267,-21.8455179729674,-10.4710914043089)) ;
#33470=CARTESIAN_POINT('Ctrl Pts',(5.0229221375274,-21.5820918098613,-10.4363885586976)) ;
#33471=CARTESIAN_POINT('Ctrl Pts',(6.12405154544231,-21.2958319946136,-10.4095514665115)) ;
#33472=CARTESIAN_POINT('Ctrl Pts',(7.70127965579003,-20.7532892737035,-10.370960661644)) ;
#33473=CARTESIAN_POINT('Ctrl Pts',(8.19782997801918,-20.5622059485252,-10.3587706550181)) ;
#33474=CARTESIAN_POINT('Ctrl Pts',(9.49776919282978,-20.0073806145368,-10.3266953770978)) ;
#33475=CARTESIAN_POINT('Ctrl Pts',(10.2871236764243,-19.613209729006,-10.3070717203552)) ;
#33476=CARTESIAN_POINT('Ctrl Pts',(11.4800427761846,-18.9256397460823,-10.276454588413)) ;
#33477=CARTESIAN_POINT('Ctrl Pts',(11.9007945870188,-18.6639306469199,-10.2654464559592)) ;
#33478=CARTESIAN_POINT('Ctrl Pts',(12.6000660078886,-18.1957142696058,-10.246546686971)) ;
#33479=CARTESIAN_POINT('Ctrl Pts',(12.8831653026854,-17.9963811083354,-10.2387144414267)) ;
#33480=CARTESIAN_POINT('Ctrl Pts',(13.5223146590674,-17.523535964734,-10.2204881226047)) ;
#33481=CARTESIAN_POINT('Ctrl Pts',(13.8749505604901,-17.2456675608656,-10.2100483139881)) ;
#33482=CARTESIAN_POINT('Ctrl Pts',(14.8138223177842,-16.4584114513644,-10.1814141036847)) ;
#33483=CARTESIAN_POINT('Ctrl Pts',(15.38209214591,-15.9285871194822,-10.1631556407688)) ;
#33484=CARTESIAN_POINT('Ctrl Pts',(16.3373450500845,-14.9390679654304,-10.1311652604074)) ;
#33485=CARTESIAN_POINT('Ctrl Pts',(16.7356857981465,-14.491425876617,-10.1173604691735)) ;
#33486=CARTESIAN_POINT('Ctrl Pts',(17.5498010528388,-13.4981469347963,-10.0880962604202)) ;
#33487=CARTESIAN_POINT('Ctrl Pts',(17.9593703875175,-12.9482242835916,-10.0727042055298)) ;
#33488=CARTESIAN_POINT('Ctrl Pts',(18.829054097094,-11.6596808707316,-10.0380285644672)) ;
#33489=CARTESIAN_POINT('Ctrl Pts',(19.2724686936224,-10.9111580964574,-10.0188501502847)) ;
#33490=CARTESIAN_POINT('Ctrl Pts',(19.8179927085283,-9.85273357247716,-9.99202394782781)) ;
#33491=CARTESIAN_POINT('Ctrl Pts',(19.9590351020614,-9.56379168728507,-9.98471958940597)) ;
#33492=CARTESIAN_POINT('Ctrl Pts',(20.3279332066873,-8.76432668004247,-9.96447782213127)) ;
#33493=CARTESIAN_POINT('Ctrl Pts',(20.5428169909606,-8.24808799080209,-9.95141534084429)) ;
#33494=CARTESIAN_POINT('Ctrl Pts',(21.0095885200011,-6.99491189769223,-9.92009218985851)) ;
#33495=CARTESIAN_POINT('Ctrl Pts',(21.2425882685759,-6.25172432944614,-9.90183686438735)) ;
#33496=CARTESIAN_POINT('Ctrl Pts',(21.5741080760839,-4.95912883785754,-9.87094197651316)) ;
#33497=CARTESIAN_POINT('Ctrl Pts',(21.691912650421,-4.41543093035463,-9.85819233589921)) ;
#33498=CARTESIAN_POINT('Ctrl Pts',(21.9388741959413,-3.0242074697657,-9.8261311893627)) ;
#33499=CARTESIAN_POINT('Ctrl Pts',(22.0395108236542,-2.17255722896388,-9.80704610589948)) ;
#33500=CARTESIAN_POINT('Ctrl Pts',(22.1207319068342,-0.810431891061295,
-9.77670275464389)) ;
#33501=CARTESIAN_POINT('Ctrl Pts',(22.1335020853793,-0.302757897646345,
-9.76542529530909)) ;
#33502=CARTESIAN_POINT('Ctrl Pts',(22.1255607590194,0.554876675373889,-9.7461702710391)) ;
#33503=CARTESIAN_POINT('Ctrl Pts',(22.1140182192634,0.90472380008027,-9.73825570784952)) ;
#33504=CARTESIAN_POINT('Ctrl Pts',(22.0674595242356,1.7249419367817,-9.71942779428143)) ;
#33505=CARTESIAN_POINT('Ctrl Pts',(22.0256947440072,2.19475769186084,-9.70845457187096)) ;
#33506=CARTESIAN_POINT('Ctrl Pts',(21.8767902027992,3.42323237869518,-9.67952435369552)) ;
#33507=CARTESIAN_POINT('Ctrl Pts',(21.7452140933535,4.17829399881221,-9.661517289963)) ;
#33508=CARTESIAN_POINT('Ctrl Pts',(21.4420736718042,5.50624659832969,-9.6298419328156)) ;
#33509=CARTESIAN_POINT('Ctrl Pts',(21.2859565341147,6.0818860057907,-9.61610449904824)) ;
#33510=CARTESIAN_POINT('Ctrl Pts',(20.8987434611677,7.31078572688398,-9.5867505051528)) ;
#33511=CARTESIAN_POINT('Ctrl Pts',(20.6598334973586,7.96092679006804,-9.57120771241524)) ;
#33512=CARTESIAN_POINT('Ctrl Pts',(20.0572804006495,9.38979628386058,-9.5366256087694)) ;
#33513=CARTESIAN_POINT('Ctrl Pts',(19.6779772234578,10.1607070876448,-9.5176810894635)) ;
#33514=CARTESIAN_POINT('Ctrl Pts',(19.0965251600906,11.1871242592951,-9.49110295988983)) ;
#33515=CARTESIAN_POINT('Ctrl Pts',(18.9321293204769,11.4631366369296,-9.48380416194124)) ;
#33516=CARTESIAN_POINT('Ctrl Pts',(18.4655201013132,12.2091157710813,-9.46357480523829)) ;
#33517=CARTESIAN_POINT('Ctrl Pts',(18.1514306729884,12.6713653519658,-9.45051946233114)) ;
#33518=CARTESIAN_POINT('Ctrl Pts',(17.3618161468266,13.7437555808279,-9.41932620432493)) ;
#33519=CARTESIAN_POINT('Ctrl Pts',(16.8711351564821,14.3418369398485,-9.40119365418368)) ;
#33520=CARTESIAN_POINT('Ctrl Pts',(15.9748183156088,15.3245308590199,-9.37039514729629)) ;
#33521=CARTESIAN_POINT('Ctrl Pts',(15.5840684437473,15.7217328453806,-9.35762334935739)) ;
#33522=CARTESIAN_POINT('Ctrl Pts',(14.537273531759,16.7083983983751,-9.32497819411947)) ;
#33523=CARTESIAN_POINT('Ctrl Pts',(13.8602448884879,17.2741576095613,-9.30535453637654)) ;
#33524=CARTESIAN_POINT('Ctrl Pts',(12.7528753303465,18.0924125734482,-9.27473740391591)) ;
#33525=CARTESIAN_POINT('Ctrl Pts',(12.3447027376042,18.3733375654329,-9.26372927195394)) ;
#33526=CARTESIAN_POINT('Ctrl Pts',(11.6358481714235,18.8269147369149,-9.24482950361424)) ;
#33527=CARTESIAN_POINT('Ctrl Pts',(11.3399092199787,19.0066341073481,-9.23699725822009)) ;
#33528=CARTESIAN_POINT('Ctrl Pts',(10.6508634620417,19.4032578182766,-9.21877093945944)) ;
#33529=CARTESIAN_POINT('Ctrl Pts',(10.2551297930757,19.6152903523379,-9.20833113074951)) ;
#33530=CARTESIAN_POINT('Ctrl Pts',(9.15802654994961,20.1608330399417,-9.17969692051981)) ;
#33531=CARTESIAN_POINT('Ctrl Pts',(8.44511392172443,20.4697019334919,-9.16143845777831)) ;
#33532=CARTESIAN_POINT('Ctrl Pts',(7.15608378908251,20.9493450914963,-9.12944807763529)) ;
#33533=CARTESIAN_POINT('Ctrl Pts',(6.5864691028667,21.1353501940812,-9.11564328644785)) ;
#33534=CARTESIAN_POINT('Ctrl Pts',(5.35045348936089,21.4841368253889,-9.08637907763762)) ;
#33535=CARTESIAN_POINT('Ctrl Pts',(4.68260693566097,21.6395168408771,-9.07098702264814)) ;
#33536=CARTESIAN_POINT('Ctrl Pts',(3.15375234121765,21.9211149890816,-9.03631138154412)) ;
#33537=CARTESIAN_POINT('Ctrl Pts',(2.29034965854265,22.0280666194252,-9.017132967415)) ;
#33538=CARTESIAN_POINT('Ctrl Pts',(1.10207481223357,22.104629039023,-8.99030676503934)) ;
#33539=CARTESIAN_POINT('Ctrl Pts',(0.780837682334844,22.118306584276,-8.9830024066474)) ;
#33540=CARTESIAN_POINT('Ctrl Pts',(-0.0994440898910114,22.1365851359504,
-8.96276063943875)) ;
#33541=CARTESIAN_POINT('Ctrl Pts',(-0.65853778333759,22.127010946221,-8.94969815818945)) ;
#33542=CARTESIAN_POINT('Ctrl Pts',(-1.99379820879595,22.0534888599294,-8.91837500790101)) ;
#33543=CARTESIAN_POINT('Ctrl Pts',(-2.76813729940817,21.9697298410208,-8.90011968308962)) ;
#33544=CARTESIAN_POINT('Ctrl Pts',(-4.08541978207517,21.7564804901518,-8.86922479573512)) ;
#33545=CARTESIAN_POINT('Ctrl Pts',(-4.63084448323932,21.6469486097091,-8.85647515500396)) ;
#33546=CARTESIAN_POINT('Ctrl Pts',(-6.00469305098502,21.3167467829983,-8.82441400514067)) ;
#33547=CARTESIAN_POINT('Ctrl Pts',(-6.82548797393584,21.0682879327733,-8.80532891859824)) ;
#33548=CARTESIAN_POINT('Ctrl Pts',(-8.106365642801,20.5978255147595,-8.77498556580996)) ;
#33549=CARTESIAN_POINT('Ctrl Pts',(-8.57675668872774,20.4064406876266,-8.76370810804303)) ;
#33550=CARTESIAN_POINT('Ctrl Pts',(-9.35960075557722,20.0560764035901,-8.74445308584147)) ;
#33551=CARTESIAN_POINT('Ctrl Pts',(-9.67561772485194,19.9055456740926,-8.73653852313158)) ;
#33552=CARTESIAN_POINT('Ctrl Pts',(-10.40872144524,19.5347565258284,-8.71771060739032)) ;
#33553=CARTESIAN_POINT('Ctrl Pts',(-10.8225995962712,19.308535117142,-8.70673738224158)) ;
#33554=CARTESIAN_POINT('Ctrl Pts',(-11.8889276660209,18.6806281565569,-8.67780716318418)) ;
#33555=CARTESIAN_POINT('Ctrl Pts',(-12.5283052020121,18.2579857965525,-8.65980010139932)) ;
#33556=CARTESIAN_POINT('Ctrl Pts',(-13.6241043880534,17.4489270313781,-8.62812474669491)) ;
#33557=CARTESIAN_POINT('Ctrl Pts',(-14.089224416217,17.0755684614998,-8.61438731345167)) ;
#33558=CARTESIAN_POINT('Ctrl Pts',(-15.0606096536722,16.2290820177373,-8.5850333187972)) ;
#33559=CARTESIAN_POINT('Ctrl Pts',(-15.5608901637451,15.7500404090239,-8.56949052482841)) ;
#33560=CARTESIAN_POINT('Ctrl Pts',(-16.6294033107615,14.6261996704882,-8.53490842062286)) ;
#33561=CARTESIAN_POINT('Ctrl Pts',(-17.1842065019089,13.9701754812838,-8.51596390193861)) ;
#33562=CARTESIAN_POINT('Ctrl Pts',(-17.8923137791708,13.0266699505038,-8.48938577332376)) ;
#33563=CARTESIAN_POINT('Ctrl Pts',(-18.0795142343541,12.7655860501095,-8.48208697573891)) ;
#33564=CARTESIAN_POINT('Ctrl Pts',(-18.5765418796839,12.0395196039001,-8.46185761985641)) ;
#33565=CARTESIAN_POINT('Ctrl Pts',(-18.8745454225178,11.5667398358092,-8.44880227742517)) ;
#33566=CARTESIAN_POINT('Ctrl Pts',(-19.5415139796137,10.4140630033365,-8.4176090279121)) ;
#33567=CARTESIAN_POINT('Ctrl Pts',(-19.8933637737102,9.72509976892042,-8.39947648578958)) ;
#33568=CARTESIAN_POINT('Ctrl Pts',(-20.435440959096,8.51051227232673,-8.36867798517615)) ;
#33569=CARTESIAN_POINT('Ctrl Pts',(-20.6431614581329,7.9934947300125,-8.35590618576802)) ;
#33570=CARTESIAN_POINT('Ctrl Pts',(-21.1286823965585,6.63940371242206,-8.3232609942182)) ;
#33571=CARTESIAN_POINT('Ctrl Pts',(-21.3763634248447,5.7925813686953,-8.3036373031048)) ;
#33572=CARTESIAN_POINT('Ctrl Pts',(-21.683303496542,4.45034500375449,-8.27302015334947)) ;
#33573=CARTESIAN_POINT('Ctrl Pts',(-21.7774862922587,3.96387550511088,-8.26201203779432)) ;
#33574=CARTESIAN_POINT('Ctrl Pts',(-21.90962047365,3.13276422986203,-8.24311229108966)) ;
#33575=CARTESIAN_POINT('Ctrl Pts',(-21.9559462791796,2.78964227698622,-8.23528005070215)) ;
#33576=CARTESIAN_POINT('Ctrl Pts',(-22.0438071261427,1.99946841653622,-8.21705373398806)) ;
#33577=CARTESIAN_POINT('Ctrl Pts',(-22.0798263009291,1.55195789694476,-8.20661392216783)) ;
#33578=CARTESIAN_POINT('Ctrl Pts',(-22.140932817188,0.328226692957887,-8.17797971439605)) ;
#33579=CARTESIAN_POINT('Ctrl Pts',(-22.1388188527382,-0.448715751631449,
-8.15972125747283)) ;
#33580=CARTESIAN_POINT('Ctrl Pts',(-22.0627506162553,-1.82198521596142,
-8.12773088461325)) ;
#33581=CARTESIAN_POINT('Ctrl Pts',(-22.0053567394348,-2.41844531940688,
-8.11392609497779)) ;
#33582=CARTESIAN_POINT('Ctrl Pts',(-21.8305664513511,-3.6907799035294,-8.0846618842678)) ;
#33583=CARTESIAN_POINT('Ctrl Pts',(-21.7058082385966,-4.36501841222752,
-8.06926982596833)) ;
#33584=CARTESIAN_POINT('Ctrl Pts',(-21.3522931415014,-5.87886159468619,
-8.03459418348151)) ;
#33585=CARTESIAN_POINT('Ctrl Pts',(-21.1049206091465,-6.7129536335092,-8.0154157711352)) ;
#33586=CARTESIAN_POINT('Ctrl Pts',(-20.699735332433,-7.83263371932115,-7.98858957146821)) ;
#33587=CARTESIAN_POINT('Ctrl Pts',(-20.5837638559451,-8.13251862181145,
-7.98128521407379)) ;
#33588=CARTESIAN_POINT('Ctrl Pts',(-20.2483703159901,-8.94660774221505,
-7.96104344906823)) ;
#33589=CARTESIAN_POINT('Ctrl Pts',(-20.0159370831783,-9.45518630418543,
-7.94798096907533)) ;
#33590=CARTESIAN_POINT('Ctrl Pts',(-19.4144002049621,-10.6495382721856,
-7.91665784207625)) ;
#33591=CARTESIAN_POINT('Ctrl Pts',(-19.0278709007639,-11.3257114971367,
-7.89840253930121)) ;
#33592=CARTESIAN_POINT('Ctrl Pts',(-18.3054661395498,-12.4476908580898,
-7.86750766930365)) ;
#33593=CARTESIAN_POINT('Ctrl Pts',(-17.986889867788,-12.9037551818864,-7.85475802465684)) ;
#33594=CARTESIAN_POINT('Ctrl Pts',(-17.1346663701311,-14.0307964313217,
-7.82269676367692)) ;
#33595=CARTESIAN_POINT('Ctrl Pts',(-16.5786020927111,-14.683664502367,-7.80361157428743)) ;
#33596=CARTESIAN_POINT('Ctrl Pts',(-15.6350224924737,-15.6693857281927,
-7.77326817030704)) ;
#33597=CARTESIAN_POINT('Ctrl Pts',(-15.2714460072982,-16.0239355730493,
-7.76199076490811)) ;
#33598=CARTESIAN_POINT('Ctrl Pts',(-14.6371726990142,-16.6012500093332,
-7.74273581179304)) ;
#33599=CARTESIAN_POINT('Ctrl Pts',(-14.3727933196505,-16.8306606707578,
-7.73482126510439)) ;
#33600=CARTESIAN_POINT('Ctrl Pts',(-13.739694001493,-17.3542215910968,-7.71599327676476)) ;
#33601=CARTESIAN_POINT('Ctrl Pts',(-13.3667923740043,-17.6430455324717,
-7.70501996014276)) ;
#33602=CARTESIAN_POINT('Ctrl Pts',(-12.3647437053928,-18.3691474574999,
-7.67608971162199)) ;
#33603=CARTESIAN_POINT('Ctrl Pts',(-11.7216195426005,-18.7860615277497,
-7.65808271489854)) ;
#33604=CARTESIAN_POINT('Ctrl Pts',(-10.5417601047706,-19.4667040855886,
-7.62640744180281)) ;
#33605=CARTESIAN_POINT('Ctrl Pts',(-10.0135125197445,-19.7436280630044,
-7.61267002606845)) ;
#33606=CARTESIAN_POINT('Ctrl Pts',(-8.84911697564473,-20.2952752545068,
-7.58331600606147)) ;
#33607=CARTESIAN_POINT('Ctrl Pts',(-8.20994309330438,-20.5621475679191,
-7.56777317096577)) ;
#33608=CARTESIAN_POINT('Ctrl Pts',(-6.75249793180721,-21.0918595977928,
-7.53319104806491)) ;
#33609=CARTESIAN_POINT('Ctrl Pts',(-5.92931129098236,-21.3379010690314,
-7.51424655014626)) ;
#33610=CARTESIAN_POINT('Ctrl Pts',(-4.78132155505225,-21.609442060917,-7.48766845355937)) ;
#33611=CARTESIAN_POINT('Ctrl Pts',(-4.46715182254049,-21.6765674490351,
-7.48036966812479)) ;
#33612=CARTESIAN_POINT('Ctrl Pts',(-3.60288431769079,-21.8416383157174,
-7.46014033964834)) ;
#33613=CARTESIAN_POINT('Ctrl Pts',(-3.05037031223361,-21.9256282809683,
-7.44708501311407)) ;
#33614=CARTESIAN_POINT('Ctrl Pts',(-1.72714298093534,-22.0757884641218,
-7.4158920472784)) ;
#33615=CARTESIAN_POINT('Ctrl Pts',(-0.954967361584291,-22.1226469352701,
-7.39775977298584)) ;
#33616=CARTESIAN_POINT('Ctrl Pts',(-0.121282485391881,-22.1295007483995,
-7.37845459755358)) ;
#33617=CARTESIAN_POINT('Ctrl Pts',(-0.0606403391054048,-22.1297499999887,
-7.37705174916909)) ;
#33618=CARTESIAN_POINT('Ctrl Pts',(-4.10971426655051E-9,-22.12975,-7.37565036637909)) ;
#33619=CARTESIAN_POINT('Ctrl Pts',(-0.00028260616559278,-22.1297499981955,
-6.91183148751768)) ;
#33620=CARTESIAN_POINT('Ctrl Pts',(-0.819491674422402,-22.129739536553,
-6.93029429545617)) ;
#33621=CARTESIAN_POINT('Ctrl Pts',(-1.63806773940101,-22.084240462302,-6.94846154174131)) ;
#33622=CARTESIAN_POINT('Ctrl Pts',(-3.00600318315989,-21.9317179538769,
-6.97908761796101)) ;
#33623=CARTESIAN_POINT('Ctrl Pts',(-3.55723973935411,-21.849081122676,-6.99151028370669)) ;
#33624=CARTESIAN_POINT('Ctrl Pts',(-4.41930546700327,-21.6863559688932,
-7.01141476232408)) ;
#33625=CARTESIAN_POINT('Ctrl Pts',(-4.7325162783671,-21.6201660877683,-7.01876110844946)) ;
#33626=CARTESIAN_POINT('Ctrl Pts',(-5.87816145295388,-21.3519717096865,
-7.04599713143021)) ;
#33627=CARTESIAN_POINT('Ctrl Pts',(-6.70010493251782,-21.1084834248527,
-7.06618291258562)) ;
#33628=CARTESIAN_POINT('Ctrl Pts',(-8.16066684744448,-20.5818817860658,
-7.10246060360338)) ;
#33629=CARTESIAN_POINT('Ctrl Pts',(-8.80397128374435,-20.3150299762997,
-7.11859724891427)) ;
#33630=CARTESIAN_POINT('Ctrl Pts',(-9.97165920235242,-19.7647567122671,
-7.1481251015603)) ;
#33631=CARTESIAN_POINT('Ctrl Pts',(-10.4992490188593,-19.4896221700088,
-7.16156512524228)) ;
#33632=CARTESIAN_POINT('Ctrl Pts',(-11.6748275289485,-18.8149620897786,
-7.1919367652821)) ;
#33633=CARTESIAN_POINT('Ctrl Pts',(-12.314579096878,-18.4025959392554,-7.20876954850381)) ;
#33634=CARTESIAN_POINT('Ctrl Pts',(-13.3206738957914,-17.6780964160283,
-7.23641034551954)) ;
#33635=CARTESIAN_POINT('Ctrl Pts',(-13.7003229402307,-17.3855282332158,
-7.24714071716105)) ;
#33636=CARTESIAN_POINT('Ctrl Pts',(-14.3392587644429,-16.8592121000339,
-7.26598459481017)) ;
#33637=CARTESIAN_POINT('Ctrl Pts',(-14.6030669509428,-16.6312298111907,
-7.27402408190463)) ;
#33638=CARTESIAN_POINT('Ctrl Pts',(-15.2342651569512,-16.0591489827275,
-7.29381182499496)) ;
#33639=CARTESIAN_POINT('Ctrl Pts',(-15.5955161441776,-15.7085637566714,
-7.30561174033497)) ;
#33640=CARTESIAN_POINT('Ctrl Pts',(-16.5447609591361,-14.7222960881541,
-7.33768930536408)) ;
#33641=CARTESIAN_POINT('Ctrl Pts',(-17.1079171943314,-14.0639364168517,
-7.35790154269754)) ;
#33642=CARTESIAN_POINT('Ctrl Pts',(-17.9673321132459,-12.9309860791216,
-7.39055633356931)) ;
#33643=CARTESIAN_POINT('Ctrl Pts',(-18.28676416075,-12.4751628089138,-7.40319231462525)) ;
#33644=CARTESIAN_POINT('Ctrl Pts',(-19.0100268947019,-11.3555141885319,
-7.43318895118883)) ;
#33645=CARTESIAN_POINT('Ctrl Pts',(-19.3967513873857,-10.6815197404428,
-7.45040991874401)) ;
#33646=CARTESIAN_POINT('Ctrl Pts',(-19.99950347,-9.48989114069963,-7.48012403571722)) ;
#33647=CARTESIAN_POINT('Ctrl Pts',(-20.2327751840765,-8.98181351738652,
-7.49258484537064)) ;
#33648=CARTESIAN_POINT('Ctrl Pts',(-20.5695113773647,-8.16849666216835,
-7.51256167368171)) ;
#33649=CARTESIAN_POINT('Ctrl Pts',(-20.6859749634242,-7.86889901321823,
-7.5199406015)) ;
#33650=CARTESIAN_POINT('Ctrl Pts',(-21.0930406976229,-6.75016920091236,
-7.54750433393836)) ;
#33651=CARTESIAN_POINT('Ctrl Pts',(-21.3418410333152,-5.91666906812547,
-7.56799044642639)) ;
#33652=CARTESIAN_POINT('Ctrl Pts',(-21.6980757449775,-4.40333921877305,
-7.60430519930574)) ;
#33653=CARTESIAN_POINT('Ctrl Pts',(-21.8240741519265,-3.72903289084975,
-7.62019173229536)) ;
#33654=CARTESIAN_POINT('Ctrl Pts',(-22.0010999877269,-2.45683656664787,
-7.64956534729555)) ;
#33655=CARTESIAN_POINT('Ctrl Pts',(-22.0595243635142,-1.86060169760572,
-7.66309216097388)) ;
#33656=CARTESIAN_POINT('Ctrl Pts',(-22.1379700816065,-0.488054587542169,
-7.69388835880274)) ;
#33657=CARTESIAN_POINT('Ctrl Pts',(-22.1414709101615,0.288411287534252,
-7.71105209490964)) ;
#33658=CARTESIAN_POINT('Ctrl Pts',(-22.0826013294025,1.51203279496765,-7.73837942155627)) ;
#33659=CARTESIAN_POINT('Ctrl Pts',(-22.0473696948826,1.95984942025784,-7.74844500470503)) ;
#33660=CARTESIAN_POINT('Ctrl Pts',(-21.9609429326348,2.74997446835613,-7.76653427809586)) ;
#33661=CARTESIAN_POINT('Ctrl Pts',(-21.9152994632171,3.09273639080316,-7.77450458383363)) ;
#33662=CARTESIAN_POINT('Ctrl Pts',(-21.784995354661,3.92221402986284,-7.79400337979991)) ;
#33663=CARTESIAN_POINT('Ctrl Pts',(-21.6920321323498,4.40743980225663,-7.80558128802677)) ;
#33664=CARTESIAN_POINT('Ctrl Pts',(-21.3875054419404,5.751758839279,-7.8378826566359)) ;
#33665=CARTESIAN_POINT('Ctrl Pts',(-21.140558805694,6.60188719486739,-7.85854191729972)) ;
#33666=CARTESIAN_POINT('Ctrl Pts',(-20.6562308893538,7.95966809178261,-7.89164180624271)) ;
#33667=CARTESIAN_POINT('Ctrl Pts',(-20.4493151968511,8.47712834705992,-7.90429166485741)) ;
#33668=CARTESIAN_POINT('Ctrl Pts',(-19.9094391876684,9.69209408409439,-7.93420761934462)) ;
#33669=CARTESIAN_POINT('Ctrl Pts',(-19.5590447922406,10.3810513237097,-7.95133765729493)) ;
#33670=CARTESIAN_POINT('Ctrl Pts',(-18.8944035734317,11.5342710713653,-7.98095466431243)) ;
#33671=CARTESIAN_POINT('Ctrl Pts',(-18.5972354215638,12.0075277654691,-7.99340979918347)) ;
#33672=CARTESIAN_POINT('Ctrl Pts',(-18.1015042952759,12.7343843025311,-8.01337550591042)) ;
#33673=CARTESIAN_POINT('Ctrl Pts',(-17.9147735950181,12.9957640875306,-8.02074922902676)) ;
#33674=CARTESIAN_POINT('Ctrl Pts',(-17.2083533153364,13.9404175073009,-8.04805931127953)) ;
#33675=CARTESIAN_POINT('Ctrl Pts',(-16.6547241497918,14.5973569020333,-8.06828974708615)) ;
#33676=CARTESIAN_POINT('Ctrl Pts',(-15.588134674716,15.723081010033,-8.10452055545454)) ;
#33677=CARTESIAN_POINT('Ctrl Pts',(-15.0886024132755,16.2030647774855,-8.12056901467968)) ;
#33678=CARTESIAN_POINT('Ctrl Pts',(-14.1186236484521,17.0512664924444,-8.15004102090566)) ;
#33679=CARTESIAN_POINT('Ctrl Pts',(-13.6541827924535,17.4253987664595,-8.16351020975757)) ;
#33680=CARTESIAN_POINT('Ctrl Pts',(-12.5599456325401,18.2362273687018,-8.19402414598921)) ;
#33681=CARTESIAN_POINT('Ctrl Pts',(-11.9214422105821,18.6598884682918,-8.21096779052898)) ;
#33682=CARTESIAN_POINT('Ctrl Pts',(-10.856148315205,19.2896982458853,-8.23856327101693)) ;
#33683=CARTESIAN_POINT('Ctrl Pts',(-10.4424585024676,19.5167484475727,-8.24913142098146)) ;
#33684=CARTESIAN_POINT('Ctrl Pts',(-9.7098270817612,19.8888801978601,-8.26783904235382)) ;
#33685=CARTESIAN_POINT('Ctrl Pts',(-9.39411082606535,20.0399344840325,-8.27591022471452)) ;
#33686=CARTESIAN_POINT('Ctrl Pts',(-8.61204959735149,20.3915676438154,-8.29583040065005)) ;
#33687=CARTESIAN_POINT('Ctrl Pts',(-8.14212790196691,20.5837115376729,-8.30773206508639)) ;
#33688=CARTESIAN_POINT('Ctrl Pts',(-6.86195215515994,21.0564510866412,-8.33971086358471)) ;
#33689=CARTESIAN_POINT('Ctrl Pts',(-6.04130908828061,21.3064104108324,-8.35972230418106)) ;
#33690=CARTESIAN_POINT('Ctrl Pts',(-4.66773502174942,21.6390239407721,-8.39217752456532)) ;
#33691=CARTESIAN_POINT('Ctrl Pts',(-4.12248992523782,21.749487131587,-8.40480777695205)) ;
#33692=CARTESIAN_POINT('Ctrl Pts',(-2.80561696346871,21.9649729147315,-8.43483858252193)) ;
#33693=CARTESIAN_POINT('Ctrl Pts',(-2.03147827827453,22.050048096241,-8.45209790799911)) ;
#33694=CARTESIAN_POINT('Ctrl Pts',(-0.696393312061845,22.1258519331186,
-8.48185293993438)) ;
#33695=CARTESIAN_POINT('Ctrl Pts',(-0.137320563919265,22.1363823437349,
-8.49431609272986)) ;
#33696=CARTESIAN_POINT('Ctrl Pts',(0.742980542592581,22.1196105906853,-8.51429755452301)) ;
#33697=CARTESIAN_POINT('Ctrl Pts',(1.06423893510949,22.1064828522234,-8.52167867267012)) ;
#33698=CARTESIAN_POINT('Ctrl Pts',(2.25263268205027,22.0319554861014,-8.54924843143638)) ;
#33699=CARTESIAN_POINT('Ctrl Pts',(3.11621067896902,21.9264828235127,-8.5697382211251)) ;
#33700=CARTESIAN_POINT('Ctrl Pts',(4.64553740269503,21.6475052213926,-8.60604961950149)) ;
#33701=CARTESIAN_POINT('Ctrl Pts',(5.31365952255052,21.4932671810344,-8.6219293971111)) ;
#33702=CARTESIAN_POINT('Ctrl Pts',(6.55027511474448,21.1465950943765,-8.65129903202456)) ;
#33703=CARTESIAN_POINT('Ctrl Pts',(7.12020155330308,20.9615678145442,-8.66482837190709)) ;
#33704=CARTESIAN_POINT('Ctrl Pts',(8.41003049428063,20.4841401775169,-8.6956369788407)) ;
#33705=CARTESIAN_POINT('Ctrl Pts',(9.12345027044491,20.1765028036385,-8.7128103966964)) ;
#33706=CARTESIAN_POINT('Ctrl Pts',(10.2214844461911,19.6328442146709,-8.74014301963547)) ;
#33707=CARTESIAN_POINT('Ctrl Pts',(10.6175902287654,19.4214852558423,-8.75020371231221)) ;
#33708=CARTESIAN_POINT('Ctrl Pts',(11.3073047997766,19.0260486529937,-8.76829806559389)) ;
#33709=CARTESIAN_POINT('Ctrl Pts',(11.6035334716215,18.846847880448,-8.77627861929453)) ;
#33710=CARTESIAN_POINT('Ctrl Pts',(12.3130898457904,18.3945364964279,-8.79582021880085)) ;
#33711=CARTESIAN_POINT('Ctrl Pts',(12.7216895063439,18.1143525614546,-8.80743101771404)) ;
#33712=CARTESIAN_POINT('Ctrl Pts',(13.8305142969275,17.2979769088126,-8.83969854471356)) ;
#33713=CARTESIAN_POINT('Ctrl Pts',(14.5086199203236,16.7332931912151,-8.86029083925275)) ;
#33714=CARTESIAN_POINT('Ctrl Pts',(15.5572016390319,15.7483188943685,-8.89332398568439)) ;
#33715=CARTESIAN_POINT('Ctrl Pts',(15.9486320401761,15.3517820863979,-8.90597167225456)) ;
#33716=CARTESIAN_POINT('Ctrl Pts',(16.8466097990481,14.3706359252785,-8.93590006812211)) ;
#33717=CARTESIAN_POINT('Ctrl Pts',(17.3382935025537,13.7734171618568,-8.95304416028605)) ;
#33718=CARTESIAN_POINT('Ctrl Pts',(18.1297296635925,12.702395101905,-8.98267618853019)) ;
#33719=CARTESIAN_POINT('Ctrl Pts',(18.4446078398806,12.2406851707781,-8.99513221240245)) ;
#33720=CARTESIAN_POINT('Ctrl Pts',(18.9124885823397,11.4955120718219,-9.01509965227807)) ;
#33721=CARTESIAN_POINT('Ctrl Pts',(19.0773561754003,11.2197816105119,-9.02247418162574)) ;
#33722=CARTESIAN_POINT('Ctrl Pts',(19.6605606607886,10.1943666345315,-9.04978642258402)) ;
#33723=CARTESIAN_POINT('Ctrl Pts',(20.0411805103896,9.42410957393968,-9.07001815227267)) ;
#33724=CARTESIAN_POINT('Ctrl Pts',(20.6461747934665,7.99628283619559,-9.10624763174809)) ;
#33725=CARTESIAN_POINT('Ctrl Pts',(20.8861999727258,7.34654581265738,-9.12229356527503)) ;
#33726=CARTESIAN_POINT('Ctrl Pts',(21.2755160488762,6.11830756564737,-9.15176399458842)) ;
#33727=CARTESIAN_POINT('Ctrl Pts',(21.4326174251605,5.54294038379523,-9.16523404087562)) ;
#33728=CARTESIAN_POINT('Ctrl Pts',(21.7380275216957,4.21552056883294,-9.19575216608417)) ;
#33729=CARTESIAN_POINT('Ctrl Pts',(21.8708940617532,3.46070025076321,-9.21269907513111)) ;
#33730=CARTESIAN_POINT('Ctrl Pts',(22.0219047515762,2.23247017538734,-9.24029328718479)) ;
#33731=CARTESIAN_POINT('Ctrl Pts',(22.0644751850135,1.76270861735612,-9.25085672297905)) ;
#33732=CARTESIAN_POINT('Ctrl Pts',(22.1124378593305,0.942559353198248,-9.26956044830227)) ;
#33733=CARTESIAN_POINT('Ctrl Pts',(22.124578721879,0.592737252509702,-9.27763261525578)) ;
#33734=CARTESIAN_POINT('Ctrl Pts',(22.1339877264747,-0.264861580769144,
-9.29755690629313)) ;
#33735=CARTESIAN_POINT('Ctrl Pts',(22.1220871878167,-0.772541899546286,
-9.309461732517)) ;
#33736=CARTESIAN_POINT('Ctrl Pts',(22.0432003575448,-2.13480431721731,-9.34143750197635)) ;
#33737=CARTESIAN_POINT('Ctrl Pts',(21.944019437397,-2.98665410439585,-9.36144274564382)) ;
#33738=CARTESIAN_POINT('Ctrl Pts',(21.6994321916444,-4.37832621090559,-9.39389181081161)) ;
#33739=CARTESIAN_POINT('Ctrl Pts',(21.5825580273603,-4.9222244130592,-9.40652189167091)) ;
#33740=CARTESIAN_POINT('Ctrl Pts',(21.2532493491615,-6.21538375154405,-9.43655372852578)) ;
#33741=CARTESIAN_POINT('Ctrl Pts',(21.0215226547319,-6.95896484435627,-9.45381421032134)) ;
#33742=CARTESIAN_POINT('Ctrl Pts',(20.5568925925635,-8.2129445255478,-9.4835704752353)) ;
#33743=CARTESIAN_POINT('Ctrl Pts',(20.3428919822577,-8.72954921137408,-9.4960336982369)) ;
#33744=CARTESIAN_POINT('Ctrl Pts',(19.9753639382984,-9.5296395531761,-9.51601529924318)) ;
#33745=CARTESIAN_POINT('Ctrl Pts',(19.8348154343114,-9.81882309668112,-9.52339648340031)) ;
#33746=CARTESIAN_POINT('Ctrl Pts',(19.291104226313,-10.8781764230762,-9.5509664236352)) ;
#33747=CARTESIAN_POINT('Ctrl Pts',(18.8489713727653,-11.6274547608296,-9.57145632400323)) ;
#33748=CARTESIAN_POINT('Ctrl Pts',(17.9815001347149,-12.9174742628897,-9.6077676215876)) ;
#33749=CARTESIAN_POINT('Ctrl Pts',(17.5728714777409,-13.4680989014952,-9.62364719604295)) ;
#33750=CARTESIAN_POINT('Ctrl Pts',(16.7604564827969,-14.4627691304093,-9.65301671142507)) ;
#33751=CARTESIAN_POINT('Ctrl Pts',(16.3628843516324,-14.9110903479753,-9.66654612743632)) ;
#33752=CARTESIAN_POINT('Ctrl Pts',(15.4093292983237,-15.9022389385818,-9.69735510837264)) ;
#33753=CARTESIAN_POINT('Ctrl Pts',(14.8419742276548,-16.4330286984593,-9.71452881803797)) ;
#33754=CARTESIAN_POINT('Ctrl Pts',(13.9044494279254,-17.2218929280114,-9.74186159953693)) ;
#33755=CARTESIAN_POINT('Ctrl Pts',(13.5522867834835,-17.5003665225471,-9.75192214371125)) ;
#33756=CARTESIAN_POINT('Ctrl Pts',(12.9139521521488,-17.974301597064,-9.77001664921732)) ;
#33757=CARTESIAN_POINT('Ctrl Pts',(12.6312011347797,-18.1741143073738,-9.77799751205913)) ;
#33758=CARTESIAN_POINT('Ctrl Pts',(11.9327619114834,-18.6435079581784,-9.79754040273362)) ;
#33759=CARTESIAN_POINT('Ctrl Pts',(11.5124812431647,-18.9059241931282,-9.8091521937653)) ;
#33760=CARTESIAN_POINT('Ctrl Pts',(10.3207332205491,-19.59554660422,-9.84141870352719)) ;
#33761=CARTESIAN_POINT('Ctrl Pts',(9.53200825225841,-19.9910935608971,-9.86200898195824)) ;
#33762=CARTESIAN_POINT('Ctrl Pts',(8.23297262702736,-20.5481600776479,-9.89446345009149)) ;
#33763=CARTESIAN_POINT('Ctrl Pts',(7.73675276523366,-20.740091202289,-9.906547564853)) ;
#33764=CARTESIAN_POINT('Ctrl Pts',(6.15822503191993,-21.2861009289065,-9.94416301132018)) ;
#33765=CARTESIAN_POINT('Ctrl Pts',(5.05524770027415,-21.5746674791876,-9.9691798774967)) ;
#33766=CARTESIAN_POINT('Ctrl Pts',(3.58489124272495,-21.840351533277,-10.0027077280322)) ;
#33767=CARTESIAN_POINT('Ctrl Pts',(3.23332624718334,-21.8951593151537,-10.010747562498)) ;
#33768=CARTESIAN_POINT('Ctrl Pts',(2.69870303513949,-21.9653475116313,-10.0230997815463)) ;
#33769=CARTESIAN_POINT('Ctrl Pts',(2.51652329890662,-21.9869643082306,-10.0273283249198)) ;
#33770=CARTESIAN_POINT('Ctrl Pts',(1.55896316255078,-22.0885277856535,-10.0496218691874)) ;
#33771=CARTESIAN_POINT('Ctrl Pts',(0.780029229939695,-22.1297305952072,
-10.0679688232123)) ;
#33772=CARTESIAN_POINT('Ctrl Pts',(0.000550716358238557,-22.1297499931475,
-10.0862038529432)) ;
#33773=CARTESIAN_POINT('Origin',(0.,0.,-10.)) ;
#33774=CARTESIAN_POINT('',(-0.000186678706946326,-22.1297499992126,-13.7265753322825)) ;
#33775=CARTESIAN_POINT('',(-0.000174491033434178,-22.1297499993121,-13.2609246410094)) ;
#33776=CARTESIAN_POINT('',(-2.71011275034311E-15,-22.12975,-10.)) ;
#33777=CARTESIAN_POINT('Ctrl Pts',(-0.000186678706946326,-22.1297499992126,
-13.7265753322825)) ;
#33778=CARTESIAN_POINT('Ctrl Pts',(0.443811682544672,-22.129753744625,-13.7164336904268)) ;
#33779=CARTESIAN_POINT('Ctrl Pts',(0.887869351187652,-22.1163909616294,
-13.706292048571)) ;
#33780=CARTESIAN_POINT('Ctrl Pts',(1.33116660457718,-22.08967701288,-13.6961504067153)) ;
#33781=CARTESIAN_POINT('Ctrl Pts',(1.77439794946708,-22.0629670359041,-13.6860102726974)) ;
#33782=CARTESIAN_POINT('Ctrl Pts',(2.21686887397983,-22.0229098716419,-13.6758701386796)) ;
#33783=CARTESIAN_POINT('Ctrl Pts',(2.65776220351048,-21.9695729392287,-13.6657300046617)) ;
#33784=CARTESIAN_POINT('Ctrl Pts',(3.09861081635288,-21.9162414164029,-13.6555908990858)) ;
#33785=CARTESIAN_POINT('Ctrl Pts',(3.53788192410997,-21.8496328434984,-13.64545179351)) ;
#33786=CARTESIAN_POINT('Ctrl Pts',(3.97476424351366,-21.7698664274953,-13.6353126879341)) ;
#33787=CARTESIAN_POINT('Ctrl Pts',(4.41162289108153,-21.6901043335198,-13.625174131731)) ;
#33788=CARTESIAN_POINT('Ctrl Pts',(4.84609278126068,-21.5971858623802,-13.6150355755279)) ;
#33789=CARTESIAN_POINT('Ctrl Pts',(5.27737184086928,-21.4912815233457,-13.6048970193247)) ;
#33790=CARTESIAN_POINT('Ctrl Pts',(5.70869218708943,-21.3853670460232,-13.5947574925514)) ;
#33791=CARTESIAN_POINT('Ctrl Pts',(6.13682086686759,-21.266464269091,-13.584617965778)) ;
#33792=CARTESIAN_POINT('Ctrl Pts',(6.56096805462135,-21.1347943744134,-13.5744784390046)) ;
#33793=CARTESIAN_POINT('Ctrl Pts',(6.98512129467272,-21.0031226008943,-13.5643387675469)) ;
#33794=CARTESIAN_POINT('Ctrl Pts',(7.40529270873749,-20.8586834162419,-13.5541990960893)) ;
#33795=CARTESIAN_POINT('Ctrl Pts',(7.82070825561196,-20.7017476905478,-13.5440594246316)) ;
#33796=CARTESIAN_POINT('Ctrl Pts',(8.23620925994095,-20.5447796807283,-13.5339176672854)) ;
#33797=CARTESIAN_POINT('Ctrl Pts',(8.64695222465578,-20.3753100725641,-13.5237759099392)) ;
#33798=CARTESIAN_POINT('Ctrl Pts',(9.05218172659114,-20.1936584365308,-13.5136341525931)) ;
#33799=CARTESIAN_POINT('Ctrl Pts',(9.3824336728765,-20.045616879686,-13.5053688730753)) ;
#33800=CARTESIAN_POINT('Ctrl Pts',(9.70902397047871,-19.8894851375713,-13.4971035935576)) ;
#33801=CARTESIAN_POINT('Ctrl Pts',(10.0315545694457,-19.7254593858478,-13.4888383140399)) ;
#33802=CARTESIAN_POINT('Ctrl Pts',(10.4387353476837,-19.5183840464794,-13.478403760056)) ;
#33803=CARTESIAN_POINT('Ctrl Pts',(10.839554832239,-19.2986698255881,-13.467969206072)) ;
#33804=CARTESIAN_POINT('Ctrl Pts',(11.2332271499225,-19.0667365550779,-13.4575346520881)) ;
#33805=CARTESIAN_POINT('Ctrl Pts',(11.6165832589122,-18.840881111009,-13.4473735362702)) ;
#33806=CARTESIAN_POINT('Ctrl Pts',(11.9931617844149,-18.6034389500622,-13.4372124204522)) ;
#33807=CARTESIAN_POINT('Ctrl Pts',(12.3622630052698,-18.3548437326782,-13.4270513046342)) ;
#33808=CARTESIAN_POINT('Ctrl Pts',(12.7313262730158,-18.1062740772833,-13.4168912336406)) ;
#33809=CARTESIAN_POINT('Ctrl Pts',(13.0929135815744,-17.8465537843947,-13.4067311626469)) ;
#33810=CARTESIAN_POINT('Ctrl Pts',(13.4463540225345,-17.5761599492941,-13.3965710916533)) ;
#33811=CARTESIAN_POINT('Ctrl Pts',(13.7997733772339,-17.3057822458928,-13.3864116268096)) ;
#33812=CARTESIAN_POINT('Ctrl Pts',(14.1450466531115,-17.0247324119128,-13.3762521619659)) ;
#33813=CARTESIAN_POINT('Ctrl Pts',(14.4815344736949,-16.7335290464888,-13.3660926971222)) ;
#33814=CARTESIAN_POINT('Ctrl Pts',(14.8339480721597,-16.4285431907863,-13.3554523905642)) ;
#33815=CARTESIAN_POINT('Ctrl Pts',(15.17672440761,-16.1124197650166,-13.3448120840061)) ;
#33816=CARTESIAN_POINT('Ctrl Pts',(15.5091690889543,-15.785800873973,-13.3341717774481)) ;
#33817=CARTESIAN_POINT('Ctrl Pts',(15.8266211638622,-15.4739118575909,-13.3240113279537)) ;
#33818=CARTESIAN_POINT('Ctrl Pts',(16.1346525681014,-15.1524531520895,-13.3138508784592)) ;
#33819=CARTESIAN_POINT('Ctrl Pts',(16.432696261367,-14.8220217461774,-13.3036904289648)) ;
#33820=CARTESIAN_POINT('Ctrl Pts',(16.7307532993377,-14.4915755454221,-13.2935295245431)) ;
#33821=CARTESIAN_POINT('Ctrl Pts',(17.0188215808823,-14.1521560135859,-13.2833686201214)) ;
#33822=CARTESIAN_POINT('Ctrl Pts',(17.2963730898947,-13.8043946987062,-13.2732077156997)) ;
#33823=CARTESIAN_POINT('Ctrl Pts',(17.5739707213121,-13.4565755942353,-13.2630451227793)) ;
#33824=CARTESIAN_POINT('Ctrl Pts',(17.8410479450515,-13.100412116321,-13.2528825298589)) ;
#33825=CARTESIAN_POINT('Ctrl Pts',(18.0971177761887,-12.7365679544081,-13.2427199369386)) ;
#33826=CARTESIAN_POINT('Ctrl Pts',(18.1333256017635,-12.6851210272459,-13.2412829641011)) ;
#33827=CARTESIAN_POINT('Ctrl Pts',(18.1693134208187,-12.6335205858924,-13.2398459912636)) ;
#33828=CARTESIAN_POINT('Ctrl Pts',(18.2050799256723,-12.5817685546342,-13.2384090184261)) ;
#33829=CARTESIAN_POINT('Ctrl Pts',(18.4647977964425,-12.2059720539304,-13.2279744644421)) ;
#33830=CARTESIAN_POINT('Ctrl Pts',(18.7129092937484,-11.822082378419,-13.2175399104582)) ;
#33831=CARTESIAN_POINT('Ctrl Pts',(18.9489227444543,-11.4308425711844,-13.2071053564743)) ;
#33832=CARTESIAN_POINT('Ctrl Pts',(19.1787514472871,-11.0498552286227,-13.1969442406583)) ;
#33833=CARTESIAN_POINT('Ctrl Pts',(19.39710792746,-10.6618982552937,-13.1867831248423)) ;
#33834=CARTESIAN_POINT('Ctrl Pts',(19.6035828749807,-10.2676858895402,-13.1766220090263)) ;
#33835=CARTESIAN_POINT('Ctrl Pts',(19.8100365915602,-9.87351405896871,-13.1664619380346)) ;
#33836=CARTESIAN_POINT('Ctrl Pts',(20.0046111094016,-9.47308832405769,-13.1563018670429)) ;
#33837=CARTESIAN_POINT('Ctrl Pts',(20.1869431201869,-9.06714743041258,-13.1461417960513)) ;
#33838=CARTESIAN_POINT('Ctrl Pts',(20.3692642530432,-8.66123075520413,-13.1359823312095)) ;
#33839=CARTESIAN_POINT('Ctrl Pts',(20.5393442440229,-8.24979978795752,-13.1258228663677)) ;
#33840=CARTESIAN_POINT('Ctrl Pts',(20.6968672602428,-7.83361478976272,-13.115663401526)) ;
#33841=CARTESIAN_POINT('Ctrl Pts',(20.8618457516162,-7.39773199128597,-13.1050230949665)) ;
#33842=CARTESIAN_POINT('Ctrl Pts',(21.0130499833048,-6.95663459065067,-13.094382788407)) ;
#33843=CARTESIAN_POINT('Ctrl Pts',(21.150174459723,-6.51121765768752,-13.0837424818475)) ;
#33844=CARTESIAN_POINT('Ctrl Pts',(21.2811148897792,-6.08588815940987,-13.073582032355)) ;
#33845=CARTESIAN_POINT('Ctrl Pts',(21.3992171990292,-5.65662030618157,-13.0634215828626)) ;
#33846=CARTESIAN_POINT('Ctrl Pts',(21.5042664660398,-5.22420891810953,-13.0532611333701)) ;
#33847=CARTESIAN_POINT('Ctrl Pts',(21.6093204365609,-4.79177816910761,-13.0431002289503)) ;
#33848=CARTESIAN_POINT('Ctrl Pts',(21.7013201452544,-4.3562038276328,-13.0329393245305)) ;
#33849=CARTESIAN_POINT('Ctrl Pts',(21.7801014345156,-3.91829255731518,-13.0227784201107)) ;
#33850=CARTESIAN_POINT('Ctrl Pts',(21.8588958153373,-3.48030851664874,-13.0126158271923)) ;
#33851=CARTESIAN_POINT('Ctrl Pts',(21.9244673470658,-3.03998699708508,-13.002453234274)) ;
#33852=CARTESIAN_POINT('Ctrl Pts',(21.9767032516041,-2.59814342433856,-12.9922906413556)) ;
#33853=CARTESIAN_POINT('Ctrl Pts',(21.9840893170606,-2.53566751665238,-12.9908536685078)) ;
#33854=CARTESIAN_POINT('Ctrl Pts',(21.9912088416097,-2.47316118821051,-12.98941669566)) ;
#33855=CARTESIAN_POINT('Ctrl Pts',(21.9980615899916,-2.41062675365442,-12.9879797228121)) ;
#33856=CARTESIAN_POINT('Ctrl Pts',(22.047822706242,-1.95653401681598,-12.9775451688282)) ;
#33857=CARTESIAN_POINT('Ctrl Pts',(22.0835251186466,-1.50084120821694,-12.9671106148443)) ;
#33858=CARTESIAN_POINT('Ctrl Pts',(22.1050896615229,-1.04443578957034,-12.9566760608604)) ;
#33859=CARTESIAN_POINT('Ctrl Pts',(22.1260891041486,-0.599990504643697,
-12.9465149450432)) ;
#33860=CARTESIAN_POINT('Ctrl Pts',(22.1336821546946,-0.154869721914559,
-12.936353829226)) ;
#33861=CARTESIAN_POINT('Ctrl Pts',(22.1278484033474,0.290103603867267,-12.9261927134089)) ;
#33862=CARTESIAN_POINT('Ctrl Pts',(22.12201525186,0.735031174931935,-12.9160326424161)) ;
#33863=CARTESIAN_POINT('Ctrl Pts',(22.1027580592561,1.17981108988913,-12.9058725714232)) ;
#33864=CARTESIAN_POINT('Ctrl Pts',(22.0701085373036,1.62362071129283,-12.8957125004304)) ;
#33865=CARTESIAN_POINT('Ctrl Pts',(22.0374609632219,2.06740385501081,-12.8855530355876)) ;
#33866=CARTESIAN_POINT('Ctrl Pts',(21.9914226728818,2.51021659196284,-12.8753935707447)) ;
#33867=CARTESIAN_POINT('Ctrl Pts',(21.9320773733454,2.95123993468679,-12.8652341059018)) ;
#33868=CARTESIAN_POINT('Ctrl Pts',(21.8699232944008,3.41313666238461,-12.8545937993432)) ;
#33869=CARTESIAN_POINT('Ctrl Pts',(21.7931723497383,3.8730702760558,-12.8439534927845)) ;
#33870=CARTESIAN_POINT('Ctrl Pts',(21.7019814482537,4.33010811437246,-12.8333131862259)) ;
#33871=CARTESIAN_POINT('Ctrl Pts',(21.6149030784992,4.76653443792858,-12.8231527367323)) ;
#33872=CARTESIAN_POINT('Ctrl Pts',(21.5146582727688,5.20032012721874,-12.8129922872387)) ;
#33873=CARTESIAN_POINT('Ctrl Pts',(21.4014359433373,5.63066378198242,-12.8028318377451)) ;
#33874=CARTESIAN_POINT('Ctrl Pts',(21.2882085444514,6.06102670509671,-12.7926709333241)) ;
#33875=CARTESIAN_POINT('Ctrl Pts',(21.1620025216004,6.48794706440571,-12.7825100289031)) ;
#33876=CARTESIAN_POINT('Ctrl Pts',(21.0230570756204,6.91063718174438,-12.7723491244821)) ;
#33877=CARTESIAN_POINT('Ctrl Pts',(20.8840885402411,7.33339754003844,-12.7621865315627)) ;
#33878=CARTESIAN_POINT('Ctrl Pts',(20.732376423431,7.75192603371615,-12.7520239386432)) ;
#33879=CARTESIAN_POINT('Ctrl Pts',(20.5682092908173,8.16545171020179,-12.7418613457237)) ;
#33880=CARTESIAN_POINT('Ctrl Pts',(20.5449963457602,8.22392351667803,-12.7404243728819)) ;
#33881=CARTESIAN_POINT('Ctrl Pts',(20.5215344610334,8.28229533056822,-12.7389874000401)) ;
#33882=CARTESIAN_POINT('Ctrl Pts',(20.4978245304077,8.3405650038301,-12.7375504271984)) ;
#33883=CARTESIAN_POINT('Ctrl Pts',(20.3256552702268,8.76368925058057,-12.7271158732144)) ;
#33884=CARTESIAN_POINT('Ctrl Pts',(20.1403578099894,9.18153545349456,-12.7166813192305)) ;
#33885=CARTESIAN_POINT('Ctrl Pts',(19.9422845404748,9.59328527508905,-12.7062467652466)) ;
#33886=CARTESIAN_POINT('Ctrl Pts',(19.7494017938981,9.9942451657711,-12.69608564943)) ;
#33887=CARTESIAN_POINT('Ctrl Pts',(19.5444043594006,10.3894238816228,-12.6859245336133)) ;
#33888=CARTESIAN_POINT('Ctrl Pts',(19.3276656383988,10.7780877725485,-12.6757634177967)) ;
#33889=CARTESIAN_POINT('Ctrl Pts',(19.1109492037187,11.1667116988178,-12.6656033468044)) ;
#33890=CARTESIAN_POINT('Ctrl Pts',(18.8824940058694,11.548821937848,-12.6554432758121)) ;
#33891=CARTESIAN_POINT('Ctrl Pts',(18.6427191461546,11.9237099050632,-12.6452832048198)) ;
#33892=CARTESIAN_POINT('Ctrl Pts',(18.402958591408,12.2985755064621,-12.6351237399774)) ;
#33893=CARTESIAN_POINT('Ctrl Pts',(18.1518798476512,12.6662195035583,-12.6249642751349)) ;
#33894=CARTESIAN_POINT('Ctrl Pts',(17.8899460201268,13.0259612489617,-12.6148048102925)) ;
#33895=CARTESIAN_POINT('Ctrl Pts',(17.6156150129077,13.4027293674133,-12.6041645037335)) ;
#33896=CARTESIAN_POINT('Ctrl Pts',(17.3293768617193,13.7708290241797,-12.5935241971745)) ;
#33897=CARTESIAN_POINT('Ctrl Pts',(17.0318131241977,14.129514385318,-12.5828838906155)) ;
#33898=CARTESIAN_POINT('Ctrl Pts',(16.7476689306716,14.4720237364879,-12.5727234411223)) ;
#33899=CARTESIAN_POINT('Ctrl Pts',(16.4531981208485,14.8059488590116,-12.5625629916292)) ;
#33900=CARTESIAN_POINT('Ctrl Pts',(16.1489479842514,15.1306746070505,-12.5524025421361)) ;
#33901=CARTESIAN_POINT('Ctrl Pts',(15.8446842250619,15.4554148944634,-12.5422416377157)) ;
#33902=CARTESIAN_POINT('Ctrl Pts',(15.5306404229071,15.7709548185611,-12.5320807332954)) ;
#33903=CARTESIAN_POINT('Ctrl Pts',(15.2074015800676,16.0767152193804,-12.5219198288751)) ;
#33904=CARTESIAN_POINT('Ctrl Pts',(14.8841090226808,16.382526430249,-12.511757235956)) ;
#33905=CARTESIAN_POINT('Ctrl Pts',(14.5516185382453,16.6785547129367,-12.5015946430369)) ;
#33906=CARTESIAN_POINT('Ctrl Pts',(14.2105506008589,16.9642590961977,-12.4914320501178)) ;
#33907=CARTESIAN_POINT('Ctrl Pts',(14.1623241917089,17.0046571957339,-12.4899950772734)) ;
#33908=CARTESIAN_POINT('Ctrl Pts',(14.1139263444979,17.0448489497629,-12.4885581044289)) ;
#33909=CARTESIAN_POINT('Ctrl Pts',(14.0653588669669,17.0848328937082,-12.4871211315845)) ;
#33910=CARTESIAN_POINT('Ctrl Pts',(13.7126869510626,17.3751756257886,-12.4766865776005)) ;
#33911=CARTESIAN_POINT('Ctrl Pts',(13.3509762733302,17.6546322121746,-12.4662520236166)) ;
#33912=CARTESIAN_POINT('Ctrl Pts',(12.9809259880184,17.9226503496578,-12.4558174696327)) ;
#33913=CARTESIAN_POINT('Ctrl Pts',(12.6205728945467,18.1836450543834,-12.4456563538159)) ;
#33914=CARTESIAN_POINT('Ctrl Pts',(12.2523118783805,18.4337929897971,-12.4354952379991)) ;
#33915=CARTESIAN_POINT('Ctrl Pts',(11.8768203035513,18.6726263428488,-12.4253341221823)) ;
#33916=CARTESIAN_POINT('Ctrl Pts',(11.5013673389252,18.9114351376817,-12.4151740511898)) ;
#33917=CARTESIAN_POINT('Ctrl Pts',(11.1186854943598,19.1389315509339,-12.4050139801974)) ;
#33918=CARTESIAN_POINT('Ctrl Pts',(10.7294804156782,19.3546915519746,-12.3948539092049)) ;
#33919=CARTESIAN_POINT('Ctrl Pts',(10.3402985569723,19.5704386807733,-12.3846944443623)) ;
#33920=CARTESIAN_POINT('Ctrl Pts',(9.94459444236979,19.7744506849794,-12.3745349795197)) ;
#33921=CARTESIAN_POINT('Ctrl Pts',(9.54309914195966,19.9663490360463,-12.3643755146771)) ;
#33922=CARTESIAN_POINT('Ctrl Pts',(9.12260129640409,20.1673298273704,-12.3537352081183)) ;
#33923=CARTESIAN_POINT('Ctrl Pts',(8.69575115004648,20.3550226323908,-12.3430949015594)) ;
#33924=CARTESIAN_POINT('Ctrl Pts',(8.26341497367153,20.529047908644,-12.3324545950005)) ;
#33925=CARTESIAN_POINT('Ctrl Pts',(7.85057631532528,20.6952249844768,-12.3222941455073)) ;
#33926=CARTESIAN_POINT('Ctrl Pts',(7.43273567196483,20.8489397919958,-12.312133696014)) ;
#33927=CARTESIAN_POINT('Ctrl Pts',(7.01066702043379,20.9899114574384,-12.3019732465208)) ;
#33928=CARTESIAN_POINT('Ctrl Pts',(6.58857947106427,21.1308894347919,-12.2918123421003)) ;
#33929=CARTESIAN_POINT('Ctrl Pts',(6.16226375373612,21.2591230596214,-12.2816514376798)) ;
#33930=CARTESIAN_POINT('Ctrl Pts',(5.73250990772562,21.374381048824,-12.2714905332593)) ;
#33931=CARTESIAN_POINT('Ctrl Pts',(5.30268464692803,21.4896581911415,-12.2613279403401)) ;
#33932=CARTESIAN_POINT('Ctrl Pts',(4.86942033754504,21.5919553299681,-12.2511653474208)) ;
#33933=CARTESIAN_POINT('Ctrl Pts',(4.43352006239451,21.681091644999,-12.2410027545016)) ;
#33934=CARTESIAN_POINT('Ctrl Pts',(4.37188452676789,21.6936953638629,-12.239565781658)) ;
#33935=CARTESIAN_POINT('Ctrl Pts',(4.3101963064683,21.7060360355789,-12.2381288088143)) ;
#33936=CARTESIAN_POINT('Ctrl Pts',(4.2484576882242,21.7181132314451,-12.2366918359707)) ;
#33937=CARTESIAN_POINT('Ctrl Pts',(3.80014375674978,21.8058115848247,-12.2262572819867)) ;
#33938=CARTESIAN_POINT('Ctrl Pts',(3.349055427096,21.8796351373696,-12.2158227280028)) ;
#33939=CARTESIAN_POINT('Ctrl Pts',(2.89607038505077,21.9394305164772,-12.2053881740189)) ;
#33940=CARTESIAN_POINT('Ctrl Pts',(2.45495584555064,21.9976589537788,-12.1952270582021)) ;
#33941=CARTESIAN_POINT('Ctrl Pts',(2.01204296917008,22.0425849991785,-12.1850659423853)) ;
#33942=CARTESIAN_POINT('Ctrl Pts',(1.568150093832,22.0741192428082,-12.1749048265685)) ;
#33943=CARTESIAN_POINT('Ctrl Pts',(1.12430286211199,22.1056502439056,-12.1647447555761)) ;
#33944=CARTESIAN_POINT('Ctrl Pts',(0.679476061608808,22.1237921775522,-12.1545846845836)) ;
#33945=CARTESIAN_POINT('Ctrl Pts',(0.234492088719243,22.1285075981827,-12.1444246135912)) ;
#33946=CARTESIAN_POINT('Ctrl Pts',(-0.210465336426893,22.1332227374911,
-12.1342651487485)) ;
#33947=CARTESIAN_POINT('Ctrl Pts',(-0.65557968575692,22.1245129616793,-12.1241056839059)) ;
#33948=CARTESIAN_POINT('Ctrl Pts',(-1.10002783592053,22.1023929433602,-12.1139462190633)) ;
#33949=CARTESIAN_POINT('Ctrl Pts',(-1.56551146527747,22.0792259971038,-12.1033059125044)) ;
#33950=CARTESIAN_POINT('Ctrl Pts',(-2.03026404861439,22.0413489224589,-12.0926656059455)) ;
#33951=CARTESIAN_POINT('Ctrl Pts',(-2.49334304585184,21.9888397947277,-12.0820252993867)) ;
#33952=CARTESIAN_POINT('Ctrl Pts',(-2.93553808382328,21.9386987262071,-12.0718648498934)) ;
#33953=CARTESIAN_POINT('Ctrl Pts',(-3.37620688762659,21.8752160462819,-12.0617044004001)) ;
#33954=CARTESIAN_POINT('Ctrl Pts',(-3.81453502899431,21.7985127376864,-12.0515439509068)) ;
#33955=CARTESIAN_POINT('Ctrl Pts',(-4.25288279619944,21.7218059947537,-12.0413830464865)) ;
#33956=CARTESIAN_POINT('Ctrl Pts',(-4.68888946590498,21.6318774823466,-12.0312221420661)) ;
#33957=CARTESIAN_POINT('Ctrl Pts',(-5.12175006271124,21.5288994460381,-12.0210612376458)) ;
#33958=CARTESIAN_POINT('Ctrl Pts',(-5.55468259057673,21.4259042972473,-12.0108986447266)) ;
#33959=CARTESIAN_POINT('Ctrl Pts',(-5.98446777763594,21.3098553447335,-12.0007360518074)) ;
#33960=CARTESIAN_POINT('Ctrl Pts',(-6.41031317178666,21.1809754284858,-11.9905734588883)) ;
#33961=CARTESIAN_POINT('Ctrl Pts',(-6.47052696485443,21.1627520340001,-11.9891364860444)) ;
#33962=CARTESIAN_POINT('Ctrl Pts',(-6.53066201211327,21.1442721856697,-11.9876995132006)) ;
#33963=CARTESIAN_POINT('Ctrl Pts',(-6.5907160980845,21.1255365938229,-11.9862625403567)) ;
#33964=CARTESIAN_POINT('Ctrl Pts',(-7.02679782691396,20.9894884107383,-11.9758279863728)) ;
#33965=CARTESIAN_POINT('Ctrl Pts',(-7.45872200889061,20.839915354729,-11.9653934323889)) ;
#33966=CARTESIAN_POINT('Ctrl Pts',(-7.88564361724271,20.677099888629,-11.954958878405)) ;
#33967=CARTESIAN_POINT('Ctrl Pts',(-8.30137771702621,20.5185510124284,-11.9447977625883)) ;
#33968=CARTESIAN_POINT('Ctrl Pts',(-8.71236784836556,20.3474449705746,-11.9346366467715)) ;
#33969=CARTESIAN_POINT('Ctrl Pts',(-9.11785160959659,20.1640922703671,-11.9244755309547)) ;
#33970=CARTESIAN_POINT('Ctrl Pts',(-9.52329367665906,19.980758423537,-11.9143154599623)) ;
#33971=CARTESIAN_POINT('Ctrl Pts',(-9.92323029549759,19.7851805282727,-11.9041553889698)) ;
#33972=CARTESIAN_POINT('Ctrl Pts',(-10.3169202058506,19.5777167343031,-11.8939953179773)) ;
#33973=CARTESIAN_POINT('Ctrl Pts',(-10.7105866286583,19.3702653176263,-11.8838358531348)) ;
#33974=CARTESIAN_POINT('Ctrl Pts',(-11.0980068845182,19.1509295259284,-11.8736763882923)) ;
#33975=CARTESIAN_POINT('Ctrl Pts',(-11.4784638584483,18.9201137024278,-11.8635169234497)) ;
#33976=CARTESIAN_POINT('Ctrl Pts',(-11.8769276454528,18.6783734967416,-11.8528766168909)) ;
#33977=CARTESIAN_POINT('Ctrl Pts',(-12.2677529454088,18.4240406018629,-11.842236310332)) ;
#33978=CARTESIAN_POINT('Ctrl Pts',(-12.6501477448703,18.15763192422,-11.8315960037731)) ;
#33979=CARTESIAN_POINT('Ctrl Pts',(-13.0152972849629,17.9032377581514,-11.8214355542798)) ;
#33980=CARTESIAN_POINT('Ctrl Pts',(-13.3727596173026,17.637832923503,-11.8112751047865)) ;
#33981=CARTESIAN_POINT('Ctrl Pts',(-13.7218758315993,17.3619111483924,-11.8011146552932)) ;
#33982=CARTESIAN_POINT('Ctrl Pts',(-14.0710076773342,17.0859770190742,-11.7909537508728)) ;
#33983=CARTESIAN_POINT('Ctrl Pts',(-14.4117924797961,16.7995251526353,-11.7807928464523)) ;
#33984=CARTESIAN_POINT('Ctrl Pts',(-14.7436040222943,16.5030898772408,-11.7706319420319)) ;
#33985=CARTESIAN_POINT('Ctrl Pts',(-15.075470703917,16.2066053414094,-11.7604693491127)) ;
#33986=CARTESIAN_POINT('Ctrl Pts',(-15.3983609749454,15.9001342346632,-11.7503067561935)) ;
#33987=CARTESIAN_POINT('Ctrl Pts',(-15.7116836954442,15.5842494370699,-11.7401441632744)) ;
#33988=CARTESIAN_POINT('Ctrl Pts',(-15.7559869794864,15.5395838798128,-11.7387071904306)) ;
#33989=CARTESIAN_POINT('Ctrl Pts',(-15.800099035216,15.4947301704647,-11.7372702175868)) ;
#33990=CARTESIAN_POINT('Ctrl Pts',(-15.844018251497,15.4496899874635,-11.735833244743)) ;
#33991=CARTESIAN_POINT('Ctrl Pts',(-16.1629368971697,15.1226314609247,-11.725398690759)) ;
#33992=CARTESIAN_POINT('Ctrl Pts',(-16.4717664484133,14.7856523720499,-11.7149641367751)) ;
#33993=CARTESIAN_POINT('Ctrl Pts',(-16.7698978695481,14.4394030523228,-11.7045295827912)) ;
#33994=CARTESIAN_POINT('Ctrl Pts',(-17.0602167373648,14.1022272185817,-11.6943684669744)) ;
#33995=CARTESIAN_POINT('Ctrl Pts',(-17.3403908348353,13.7562609764049,-11.6842073511576)) ;
#33996=CARTESIAN_POINT('Ctrl Pts',(-17.609897147207,13.402140035356,-11.6740462353408)) ;
#33997=CARTESIAN_POINT('Ctrl Pts',(-17.8793757473911,13.0480555070571,-11.6638861643483)) ;
#33998=CARTESIAN_POINT('Ctrl Pts',(-18.138188614594,12.685818137402,-11.6537260933558)) ;
#33999=CARTESIAN_POINT('Ctrl Pts',(-18.3858539882545,12.3160954926911,-11.6435660223633)) ;
#34000=CARTESIAN_POINT('Ctrl Pts',(-18.6335045861991,11.9463949056329,-11.6334065575206)) ;
#34001=CARTESIAN_POINT('Ctrl Pts',(-18.8700088915731,11.569210126359,-11.6232470926779)) ;
#34002=CARTESIAN_POINT('Ctrl Pts',(-19.0949283514416,11.1852378747979,-11.6130876278352)) ;
#34003=CARTESIAN_POINT('Ctrl Pts',(-19.3304931219399,10.7830924340715,-11.6024473212764)) ;
#34004=CARTESIAN_POINT('Ctrl Pts',(-19.5533499527906,10.3735018220648,-11.5918070147175)) ;
#34005=CARTESIAN_POINT('Ctrl Pts',(-19.7630479330817,9.95729739724672,-11.5811667081587)) ;
#34006=CARTESIAN_POINT('Ctrl Pts',(-19.9632889436028,9.55986297993257,-11.5710062586654)) ;
#34007=CARTESIAN_POINT('Ctrl Pts',(-20.1515314844915,9.15639824653307,-11.560845809172)) ;
#34008=CARTESIAN_POINT('Ctrl Pts',(-20.3274307117808,8.74765086867624,-11.5506853596787)) ;
#34009=CARTESIAN_POINT('Ctrl Pts',(-20.5033378148358,8.33888518943948,-11.5405244552583)) ;
#34010=CARTESIAN_POINT('Ctrl Pts',(-20.6669004115264,7.9248366049264,-11.530363550838)) ;
#34011=CARTESIAN_POINT('Ctrl Pts',(-20.8178217254164,7.50627295475458,-11.5202026464176)) ;
#34012=CARTESIAN_POINT('Ctrl Pts',(-20.9687681188101,7.08763974934033,-11.5100400534985)) ;
#34013=CARTESIAN_POINT('Ctrl Pts',(-21.1070689541603,6.66449019500752,-11.4998774605794)) ;
#34014=CARTESIAN_POINT('Ctrl Pts',(-21.2324766450028,6.23760936432466,-11.4897148676604)) ;
#34015=CARTESIAN_POINT('Ctrl Pts',(-21.2502090728956,6.17724916234625,-11.4882778948166)) ;
#34016=CARTESIAN_POINT('Ctrl Pts',(-21.267683803721,6.11681438357297,-11.4868409219728)) ;
#34017=CARTESIAN_POINT('Ctrl Pts',(-21.2849002183608,6.05630727068284,-11.4854039491291)) ;
#34018=CARTESIAN_POINT('Ctrl Pts',(-21.4099169218747,5.61693589453045,-11.4749693951451)) ;
#34019=CARTESIAN_POINT('Ctrl Pts',(-21.5213406419892,5.17363537269906,-11.4645348411612)) ;
#34020=CARTESIAN_POINT('Ctrl Pts',(-21.618944881532,4.72726742122561,-11.4541002871773)) ;
#34021=CARTESIAN_POINT('Ctrl Pts',(-21.7139913956172,4.29259657100826,-11.4439391713605)) ;
#34022=CARTESIAN_POINT('Ctrl Pts',(-21.7959333929137,3.85501723569015,-11.4337780555437)) ;
#34023=CARTESIAN_POINT('Ctrl Pts',(-21.8646130944639,3.41533736135931,-11.423616939727)) ;
#34024=CARTESIAN_POINT('Ctrl Pts',(-21.9332857339723,2.97570269744167,-11.4134568687345)) ;
#34025=CARTESIAN_POINT('Ctrl Pts',(-21.9886987663005,2.53396815266412,-11.4032967977421)) ;
#34026=CARTESIAN_POINT('Ctrl Pts',(-22.0307458528026,2.09095007872548,-11.3931367267497)) ;
#34027=CARTESIAN_POINT('Ctrl Pts',(-22.0727904307749,1.64795843525155,-11.3829772619072)) ;
#34028=CARTESIAN_POINT('Ctrl Pts',(-22.1014706343473,1.20368364405753,-11.3728177970648)) ;
#34029=CARTESIAN_POINT('Ctrl Pts',(-22.1167319981389,0.758947155603138,
-11.3626583322224)) ;
#34030=CARTESIAN_POINT('Ctrl Pts',(-22.1327156736345,0.293161541057203,
-11.3520180256634)) ;
#34031=CARTESIAN_POINT('Ctrl Pts',(-22.1339797673999,-0.17313025446473,
-11.3413777191045)) ;
#34032=CARTESIAN_POINT('Ctrl Pts',(-22.1205229701666,-0.638982463634,-11.3307374125456)) ;
#34033=CARTESIAN_POINT('Ctrl Pts',(-22.1076730482332,-1.08382564708693,
-11.3205769630523)) ;
#34034=CARTESIAN_POINT('Ctrl Pts',(-22.0814004911738,-1.52826776709898,
-11.3104165135591)) ;
#34035=CARTESIAN_POINT('Ctrl Pts',(-22.041757498408,-1.97148711481321,-11.3002560640658)) ;
#34036=CARTESIAN_POINT('Ctrl Pts',(-22.0021127306535,-2.41472630738025,
-11.2900951596452)) ;
#34037=CARTESIAN_POINT('Ctrl Pts',(-21.9490963538971,-2.85674238987022,
-11.2799342552245)) ;
#34038=CARTESIAN_POINT('Ctrl Pts',(-21.8828124429122,-3.2967187703575,-11.2697733508038)) ;
#34039=CARTESIAN_POINT('Ctrl Pts',(-21.8165175171327,-3.73676826435554,
-11.2596107578848)) ;
#34040=CARTESIAN_POINT('Ctrl Pts',(-21.7369506859879,-4.17477715213099,
-11.2494481649658)) ;
#34041=CARTESIAN_POINT('Ctrl Pts',(-21.6442674912479,-4.60993707438697,
-11.2392855720468)) ;
#34042=CARTESIAN_POINT('Ctrl Pts',(-21.6311622498018,-4.67146792542045,
-11.2378485992029)) ;
#34043=CARTESIAN_POINT('Ctrl Pts',(-21.6177948501307,-4.73294183313134,
-11.2364116263591)) ;
#34044=CARTESIAN_POINT('Ctrl Pts',(-21.6041658141075,-4.79435653023914,
-11.2349746535153)) ;
#34045=CARTESIAN_POINT('Ctrl Pts',(-21.5051987997055,-5.24031831380347,
-11.2245400995313)) ;
#34046=CARTESIAN_POINT('Ctrl Pts',(-21.3924056844949,-5.68327238729325,
-11.2141055455474)) ;
#34047=CARTESIAN_POINT('Ctrl Pts',(-21.2659970100249,-6.12235299799939,
-11.2036709915635)) ;
#34048=CARTESIAN_POINT('Ctrl Pts',(-21.1429008831067,-6.54992747268951,
-11.1935098757467)) ;
#34049=CARTESIAN_POINT('Ctrl Pts',(-21.0068937286801,-6.97382866349173,
-11.1833487599299)) ;
#34050=CARTESIAN_POINT('Ctrl Pts',(-20.8582209686787,-7.39327079743941,
-11.1731876441131)) ;
#34051=CARTESIAN_POINT('Ctrl Pts',(-20.7095634960657,-7.81266980193434,
-11.1630275731207)) ;
#34052=CARTESIAN_POINT('Ctrl Pts',(-20.5482430959642,-8.22761044915114,
-11.1528675021283)) ;
#34053=CARTESIAN_POINT('Ctrl Pts',(-20.3745544390668,-8.63732403421366,
-11.1427074311358)) ;
#34054=CARTESIAN_POINT('Ctrl Pts',(-20.2008761444342,-9.04701317576482,
-11.1325479662932)) ;
#34055=CARTESIAN_POINT('Ctrl Pts',(-20.0148311567656,-9.45147566690294,
-11.1223885014506)) ;
#34056=CARTESIAN_POINT('Ctrl Pts',(-19.8167622038062,-9.84996298573239,
-11.112229036608)) ;
#34057=CARTESIAN_POINT('Ctrl Pts',(-19.6093187594976,-10.2673104836424,
-11.1015887300491)) ;
#34058=CARTESIAN_POINT('Ctrl Pts',(-19.38868594734,-10.6781033739189,-11.0909484234902)) ;
#34059=CARTESIAN_POINT('Ctrl Pts',(-19.1553123747469,-11.0815090528488,
-11.0803081169313)) ;
#34060=CARTESIAN_POINT('Ctrl Pts',(-18.9324634949436,-11.4667219227418,
-11.070147667438)) ;
#34061=CARTESIAN_POINT('Ctrl Pts',(-18.6979975965305,-11.8451988543758,
-11.0599872179446)) ;
#34062=CARTESIAN_POINT('Ctrl Pts',(-18.452351361982,-12.2162418229365,-11.0498267684513)) ;
#34063=CARTESIAN_POINT('Ctrl Pts',(-18.2066941287932,-12.5873014046895,
-11.0396658640309)) ;
#34064=CARTESIAN_POINT('Ctrl Pts',(-17.9498556879653,-12.9509261682689,
-11.0295049596105)) ;
#34065=CARTESIAN_POINT('Ctrl Pts',(-17.6823159227956,-13.306447259466,-11.01934405519)) ;
#34066=CARTESIAN_POINT('Ctrl Pts',(-17.4147316989321,-13.6620274297435,
-11.0091814622709)) ;
#34067=CARTESIAN_POINT('Ctrl Pts',(-17.1364427354867,-14.0095010535141,
-10.9990188693518)) ;
#34068=CARTESIAN_POINT('Ctrl Pts',(-16.8479702756838,-14.3482309938256,
-10.9888562764327)) ;
#34069=CARTESIAN_POINT('Ctrl Pts',(-16.8071807749903,-14.3961268142608,
-10.9874193035889)) ;
#34070=CARTESIAN_POINT('Ctrl Pts',(-16.7661877359645,-14.4438478730751,
-10.9859823307451)) ;
#34071=CARTESIAN_POINT('Ctrl Pts',(-16.7249926958962,-14.4913924239432,
-10.9845453579013)) ;
#34072=CARTESIAN_POINT('Ctrl Pts',(-16.4258556096824,-14.8366363753617,
-10.9741108039174)) ;
#34073=CARTESIAN_POINT('Ctrl Pts',(-16.115986170001,-15.1726594823227,-10.9636762499335)) ;
#34074=CARTESIAN_POINT('Ctrl Pts',(-15.7959812961833,-15.4988002746383,
-10.9532416959496)) ;
#34075=CARTESIAN_POINT('Ctrl Pts',(-15.4843621709359,-15.8163945262395,
-10.9430805801328)) ;
#34076=CARTESIAN_POINT('Ctrl Pts',(-15.163132185395,-16.1246175980715,-10.932919464316)) ;
#34077=CARTESIAN_POINT('Ctrl Pts',(-14.8328809084565,-16.4228949645928,
-10.9227583484991)) ;
#34078=CARTESIAN_POINT('Ctrl Pts',(-14.502663589852,-16.7211416605213,-10.9125982775066)) ;
#34079=CARTESIAN_POINT('Ctrl Pts',(-14.1634270030494,-17.009444540111,-10.9024382065141)) ;
#34080=CARTESIAN_POINT('Ctrl Pts',(-13.8157959238133,-17.2872675126535,
-10.8922781355216)) ;
#34081=CARTESIAN_POINT('Ctrl Pts',(-13.4681855842518,-17.5650739102738,
-10.882118670679)) ;
#34082=CARTESIAN_POINT('Ctrl Pts',(-13.1121819320761,-17.8324015066964,
-10.8719592058365)) ;
#34083=CARTESIAN_POINT('Ctrl Pts',(-12.7484424203036,-18.0887548194646,
-10.8617997409939)) ;
#34084=CARTESIAN_POINT('Ctrl Pts',(-12.3674873234739,-18.3572411893184,
-10.8511594344351)) ;
#34085=CARTESIAN_POINT('Ctrl Pts',(-11.9780467254352,-18.6136893460692,
-10.8405191278762)) ;
#34086=CARTESIAN_POINT('Ctrl Pts',(-11.5809112054464,-18.8575801924337,
-10.8298788213173)) ;
#34087=CARTESIAN_POINT('Ctrl Pts',(-11.201685722563,-19.0904720374795,-10.8197183718241)) ;
#34088=CARTESIAN_POINT('Ctrl Pts',(-10.8154441484443,-19.3119138847356,
-10.8095579223309)) ;
#34089=CARTESIAN_POINT('Ctrl Pts',(-10.4229025731864,-19.5214993535938,
-10.7993974728376)) ;
#34090=CARTESIAN_POINT('Ctrl Pts',(-10.0303434221401,-19.7310942065023,
-10.789236568417)) ;
#34091=CARTESIAN_POINT('Ctrl Pts',(-9.63148390994459,-19.9288315143467,
-10.7790756639964)) ;
#34092=CARTESIAN_POINT('Ctrl Pts',(-9.22706425791738,-20.1143511017075,
-10.7689147595758)) ;
#34093=CARTESIAN_POINT('Ctrl Pts',(-8.82257740104682,-20.2999015179728,
-10.7587521666567)) ;
#34094=CARTESIAN_POINT('Ctrl Pts',(-8.41252876678408,-20.4732300613035,
-10.7485895737375)) ;
#34095=CARTESIAN_POINT('Ctrl Pts',(-7.99767987719359,-20.6340241262928,
-10.7384269808184)) ;
#34096=CARTESIAN_POINT('Ctrl Pts',(-7.93902097062444,-20.6567601255247,
-10.7369900079748)) ;
#34097=CARTESIAN_POINT('Ctrl Pts',(-7.88026612142671,-20.6792455963373,
-10.7355530351312)) ;
#34098=CARTESIAN_POINT('Ctrl Pts',(-7.82141751240148,-20.7014797335649,
-10.7341160622875)) ;
#34099=CARTESIAN_POINT('Ctrl Pts',(-7.40624151015085,-20.8583412186629,
-10.7239782416927)) ;
#34100=CARTESIAN_POINT('Ctrl Pts',(-6.98628722558425,-21.0027307383675,
-10.7138404210978)) ;
#34101=CARTESIAN_POINT('Ctrl Pts',(-6.56232615274566,-21.1343727261419,
-10.703702600503)) ;
#34102=CARTESIAN_POINT('Ctrl Pts',(-6.13843308668183,-21.26599359748,-10.6935664060963)) ;
#34103=CARTESIAN_POINT('Ctrl Pts',(-5.71053473731159,-21.3848709522725,
-10.6834302116896)) ;
#34104=CARTESIAN_POINT('Ctrl Pts',(-5.27941863444923,-21.4907788119633,
-10.673294017283)) ;
#34105=CARTESIAN_POINT('Ctrl Pts',(-4.84800360564933,-21.5967601057152,
-10.6631507946735)) ;
#34106=CARTESIAN_POINT('Ctrl Pts',(-4.41336658261689,-21.6897538469575,
-10.6530075720639)) ;
#34107=CARTESIAN_POINT('Ctrl Pts',(-3.97630984636663,-21.7695841730656,
-10.6428643494544)) ;
#34108=CARTESIAN_POINT('Ctrl Pts',(-3.53961532798087,-21.8493483384951,
-10.6327295332053)) ;
#34109=CARTESIAN_POINT('Ctrl Pts',(-3.10050533466276,-21.915970861745,-10.6225947169562)) ;
#34110=CARTESIAN_POINT('Ctrl Pts',(-2.65978984330864,-21.9693275512004,
-10.612459900707)) ;
#34111=CARTESIAN_POINT('Ctrl Pts',(-2.21852602234166,-22.0227506260074,
-10.6023124749173)) ;
#34112=CARTESIAN_POINT('Ctrl Pts',(-1.77565293561,-22.0628747976657,-10.5921650491276)) ;
#34113=CARTESIAN_POINT('Ctrl Pts',(-1.331989863321,-22.0896273863212,-10.5820176233379)) ;
#34114=CARTESIAN_POINT('Ctrl Pts',(-0.888326791031996,-22.1163799749766,
-10.5718701975482)) ;
#34115=CARTESIAN_POINT('Ctrl Pts',(-0.443873966088516,-22.1297609690224,
-10.5617227717585)) ;
#34116=CARTESIAN_POINT('Ctrl Pts',(0.000546534359808369,-22.1297499932512,
-10.5515753459688)) ;
#34117=CARTESIAN_POINT('Ctrl Pts',(0.000544184811332343,-22.1297499933091,
-10.0859246540312)) ;
#34118=CARTESIAN_POINT('Ctrl Pts',(-0.443392383725113,-22.1297609099953,
-10.0960609647218)) ;
#34119=CARTESIAN_POINT('Ctrl Pts',(-0.887360401803858,-22.1164090174797,
-10.1061972754123)) ;
#34120=CARTESIAN_POINT('Ctrl Pts',(-1.3305405724524,-22.0897147298818,-10.1163335861029)) ;
#34121=CARTESIAN_POINT('Ctrl Pts',(-1.77369351406842,-22.0630220823836,
-10.1264692740175)) ;
#34122=CARTESIAN_POINT('Ctrl Pts',(-2.21605847372859,-22.0229886914173,
-10.1366049619322)) ;
#34123=CARTESIAN_POINT('Ctrl Pts',(-2.65681909988972,-21.969687010355,-10.1467406498468)) ;
#34124=CARTESIAN_POINT('Ctrl Pts',(-3.09762117372998,-21.916380316978,-10.1568772908882)) ;
#34125=CARTESIAN_POINT('Ctrl Pts',(-3.53681838216302,-21.8498028649715,
-10.1670139319296)) ;
#34126=CARTESIAN_POINT('Ctrl Pts',(-3.97360040099842,-21.7700788908925,
-10.177150572971)) ;
#34127=CARTESIAN_POINT('Ctrl Pts',(-4.41038596564575,-21.6903542696116,
-10.187287296302)) ;
#34128=CARTESIAN_POINT('Ctrl Pts',(-4.844756073909,-21.5974829566014,-10.197424019633)) ;
#34129=CARTESIAN_POINT('Ctrl Pts',(-5.27591007353012,-21.491640420371,-10.207560742964)) ;
#34130=CARTESIAN_POINT('Ctrl Pts',(-5.70715822137385,-21.385774772012,-10.2176996797837)) ;
#34131=CARTESIAN_POINT('Ctrl Pts',(-6.13518863136855,-21.2669322928212,
-10.2278386166034)) ;
#34132=CARTESIAN_POINT('Ctrl Pts',(-6.55921321524739,-21.13533905712,-10.237977553423)) ;
#34133=CARTESIAN_POINT('Ctrl Pts',(-6.97217961022537,-21.0071776574816,
-10.2478520756713)) ;
#34134=CARTESIAN_POINT('Ctrl Pts',(-7.38134625824425,-20.8669221562401,
-10.2577265979196)) ;
#34135=CARTESIAN_POINT('Ctrl Pts',(-7.78600007850508,-20.7148265220836,
-10.2676011201678)) ;
#34136=CARTESIAN_POINT('Ctrl Pts',(-8.21360376667814,-20.5541048116635,
-10.2780356741518)) ;
#34137=CARTESIAN_POINT('Ctrl Pts',(-8.63628456897859,-20.3801176356223,
-10.2884702281357)) ;
#34138=CARTESIAN_POINT('Ctrl Pts',(-9.05321496226866,-20.1931952377392,
-10.2989047821196)) ;
#34139=CARTESIAN_POINT('Ctrl Pts',(-9.45921966743386,-20.0111711534733,
-10.3090658979364)) ;
#34140=CARTESIAN_POINT('Ctrl Pts',(-9.85977126683292,-19.8168812107641,
-10.3192270137532)) ;
#34141=CARTESIAN_POINT('Ctrl Pts',(-10.254126328709,-19.610678935146,-10.32938812957)) ;
#34142=CARTESIAN_POINT('Ctrl Pts',(-10.6484408407306,-19.4044978624312,
-10.3395482005625)) ;
#34143=CARTESIAN_POINT('Ctrl Pts',(-11.0365598846075,-19.1864070098415,
-10.3497082715549)) ;
#34144=CARTESIAN_POINT('Ctrl Pts',(-11.4177638553577,-18.9568062607019,
-10.3598683425474)) ;
#34145=CARTESIAN_POINT('Ctrl Pts',(-11.7989450834734,-18.7272192095464,
-10.3700278073899)) ;
#34146=CARTESIAN_POINT('Ctrl Pts',(-12.1732118661025,-18.4861237521248,
-10.3801872722323)) ;
#34147=CARTESIAN_POINT('Ctrl Pts',(-12.5398713412977,-18.2339645114879,
-10.3903467370748)) ;
#34148=CARTESIAN_POINT('Ctrl Pts',(-12.9238846017689,-17.969870716821,-10.4009870436337)) ;
#34149=CARTESIAN_POINT('Ctrl Pts',(-13.2995529305382,-17.6936408428704,
-10.4116273501926)) ;
#34150=CARTESIAN_POINT('Ctrl Pts',(-13.6661151154515,-17.4058361681859,
-10.4222676567515)) ;
#34151=CARTESIAN_POINT('Ctrl Pts',(-14.01614606102,-17.1310109227976,-10.4324281062448)) ;
#34152=CARTESIAN_POINT('Ctrl Pts',(-14.3578737493921,-16.8456318200322,
-10.442588555738)) ;
#34153=CARTESIAN_POINT('Ctrl Pts',(-14.6906685312681,-16.5502293992232,
-10.4527490052313)) ;
#34154=CARTESIAN_POINT('Ctrl Pts',(-15.0234782138073,-16.2548137519687,
-10.4629099096519)) ;
#34155=CARTESIAN_POINT('Ctrl Pts',(-15.3473540206489,-15.9493740441314,
-10.4730708140725)) ;
#34156=CARTESIAN_POINT('Ctrl Pts',(-15.6617012605832,-15.6344794824371,
-10.483231718493)) ;
#34157=CARTESIAN_POINT('Ctrl Pts',(-15.9761007374898,-15.3195325928188,
-10.4933943114122)) ;
#34158=CARTESIAN_POINT('Ctrl Pts',(-16.2809683214846,-14.9951278724074,
-10.5035569043314)) ;
#34159=CARTESIAN_POINT('Ctrl Pts',(-16.5757465417907,-14.6618710144652,
-10.5137194972506)) ;
#34160=CARTESIAN_POINT('Ctrl Pts',(-16.6174276659735,-14.6147490782983,
-10.5151564700943)) ;
#34161=CARTESIAN_POINT('Ctrl Pts',(-16.6589071323296,-14.5674502139036,
-10.516593442938)) ;
#34162=CARTESIAN_POINT('Ctrl Pts',(-16.7001834281708,-14.5199761889595,
-10.5180304157816)) ;
#34163=CARTESIAN_POINT('Ctrl Pts',(-16.999910551831,-14.175244360313,-10.5284649697656)) ;
#34164=CARTESIAN_POINT('Ctrl Pts',(-17.2889986817735,-13.8211841236492,
-10.5388995237495)) ;
#34165=CARTESIAN_POINT('Ctrl Pts',(-17.5668769022766,-13.4584795189784,
-10.5493340777334)) ;
#34166=CARTESIAN_POINT('Ctrl Pts',(-17.8374733059035,-13.1052796121086,
-10.5594951935502)) ;
#34167=CARTESIAN_POINT('Ctrl Pts',(-18.0974396498937,-12.7438827864294,
-10.569656309367)) ;
#34168=CARTESIAN_POINT('Ctrl Pts',(-18.3462900644125,-12.3749535730418,
-10.5798174251838)) ;
#34169=CARTESIAN_POINT('Ctrl Pts',(-18.5951148907004,-12.0060622950777,
-10.5899774961762)) ;
#34170=CARTESIAN_POINT('Ctrl Pts',(-18.8328259423312,-11.6296403667387,
-10.6001375671687)) ;
#34171=CARTESIAN_POINT('Ctrl Pts',(-19.0589803550444,-11.2463817687526,
-10.6102976381611)) ;
#34172=CARTESIAN_POINT('Ctrl Pts',(-19.2851212753845,-10.863146035976,-10.6204571030037)) ;
#34173=CARTESIAN_POINT('Ctrl Pts',(-19.4997068176385,-10.4730746460644,
-10.6306165678462)) ;
#34174=CARTESIAN_POINT('Ctrl Pts',(-19.7023389190521,-10.076888219153,-10.6407760326888)) ;
#34175=CARTESIAN_POINT('Ctrl Pts',(-19.914561483048,-9.66195051306934,-10.6514163392477)) ;
#34176=CARTESIAN_POINT('Ctrl Pts',(-20.1136717964291,-9.24030525979585,
-10.6620566458066)) ;
#34177=CARTESIAN_POINT('Ctrl Pts',(-20.2992671449799,-8.81280820392919,
-10.6726969523655)) ;
#34178=CARTESIAN_POINT('Ctrl Pts',(-20.4764925054238,-8.40459043119787,
-10.6828574018587)) ;
#34179=CARTESIAN_POINT('Ctrl Pts',(-20.6413947006628,-7.99103715615273,
-10.693017851352)) ;
#34180=CARTESIAN_POINT('Ctrl Pts',(-20.7936721328555,-7.57291451779358,
-10.7031783008453)) ;
#34181=CARTESIAN_POINT('Ctrl Pts',(-20.9459563831685,-7.15477315827262,
-10.7133392052659)) ;
#34182=CARTESIAN_POINT('Ctrl Pts',(-21.085614664725,-6.73206224313735,-10.7235001096865)) ;
#34183=CARTESIAN_POINT('Ctrl Pts',(-21.2123945201883,-6.30556530236464,
-10.7336610141071)) ;
#34184=CARTESIAN_POINT('Ctrl Pts',(-21.3391954434224,-5.8789974880314,-10.7438236070262)) ;
#34185=CARTESIAN_POINT('Ctrl Pts',(-21.4531135990334,-5.44864261096266,
-10.7539861999454)) ;
#34186=CARTESIAN_POINT('Ctrl Pts',(-21.5539466232426,-5.01529859778159,
-10.7641487928646)) ;
#34187=CARTESIAN_POINT('Ctrl Pts',(-21.568204236303,-4.95402451312071,-10.7655857657082)) ;
#34188=CARTESIAN_POINT('Ctrl Pts',(-21.5822003150699,-4.8926906849236,-10.7670227385519)) ;
#34189=CARTESIAN_POINT('Ctrl Pts',(-21.5959343694665,-4.83129938755548,
-10.7684597113956)) ;
#34190=CARTESIAN_POINT('Ctrl Pts',(-21.6956639730229,-4.38550752074539,
-10.7788942653795)) ;
#34191=CARTESIAN_POINT('Ctrl Pts',(-21.7815984515182,-3.93656892420253,
-10.7893288193634)) ;
#34192=CARTESIAN_POINT('Ctrl Pts',(-21.8535608715591,-3.48535683905719,
-10.7997633733473)) ;
#34193=CARTESIAN_POINT('Ctrl Pts',(-21.9236375116933,-3.04596879600585,
-10.8099244891641)) ;
#34194=CARTESIAN_POINT('Ctrl Pts',(-21.980464965085,-2.60442513320454,-10.8200856049809)) ;
#34195=CARTESIAN_POINT('Ctrl Pts',(-22.023931834818,-2.16154148648363,-10.8302467207977)) ;
#34196=CARTESIAN_POINT('Ctrl Pts',(-22.0673942350375,-1.71870337960595,
-10.8404067917901)) ;
#34197=CARTESIAN_POINT('Ctrl Pts',(-22.0974987733527,-1.27452579240092,
-10.8505668627826)) ;
#34198=CARTESIAN_POINT('Ctrl Pts',(-22.1141858891321,-0.829829815932281,
-10.860726933775)) ;
#34199=CARTESIAN_POINT('Ctrl Pts',(-22.1308720093581,-0.385160370027927,
-10.8708863986176)) ;
#34200=CARTESIAN_POINT('Ctrl Pts',(-22.1341422976873,0.0600271740320306,
-10.8810458634601)) ;
#34201=CARTESIAN_POINT('Ctrl Pts',(-22.1239892732356,0.504909596124077,
-10.8912053283027)) ;
#34202=CARTESIAN_POINT('Ctrl Pts',(-22.1133557118875,0.970848051257177,
-10.9018456348616)) ;
#34203=CARTESIAN_POINT('Ctrl Pts',(-22.0879976776636,1.43645153771628,-10.9124859414205)) ;
#34204=CARTESIAN_POINT('Ctrl Pts',(-22.0479678562076,1.90077575587892,-10.9231262479794)) ;
#34205=CARTESIAN_POINT('Ctrl Pts',(-22.0097433015976,2.34415985773987,-10.9332866974726)) ;
#34206=CARTESIAN_POINT('Ctrl Pts',(-21.9581408990753,2.7863772673351,-10.9434471469659)) ;
#34207=CARTESIAN_POINT('Ctrl Pts',(-21.893259673349,3.22661059593695,-10.9536075964591)) ;
#34208=CARTESIAN_POINT('Ctrl Pts',(-21.8283755426094,3.66686363568972,-10.9637685008797)) ;
#34209=CARTESIAN_POINT('Ctrl Pts',(-21.7502114365678,4.10513219023872,-10.9739294053002)) ;
#34210=CARTESIAN_POINT('Ctrl Pts',(-21.6589178785627,4.54060694094708,-10.9840903097208)) ;
#34211=CARTESIAN_POINT('Ctrl Pts',(-21.5676091497579,4.97615405711429,-10.9942529026399)) ;
#34212=CARTESIAN_POINT('Ctrl Pts',(-21.4631666566022,5.40890621715232,-11.0044154955591)) ;
#34213=CARTESIAN_POINT('Ctrl Pts',(-21.3457918355023,5.83806525981865,-11.0145780884782)) ;
#34214=CARTESIAN_POINT('Ctrl Pts',(-21.3291952413263,5.89874759697905,-11.0160150613219)) ;
#34215=CARTESIAN_POINT('Ctrl Pts',(-21.3123401673082,5.95935811737186,-11.0174520341656)) ;
#34216=CARTESIAN_POINT('Ctrl Pts',(-21.2952272639061,6.01989458720738,-11.0188890070094)) ;
#34217=CARTESIAN_POINT('Ctrl Pts',(-21.1709622054873,6.4594791383414,-11.0293235609933)) ;
#34218=CARTESIAN_POINT('Ctrl Pts',(-21.0330653019663,6.89527156835765,-11.0397581149772)) ;
#34219=CARTESIAN_POINT('Ctrl Pts',(-20.8817961763543,7.32641955607873,-11.0501926689611)) ;
#34220=CARTESIAN_POINT('Ctrl Pts',(-20.7344910680365,7.74626928268595,-11.0603537847779)) ;
#34221=CARTESIAN_POINT('Ctrl Pts',(-20.5745056923739,8.16171464033577,-11.0705149005947)) ;
#34222=CARTESIAN_POINT('Ctrl Pts',(-20.4021299299239,8.57198514843583,-11.0806760164115)) ;
#34223=CARTESIAN_POINT('Ctrl Pts',(-20.2297718921408,8.98221347016345,-11.0908360874039)) ;
#34224=CARTESIAN_POINT('Ctrl Pts',(-20.0450261013507,9.38726779366562,-11.1009961583964)) ;
#34225=CARTESIAN_POINT('Ctrl Pts',(-19.848230632152,9.78639749015959,-11.1111562293888)) ;
#34226=CARTESIAN_POINT('Ctrl Pts',(-19.6514469037722,10.1855033745736,-11.1213156942314)) ;
#34227=CARTESIAN_POINT('Ctrl Pts',(-19.4426150346879,10.5786851323224,-11.131475159074)) ;
#34228=CARTESIAN_POINT('Ctrl Pts',(-19.2221199259505,10.9652150282097,-11.1416346239165)) ;
#34229=CARTESIAN_POINT('Ctrl Pts',(-18.9911889086123,11.370039165126,-11.1522749304754)) ;
#34230=CARTESIAN_POINT('Ctrl Pts',(-18.7474642290177,11.7675664183543,-11.1629152370343)) ;
#34231=CARTESIAN_POINT('Ctrl Pts',(-18.4914412953425,12.1569911525592,-11.1735555435932)) ;
#34232=CARTESIAN_POINT('Ctrl Pts',(-18.2469644964523,12.5288535910541,-11.1837159930865)) ;
#34233=CARTESIAN_POINT('Ctrl Pts',(-17.9912741721608,12.893327874591,-11.1938764425798)) ;
#34234=CARTESIAN_POINT('Ctrl Pts',(-17.7248461421975,13.2497420464674,-11.2040368920731)) ;
#34235=CARTESIAN_POINT('Ctrl Pts',(-17.458406183098,13.6061721765492,-11.2141977964937)) ;
#34236=CARTESIAN_POINT('Ctrl Pts',(-17.1812276970607,13.9545412915113,-11.2243587009142)) ;
#34237=CARTESIAN_POINT('Ctrl Pts',(-16.893827968865,14.2942090239683,-11.2345196053348)) ;
#34238=CARTESIAN_POINT('Ctrl Pts',(-16.6063804817296,14.6339332010532,-11.244682198254)) ;
#34239=CARTESIAN_POINT('Ctrl Pts',(-16.3087085068463,14.9649529312239,-11.2548447911731)) ;
#34240=CARTESIAN_POINT('Ctrl Pts',(-16.0013688107662,15.2866618738147,-11.2650073840922)) ;
#34241=CARTESIAN_POINT('Ctrl Pts',(-15.9579115159039,15.3321509549725,-11.2664443569359)) ;
#34242=CARTESIAN_POINT('Ctrl Pts',(-15.9142609916012,15.3774539397569,-11.2678813297796)) ;
#34243=CARTESIAN_POINT('Ctrl Pts',(-15.8704188723364,15.4225691724527,-11.2693183026233)) ;
#34244=CARTESIAN_POINT('Ctrl Pts',(-15.5520600653141,15.7501726711075,-11.2797528566072)) ;
#34245=CARTESIAN_POINT('Ctrl Pts',(-15.2235128156921,16.0679576657595,-11.2901874105911)) ;
#34246=CARTESIAN_POINT('Ctrl Pts',(-14.8854108318645,16.375297842455,-11.300621964575)) ;
#34247=CARTESIAN_POINT('Ctrl Pts',(-14.556168832556,16.6745841497919,-11.3107830803918)) ;
#34248=CARTESIAN_POINT('Ctrl Pts',(-14.2178666372514,16.9639658877613,-11.3209441962086)) ;
#34249=CARTESIAN_POINT('Ctrl Pts',(-13.8711256523269,17.24290312563,-11.3311053120254)) ;
#34250=CARTESIAN_POINT('Ctrl Pts',(-13.5244203213032,17.5218116815687,-11.3412653830178)) ;
#34251=CARTESIAN_POINT('Ctrl Pts',(-13.1692781127201,17.7902777388003,-11.3514254540103)) ;
#34252=CARTESIAN_POINT('Ctrl Pts',(-12.8063533882028,18.0478017486609,-11.3615855250028)) ;
#34253=CARTESIAN_POINT('Ctrl Pts',(-12.4434503157737,18.3053103946397,-11.3717449898454)) ;
#34254=CARTESIAN_POINT('Ctrl Pts',(-12.0727658421736,18.5518781646479,-11.381904454688)) ;
#34255=CARTESIAN_POINT('Ctrl Pts',(-11.6949846347086,18.7870479175529,-11.3920639195307)) ;
#34256=CARTESIAN_POINT('Ctrl Pts',(-11.2993232566861,19.0333481216525,-11.4027042260896)) ;
#34257=CARTESIAN_POINT('Ctrl Pts',(-10.8958774642939,19.2671453181775,-11.4133445326484)) ;
#34258=CARTESIAN_POINT('Ctrl Pts',(-10.4854661821076,19.4879663897077,-11.4239848392073)) ;
#34259=CARTESIAN_POINT('Ctrl Pts',(-10.0935636479973,19.6988288617544,-11.4341452887006)) ;
#34260=CARTESIAN_POINT('Ctrl Pts',(-9.69531013249103,19.8978594691585,-11.4443057381939)) ;
#34261=CARTESIAN_POINT('Ctrl Pts',(-9.29144375761979,20.0846933748436,-11.4544661876872)) ;
#34262=CARTESIAN_POINT('Ctrl Pts',(-8.88755929990611,20.2715356458899,-11.4646270921077)) ;
#34263=CARTESIAN_POINT('Ctrl Pts',(-8.47806169000838,20.4461800299017,-11.4747879965283)) ;
#34264=CARTESIAN_POINT('Ctrl Pts',(-8.06371050402149,20.6083091972591,-11.4849489009488)) ;
#34265=CARTESIAN_POINT('Ctrl Pts',(-7.6492904628022,20.7704653065968,-11.495111493868)) ;
#34266=CARTESIAN_POINT('Ctrl Pts',(-7.23001544766253,20.9201019601147,-11.5052740867872)) ;
#34267=CARTESIAN_POINT('Ctrl Pts',(-6.80666358498739,21.0569505366591,-11.5154366797064)) ;
#34268=CARTESIAN_POINT('Ctrl Pts',(-6.74680237291455,21.076300685754,-11.51687365255)) ;
#34269=CARTESIAN_POINT('Ctrl Pts',(-6.68685967706741,21.0953952377611,-11.5183106253936)) ;
#34270=CARTESIAN_POINT('Ctrl Pts',(-6.62683772265301,21.1142335134412,-11.5197475982372)) ;
#34271=CARTESIAN_POINT('Ctrl Pts',(-6.19098931650444,21.2510273334671,-11.5301821522211)) ;
#34272=CARTESIAN_POINT('Ctrl Pts',(-5.75084743422553,21.3743388151877,-11.540616706205)) ;
#34273=CARTESIAN_POINT('Ctrl Pts',(-5.30726738537913,21.4839183568219,-11.5510512601889)) ;
#34274=CARTESIAN_POINT('Ctrl Pts',(-4.87531138061828,21.590626359427,-11.5612123760057)) ;
#34275=CARTESIAN_POINT('Ctrl Pts',(-4.44009533416375,21.6843128500613,-11.5713734918225)) ;
#34276=CARTESIAN_POINT('Ctrl Pts',(-4.00242265413292,21.7647983670923,-11.5815346076393)) ;
#34277=CARTESIAN_POINT('Ctrl Pts',(-3.56479497812494,21.8452756081394,-11.5916946786317)) ;
#34278=CARTESIAN_POINT('Ctrl Pts',(-3.12471139879775,21.9125545454665,-11.6018547496242)) ;
#34279=CARTESIAN_POINT('Ctrl Pts',(-2.68298511096576,21.9665069129535,-11.6120148206166)) ;
#34280=CARTESIAN_POINT('Ctrl Pts',(-2.24128517652377,22.0204560616424,-11.6221742854592)) ;
#34281=CARTESIAN_POINT('Ctrl Pts',(-1.79794295716301,22.0610802010845,-11.6323337503018)) ;
#34282=CARTESIAN_POINT('Ctrl Pts',(-1.35377814039208,22.0883027824479,-11.6424932151443)) ;
#34283=CARTESIAN_POINT('Ctrl Pts',(-0.888591254434927,22.1168137931674,
-11.6531335217032)) ;
#34284=CARTESIAN_POINT('Ctrl Pts',(-0.42250230375543,22.130624171767,-11.6637738282621)) ;
#34285=CARTESIAN_POINT('Ctrl Pts',(0.0435433219828738,22.1297071612259,
-11.674414134821)) ;
#34286=CARTESIAN_POINT('Ctrl Pts',(0.48857119929579,22.1288315060709,-11.6845745843143)) ;
#34287=CARTESIAN_POINT('Ctrl Pts',(0.93355932782238,22.1145272841406,-11.6947350338075)) ;
#34288=CARTESIAN_POINT('Ctrl Pts',(1.37768489166807,22.0868245658304,-11.7048954833007)) ;
#34289=CARTESIAN_POINT('Ctrl Pts',(1.82183034094231,22.0591206071493,-11.7150563877214)) ;
#34290=CARTESIAN_POINT('Ctrl Pts',(2.26511291944918,22.018016970129,-11.725217292142)) ;
#34291=CARTESIAN_POINT('Ctrl Pts',(2.70671353053708,21.9635957194196,-11.7353781965627)) ;
#34292=CARTESIAN_POINT('Ctrl Pts',(3.14838752505139,21.9091654252041,-11.7455407894819)) ;
#34293=CARTESIAN_POINT('Ctrl Pts',(3.58837876587045,21.8414131234149,-11.7557033824011)) ;
#34294=CARTESIAN_POINT('Ctrl Pts',(4.02587500114296,21.7604725485839,-11.7658659753202)) ;
#34295=CARTESIAN_POINT('Ctrl Pts',(4.08773620273373,21.7490276930336,-11.7673029481638)) ;
#34296=CARTESIAN_POINT('Ctrl Pts',(4.14954753563977,21.7373192419766,-11.7687399210074)) ;
#34297=CARTESIAN_POINT('Ctrl Pts',(4.21130671935913,21.7253476560901,-11.770176893851)) ;
#34298=CARTESIAN_POINT('Ctrl Pts',(4.65976998670447,21.6384161877862,-11.7806114478349)) ;
#34299=CARTESIAN_POINT('Ctrl Pts',(5.10559865867327,21.5375826947857,-11.7910460018188)) ;
#34300=CARTESIAN_POINT('Ctrl Pts',(5.54792163087631,21.423034347173,-11.8014805558027)) ;
#34301=CARTESIAN_POINT('Ctrl Pts',(5.97865350076954,21.3114877464739,-11.8116416716195)) ;
#34302=CARTESIAN_POINT('Ctrl Pts',(6.40606082013145,21.186935954134,-11.8218027874363)) ;
#34303=CARTESIAN_POINT('Ctrl Pts',(6.82935149681334,21.0496031600473,-11.8319639032532)) ;
#34304=CARTESIAN_POINT('Ctrl Pts',(7.25259864831268,20.9122844873086,-11.8421239742456)) ;
#34305=CARTESIAN_POINT('Ctrl Pts',(7.67172978439449,20.7621875087635,-11.852284045238)) ;
#34306=CARTESIAN_POINT('Ctrl Pts',(8.0859685496601,20.5995861044927,-11.8624441162304)) ;
#34307=CARTESIAN_POINT('Ctrl Pts',(8.50018260144122,20.4369944010216,-11.872603581073)) ;
#34308=CARTESIAN_POINT('Ctrl Pts',(8.90950465192139,20.2618998460975,-11.8827630459156)) ;
#34309=CARTESIAN_POINT('Ctrl Pts',(9.31317722828008,20.0746249025267,-11.8929225107582)) ;
#34310=CARTESIAN_POINT('Ctrl Pts',(9.73595539902207,19.8784863419565,-11.9035628173171)) ;
#34311=CARTESIAN_POINT('Ctrl Pts',(10.1525362281744,19.6689868209902,-11.914203123876)) ;
#34312=CARTESIAN_POINT('Ctrl Pts',(10.5620753425864,19.4465523813356,-11.9248434304349)) ;
#34313=CARTESIAN_POINT('Ctrl Pts',(10.9531450419859,19.2341493009199,-11.9350038799281)) ;
#34314=CARTESIAN_POINT('Ctrl Pts',(11.3377938268513,19.0099521608913,-11.9451643294214)) ;
#34315=CARTESIAN_POINT('Ctrl Pts',(11.7153121750737,18.7743787035169,-11.9553247789147)) ;
#34316=CARTESIAN_POINT('Ctrl Pts',(12.0928474264256,18.5387946984998,-11.9654856833352)) ;
#34317=CARTESIAN_POINT('Ctrl Pts',(12.4632514097936,18.2918334819398,-11.9756465877557)) ;
#34318=CARTESIAN_POINT('Ctrl Pts',(12.8258426006866,18.0339567661929,-11.9858074921763)) ;
#34319=CARTESIAN_POINT('Ctrl Pts',(13.1884940455382,17.7760371975213,-11.9959700850954)) ;
#34320=CARTESIAN_POINT('Ctrl Pts',(13.5433299167266,17.5071986383238,-12.0061326780146)) ;
#34321=CARTESIAN_POINT('Ctrl Pts',(13.8896992826413,17.2279449993403,-12.0162952709337)) ;
#34322=CARTESIAN_POINT('Ctrl Pts',(13.9386753044767,17.1884590237709,-12.0177322437774)) ;
#34323=CARTESIAN_POINT('Ctrl Pts',(13.9874821046735,17.148764881168,-12.0191692166211)) ;
#34324=CARTESIAN_POINT('Ctrl Pts',(14.0361178961741,17.1088640612754,-12.0206061894648)) ;
#34325=CARTESIAN_POINT('Ctrl Pts',(14.3892858729975,16.8191249329445,-12.0310407434487)) ;
#34326=CARTESIAN_POINT('Ctrl Pts',(14.7335251246837,16.5184092272378,-12.0414752974326)) ;
#34327=CARTESIAN_POINT('Ctrl Pts',(15.0681583589428,16.2072958488553,-12.0519098514165)) ;
#34328=CARTESIAN_POINT('Ctrl Pts',(15.3940225074922,15.9043352168266,-12.0620709672334)) ;
#34329=CARTESIAN_POINT('Ctrl Pts',(15.7107774734568,15.5915150493888,-12.0722320830502)) ;
#34330=CARTESIAN_POINT('Ctrl Pts',(16.0178330754948,15.2694092429303,-12.082393198867)) ;
#34331=CARTESIAN_POINT('Ctrl Pts',(16.3248571043089,14.9473365572442,-12.0925532698594)) ;
#34332=CARTESIAN_POINT('Ctrl Pts',(16.6221836030454,14.6159803058319,-12.1027133408518)) ;
#34333=CARTESIAN_POINT('Ctrl Pts',(16.9092598639506,14.2759506133878,-12.1128734118442)) ;
#34334=CARTESIAN_POINT('Ctrl Pts',(17.1963189978866,13.9359412071146,-12.1230328766868)) ;
#34335=CARTESIAN_POINT('Ctrl Pts',(17.4731289676943,13.5872595689571,-12.1331923415294)) ;
#34336=CARTESIAN_POINT('Ctrl Pts',(17.7391767799057,13.2305495816974,-12.143351806372)) ;
#34337=CARTESIAN_POINT('Ctrl Pts',(18.0178164843697,12.8569567127946,-12.1539921129309)) ;
#34338=CARTESIAN_POINT('Ctrl Pts',(18.2846506579833,12.474557496929,-12.1646324194898)) ;
#34339=CARTESIAN_POINT('Ctrl Pts',(18.5391391189094,12.0841282595074,-12.1752727260487)) ;
#34340=CARTESIAN_POINT('Ctrl Pts',(18.782150646777,11.7113066189316,-12.1854331755419)) ;
#34341=CARTESIAN_POINT('Ctrl Pts',(19.0139051079951,11.3311633367331,-12.1955936250352)) ;
#34342=CARTESIAN_POINT('Ctrl Pts',(19.2339770009059,10.944403309049,-12.2057540745284)) ;
#34343=CARTESIAN_POINT('Ctrl Pts',(19.4540587473879,10.5576259644446,-12.215914978949)) ;
#34344=CARTESIAN_POINT('Ctrl Pts',(19.6624567690063,10.164231483083,-12.2260758833696)) ;
#34345=CARTESIAN_POINT('Ctrl Pts',(19.8587911032522,9.76495012685115,-12.2362367877901)) ;
#34346=CARTESIAN_POINT('Ctrl Pts',(20.0551580635548,9.36560241963596,-12.2463993807092)) ;
#34347=CARTESIAN_POINT('Ctrl Pts',(20.2394572295999,8.96036608885079,-12.2565619736284)) ;
#34348=CARTESIAN_POINT('Ctrl Pts',(20.411355618518,8.54999396940693,-12.2667245665475)) ;
#34349=CARTESIAN_POINT('Ctrl Pts',(20.4356617497113,8.49196807029265,-12.2681615393912)) ;
#34350=CARTESIAN_POINT('Ctrl Pts',(20.4597200247701,8.43383952219665,-12.269598512235)) ;
#34351=CARTESIAN_POINT('Ctrl Pts',(20.4835295800864,8.3756104854646,-12.2710354850787)) ;
#34352=CARTESIAN_POINT('Ctrl Pts',(20.6564222630383,7.9527813207642,-12.2814700390626)) ;
#34353=CARTESIAN_POINT('Ctrl Pts',(20.8162405392581,7.52454223258302,-12.2919045930465)) ;
#34354=CARTESIAN_POINT('Ctrl Pts',(20.9626639000163,7.09172456299961,-12.3023391470304)) ;
#34355=CARTESIAN_POINT('Ctrl Pts',(21.1052502270643,6.67024890865189,-12.3125002628472)) ;
#34356=CARTESIAN_POINT('Ctrl Pts',(21.2351346096812,6.24443179677039,-12.322661378664)) ;
#34357=CARTESIAN_POINT('Ctrl Pts',(21.3520707879779,5.8150587381111,-12.3328224944809)) ;
#34358=CARTESIAN_POINT('Ctrl Pts',(21.4689949422243,5.3857298300585,-12.3429825654733)) ;
#34359=CARTESIAN_POINT('Ctrl Pts',(21.5729734913214,4.95284592699653,-12.3531426364658)) ;
#34360=CARTESIAN_POINT('Ctrl Pts',(21.6638103688342,4.51720658877718,-12.3633027074582)) ;
#34361=CARTESIAN_POINT('Ctrl Pts',(21.7546418270177,4.08159324080682,-12.3734621723007)) ;
#34362=CARTESIAN_POINT('Ctrl Pts',(21.8323331331515,3.64322501075395,-12.3836216371431)) ;
#34363=CARTESIAN_POINT('Ctrl Pts',(21.8967392106614,3.20291226898011,-12.3937811019856)) ;
#34364=CARTESIAN_POINT('Ctrl Pts',(21.9641935913388,2.74175977454134,-12.4044214085445)) ;
#34365=CARTESIAN_POINT('Ctrl Pts',(22.0170749229654,2.27847454785169,-12.4150617151035)) ;
#34366=CARTESIAN_POINT('Ctrl Pts',(22.0552771946797,1.81399639700398,-12.4257020216624)) ;
#34367=CARTESIAN_POINT('Ctrl Pts',(22.0917566184751,1.37046530452788,-12.4358624711555)) ;
#34368=CARTESIAN_POINT('Ctrl Pts',(22.1148515219845,0.925846736851711,-12.4460229206486)) ;
#34369=CARTESIAN_POINT('Ctrl Pts',(22.1245228090838,0.480963130427781,-12.4561833701418)) ;
#34370=CARTESIAN_POINT('Ctrl Pts',(22.1341945292086,0.0360596046334728,
-12.4663442745624)) ;
#34371=CARTESIAN_POINT('Ctrl Pts',(22.130441429444,-0.409108754106105,-12.4765051789829)) ;
#34372=CARTESIAN_POINT('Ctrl Pts',(22.113276536622,-0.853718851487109,-12.4866660834035)) ;
#34373=CARTESIAN_POINT('Ctrl Pts',(22.0961087914068,-1.2984028323929,-12.4968286763225)) ;
#34374=CARTESIAN_POINT('Ctrl Pts',(22.06552480876,-1.74252813722489,-12.5069912692414)) ;
#34375=CARTESIAN_POINT('Ctrl Pts',(22.0215896775743,-2.18527415558157,-12.5171538621604)) ;
#34376=CARTESIAN_POINT('Ctrl Pts',(22.015377326955,-2.24787766732996,-12.5185908350045)) ;
#34377=CARTESIAN_POINT('Ctrl Pts',(22.0088981253569,-2.31045361039959,-12.5200278078485)) ;
#34378=CARTESIAN_POINT('Ctrl Pts',(22.0021523404249,-2.37299967366979,-12.5214647806926)) ;
#34379=CARTESIAN_POINT('Ctrl Pts',(21.9531679373253,-2.82717685340531,-12.5318993346765)) ;
#34380=CARTESIAN_POINT('Ctrl Pts',(21.890109436478,-3.27989555583653,-12.5423338886604)) ;
#34381=CARTESIAN_POINT('Ctrl Pts',(21.8130902341816,-3.73027204074327,-12.5527684426443)) ;
#34382=CARTESIAN_POINT('Ctrl Pts',(21.7380893251005,-4.1688463805134,-12.5629295584611)) ;
#34383=CARTESIAN_POINT('Ctrl Pts',(21.6498500776779,-4.60519944952066,-12.5730906742779)) ;
#34384=CARTESIAN_POINT('Ctrl Pts',(21.5485294090372,-5.03852313385167,-12.5832517900946)) ;
#34385=CARTESIAN_POINT('Ctrl Pts',(21.4472191587707,-5.47180226134795,-12.593411861087)) ;
#34386=CARTESIAN_POINT('Ctrl Pts',(21.332830226361,-5.9020524029421,-12.6035719320794)) ;
#34387=CARTESIAN_POINT('Ctrl Pts',(21.2055703646003,-6.32847695535699,-12.6137320030718)) ;
#34388=CARTESIAN_POINT('Ctrl Pts',(21.078318095163,-6.75487606728283,-12.6238914679143)) ;
#34389=CARTESIAN_POINT('Ctrl Pts',(20.9381964961067,-7.17744982610941,-12.6340509327568)) ;
#34390=CARTESIAN_POINT('Ctrl Pts',(20.7854633163735,-7.59541636687505,-12.6442103975994)) ;
#34391=CARTESIAN_POINT('Ctrl Pts',(20.6255013617559,-8.03316502726702,-12.6548507041583)) ;
#34392=CARTESIAN_POINT('Ctrl Pts',(20.4517054368565,-8.46585962278698,-12.6654910107172)) ;
#34393=CARTESIAN_POINT('Ctrl Pts',(20.2644292103402,-8.89262300120791,-12.6761313172761)) ;
#34394=CARTESIAN_POINT('Ctrl Pts',(20.0855987762474,-9.30014018391493,-12.6862917667694)) ;
#34395=CARTESIAN_POINT('Ctrl Pts',(19.8944769789702,-9.70224900488492,-12.6964522162627)) ;
#34396=CARTESIAN_POINT('Ctrl Pts',(19.6914205353077,-10.0982073836975,-12.706612665756)) ;
#34397=CARTESIAN_POINT('Ctrl Pts',(19.4883549999242,-10.4941834912906,-12.7167735701768)) ;
#34398=CARTESIAN_POINT('Ctrl Pts',(19.2733538573369,-10.8840084033699,-12.7269344745977)) ;
#34399=CARTESIAN_POINT('Ctrl Pts',(19.0468199891755,-11.2669642478551,-12.7370953790185)) ;
#34400=CARTESIAN_POINT('Ctrl Pts',(18.8202484765266,-11.6499837304029,-12.7472579719376)) ;
#34401=CARTESIAN_POINT('Ctrl Pts',(18.5821405258547,-12.0261316670165,-12.7574205648567)) ;
#34402=CARTESIAN_POINT('Ctrl Pts',(18.3329436359918,-12.3947171287629,-12.7675831577758)) ;
#34403=CARTESIAN_POINT('Ctrl Pts',(18.2977076321218,-12.4468344676417,-12.7690201306194)) ;
#34404=CARTESIAN_POINT('Ctrl Pts',(18.2622499926592,-12.4988006538132,-12.7704571034629)) ;
#34405=CARTESIAN_POINT('Ctrl Pts',(18.2265720521004,-12.5506137814887,-12.7718940763064)) ;
#34406=CARTESIAN_POINT('Ctrl Pts',(17.9674972905483,-12.9268539312153,-12.7823286302903)) ;
#34407=CARTESIAN_POINT('Ctrl Pts',(17.6967352785155,-13.2951181446547,-12.7927631842742)) ;
#34408=CARTESIAN_POINT('Ctrl Pts',(17.4148060316788,-13.6546829308302,-12.8031977382582)) ;
#34409=CARTESIAN_POINT('Ctrl Pts',(17.1402647591279,-14.0048252983522,-12.8133588540749)) ;
#34410=CARTESIAN_POINT('Ctrl Pts',(16.8551341904644,-14.3467181535442,-12.8235199698917)) ;
#34411=CARTESIAN_POINT('Ctrl Pts',(16.5599366621038,-14.6797252293635,-12.8336810857085)) ;
#34412=CARTESIAN_POINT('Ctrl Pts',(16.2647694876492,-15.0126980634819,-12.8438411567009)) ;
#34413=CARTESIAN_POINT('Ctrl Pts',(15.9595375733945,-15.3367867715904,-12.8540012276934)) ;
#34414=CARTESIAN_POINT('Ctrl Pts',(15.6448025014556,-15.651389387302,-12.8641612986859)) ;
#34415=CARTESIAN_POINT('Ctrl Pts',(15.3300862066105,-15.965973233822,-12.8743207635285)) ;
#34416=CARTESIAN_POINT('Ctrl Pts',(15.0058680490801,-16.2710719563738,-12.8844802283712)) ;
#34417=CARTESIAN_POINT('Ctrl Pts',(14.6727465832436,-16.5661203293472,-12.8946396932138)) ;
#34418=CARTESIAN_POINT('Ctrl Pts',(14.323858667124,-16.875133174685,-12.9052799997727)) ;
#34419=CARTESIAN_POINT('Ctrl Pts',(13.9652046178105,-17.1731212774895,-12.9159203063315)) ;
#34420=CARTESIAN_POINT('Ctrl Pts',(13.597512683015,-17.4594812035681,-12.9265606128904)) ;
#34421=CARTESIAN_POINT('Ctrl Pts',(13.2464029370764,-17.7329268556963,-12.9367210623838)) ;
#34422=CARTESIAN_POINT('Ctrl Pts',(12.887052558089,-17.9957696802504,-12.9468815118771)) ;
#34423=CARTESIAN_POINT('Ctrl Pts',(12.5201282418468,-18.2475265137555,-12.9570419613704)) ;
#34424=CARTESIAN_POINT('Ctrl Pts',(12.1531874968068,-18.4992946195093,-12.9672028657913)) ;
#34425=CARTESIAN_POINT('Ctrl Pts',(11.7786723275488,-18.7399756145782,-12.9773637702121)) ;
#34426=CARTESIAN_POINT('Ctrl Pts',(11.3972785282958,-18.9691295849585,-12.987524674633)) ;
#34427=CARTESIAN_POINT('Ctrl Pts',(11.0158213505471,-19.1983216352288,-12.9976872675523)) ;
#34428=CARTESIAN_POINT('Ctrl Pts',(10.6274834555761,-19.4159827151883,-13.0078498604716)) ;
#34429=CARTESIAN_POINT('Ctrl Pts',(10.2329870740668,-19.6217178301106,-13.0180124533909)) ;
#34430=CARTESIAN_POINT('Ctrl Pts',(10.1772059765213,-19.6508084150993,-13.019449426234)) ;
#34431=CARTESIAN_POINT('Ctrl Pts',(10.1213017891803,-19.6796606340271,-13.0208863990771)) ;
#34432=CARTESIAN_POINT('Ctrl Pts',(10.0652765922826,-19.7082734450116,-13.0223233719203)) ;
#34433=CARTESIAN_POINT('Ctrl Pts',(9.66981891971409,-19.910238922406,-13.0324663427184)) ;
#34434=CARTESIAN_POINT('Ctrl Pts',(9.26822673759724,-20.100325336545,-13.0426093135165)) ;
#34435=CARTESIAN_POINT('Ctrl Pts',(8.86123712984376,-20.2781732804308,-13.0527522843147)) ;
#34436=CARTESIAN_POINT('Ctrl Pts',(8.45430968843143,-20.4559940586207,-13.0628937058069)) ;
#34437=CARTESIAN_POINT('Ctrl Pts',(8.04198667986045,-20.6215800075577,-13.0730351272992)) ;
#34438=CARTESIAN_POINT('Ctrl Pts',(7.62502660957808,-20.7746192327495,-13.0831765487915)) ;
#34439=CARTESIAN_POINT('Ctrl Pts',(7.20811061852015,-20.927642279293,-13.0933168981763)) ;
#34440=CARTESIAN_POINT('Ctrl Pts',(6.786558762008,-21.0681211717514,-13.1034572475611)) ;
#34441=CARTESIAN_POINT('Ctrl Pts',(6.36114786884429,-21.1957928102064,-13.1135975969459)) ;
#34442=CARTESIAN_POINT('Ctrl Pts',(5.93576194770578,-21.3234569542144,-13.1237373510826)) ;
#34443=CARTESIAN_POINT('Ctrl Pts',(5.50651766400403,-21.4383152797041,-13.1338771052192)) ;
#34444=CARTESIAN_POINT('Ctrl Pts',(5.07420699489083,-21.5401545592296,-13.1440168593559)) ;
#34445=CARTESIAN_POINT('Ctrl Pts',(4.64185758808263,-21.642002964181,-13.1541575220769)) ;
#34446=CARTESIAN_POINT('Ctrl Pts',(4.20644147134835,-21.7308299361701,-13.1642981847978)) ;
#34447=CARTESIAN_POINT('Ctrl Pts',(3.7687627767461,-21.8064729425717,-13.1744388475188)) ;
#34448=CARTESIAN_POINT('Ctrl Pts',(3.33107979540985,-21.8821166898398,-13.18457960956)) ;
#34449=CARTESIAN_POINT('Ctrl Pts',(2.89113442025274,-21.9445761760917,-13.1947203716011)) ;
#34450=CARTESIAN_POINT('Ctrl Pts',(2.44973934653467,-21.9937402957419,-13.2048611336423)) ;
#34451=CARTESIAN_POINT('Ctrl Pts',(2.0082552664889,-22.0429143292266,-13.2150039405454)) ;
#34452=CARTESIAN_POINT('Ctrl Pts',(1.56532113348893,-22.0787876108243,-13.2251467474485)) ;
#34453=CARTESIAN_POINT('Ctrl Pts',(1.12175523603032,-22.1013008724133,-13.2352895543516)) ;
#34454=CARTESIAN_POINT('Ctrl Pts',(0.748063471728612,-22.1202676606439,
-13.2438345832375)) ;
#34455=CARTESIAN_POINT('Ctrl Pts',(0.373923466354012,-22.1297529490399,
-13.2523796121235)) ;
#34456=CARTESIAN_POINT('Ctrl Pts',(-0.000174491033434178,-22.1297499993121,
-13.2609246410094)) ;
#34457=CARTESIAN_POINT('Origin',(0.,0.,-10.)) ;
#34458=CARTESIAN_POINT('',(-0.000385679535181172,-22.1297499966392,-16.9015753636525)) ;
#34459=CARTESIAN_POINT('',(-0.000394050632519626,-22.1297499964917,-16.4359246717926)) ;
#34460=CARTESIAN_POINT('',(-2.71011275034311E-15,-22.12975,-10.)) ;
#34461=CARTESIAN_POINT('Ctrl Pts',(-0.000398697885898679,-22.1294066254737,
-16.900980646995)) ;
#34462=CARTESIAN_POINT('Ctrl Pts',(0.445515082507069,-22.129342469394,-16.8906755313063)) ;
#34463=CARTESIAN_POINT('Ctrl Pts',(0.891431958115295,-22.1158270854489,
-16.8804240694696)) ;
#34464=CARTESIAN_POINT('Ctrl Pts',(1.33653233619602,-22.0888918978169,-16.870238980174)) ;
#34465=CARTESIAN_POINT('Ctrl Pts',(1.79786390062111,-22.0609744821951,-16.8596824778435)) ;
#34466=CARTESIAN_POINT('Ctrl Pts',(2.25831851995547,-22.0186423035969,-16.8491963171386)) ;
#34467=CARTESIAN_POINT('Ctrl Pts',(2.71698571375422,-21.9619713359938,-16.8387691144879)) ;
#34468=CARTESIAN_POINT('Ctrl Pts',(3.15957854718771,-21.9072864479878,-16.8287073415328)) ;
#34469=CARTESIAN_POINT('Ctrl Pts',(3.60050714112743,-21.8392512117159,-16.8186997539423)) ;
#34470=CARTESIAN_POINT('Ctrl Pts',(4.03895502150918,-21.7579752470251,-16.808711591363)) ;
#34471=CARTESIAN_POINT('Ctrl Pts',(4.47742742234612,-21.6766947369282,-16.7987228701899)) ;
#34472=CARTESIAN_POINT('Ctrl Pts',(4.91341883197495,-21.5821718771262,-16.788753457181)) ;
#34473=CARTESIAN_POINT('Ctrl Pts',(5.34611384725787,-21.4745565329947,-16.7787470699779)) ;
#34474=CARTESIAN_POINT('Ctrl Pts',(5.77888324139644,-21.3669226901381,-16.7687389627095)) ;
#34475=CARTESIAN_POINT('Ctrl Pts',(6.20835506704735,-21.2461916635369,-16.7586936895793)) ;
#34476=CARTESIAN_POINT('Ctrl Pts',(6.63371499978502,-21.112556176669,-16.7485356440111)) ;
#34477=CARTESIAN_POINT('Ctrl Pts',(6.67992922727902,-21.0980370357813,-16.7474319993265)) ;
#34478=CARTESIAN_POINT('Ctrl Pts',(6.72609491888823,-21.0833656108719,-16.7463270063693)) ;
#34479=CARTESIAN_POINT('Ctrl Pts',(6.77221103175265,-21.0685421811914,-16.7452205560158)) ;
#34480=CARTESIAN_POINT('Ctrl Pts',(7.20711644354217,-20.928747445926,-16.7347859981845)) ;
#34481=CARTESIAN_POINT('Ctrl Pts',(7.6377212435629,-20.7753936054156,-16.7242215297243)) ;
#34482=CARTESIAN_POINT('Ctrl Pts',(8.06319260124452,-20.6088199087664,-16.7136124369833)) ;
#34483=CARTESIAN_POINT('Ctrl Pts',(8.4775141851523,-20.4466113920542,-16.7032813629195)) ;
#34484=CARTESIAN_POINT('Ctrl Pts',(8.88696805208349,-20.2718671255665,-16.6929080437768)) ;
#34485=CARTESIAN_POINT('Ctrl Pts',(9.29080806907081,-20.0849356837908,-16.6825508059184)) ;
#34486=CARTESIAN_POINT('Ctrl Pts',(9.69460655854542,-19.8980234644733,-16.6721946331112)) ;
#34487=CARTESIAN_POINT('Ctrl Pts',(10.0927924334806,-19.6989266563173,-16.6618546330045)) ;
#34488=CARTESIAN_POINT('Ctrl Pts',(10.4846410750577,-19.4880268263416,-16.651567069552)) ;
#34489=CARTESIAN_POINT('Ctrl Pts',(10.8764663371707,-19.2771395796047,-16.641280119902)) ;
#34490=CARTESIAN_POINT('Ctrl Pts',(11.2619552371151,-19.054450703537,-16.6310456413425)) ;
#34491=CARTESIAN_POINT('Ctrl Pts',(11.6404015585227,-18.8203712583942,-16.6208788072008)) ;
#34492=CARTESIAN_POINT('Ctrl Pts',(12.0367599774297,-18.5752126889297,-16.6102307705368)) ;
#34493=CARTESIAN_POINT('Ctrl Pts',(12.4254010070655,-18.3175714676348,-16.5996488710798)) ;
#34494=CARTESIAN_POINT('Ctrl Pts',(12.8055292672146,-18.0479464061951,-16.5891310273476)) ;
#34495=CARTESIAN_POINT('Ctrl Pts',(13.1685140729281,-17.7904812008885,-16.5790875292342)) ;
#34496=CARTESIAN_POINT('Ctrl Pts',(13.5237401762096,-17.5220942682271,-16.5690985128436)) ;
#34497=CARTESIAN_POINT('Ctrl Pts',(13.8705432665648,-17.2432669395589,-16.5591300729815)) ;
#34498=CARTESIAN_POINT('Ctrl Pts',(14.2173618847343,-16.9644271266335,-16.549161186791)) ;
#34499=CARTESIAN_POINT('Ctrl Pts',(14.5557566675438,-16.675145864195,-16.539212762678)) ;
#34500=CARTESIAN_POINT('Ctrl Pts',(14.8850834384798,-16.3759393909295,-16.5292295000744)) ;
#34501=CARTESIAN_POINT('Ctrl Pts',(15.2144649363044,-16.0766831961085,-16.5192445784714)) ;
#34502=CARTESIAN_POINT('Ctrl Pts',(15.5347752782515,-15.7674983418902,-16.5092246313089)) ;
#34503=CARTESIAN_POINT('Ctrl Pts',(15.8453916701938,-15.4489382005339,-16.4990951144533)) ;
#34504=CARTESIAN_POINT('Ctrl Pts',(15.8893133897355,-15.4038932204594,-16.4976627824516)) ;
#34505=CARTESIAN_POINT('Ctrl Pts',(15.9330413214005,-15.3586608489135,-16.496228231026)) ;
#34506=CARTESIAN_POINT('Ctrl Pts',(15.9765737421392,-15.3132427127179,-16.4947912219427)) ;
#34507=CARTESIAN_POINT('Ctrl Pts',(16.2926759308042,-14.9834477687908,-16.4843566605601)) ;
#34508=CARTESIAN_POINT('Ctrl Pts',(16.5985468894886,-14.6437701875884,-16.4737921907038)) ;
#34509=CARTESIAN_POINT('Ctrl Pts',(16.8936153172396,-14.2949044544625,-16.4631830980188)) ;
#34510=CARTESIAN_POINT('Ctrl Pts',(17.1809515893413,-13.955180614862,-16.4528520125627)) ;
#34511=CARTESIAN_POINT('Ctrl Pts',(17.4580443900343,-13.606744039089,-16.4424786833142)) ;
#34512=CARTESIAN_POINT('Ctrl Pts',(17.7244031181186,-13.250256189044,-16.4321214362433)) ;
#34513=CARTESIAN_POINT('Ctrl Pts',(17.9907344586636,-12.8938049937956,-16.4217652541253)) ;
#34514=CARTESIAN_POINT('Ctrl Pts',(18.2463340431563,-12.5293042118981,-16.4114252456008)) ;
#34515=CARTESIAN_POINT('Ctrl Pts',(18.4907458857281,-12.1574340973639,-16.4011376742207)) ;
#34516=CARTESIAN_POINT('Ctrl Pts',(18.7351431473738,-11.7855861675594,-16.3908507165682)) ;
#34517=CARTESIAN_POINT('Ctrl Pts',(18.9683540956518,-11.4063697154289,-16.3806162304964)) ;
#34518=CARTESIAN_POINT('Ctrl Pts',(19.1899529460168,-11.0204821823412,-16.3704493970263)) ;
#34519=CARTESIAN_POINT('Ctrl Pts',(19.4220397597607,-10.6163311325035,-16.3598013815604)) ;
#34520=CARTESIAN_POINT('Ctrl Pts',(19.6414016093852,-10.2048692691444,-16.3492194780429)) ;
#34521=CARTESIAN_POINT('Ctrl Pts',(19.8475759560782,-9.78691359598903,-16.3387016462685)) ;
#34522=CARTESIAN_POINT('Ctrl Pts',(20.0444523991574,-9.38780658963541,-16.3286581401685)) ;
#34523=CARTESIAN_POINT('Ctrl Pts',(20.229309747748,-8.98278149620444,-16.318669115497)) ;
#34524=CARTESIAN_POINT('Ctrl Pts',(20.4017925113281,-8.5725776517286,-16.3087006667177)) ;
#34525=CARTESIAN_POINT('Ctrl Pts',(20.5742829976723,-8.16235544073625,-16.2987317716098)) ;
#34526=CARTESIAN_POINT('Ctrl Pts',(20.7343976745234,-7.74695394304696,-16.2887833379422)) ;
#34527=CARTESIAN_POINT('Ctrl Pts',(20.8818153631735,-7.32713362764678,-16.2788000648346)) ;
#34528=CARTESIAN_POINT('Ctrl Pts',(21.0292575488269,-6.90724354897934,-16.2688151327655)) ;
#34529=CARTESIAN_POINT('Ctrl Pts',(21.1639983406575,-6.48293311409231,-16.2587951741862)) ;
#34530=CARTESIAN_POINT('Ctrl Pts',(21.2857530286841,-6.05498528965268,-16.2486656447027)) ;
#34531=CARTESIAN_POINT('Ctrl Pts',(21.3029686234128,-5.99447528851859,-16.2472333723425)) ;
#34532=CARTESIAN_POINT('Ctrl Pts',(21.3199246528324,-5.93389260301837,-16.2457988807246)) ;
#34533=CARTESIAN_POINT('Ctrl Pts',(21.3366203749226,-5.87323948335914,-16.2443619316455)) ;
#34534=CARTESIAN_POINT('Ctrl Pts',(21.4578581694875,-5.43280028455092,-16.2339273702463)) ;
#34535=CARTESIAN_POINT('Ctrl Pts',(21.5653959819834,-4.98853289155693,-16.223362899899)) ;
#34536=CARTESIAN_POINT('Ctrl Pts',(21.6590615068585,-4.5413199178888,-16.2127538065303)) ;
#34537=CARTESIAN_POINT('Ctrl Pts',(21.7502724984438,-4.10582629488816,-16.2024227276486)) ;
#34538=CARTESIAN_POINT('Ctrl Pts',(21.8283291030326,-3.66753945279771,-16.1920494048484)) ;
#34539=CARTESIAN_POINT('Ctrl Pts',(21.8931143018501,-3.22727457632972,-16.181692164185)) ;
#34540=CARTESIAN_POINT('Ctrl Pts',(21.9578928389617,-2.78705497123813,-16.1713359885318)) ;
#34541=CARTESIAN_POINT('Ctrl Pts',(22.009402810843,-2.344857714738,-16.1609959864312)) ;
#34542=CARTESIAN_POINT('Ctrl Pts',(22.0475665860202,-1.90149806147783,-16.15070842152)) ;
#34543=CARTESIAN_POINT('Ctrl Pts',(22.0857280842954,-1.45816485964926,-16.1404214703788)) ;
#34544=CARTESIAN_POINT('Ctrl Pts',(22.110545028001,-1.01366929450376,-16.130186990863)) ;
#34545=CARTESIAN_POINT('Ctrl Pts',(22.1219745248157,-0.568827378077672,
-16.1200201652694)) ;
#34546=CARTESIAN_POINT('Ctrl Pts',(22.1339449782719,-0.102931149895318,
-16.1093721451036)) ;
#34547=CARTESIAN_POINT('Ctrl Pts',(22.1312447587415,0.363344973380265,-16.098790233538)) ;
#34548=CARTESIAN_POINT('Ctrl Pts',(22.1138554908743,0.829062320497137,-16.0882723965198)) ;
#34549=CARTESIAN_POINT('Ctrl Pts',(22.0972504520552,1.27377653656697,-16.0782288976609)) ;
#34550=CARTESIAN_POINT('Ctrl Pts',(22.0672580237881,1.71798115666027,-16.0682398804317)) ;
#34551=CARTESIAN_POINT('Ctrl Pts',(22.0239170757187,2.16085674282196,-16.0582714393598)) ;
#34552=CARTESIAN_POINT('Ctrl Pts',(21.9805741870779,2.6037521585392,-16.0483025519555)) ;
#34553=CARTESIAN_POINT('Ctrl Pts',(21.9238814467325,3.04531842922831,-16.0383541262568)) ;
#34554=CARTESIAN_POINT('Ctrl Pts',(21.8539179578104,3.48473384348501,-16.0283708614441)) ;
#34555=CARTESIAN_POINT('Ctrl Pts',(21.7839428425521,3.92422227856224,-16.0183859376406)) ;
#34556=CARTESIAN_POINT('Ctrl Pts',(21.7006923714283,4.36155911551283,-16.0083659876531)) ;
#34557=CARTESIAN_POINT('Ctrl Pts',(21.6042884274474,4.7959201946728,-15.998236467137)) ;
#34558=CARTESIAN_POINT('Ctrl Pts',(21.5906569511857,4.85733866465523,-15.9968041572879)) ;
#34559=CARTESIAN_POINT('Ctrl Pts',(21.5767625593062,4.91869763501853,-15.9953696280684)) ;
#34560=CARTESIAN_POINT('Ctrl Pts',(21.5626056691803,4.97999477322625,-15.9939326412558)) ;
#34561=CARTESIAN_POINT('Ctrl Pts',(21.4598065866317,5.42509885432025,-15.9834980807941)) ;
#34562=CARTESIAN_POINT('Ctrl Pts',(21.3431352851995,5.86705553464502,-15.9729336112498)) ;
#34563=CARTESIAN_POINT('Ctrl Pts',(21.2128599161341,6.30500644933931,-15.9623245184797)) ;
#34564=CARTESIAN_POINT('Ctrl Pts',(21.0859984091412,6.73148087367288,-15.951993436662)) ;
#34565=CARTESIAN_POINT('Ctrl Pts',(20.9462368104512,7.15415689631851,-15.9416201107047)) ;
#34566=CARTESIAN_POINT('Ctrl Pts',(20.7938598409848,7.57226175957971,-15.9312628666886)) ;
#34567=CARTESIAN_POINT('Ctrl Pts',(20.6414985396916,7.9903236311775,-15.920906687657)) ;
#34568=CARTESIAN_POINT('Ctrl Pts',(20.4765245484738,8.40381535729372,-15.9105666819826)) ;
#34569=CARTESIAN_POINT('Ctrl Pts',(20.2992572700811,8.81198284934143,-15.9002791133298)) ;
#34570=CARTESIAN_POINT('Ctrl Pts',(20.1220005673712,9.22012599030738,-15.8899921584286)) ;
#34571=CARTESIAN_POINT('Ctrl Pts',(19.9324520379643,9.622945648585,-15.8797576749853)) ;
#34572=CARTESIAN_POINT('Ctrl Pts',(19.7309620091718,10.0197035923024,-15.8695908421538)) ;
#34573=CARTESIAN_POINT('Ctrl Pts',(19.5199356073603,10.4352397940418,-15.8589428206953)) ;
#34574=CARTESIAN_POINT('Ctrl Pts',(19.2958229094729,10.8441335486082,-15.848360917402)) ;
#34575=CARTESIAN_POINT('Ctrl Pts',(19.0590541601682,11.2455503929158,-15.8378430819796)) ;
#34576=CARTESIAN_POINT('Ctrl Pts',(18.8329631809739,11.6288641860625,-15.8277995787021)) ;
#34577=CARTESIAN_POINT('Ctrl Pts',(18.5953377935072,12.0053633218949,-15.8178105569502)) ;
#34578=CARTESIAN_POINT('Ctrl Pts',(18.3466018745999,12.3743454338818,-15.8078421112832)) ;
#34579=CARTESIAN_POINT('Ctrl Pts',(18.0978548187502,12.7433440667337,-15.7978732192874)) ;
#34580=CARTESIAN_POINT('Ctrl Pts',(17.8379961126401,13.1048249446298,-15.7879247889248)) ;
#34581=CARTESIAN_POINT('Ctrl Pts',(17.5674861071872,13.4581028341233,-15.7779415194025)) ;
#34582=CARTESIAN_POINT('Ctrl Pts',(17.2969311496136,13.8114394297275,-15.767956590906)) ;
#34583=CARTESIAN_POINT('Ctrl Pts',(17.0157211924628,14.1565701935021,-15.75793663618)) ;
#34584=CARTESIAN_POINT('Ctrl Pts',(16.7243553839128,14.4928280822395,-15.7478071109031)) ;
#34585=CARTESIAN_POINT('Ctrl Pts',(16.6831569244332,14.5403741792672,-15.7463748191776)) ;
#34586=CARTESIAN_POINT('Ctrl Pts',(16.6417554811955,14.5877429102753,-15.7449403081396)) ;
#34587=CARTESIAN_POINT('Ctrl Pts',(16.6001525305366,14.6349324219095,-15.7435033395758)) ;
#34588=CARTESIAN_POINT('Ctrl Pts',(16.2980522969234,14.9775995227523,-15.7330687782776)) ;
#34589=CARTESIAN_POINT('Ctrl Pts',(15.9852455699344,15.3109009638877,-15.7225043081408)) ;
#34590=CARTESIAN_POINT('Ctrl Pts',(15.6623764342191,15.6342091702737,-15.7118952150116)) ;
#34591=CARTESIAN_POINT('Ctrl Pts',(15.3479681131464,15.9490450561309,-15.7015641341187)) ;
#34592=CARTESIAN_POINT('Ctrl Pts',(15.0240180537662,16.2544049007209,-15.6911908093172)) ;
#34593=CARTESIAN_POINT('Ctrl Pts',(14.6911442062324,16.5497443165883,-15.680833566643)) ;
#34594=CARTESIAN_POINT('Ctrl Pts',(14.3583045867446,16.8450533639207,-15.6704773889614)) ;
#34595=CARTESIAN_POINT('Ctrl Pts',(14.0165430552721,17.1303441493424,-15.6601373848229)) ;
#34596=CARTESIAN_POINT('Ctrl Pts',(13.6664991931125,17.4051052013234,-15.6498498178448)) ;
#34597=CARTESIAN_POINT('Ctrl Pts',(13.3164762145977,17.679849861038,-15.6395628646238)) ;
#34598=CARTESIAN_POINT('Ctrl Pts',(12.95817183278,17.9440661428831,-15.6293283829993)) ;
#34599=CARTESIAN_POINT('Ctrl Pts',(12.5922452900304,18.1972712266993,-15.6191615546121)) ;
#34600=CARTESIAN_POINT('Ctrl Pts',(12.2089996346471,18.4624603752217,-15.608513535534)) ;
#34601=CARTESIAN_POINT('Ctrl Pts',(11.8174009269038,18.7155830642744,-15.5979316269133)) ;
#34602=CARTESIAN_POINT('Ctrl Pts',(11.4182244644345,18.9561098095404,-15.5874137914221)) ;
#34603=CARTESIAN_POINT('Ctrl Pts',(11.0370500981217,19.1857892579249,-15.5773702902258)) ;
#34604=CARTESIAN_POINT('Ctrl Pts',(10.6489697482767,19.4039887484891,-15.5673812705962)) ;
#34605=CARTESIAN_POINT('Ctrl Pts',(10.2546903045263,19.6102919916142,-15.5574128270476)) ;
#34606=CARTESIAN_POINT('Ctrl Pts',(9.86039320715561,19.8166044718404,-15.5474439371681)) ;
#34607=CARTESIAN_POINT('Ctrl Pts',(9.45989637934238,20.0110195294185,-15.5374955089177)) ;
#34608=CARTESIAN_POINT('Ctrl Pts',(9.05393064893995,20.1931532917484,-15.527512241464)) ;
#34609=CARTESIAN_POINT('Ctrl Pts',(8.64789745668619,20.3753173203787,-15.5175273150286)) ;
#34610=CARTESIAN_POINT('Ctrl Pts',(8.23639345897018,20.5451957927667,-15.5075073623198)) ;
#34611=CARTESIAN_POINT('Ctrl Pts',(7.8201749628121,20.7024392880846,-15.4973778389826)) ;
#34612=CARTESIAN_POINT('Ctrl Pts',(7.76132233973509,20.7246732643415,-15.495945540744)) ;
#34613=CARTESIAN_POINT('Ctrl Pts',(7.70237549952867,20.7466546825148,-15.4945110231702)) ;
#34614=CARTESIAN_POINT('Ctrl Pts',(7.6433366223019,20.7683826142873,-15.4930740480446)) ;
#34615=CARTESIAN_POINT('Ctrl Pts',(7.21462721564321,20.9261594754961,-15.482639487253)) ;
#34616=CARTESIAN_POINT('Ctrl Pts',(6.7809532594462,21.0706060016275,-15.4720750174389)) ;
#34617=CARTESIAN_POINT('Ctrl Pts',(6.34317979086824,21.2014764159842,-15.4614659244762)) ;
#34618=CARTESIAN_POINT('Ctrl Pts',(5.91687820583473,21.328917362224,-15.4511348435168)) ;
#34619=CARTESIAN_POINT('Ctrl Pts',(5.4866891851808,21.4434847700754,-15.440761518499)) ;
#34620=CARTESIAN_POINT('Ctrl Pts',(5.05341521606951,21.5449936137857,-15.4304042754925)) ;
#34621=CARTESIAN_POINT('Ctrl Pts',(4.62018579870428,21.646492019767,-15.4200480974779)) ;
#34622=CARTESIAN_POINT('Ctrl Pts',(4.18387205289975,21.7349346599373,-15.4097080928905)) ;
#34623=CARTESIAN_POINT('Ctrl Pts',(3.74527984134167,21.8101757510026,-15.3994205253827)) ;
#34624=CARTESIAN_POINT('Ctrl Pts',(3.30671379622569,21.8854123531791,-15.3891335716319)) ;
#34625=CARTESIAN_POINT('Ctrl Pts',(2.86586945657449,21.9474490397433,-15.3788990893969)) ;
#34626=CARTESIAN_POINT('Ctrl Pts',(2.4235563556766,21.9961745840213,-15.3687322589047)) ;
#34627=CARTESIAN_POINT('Ctrl Pts',(1.96030882380211,22.0472062809803,-15.3580842380277)) ;
#34628=CARTESIAN_POINT('Ctrl Pts',(1.49545140178371,22.0836509495794,-15.3475023320353)) ;
#34629=CARTESIAN_POINT('Ctrl Pts',(1.02991790758809,22.1054115135611,-15.3369844961912)) ;
#34630=CARTESIAN_POINT('Ctrl Pts',(0.585379068081297,22.1261907184518,-15.3269409942765)) ;
#34631=CARTESIAN_POINT('Ctrl Pts',(0.140224399000022,22.1335869935488,-15.3169519739188)) ;
#34632=CARTESIAN_POINT('Ctrl Pts',(-0.304726290300343,22.1275702944762,
-15.3069835296644)) ;
#34633=CARTESIAN_POINT('Ctrl Pts',(-0.74969690195301,22.1215533260101,-15.2970146390799)) ;
#34634=CARTESIAN_POINT('Ctrl Pts',(-1.19446353490935,22.1021220468533,-15.2870662101471)) ;
#34635=CARTESIAN_POINT('Ctrl Pts',(-1.63820073751772,22.0692863133329,-15.2770829420619)) ;
#34636=CARTESIAN_POINT('Ctrl Pts',(-2.08201167859416,22.036445123302,-15.2670980149973)) ;
#34637=CARTESIAN_POINT('Ctrl Pts',(-2.52479283694592,21.9901948256536,-15.2570780617106)) ;
#34638=CARTESIAN_POINT('Ctrl Pts',(-2.9657127307059,21.93058770016,-15.2469485378707)) ;
#34639=CARTESIAN_POINT('Ctrl Pts',(-3.02805803913257,21.9221593559734,-15.2455162407643)) ;
#34640=CARTESIAN_POINT('Ctrl Pts',(-3.09036612552438,21.913464034756,-15.2440817243279)) ;
#34641=CARTESIAN_POINT('Ctrl Pts',(-3.15263463060782,21.9045019566268,-15.2426447503456)) ;
#34642=CARTESIAN_POINT('Ctrl Pts',(-3.60479627335464,21.8394239856061,-15.232210189317)) ;
#34643=CARTESIAN_POINT('Ctrl Pts',(-4.05498594158336,21.7602585768977,-15.2216457193675)) ;
#34644=CARTESIAN_POINT('Ctrl Pts',(-4.5023257926841,21.6672008914192,-15.2110366263487)) ;
#34645=CARTESIAN_POINT('Ctrl Pts',(-4.93794307784933,21.576581787818,-15.2007055452086)) ;
#34646=CARTESIAN_POINT('Ctrl Pts',(-5.37085809264521,21.472789306177,-15.1903322200844)) ;
#34647=CARTESIAN_POINT('Ctrl Pts',(-5.80027690904801,21.3560423037386,-15.1799749770272)) ;
#34648=CARTESIAN_POINT('Ctrl Pts',(-6.22965157017806,21.2393073058875,-15.1696187989604)) ;
#34649=CARTESIAN_POINT('Ctrl Pts',(-6.65553081823553,21.1096205437445,-15.1592787943764)) ;
#34650=CARTESIAN_POINT('Ctrl Pts',(-7.07713641751565,20.9672370009374,-15.1489912269084)) ;
#34651=CARTESIAN_POINT('Ctrl Pts',(-7.49871686383038,20.8248619527241,-15.1387042731961)) ;
#34652=CARTESIAN_POINT('Ctrl Pts',(-7.91602428757526,20.6697916422236,-15.128469791036)) ;
#34653=CARTESIAN_POINT('Ctrl Pts',(-8.32829365695817,20.5023131966915,-15.1183029612768)) ;
#34654=CARTESIAN_POINT('Ctrl Pts',(-8.76007549515082,20.3269080940089,-15.1076549413947)) ;
#34655=CARTESIAN_POINT('Ctrl Pts',(-9.18633668357024,20.1379053643401,-15.0970730344294)) ;
#34656=CARTESIAN_POINT('Ctrl Pts',(-9.60620958610337,19.9356636821395,-15.0865551989198)) ;
#34657=CARTESIAN_POINT('Ctrl Pts',(-10.0071470463981,19.7425427021048,-15.0765116971086)) ;
#34658=CARTESIAN_POINT('Ctrl Pts',(-10.4022619996847,19.5373560485768,-15.0665226768525)) ;
#34659=CARTESIAN_POINT('Ctrl Pts',(-10.7908189811037,19.3204671517673,-15.0565542326806)) ;
#34660=CARTESIAN_POINT('Ctrl Pts',(-11.1793933598962,19.1035685439055,-15.0465853421784)) ;
#34661=CARTESIAN_POINT('Ctrl Pts',(-11.561409132193,18.8749665165229,-15.0366369133088)) ;
#34662=CARTESIAN_POINT('Ctrl Pts',(-11.9361448444259,18.6350622832329,-15.0266536452525)) ;
#34663=CARTESIAN_POINT('Ctrl Pts',(-12.3109428287427,18.3951181836155,-15.0166687182166)) ;
#34664=CARTESIAN_POINT('Ctrl Pts',(-12.678458230161,18.1438679522468,-15.006648764924)) ;
#34665=CARTESIAN_POINT('Ctrl Pts',(-13.0379844648463,17.8817529898452,-14.9965192410308)) ;
#34666=CARTESIAN_POINT('Ctrl Pts',(-13.0888208267137,17.8446904063839,-14.9950869446015)) ;
#34667=CARTESIAN_POINT('Ctrl Pts',(-13.1394974841268,17.8074106672942,-14.9936524288434)) ;
#34668=CARTESIAN_POINT('Ctrl Pts',(-13.190012466339,17.7699150881616,-14.9922154555409)) ;
#34669=CARTESIAN_POINT('Ctrl Pts',(-13.556826282387,17.4976414801302,-14.9817808945932)) ;
#34670=CARTESIAN_POINT('Ctrl Pts',(-13.9152061005742,17.2139130798917,-14.9712164246814)) ;
#34671=CARTESIAN_POINT('Ctrl Pts',(-14.2644725010906,16.9193190259568,-14.9606073316696)) ;
#34672=CARTESIAN_POINT('Ctrl Pts',(-14.6045863502757,16.6324448305496,-14.9502762507089)) ;
#34673=CARTESIAN_POINT('Ctrl Pts',(-14.9360584492507,16.3352672232955,-14.9399029257363)) ;
#34674=CARTESIAN_POINT('Ctrl Pts',(-15.2582944657499,16.028356282535,-14.929545682811)) ;
#34675=CARTESIAN_POINT('Ctrl Pts',(-15.5804973480705,15.7214769001399,-14.9191895048776)) ;
#34676=CARTESIAN_POINT('Ctrl Pts',(-15.8934661496102,15.4048662356502,-14.9088495004071)) ;
#34677=CARTESIAN_POINT('Ctrl Pts',(-16.1966375223475,15.0791186849163,-14.8985619330411)) ;
#34678=CARTESIAN_POINT('Ctrl Pts',(-16.4997908078651,14.7533905682978,-14.8882749794318)) ;
#34679=CARTESIAN_POINT('Ctrl Pts',(-16.7931479375089,14.4185266033491,-14.878040497363)) ;
#34680=CARTESIAN_POINT('Ctrl Pts',(-17.0761724647569,14.0751431834048,-14.8678736674933)) ;
#34681=CARTESIAN_POINT('Ctrl Pts',(-17.3725923864151,13.7155076160272,-14.8572256471864)) ;
#34682=CARTESIAN_POINT('Ctrl Pts',(-17.6576895078092,13.3465357073017,-14.8466437404107)) ;
#34683=CARTESIAN_POINT('Ctrl Pts',(-17.9308711478129,12.9689555842401,-14.8361259046928)) ;
#34684=CARTESIAN_POINT('Ctrl Pts',(-18.191732825452,12.6084035927385,-14.8260824029755)) ;
#34685=CARTESIAN_POINT('Ctrl Pts',(-18.4417346834897,12.2400064517195,-14.8160933828175)) ;
#34686=CARTESIAN_POINT('Ctrl Pts',(-18.6804025706626,11.864433616645,-14.806124938755)) ;
#34687=CARTESIAN_POINT('Ctrl Pts',(-18.9190811440305,11.4888439655482,-14.796156048362)) ;
#34688=CARTESIAN_POINT('Ctrl Pts',(-19.1464246288981,11.1060778874681,-14.7862076196129)) ;
#34689=CARTESIAN_POINT('Ctrl Pts',(-19.3619891674588,10.7168314124428,-14.7762243516947)) ;
#34690=CARTESIAN_POINT('Ctrl Pts',(-19.5775895276811,10.3275202539795,-14.7662394247966)) ;
#34691=CARTESIAN_POINT('Ctrl Pts',(-19.781406855353,9.93172644478167,-14.7562194716594)) ;
#34692=CARTESIAN_POINT('Ctrl Pts',(-19.9730294843648,9.53017429574671,-14.7460899479446)) ;
#34693=CARTESIAN_POINT('Ctrl Pts',(-20.00012459641,9.47339550857423,-14.744657650614)) ;
#34694=CARTESIAN_POINT('Ctrl Pts',(-20.0269759496543,9.41650163921464,-14.7432231339523)) ;
#34695=CARTESIAN_POINT('Ctrl Pts',(-20.053582436078,9.35949478216512,-14.7417861597431)) ;
#34696=CARTESIAN_POINT('Ctrl Pts',(-20.2467849324901,8.9455405711805,-14.7313515987845)) ;
#34697=CARTESIAN_POINT('Ctrl Pts',(-20.427120813459,8.52552048915342,-14.7207871288741)) ;
#34698=CARTESIAN_POINT('Ctrl Pts',(-20.594272565392,8.10027589246691,-14.7101780358706)) ;
#34699=CARTESIAN_POINT('Ctrl Pts',(-20.7570440954759,7.68617485635989,-14.699846954796)) ;
#34700=CARTESIAN_POINT('Ctrl Pts',(-20.9073137907143,7.26711960221349,-14.6894736297151)) ;
#34701=CARTESIAN_POINT('Ctrl Pts',(-21.0448299240249,6.84389425607836,-14.6791163866848)) ;
#34702=CARTESIAN_POINT('Ctrl Pts',(-21.18233191714,6.42071242839394,-14.6687602086454)) ;
#34703=CARTESIAN_POINT('Ctrl Pts',(-21.3070830847419,5.99336136141939,-14.6584202040724)) ;
#34704=CARTESIAN_POINT('Ctrl Pts',(-21.4188705204252,5.56263183850919,-14.6481326366048)) ;
#34705=CARTESIAN_POINT('Ctrl Pts',(-21.5306512868717,5.13192801291597,-14.6378456828932)) ;
#34706=CARTESIAN_POINT('Ctrl Pts',(-21.6294699347588,4.69784603908703,-14.6276112007232)) ;
#34707=CARTESIAN_POINT('Ctrl Pts',(-21.7151476835065,4.26118325832356,-14.6174443707622)) ;
#34708=CARTESIAN_POINT('Ctrl Pts',(-21.8048805109009,3.80385347890562,-14.6067963505777)) ;
#34709=CARTESIAN_POINT('Ctrl Pts',(-21.8802129037667,3.34369517484707,-14.5962144438847)) ;
#34710=CARTESIAN_POINT('Ctrl Pts',(-21.9409697473836,2.88163072060197,-14.5856966082665)) ;
#34711=CARTESIAN_POINT('Ctrl Pts',(-21.9989865763307,2.44040446840396,-14.5756531064382)) ;
#34712=CARTESIAN_POINT('Ctrl Pts',(-22.0437193846154,1.99744130624142,-14.5656640861658)) ;
#34713=CARTESIAN_POINT('Ctrl Pts',(-22.0750694257953,1.5535556291076,-14.5556956419838)) ;
#34714=CARTESIAN_POINT('Ctrl Pts',(-22.1064208706525,1.10965007728892,-14.5457267514713)) ;
#34715=CARTESIAN_POINT('Ctrl Pts',(-22.12438821669,0.664821897241222,-14.5357783225975)) ;
#34716=CARTESIAN_POINT('Ctrl Pts',(-22.1289120038117,0.219894455284174,
-14.5257950545478)) ;
#34717=CARTESIAN_POINT('Ctrl Pts',(-22.1334365426781,-0.225106922927372,
-14.5158101275186)) ;
#34718=CARTESIAN_POINT('Ctrl Pts',(-22.1245128562186,-0.670207602470856,
-14.5057901742436)) ;
#34719=CARTESIAN_POINT('Ctrl Pts',(-22.1021232519658,-1.11457464741053,
-14.4956606503828)) ;
#34720=CARTESIAN_POINT('Ctrl Pts',(-22.0989574016564,-1.17740735900297,
-14.4942283536844)) ;
#34721=CARTESIAN_POINT('Ctrl Pts',(-22.0955223923823,-1.2402253877673,-14.4927938376568)) ;
#34722=CARTESIAN_POINT('Ctrl Pts',(-22.0918182454677,-1.30302636428287,
-14.491356864084)) ;
#34723=CARTESIAN_POINT('Ctrl Pts',(-22.064920640979,-1.75905466627196,-14.4809223031142)) ;
#34724=CARTESIAN_POINT('Ctrl Pts',(-22.0238197949282,-2.21430033586412,
-14.4703578331927)) ;
#34725=CARTESIAN_POINT('Ctrl Pts',(-21.9686365006969,-2.66787224769554,
-14.4597487401799)) ;
#34726=CARTESIAN_POINT('Ctrl Pts',(-21.9148992883904,-3.10955827717089,
-14.4494176591608)) ;
#34727=CARTESIAN_POINT('Ctrl Pts',(-21.8478083741637,-3.54965723659662,
-14.4390443341377)) ;
#34728=CARTESIAN_POINT('Ctrl Pts',(-21.7675152072097,-3.98735963025754,
-14.4286870911672)) ;
#34729=CARTESIAN_POINT('Ctrl Pts',(-21.6872302964613,-4.42501701683854,
-14.4183309131881)) ;
#34730=CARTESIAN_POINT('Ctrl Pts',(-21.5937459456807,-4.86027838884591,
-14.4079909086775)) ;
#34731=CARTESIAN_POINT('Ctrl Pts',(-21.4872509200593,-5.29234685536064,
-14.3977033412744)) ;
#34732=CARTESIAN_POINT('Ctrl Pts',(-21.3807622479327,-5.7243895446642,-14.3874163876277)) ;
#34733=CARTESIAN_POINT('Ctrl Pts',(-21.2612644665466,-6.15323982502812,
-14.3771819055247)) ;
#34734=CARTESIAN_POINT('Ctrl Pts',(-21.1289794797663,-6.5781112650732,-14.3670150756742)) ;
#34735=CARTESIAN_POINT('Ctrl Pts',(-20.9904335190314,-7.0230916311942,-14.3563670554903)) ;
#34736=CARTESIAN_POINT('Ctrl Pts',(-20.8378745514713,-7.46371210013524,
-14.345785148674)) ;
#34737=CARTESIAN_POINT('Ctrl Pts',(-20.6715871649445,-7.89907799341329,
-14.3352673130205)) ;
#34738=CARTESIAN_POINT('Ctrl Pts',(-20.5127990156401,-8.31480973295033,
-14.3252238112674)) ;
#34739=CARTESIAN_POINT('Ctrl Pts',(-20.3414990733482,-8.7257522039684,-14.3152347910721)) ;
#34740=CARTESIAN_POINT('Ctrl Pts',(-20.1579877570251,-9.13114203336038,
-14.3052663469689)) ;
#34741=CARTESIAN_POINT('Ctrl Pts',(-19.9744682241009,-9.5365500138209,-14.295297456535)) ;
#34742=CARTESIAN_POINT('Ctrl Pts',(-19.7787360917902,-9.93640481898993,
-14.2853490277415)) ;
#34743=CARTESIAN_POINT('Ctrl Pts',(-19.5711306051236,-10.3299538663865,
-14.2753657597736)) ;
#34744=CARTESIAN_POINT('Ctrl Pts',(-19.3634906194045,-10.7235683121954,
-14.265380832826)) ;
#34745=CARTESIAN_POINT('Ctrl Pts',(-19.1439731555917,-11.110874815802,-14.2553608796341)) ;
#34746=CARTESIAN_POINT('Ctrl Pts',(-18.9129587520637,-11.491132239014,-14.2452313558577)) ;
#34747=CARTESIAN_POINT('Ctrl Pts',(-18.8802937175048,-11.5448999767862,
-14.243799058827)) ;
#34748=CARTESIAN_POINT('Ctrl Pts',(-18.8473988890757,-11.5985267997651,
-14.2423645424659)) ;
#34749=CARTESIAN_POINT('Ctrl Pts',(-18.814275412313,-11.6520106337357,-14.2409275685585)) ;
#34750=CARTESIAN_POINT('Ctrl Pts',(-18.5737498637265,-12.0403825609475,
-14.2304930076016)) ;
#34751=CARTESIAN_POINT('Ctrl Pts',(-18.3211020605776,-12.4213116708992,
-14.2199285376896)) ;
#34752=CARTESIAN_POINT('Ctrl Pts',(-18.0568620376773,-12.7940714936667,
-14.2093194446831)) ;
#34753=CARTESIAN_POINT('Ctrl Pts',(-17.7995464416389,-13.1570631212096,
-14.1989883636437)) ;
#34754=CARTESIAN_POINT('Ctrl Pts',(-17.5312384715473,-13.5123082746593,
-14.1886150385969)) ;
#34755=CARTESIAN_POINT('Ctrl Pts',(-17.252456310858,-13.8591668711441,-14.1782577956)) ;
#34756=CARTESIAN_POINT('Ctrl Pts',(-16.9737028161546,-14.2059898016321,
-14.1679016175944)) ;
#34757=CARTESIAN_POINT('Ctrl Pts',(-16.6844773430316,-14.5444279976077,
-14.1575616130545)) ;
#34758=CARTESIAN_POINT('Ctrl Pts',(-16.3853249072146,-14.873870210102,-14.1472740456199)) ;
#34759=CARTESIAN_POINT('Ctrl Pts',(-16.0861903188295,-15.2032927680765,
-14.1369870919415)) ;
#34760=CARTESIAN_POINT('Ctrl Pts',(-15.77712990884,-15.5237205238918,-14.1267526098046)) ;
#34761=CARTESIAN_POINT('Ctrl Pts',(-15.4587128707131,-15.8345671888533,
-14.1165857798786)) ;
#34762=CARTESIAN_POINT('Ctrl Pts',(-15.1252253348865,-16.1601260500491,
-14.1059377596624)) ;
#34763=CARTESIAN_POINT('Ctrl Pts',(-14.781484058204,-16.4751856795172,-14.0953558529352)) ;
#34764=CARTESIAN_POINT('Ctrl Pts',(-14.4281648535965,-16.7790943743333,
-14.0848380172876)) ;
#34765=CARTESIAN_POINT('Ctrl Pts',(-14.090779655408,-17.0692973802685,-14.0747945154959)) ;
#34766=CARTESIAN_POINT('Ctrl Pts',(-13.7446655050044,-17.3493373427742,
-14.0648054952612)) ;
#34767=CARTESIAN_POINT('Ctrl Pts',(-13.3904496993175,-17.6186855950221,
-14.0548370511184)) ;
#34768=CARTESIAN_POINT('Ctrl Pts',(-13.0362180338587,-17.8880459071547,
-14.0448681606453)) ;
#34769=CARTESIAN_POINT('Ctrl Pts',(-12.67388388897,-18.1467134568534,-14.0349197318125)) ;
#34770=CARTESIAN_POINT('Ctrl Pts',(-12.3041035849764,-18.3941875334039,
-14.0249364638055)) ;
#34771=CARTESIAN_POINT('Ctrl Pts',(-11.9342618323657,-18.6417027342102,
-14.0149515368189)) ;
#34772=CARTESIAN_POINT('Ctrl Pts',(-11.5569713318479,-18.8780205792078,
-14.0049315835884)) ;
#34773=CARTESIAN_POINT('Ctrl Pts',(-11.1729192867255,-19.1026700621272,
-13.9948020597743)) ;
#34774=CARTESIAN_POINT('Ctrl Pts',(-11.1186150012861,-19.1344351049104,
-13.9933697628771)) ;
#34775=CARTESIAN_POINT('Ctrl Pts',(-11.0641755806956,-19.1659669081917,
-13.9919352466501)) ;
#34776=CARTESIAN_POINT('Ctrl Pts',(-11.0096030190606,-19.1972641920671,
-13.9904982728772)) ;
#34777=CARTESIAN_POINT('Ctrl Pts',(-10.613325277484,-19.4245288943289,-13.9800637119116)) ;
#34778=CARTESIAN_POINT('Ctrl Pts',(-10.2099231501165,-19.6394815004455,
-13.969499241994)) ;
#34779=CARTESIAN_POINT('Ctrl Pts',(-9.80020837513221,-19.8417350006139,
-13.9588901489843)) ;
#34780=CARTESIAN_POINT('Ctrl Pts',(-9.40123020254088,-20.0386884346229,
-13.9485590679486)) ;
#34781=CARTESIAN_POINT('Ctrl Pts',(-8.99626599144153,-20.2235999630236,
-13.938185742908)) ;
#34782=CARTESIAN_POINT('Ctrl Pts',(-8.58607597318324,-20.3961529338449,
-13.9278284999193)) ;
#34783=CARTESIAN_POINT('Ctrl Pts',(-8.17592813301714,-20.5686881617793,
-13.9174723219217)) ;
#34784=CARTESIAN_POINT('Ctrl Pts',(-7.76055556505427,-20.7288674873255,
-13.9071323173917)) ;
#34785=CARTESIAN_POINT('Ctrl Pts',(-7.34072839274776,-20.8764123834507,
-13.8968447499685)) ;
#34786=CARTESIAN_POINT('Ctrl Pts',(-6.92092626733406,-21.023948477046,-13.8865577963017)) ;
#34787=CARTESIAN_POINT('Ctrl Pts',(-6.49666997960255,-21.1588517230617,
-13.8763233141777)) ;
#34788=CARTESIAN_POINT('Ctrl Pts',(-6.06873905204388,-21.2808770494131,
-13.8661564842907)) ;
#34789=CARTESIAN_POINT('Ctrl Pts',(-5.62055439605247,-21.4086777653488,
-13.8555084641033)) ;
#34790=CARTESIAN_POINT('Ctrl Pts',(-5.16834254152024,-21.5223662618714,
-13.8449265573283)) ;
#34791=CARTESIAN_POINT('Ctrl Pts',(-4.71300791056191,-21.6216906253759,
-13.8344087216846)) ;
#34792=CARTESIAN_POINT('Ctrl Pts',(-4.2782079830875,-21.7165356538712,-13.8243652199078)) ;
#34793=CARTESIAN_POINT('Ctrl Pts',(-3.84056232262998,-21.7982893164388,
-13.8143761996884)) ;
#34794=CARTESIAN_POINT('Ctrl Pts',(-3.40087416261841,-21.866784861429,-13.8044077555605)) ;
#34795=CARTESIAN_POINT('Ctrl Pts',(-2.96116631586805,-21.9352834732607,
-13.7944388651022)) ;
#34796=CARTESIAN_POINT('Ctrl Pts',(-2.51941574493279,-21.9905226500052,
-13.7844904362839)) ;
#34797=CARTESIAN_POINT('Ctrl Pts',(-2.07643792028521,-22.0323740347578,
-13.7745071682909)) ;
#34798=CARTESIAN_POINT('Ctrl Pts',(-1.63338648334986,-22.0742323742065,
-13.7645222413182)) ;
#34799=CARTESIAN_POINT('Ctrl Pts',(-1.18910736175828,-22.1026982750266,
-13.7545022881008)) ;
#34800=CARTESIAN_POINT('Ctrl Pts',(-0.744429067465207,-22.11768419737,-13.7443727642986)) ;
#34801=CARTESIAN_POINT('Ctrl Pts',(-0.681552335208617,-22.1198031805515,
-13.7429404673681)) ;
#34802=CARTESIAN_POINT('Ctrl Pts',(-0.61866764297327,-22.1216527220511,
-13.7415059511075)) ;
#34803=CARTESIAN_POINT('Ctrl Pts',(-0.55577735361064,-22.1232326442476,
-13.7400689773009)) ;
#34804=CARTESIAN_POINT('Ctrl Pts',(-0.37061492733742,-22.1278842721889,
-13.7358382199103)) ;
#34805=CARTESIAN_POINT('Ctrl Pts',(-0.185394205576265,-22.1301988329937,
-13.7315860326588)) ;
#34806=CARTESIAN_POINT('Ctrl Pts',(-0.000170111177784315,-22.1301789835866,
-13.7273184261236)) ;
#34807=CARTESIAN_POINT('Ctrl Pts',(-0.000192018545400235,-22.1301832392792,
-13.2601742013415)) ;
#34808=CARTESIAN_POINT('Ctrl Pts',(-0.17280475386243,-22.1302004171725,
-13.2640845203255)) ;
#34809=CARTESIAN_POINT('Ctrl Pts',(-0.34541413006999,-22.1281900578278,
-13.2680085775377)) ;
#34810=CARTESIAN_POINT('Ctrl Pts',(-0.517975506591968,-22.1241500110886,
-13.2719512513423)) ;
#34811=CARTESIAN_POINT('Ctrl Pts',(-0.974671214221961,-22.1134577458689,
-13.2823858123052)) ;
#34812=CARTESIAN_POINT('Ctrl Pts',(-1.43108897853208,-22.0885434086334,
-13.2929502822213)) ;
#34813=CARTESIAN_POINT('Ctrl Pts',(-1.8863339478131,-22.0494960828901,-13.3035593752302)) ;
#34814=CARTESIAN_POINT('Ctrl Pts',(-2.3296491930147,-22.0114719948618,-13.3138904562656)) ;
#34815=CARTESIAN_POINT('Ctrl Pts',(-2.77185240675326,-21.9600462825204,
-13.3242637813067)) ;
#34816=CARTESIAN_POINT('Ctrl Pts',(-3.21212922727595,-21.8953415636052,
-13.3346210242967)) ;
#34817=CARTESIAN_POINT('Ctrl Pts',(-3.65236077600423,-21.8306434980013,
-13.3449772022954)) ;
#34818=CARTESIAN_POINT('Ctrl Pts',(-4.09066638251384,-21.7526692563123,
-13.3553172068271)) ;
#34819=CARTESIAN_POINT('Ctrl Pts',(-4.5262429572339,-21.6615791962104,-13.3656047742524)) ;
#34820=CARTESIAN_POINT('Ctrl Pts',(-4.96179354545244,-21.570494570542,-13.3758917279215)) ;
#34821=CARTESIAN_POINT('Ctrl Pts',(-5.39461557736581,-21.4662956991814,
-13.3861262100481)) ;
#34822=CARTESIAN_POINT('Ctrl Pts',(-5.82391466313536,-21.3491747257555,
-13.3962920035461)) ;
#34823=CARTESIAN_POINT('Ctrl Pts',(-6.27353223145597,-21.2265104830011,
-13.4069389382919)) ;
#34824=CARTESIAN_POINT('Ctrl Pts',(-6.71929162805928,-21.0896926339765,
-13.417522966905)) ;
#34825=CARTESIAN_POINT('Ctrl Pts',(-7.16028609751094,-20.9389649531089,
-13.4280408025512)) ;
#34826=CARTESIAN_POINT('Ctrl Pts',(-7.58139257681946,-20.795034796562,-13.4380843043312)) ;
#34827=CARTESIAN_POINT('Ctrl Pts',(-7.99815695782829,-20.6384307203011,
-13.4480733245541)) ;
#34828=CARTESIAN_POINT('Ctrl Pts',(-8.40980568409793,-20.4694258552265,
-13.4580417686853)) ;
#34829=CARTESIAN_POINT('Ctrl Pts',(-8.82147284165773,-20.3004134230746,
-13.4680106591467)) ;
#34830=CARTESIAN_POINT('Ctrl Pts',(-9.22802385464807,-20.1189989585829,
-13.4779590879682)) ;
#34831=CARTESIAN_POINT('Ctrl Pts',(-9.62869457218019,-19.9254947773076,
-13.4879423559642)) ;
#34832=CARTESIAN_POINT('Ctrl Pts',(-10.0294318715792,-19.7319584402767,
-13.4979272829399)) ;
#34833=CARTESIAN_POINT('Ctrl Pts',(-10.4242868388537,-19.5263281877794,
-13.5079472361601)) ;
#34834=CARTESIAN_POINT('Ctrl Pts',(-10.8125052943334,-19.3089580089504,
-13.5180767599648)) ;
#34835=CARTESIAN_POINT('Ctrl Pts',(-10.86739870413,-19.2782222463004,-13.519509056893)) ;
#34836=CARTESIAN_POINT('Ctrl Pts',(-10.922159445338,-19.2472518323632,-13.5209435731512)) ;
#34837=CARTESIAN_POINT('Ctrl Pts',(-10.9767854043858,-19.2160478383213,
-13.5223805469554)) ;
#34838=CARTESIAN_POINT('Ctrl Pts',(-11.3734508816389,-18.9894605636156,
-13.5328151079184)) ;
#34839=CARTESIAN_POINT('Ctrl Pts',(-11.7631085562476,-18.7504944647731,
-13.5433795778345)) ;
#34840=CARTESIAN_POINT('Ctrl Pts',(-12.1450136006463,-18.4996534538397,
-13.5539886708435)) ;
#34841=CARTESIAN_POINT('Ctrl Pts',(-12.5169107984637,-18.2553857479478,
-13.5643197518786)) ;
#34842=CARTESIAN_POINT('Ctrl Pts',(-12.881456618974,-17.9998576069013,-13.5746930769196)) ;
#34843=CARTESIAN_POINT('Ctrl Pts',(-13.2379929879246,-17.7335641654828,
-13.5850503199094)) ;
#34844=CARTESIAN_POINT('Ctrl Pts',(-13.5944926957544,-17.4672981058882,
-13.5954064979078)) ;
#34845=CARTESIAN_POINT('Ctrl Pts',(-13.942984694799,-17.1902690214,-13.6057465024393)) ;
#34846=CARTESIAN_POINT('Ctrl Pts',(-14.2828387740266,-16.9029998857225,
-13.6160340698645)) ;
#34847=CARTESIAN_POINT('Ctrl Pts',(-14.6226725775584,-16.6157478885228,
-13.6263210235333)) ;
#34848=CARTESIAN_POINT('Ctrl Pts',(-14.9538696274581,-16.3182569975224,
-13.6365555056598)) ;
#34849=CARTESIAN_POINT('Ctrl Pts',(-15.2758224815446,-16.0110740110271,
-13.6467212991572)) ;
#34850=CARTESIAN_POINT('Ctrl Pts',(-15.613013181862,-15.6893522277684,-13.657368233903)) ;
#34851=CARTESIAN_POINT('Ctrl Pts',(-15.9400791509408,-15.3570144246928,
-13.6679522625174)) ;
#34852=CARTESIAN_POINT('Ctrl Pts',(-16.2563386528229,-15.0147062545501,
-13.678470098164)) ;
#34853=CARTESIAN_POINT('Ctrl Pts',(-16.5583354682104,-14.6878355150181,
-13.6885135999438)) ;
#34854=CARTESIAN_POINT('Ctrl Pts',(-16.8504855116544,-14.3518805506525,
-13.6985026201664)) ;
#34855=CARTESIAN_POINT('Ctrl Pts',(-17.1322381813423,-14.0074494960581,
-13.7084710642973)) ;
#34856=CARTESIAN_POINT('Ctrl Pts',(-17.4140034663123,-13.6630030197999,
-13.7184399547584)) ;
#34857=CARTESIAN_POINT('Ctrl Pts',(-17.6853703552699,-13.3100795923354,
-13.7283883835796)) ;
#34858=CARTESIAN_POINT('Ctrl Pts',(-17.9458151546047,-12.9493173457743,
-13.7383716515752)) ;
#34859=CARTESIAN_POINT('Ctrl Pts',(-18.2063032336216,-12.5884951491763,
-13.7483565785506)) ;
#34860=CARTESIAN_POINT('Ctrl Pts',(-18.4558654347015,-12.2198314084818,
-13.7583765317704)) ;
#34861=CARTESIAN_POINT('Ctrl Pts',(-18.6940066536534,-11.8439961737811,
-13.7685060555746)) ;
#34862=CARTESIAN_POINT('Ctrl Pts',(-18.7276794050476,-11.7908537296509,
-13.7699383525045)) ;
#34863=CARTESIAN_POINT('Ctrl Pts',(-18.761123861049,-11.7375679558486,-13.7713728687645)) ;
#34864=CARTESIAN_POINT('Ctrl Pts',(-18.7943386717719,-11.6841407997898,
-13.7728098425704)) ;
#34865=CARTESIAN_POINT('Ctrl Pts',(-19.0355274574803,-11.2961804106372,
-13.7832444035333)) ;
#34866=CARTESIAN_POINT('Ctrl Pts',(-19.2646648130735,-10.9006630632944,
-13.7938088734492)) ;
#34867=CARTESIAN_POINT('Ctrl Pts',(-19.4813351570666,-10.4983862459944,
-13.804417966458)) ;
#34868=CARTESIAN_POINT('Ctrl Pts',(-19.6923276405839,-10.1066511188915,
-13.8147490474935)) ;
#34869=CARTESIAN_POINT('Ctrl Pts',(-19.8914983044428,-9.70850625480636,
-13.8251223725349)) ;
#34870=CARTESIAN_POINT('Ctrl Pts',(-20.0785037090679,-9.30470016521747,
-13.835479615525)) ;
#34871=CARTESIAN_POINT('Ctrl Pts',(-20.2654898847221,-8.90093559729271,
-13.8458357935238)) ;
#34872=CARTESIAN_POINT('Ctrl Pts',(-20.4403134163448,-8.49151097680173,
-13.8561757980556)) ;
#34873=CARTESIAN_POINT('Ctrl Pts',(-20.6026686141136,-8.07718605447576,
-13.8664633654812)) ;
#34874=CARTESIAN_POINT('Ctrl Pts',(-20.7650141257705,-7.66288585077699,
-13.8767503191504)) ;
#34875=CARTESIAN_POINT('Ctrl Pts',(-20.914892879849,-7.2436858088065,-13.8869848012772)) ;
#34876=CARTESIAN_POINT('Ctrl Pts',(-21.0520305458122,-6.82035580981904,
-13.8971505947757)) ;
#34877=CARTESIAN_POINT('Ctrl Pts',(-21.1956588598171,-6.37698984179532,
-13.9077975295215)) ;
#34878=CARTESIAN_POINT('Ctrl Pts',(-21.3253321166679,-5.92909988888031,
-13.918381558134)) ;
#34879=CARTESIAN_POINT('Ctrl Pts',(-21.4407576405948,-5.47757812386213,
-13.92889939378)) ;
#34880=CARTESIAN_POINT('Ctrl Pts',(-21.5509776986048,-5.04641910946049,
-13.9389428955603)) ;
#34881=CARTESIAN_POINT('Ctrl Pts',(-21.6482156614984,-4.61195142992625,
-13.9489319157834)) ;
#34882=CARTESIAN_POINT('Ctrl Pts',(-21.7322763690278,-4.1749718929724,-13.9589003599148)) ;
#34883=CARTESIAN_POINT('Ctrl Pts',(-21.8163408403181,-3.73797279055698,
-13.9688692503766)) ;
#34884=CARTESIAN_POINT('Ctrl Pts',(-21.8872267475388,-3.29846155946272,
-13.9788176791983)) ;
#34885=CARTESIAN_POINT('Ctrl Pts',(-21.9447768665892,-2.85724859969611,
-13.9888009471946)) ;
#34886=CARTESIAN_POINT('Ctrl Pts',(-22.0023365490894,-2.41596232091478,
-13.9987858741707)) ;
#34887=CARTESIAN_POINT('Ctrl Pts',(-22.0465558150088,-1.97297371783978,
-14.0088058273912)) ;
#34888=CARTESIAN_POINT('Ctrl Pts',(-22.0773177686225,-1.52910767268793,
-14.0189353511962)) ;
#34889=CARTESIAN_POINT('Ctrl Pts',(-22.0816674549924,-1.46634579121217,
-14.0203676481231)) ;
#34890=CARTESIAN_POINT('Ctrl Pts',(-22.0857481520724,-1.40356638996004,
-14.0218021643801)) ;
#34891=CARTESIAN_POINT('Ctrl Pts',(-22.0895595984754,-1.34077182398876,
-14.0232391381831)) ;
#34892=CARTESIAN_POINT('Ctrl Pts',(-22.1172363520578,-0.884790145393343,
-14.0336736991461)) ;
#34893=CARTESIAN_POINT('Ctrl Pts',(-22.1307178879002,-0.427891745342189,
-14.0442381690622)) ;
#34894=CARTESIAN_POINT('Ctrl Pts',(-22.1300178686683,0.0290242049999805,
-14.0548472620713)) ;
#34895=CARTESIAN_POINT('Ctrl Pts',(-22.129336193486,0.47396664305618,-14.0651783431059)) ;
#34896=CARTESIAN_POINT('Ctrl Pts',(-22.1152068468041,0.918925795854455,
-14.0755516681463)) ;
#34897=CARTESIAN_POINT('Ctrl Pts',(-22.0876836628607,1.36307988358833,-14.0859089111354)) ;
#34898=CARTESIAN_POINT('Ctrl Pts',(-22.0601633090093,1.80718830084565,-14.0962650891334)) ;
#34899=CARTESIAN_POINT('Ctrl Pts',(-22.0192519762506,2.25049186487643,-14.1066050936642)) ;
#34900=CARTESIAN_POINT('Ctrl Pts',(-21.9650420516846,2.69217686070395,-14.1168926610888)) ;
#34901=CARTESIAN_POINT('Ctrl Pts',(-21.910835361283,3.13383550560166,-14.127179614757)) ;
#34902=CARTESIAN_POINT('Ctrl Pts',(-21.8433316861536,3.57387592410145,-14.1374140968829)) ;
#34903=CARTESIAN_POINT('Ctrl Pts',(-21.7626558173783,4.01149040240759,-14.1475798903798)) ;
#34904=CARTESIAN_POINT('Ctrl Pts',(-21.6781616054206,4.46981692615091,-14.1582268251261)) ;
#34905=CARTESIAN_POINT('Ctrl Pts',(-21.5792399048857,4.92548682932996,-14.1688108537404)) ;
#34906=CARTESIAN_POINT('Ctrl Pts',(-21.4660575244286,5.3775760955686,-14.1793286893873)) ;
#34907=CARTESIAN_POINT('Ctrl Pts',(-21.3579794485149,5.80927701791184,-14.1893721911665)) ;
#34908=CARTESIAN_POINT('Ctrl Pts',(-21.236907732684,6.23771490789214,-14.1993612113885)) ;
#34909=CARTESIAN_POINT('Ctrl Pts',(-21.1030496181128,6.66209601419537,-14.2093296555187)) ;
#34910=CARTESIAN_POINT('Ctrl Pts',(-20.9691855101354,7.08649612187432,-14.2192985459793)) ;
#34911=CARTESIAN_POINT('Ctrl Pts',(-20.8225337231665,7.5068390621459,-14.2292469747998)) ;
#34912=CARTESIAN_POINT('Ctrl Pts',(-20.663341334201,7.92233716722134,-14.2392302427949)) ;
#34913=CARTESIAN_POINT('Ctrl Pts',(-20.5041224912775,8.33790431811922,-14.2492151697698)) ;
#34914=CARTESIAN_POINT('Ctrl Pts',(-20.332358691548,8.74862495674422,-14.259235122989)) ;
#34915=CARTESIAN_POINT('Ctrl Pts',(-20.1483393754432,9.15371785360323,-14.2693646467927)) ;
#34916=CARTESIAN_POINT('Ctrl Pts',(-20.1223193662966,9.21099728004941,-14.2707969437254)) ;
#34917=CARTESIAN_POINT('Ctrl Pts',(-20.0960543987149,9.26816420073129,-14.2722314599881)) ;
#34918=CARTESIAN_POINT('Ctrl Pts',(-20.0695453627053,9.32521641962857,-14.2736684337969)) ;
#34919=CARTESIAN_POINT('Ctrl Pts',(-19.8770504469171,9.73950014040196,-14.2841029947598)) ;
#34920=CARTESIAN_POINT('Ctrl Pts',(-19.6716322081881,10.1478397624984,-14.2946674646759)) ;
#34921=CARTESIAN_POINT('Ctrl Pts',(-19.4537302657956,10.5494507922323,-14.305276557685)) ;
#34922=CARTESIAN_POINT('Ctrl Pts',(-19.2415384579781,10.9405375788069,-14.3156076387216)) ;
#34923=CARTESIAN_POINT('Ctrl Pts',(-19.0175089331266,11.3252440359465,-14.325980963764)) ;
#34924=CARTESIAN_POINT('Ctrl Pts',(-18.7820798455872,11.7028728538607,-14.3363382067553)) ;
#34925=CARTESIAN_POINT('Ctrl Pts',(-18.5466749662204,12.0804628418083,-14.3466943847554)) ;
#34926=CARTESIAN_POINT('Ctrl Pts',(-18.2998729378895,12.4509767361701,-14.3570343892884)) ;
#34927=CARTESIAN_POINT('Ctrl Pts',(-18.0421419942429,12.8137426554905,-14.3673219567152)) ;
#34928=CARTESIAN_POINT('Ctrl Pts',(-17.7844264268254,13.1764869321948,-14.3776089103856)) ;
#34929=CARTESIAN_POINT('Ctrl Pts',(-17.5157831952769,13.5314842987859,-14.3878433925137)) ;
#34930=CARTESIAN_POINT('Ctrl Pts',(-17.2367061848117,13.8780835626764,-14.3980091860119)) ;
#34931=CARTESIAN_POINT('Ctrl Pts',(-16.9444206175783,14.2410871733287,-14.408656120756)) ;
#34932=CARTESIAN_POINT('Ctrl Pts',(-16.6407067022616,14.5948927994589,-14.4192401493713)) ;
#34933=CARTESIAN_POINT('Ctrl Pts',(-16.3261505940965,14.9387669198136,-14.4297579850172)) ;
#34934=CARTESIAN_POINT('Ctrl Pts',(-16.0257803526236,15.267132988334,-14.4398014867987)) ;
#34935=CARTESIAN_POINT('Ctrl Pts',(-15.7155314827287,15.5864494845368,-14.4497905070229)) ;
#34936=CARTESIAN_POINT('Ctrl Pts',(-15.3959637602158,15.896116707577,-14.4597589511553)) ;
#34937=CARTESIAN_POINT('Ctrl Pts',(-15.0763817292767,16.2057977957552,-14.469727841618)) ;
#34938=CARTESIAN_POINT('Ctrl Pts',(-14.7474799019799,16.5058286643848,-14.4796762704406)) ;
#34939=CARTESIAN_POINT('Ctrl Pts',(-14.4098502042424,16.7956339081327,-14.4896595384377)) ;
#34940=CARTESIAN_POINT('Ctrl Pts',(-14.0721644005434,17.0854873105644,-14.4996444654145)) ;
#34941=CARTESIAN_POINT('Ctrl Pts',(-13.7257476930588,17.3651115418814,-14.5096644186357)) ;
#34942=CARTESIAN_POINT('Ctrl Pts',(-13.3712262126238,17.6339570063594,-14.5197939424411)) ;
#34943=CARTESIAN_POINT('Ctrl Pts',(-13.3210974962862,17.6719712841147,-14.5212262393639)) ;
#34944=CARTESIAN_POINT('Ctrl Pts',(-13.270806794774,17.7097701019362,-14.5226607556166)) ;
#34945=CARTESIAN_POINT('Ctrl Pts',(-13.2203559353334,17.7473519512511,-14.5240977294154)) ;
#34946=CARTESIAN_POINT('Ctrl Pts',(-12.8540078718454,18.0202519151262,-14.5345322903779)) ;
#34947=CARTESIAN_POINT('Ctrl Pts',(-12.4791180167024,18.2817772414142,-14.5450967602933)) ;
#34948=CARTESIAN_POINT('Ctrl Pts',(-12.096446163701,18.5314468803889,-14.5557058533015)) ;
#34949=CARTESIAN_POINT('Ctrl Pts',(-11.7238022515889,18.7745739101754,-14.5660369343347)) ;
#34950=CARTESIAN_POINT('Ctrl Pts',(-11.3437789926822,19.0064588143181,-14.5764102593736)) ;
#34951=CARTESIAN_POINT('Ctrl Pts',(-10.9570934318374,19.2266965411546,-14.5867675023611)) ;
#34952=CARTESIAN_POINT('Ctrl Pts',(-10.5704476322249,19.446911621882,-14.5971236803574)) ;
#34953=CARTESIAN_POINT('Ctrl Pts',(-10.1771409189719,19.6554820328309,-14.6074636848866)) ;
#34954=CARTESIAN_POINT('Ctrl Pts',(-9.77790470493387,19.8520393955615,-14.6177512523094)) ;
#34955=CARTESIAN_POINT('Ctrl Pts',(-9.37869230932992,20.0485850316789,-14.628038205976)) ;
#34956=CARTESIAN_POINT('Ctrl Pts',(-8.97355100716818,20.233119151384,-14.6382726881001)) ;
#34957=CARTESIAN_POINT('Ctrl Pts',(-8.56322493812592,20.4053037746043,-14.6484384815999)) ;
#34958=CARTESIAN_POINT('Ctrl Pts',(-8.13347836857059,20.5856377985473,-14.6590854163499)) ;
#34959=CARTESIAN_POINT('Ctrl Pts',(-7.69805250397178,20.7524457118887,-14.6696694449544)) ;
#34960=CARTESIAN_POINT('Ctrl Pts',(-7.25781180429722,20.9053609899327,-14.6801872806006)) ;
#34961=CARTESIAN_POINT('Ctrl Pts',(-6.83742510131523,21.0513800872584,-14.6902307823785)) ;
#34962=CARTESIAN_POINT('Ctrl Pts',(-6.41265179725684,21.1847405989812,-14.7002198025993)) ;
#34963=CARTESIAN_POINT('Ctrl Pts',(-5.98426950815016,21.3051811759733,-14.7101882467287)) ;
#34964=CARTESIAN_POINT('Ctrl Pts',(-5.55586803851677,21.4256271456107,-14.7201571371884)) ;
#34965=CARTESIAN_POINT('Ctrl Pts',(-5.12385720369097,21.5331518991969,-14.7301055660084)) ;
#34966=CARTESIAN_POINT('Ctrl Pts',(-4.68903134808266,21.627530749068,-14.7400888340033)) ;
#34967=CARTESIAN_POINT('Ctrl Pts',(-4.2541332348432,21.721925282441,-14.7500737609779)) ;
#34968=CARTESIAN_POINT('Ctrl Pts',(-3.81641911883025,21.8031693500113,-14.7600937141973)) ;
#34969=CARTESIAN_POINT('Ctrl Pts',(-3.37670116039764,21.871077234674,-14.7702232380016)) ;
#34970=CARTESIAN_POINT('Ctrl Pts',(-3.31452581075605,21.8806792906995,-14.7716555349368)) ;
#34971=CARTESIAN_POINT('Ctrl Pts',(-3.2523104264018,21.8900147770267,-14.7730900512021)) ;
#34972=CARTESIAN_POINT('Ctrl Pts',(-3.19005733214379,21.8990832355265,-14.7745270250134)) ;
#34973=CARTESIAN_POINT('Ctrl Pts',(-2.73800754381034,21.9649336931498,-14.7849615859776)) ;
#34974=CARTESIAN_POINT('Ctrl Pts',(-2.28385283854564,22.0167159629141,-14.7955260558956)) ;
#34975=CARTESIAN_POINT('Ctrl Pts',(-1.82849036152256,22.0543681902254,-14.8061351489068)) ;
#34976=CARTESIAN_POINT('Ctrl Pts',(-1.38506068790057,22.0910337384651,-14.8164662299439)) ;
#34977=CARTESIAN_POINT('Ctrl Pts',(-0.94048567128749,22.1143004681896,-14.8268395549872)) ;
#34978=CARTESIAN_POINT('Ctrl Pts',(-0.495588710245009,22.1241530502275,
-14.8371967979794)) ;
#34979=CARTESIAN_POINT('Ctrl Pts',(-0.0507374960671489,22.1340046191662,
-14.8475529759804)) ;
#34980=CARTESIAN_POINT('Ctrl Pts',(0.394435633723673,22.130444906467,-14.8578929805146)) ;
#34981=CARTESIAN_POINT('Ctrl Pts',(0.839112081126021,22.1134976766824,-14.8681805479425)) ;
#34982=CARTESIAN_POINT('Ctrl Pts',(1.28376199912979,22.0965514579695,-14.878467501614)) ;
#34983=CARTESIAN_POINT('Ctrl Pts',(1.72791544045982,22.0662193522683,-14.8887019837431)) ;
#34984=CARTESIAN_POINT('Ctrl Pts',(2.17075706739576,22.022557917448,-14.8988677772327)) ;
#34985=CARTESIAN_POINT('Ctrl Pts',(2.63455813772609,21.9768300116459,-14.9095147119707)) ;
#34986=CARTESIAN_POINT('Ctrl Pts',(3.09692288641447,21.9165025497567,-14.9200987406087)) ;
#34987=CARTESIAN_POINT('Ctrl Pts',(3.55691655691509,21.8416641974045,-14.9306165762575)) ;
#34988=CARTESIAN_POINT('Ctrl Pts',(3.99616541033259,21.7702009087324,-14.940660078039)) ;
#34989=CARTESIAN_POINT('Ctrl Pts',(4.43325332453221,21.6855159560118,-14.9506490982629)) ;
#34990=CARTESIAN_POINT('Ctrl Pts',(4.86737195482524,21.587749228196,-14.9606175423944)) ;
#34991=CARTESIAN_POINT('Ctrl Pts',(5.30151002248591,21.4899781229412,-14.9705864328562)) ;
#34992=CARTESIAN_POINT('Ctrl Pts',(5.73267853131744,21.3791239346503,-14.9805348616774)) ;
#34993=CARTESIAN_POINT('Ctrl Pts',(6.16007185520018,21.2553667581344,-14.9905181296721)) ;
#34994=CARTESIAN_POINT('Ctrl Pts',(6.5875362016034,21.1315890161439,-15.0005030566466)) ;
#34995=CARTESIAN_POINT('Ctrl Pts',(7.0112240574055,20.9949038057253,-15.0105230098646)) ;
#34996=CARTESIAN_POINT('Ctrl Pts',(7.43033265642514,20.8455339760244,-15.0206525336659)) ;
#34997=CARTESIAN_POINT('Ctrl Pts',(7.48959387855016,20.8244133436218,-15.0220848305966)) ;
#34998=CARTESIAN_POINT('Ctrl Pts',(7.54876355168885,20.8030391743093,-15.0235193468573)) ;
#34999=CARTESIAN_POINT('Ctrl Pts',(7.60783941286998,20.7814121706377,-15.024956320664)) ;
#35000=CARTESIAN_POINT('Ctrl Pts',(8.03681777829409,20.6243680497633,-15.0353908816239)) ;
#35001=CARTESIAN_POINT('Ctrl Pts',(8.46095769649285,20.4539473069933,-15.0459553515357)) ;
#35002=CARTESIAN_POINT('Ctrl Pts',(8.87944054383028,20.2705221664442,-15.0565644445398)) ;
#35003=CARTESIAN_POINT('Ctrl Pts',(9.28695702112645,20.0919036935493,-15.0668955255765)) ;
#35004=CARTESIAN_POINT('Ctrl Pts',(9.68910924282036,19.9009537604632,-15.0772688506184)) ;
#35005=CARTESIAN_POINT('Ctrl Pts',(10.0851655844955,19.6980504490424,-15.0876260936088)) ;
#35006=CARTESIAN_POINT('Ctrl Pts',(10.4811812013808,19.4951680013064,-15.097982271608)) ;
#35007=CARTESIAN_POINT('Ctrl Pts',(10.8711022758455,19.2803347101707,-15.1083222761399)) ;
#35008=CARTESIAN_POINT('Ctrl Pts',(11.254219997474,19.053960764905,-15.1186098435656)) ;
#35009=CARTESIAN_POINT('Ctrl Pts',(11.6373148622978,18.8276003251097,-15.128896797235)) ;
#35010=CARTESIAN_POINT('Ctrl Pts',(12.0136073304412,18.589700567336,-15.1391312793621)) ;
#35011=CARTESIAN_POINT('Ctrl Pts',(12.3824070543977,18.3406989783901,-15.1492970728808)) ;
#35012=CARTESIAN_POINT('Ctrl Pts',(12.7686618599914,18.0799122855504,-15.1599440076376)) ;
#35013=CARTESIAN_POINT('Ctrl Pts',(13.1467103378622,17.8069655660871,-15.1705280362015)) ;
#35014=CARTESIAN_POINT('Ctrl Pts',(13.5157723580305,17.5223813413833,-15.18104587184)) ;
#35015=CARTESIAN_POINT('Ctrl Pts',(13.8681904015218,17.250631309687,-15.1910893736226)) ;
#35016=CARTESIAN_POINT('Ctrl Pts',(14.2124199351184,16.9682779594212,-15.201078393849)) ;
#35017=CARTESIAN_POINT('Ctrl Pts',(14.5478163910286,16.675828757253,-15.211046837985)) ;
#35018=CARTESIAN_POINT('Ctrl Pts',(14.8832278640873,16.3833664608704,-15.2210157284513)) ;
#35019=CARTESIAN_POINT('Ctrl Pts',(15.2098053956224,16.0808072927439,-15.2309641572789)) ;
#35020=CARTESIAN_POINT('Ctrl Pts',(15.526925929212,15.7686927953774,-15.2409474252827)) ;
#35021=CARTESIAN_POINT('Ctrl Pts',(15.844099160628,15.4565264320678,-15.2509323522662)) ;
#35022=CARTESIAN_POINT('Ctrl Pts',(16.1518121149721,15.1348014192352,-15.2609523054958)) ;
#35023=CARTESIAN_POINT('Ctrl Pts',(16.4494645834814,14.8040955498571,-15.2710818293117)) ;
#35024=CARTESIAN_POINT('Ctrl Pts',(16.4915521203773,14.7573343200617,-15.2725141262098)) ;
#35025=CARTESIAN_POINT('Ctrl Pts',(16.5334385533032,14.7103935927233,-15.2739486424378)) ;
#35026=CARTESIAN_POINT('Ctrl Pts',(16.5751222256453,14.6632750620232,-15.2753856162117)) ;
#35027=CARTESIAN_POINT('Ctrl Pts',(16.8778075135283,14.3211246412901,-15.2858201771801)) ;
#35028=CARTESIAN_POINT('Ctrl Pts',(17.1698752271347,13.9695078748294,-15.2963846471033)) ;
#35029=CARTESIAN_POINT('Ctrl Pts',(17.4507822432622,13.6091415001395,-15.3069937401202)) ;
#35030=CARTESIAN_POINT('Ctrl Pts',(17.7243280722034,13.2582185504531,-15.3173248211435)) ;
#35031=CARTESIAN_POINT('Ctrl Pts',(17.9872908051944,12.8989987202108,-15.3276981461732)) ;
#35032=CARTESIAN_POINT('Ctrl Pts',(18.2392066369358,12.5321625274619,-15.3380553891518)) ;
#35033=CARTESIAN_POINT('Ctrl Pts',(18.4910965652423,12.1653640549205,-15.3484115671391)) ;
#35034=CARTESIAN_POINT('Ctrl Pts',(18.7319419744567,11.7909508137328,-15.3587515716595)) ;
#35035=CARTESIAN_POINT('Ctrl Pts',(18.9613143971691,11.4096207172977,-15.3690391390733)) ;
#35036=CARTESIAN_POINT('Ctrl Pts',(19.1906731355211,11.0283133710189,-15.3793260927307)) ;
#35037=CARTESIAN_POINT('Ctrl Pts',(19.4085603638977,10.6400898901897,-15.3895605748454)) ;
#35038=CARTESIAN_POINT('Ctrl Pts',(19.6145768377597,10.245663421493,-15.3997263683028)) ;
#35039=CARTESIAN_POINT('Ctrl Pts',(19.8303439553452,9.83256897008963,-15.4103733030414)) ;
#35040=CARTESIAN_POINT('Ctrl Pts',(20.033109362744,9.41267999232148,-15.4209573317316)) ;
#35041=CARTESIAN_POINT('Ctrl Pts',(20.2224352726086,8.98682713471104,-15.4314751673962)) ;
#35042=CARTESIAN_POINT('Ctrl Pts',(20.4032229527388,8.58017941143189,-15.4415186691607)) ;
#35043=CARTESIAN_POINT('Ctrl Pts',(20.5717648884173,8.16809810738047,-15.4515076893666)) ;
#35044=CARTESIAN_POINT('Ctrl Pts',(20.7277353859778,7.7513361592637,-15.4614761334789)) ;
#35045=CARTESIAN_POINT('Ctrl Pts',(20.883712867013,7.33455555090941,-15.4714450239216)) ;
#35046=CARTESIAN_POINT('Ctrl Pts',(21.027117665037,6.91309381214329,-15.4813934527224)) ;
#35047=CARTESIAN_POINT('Ctrl Pts',(21.1576592144443,6.48772362609034,-15.4913767206954)) ;
#35048=CARTESIAN_POINT('Ctrl Pts',(21.2882224567299,6.06228275370249,-15.5013616476484)) ;
#35049=CARTESIAN_POINT('Ctrl Pts',(21.4059179868281,5.63293207259755,-15.5113816008435)) ;
#35050=CARTESIAN_POINT('Ctrl Pts',(21.510492576861,5.20046528985004,-15.5215111246202)) ;
#35051=CARTESIAN_POINT('Ctrl Pts',(21.5252792418472,5.13931523961193,-15.5229434216487)) ;
#35052=CARTESIAN_POINT('Ctrl Pts',(21.5398036378763,5.07810292224206,-15.5243779380074)) ;
#35053=CARTESIAN_POINT('Ctrl Pts',(21.5540651133108,5.01683061589433,-15.5258149119125)) ;
#35054=CARTESIAN_POINT('Ctrl Pts',(21.6576245685067,4.5719028317288,-15.5362494728682)) ;
#35055=CARTESIAN_POINT('Ctrl Pts',(21.7473421448813,4.12369678955954,-15.5468139427755)) ;
#35056=CARTESIAN_POINT('Ctrl Pts',(21.8230809070896,3.67310127741325,-15.5574230357757)) ;
#35057=CARTESIAN_POINT('Ctrl Pts',(21.8968349304165,3.23431364813468,-15.567754116847)) ;
#35058=CARTESIAN_POINT('Ctrl Pts',(21.9573335435185,2.79326013028553,-15.5781274419242)) ;
#35059=CARTESIAN_POINT('Ctrl Pts',(22.0044923619925,2.35075993046879,-15.5884846849508)) ;
#35060=CARTESIAN_POINT('Ctrl Pts',(22.0516463313258,1.90830523106504,-15.5988408629862)) ;
#35061=CARTESIAN_POINT('Ctrl Pts',(22.085463359548,1.46440411896152,-15.609180867555)) ;
#35062=CARTESIAN_POINT('Ctrl Pts',(22.1058984209575,1.0198742983453,-15.6194684350184)) ;
#35063=CARTESIAN_POINT('Ctrl Pts',(22.1263322632109,0.575370998383557,-15.6297553887254)) ;
#35064=CARTESIAN_POINT('Ctrl Pts',(22.1333857802633,0.130238921738118,-15.6399898708908)) ;
#35065=CARTESIAN_POINT('Ctrl Pts',(22.1270468977107,-0.314704723780525,
-15.6501556644476)) ;
#35066=CARTESIAN_POINT('Ctrl Pts',(22.1204079994866,-0.780707296565286,
-15.6608025991765)) ;
#35067=CARTESIAN_POINT('Ctrl Pts',(22.0991005065641,-1.24650398272563,-15.6713866277163)) ;
#35068=CARTESIAN_POINT('Ctrl Pts',(22.0631343161778,-1.71115588215796,-15.6819044633305)) ;
#35069=CARTESIAN_POINT('Ctrl Pts',(22.0287901305526,-2.1548528907594,-15.6919479651533)) ;
#35070=CARTESIAN_POINT('Ctrl Pts',(21.9810895618747,-2.59750630302009,-15.7019369854204)) ;
#35071=CARTESIAN_POINT('Ctrl Pts',(21.9201041596768,-3.03829888535571,-15.7119054295972)) ;
#35072=CARTESIAN_POINT('Ctrl Pts',(21.8591160269008,-3.47911120386594,-15.721874320104)) ;
#35073=CARTESIAN_POINT('Ctrl Pts',(21.7848417342053,-3.91806252827625,-15.7318227489723)) ;
#35074=CARTESIAN_POINT('Ctrl Pts',(21.6973931232892,-4.35433495942962,-15.7418060170167)) ;
#35075=CARTESIAN_POINT('Ctrl Pts',(21.6099299805154,-4.79067988857734,-15.7517909440404)) ;
#35076=CARTESIAN_POINT('Ctrl Pts',(21.5092879455416,-5.22434499945482,-15.7618108973102)) ;
#35077=CARTESIAN_POINT('Ctrl Pts',(21.3956217035828,-5.65451165430317,-15.7719404211659)) ;
#35078=CARTESIAN_POINT('Ctrl Pts',(21.3795494986091,-5.7153364562003,-15.7733727178698)) ;
#35079=CARTESIAN_POINT('Ctrl Pts',(21.3632169675423,-5.77609131197269,-15.774807233903)) ;
#35080=CARTESIAN_POINT('Ctrl Pts',(21.3466246205186,-5.83677390766786,-15.7762442074813)) ;
#35081=CARTESIAN_POINT('Ctrl Pts',(21.2261395543992,-6.27741961886123,-15.7866787684481)) ;
#35082=CARTESIAN_POINT('Ctrl Pts',(21.0919189661969,-6.71436667920628,-15.7972432383664)) ;
#35083=CARTESIAN_POINT('Ctrl Pts',(20.9442650580843,-7.14676811213256,-15.8078523313749)) ;
#35084=CARTESIAN_POINT('Ctrl Pts',(20.8004804313346,-7.56783843417188,-15.8181834123322)) ;
#35085=CARTESIAN_POINT('Ctrl Pts',(20.6439576245207,-7.98459843006223,-15.8285567372921)) ;
#35086=CARTESIAN_POINT('Ctrl Pts',(20.47501197888,-8.39628732384464,-15.8389139801985)) ;
#35087=CARTESIAN_POINT('Ctrl Pts',(20.3060837052022,-8.80793388540734,-15.8492701581137)) ;
#35088=CARTESIAN_POINT('Ctrl Pts',(20.1247352309551,-9.21451046497884,-15.8596101625594)) ;
#35089=CARTESIAN_POINT('Ctrl Pts',(19.9313158063182,-9.61527632526949,-15.8698977298976)) ;
#35090=CARTESIAN_POINT('Ctrl Pts',(19.7379079210824,-10.0160182758726,-15.8801846834797)) ;
#35091=CARTESIAN_POINT('Ctrl Pts',(19.5324304971458,-10.4109503478303,-15.8904191655179)) ;
#35092=CARTESIAN_POINT('Ctrl Pts',(19.3152615355607,-10.7993479105026,-15.9005849589674)) ;
#35093=CARTESIAN_POINT('Ctrl Pts',(19.0878140871097,-11.2061281150475,-15.9112318937997)) ;
#35094=CARTESIAN_POINT('Ctrl Pts',(18.8475607465869,-11.6057515606328,-15.9218159223724)) ;
#35095=CARTESIAN_POINT('Ctrl Pts',(18.594956714121,-11.9973970138781,-15.93233375806)) ;
#35096=CARTESIAN_POINT('Ctrl Pts',(18.3537446337449,-12.371380016544,-15.9423772597511)) ;
#35097=CARTESIAN_POINT('Ctrl Pts',(18.1012793724234,-12.7380933581479,-15.952366279886)) ;
#35098=CARTESIAN_POINT('Ctrl Pts',(17.83801250649,-13.0968521526768,-15.9623347239313)) ;
#35099=CARTESIAN_POINT('Ctrl Pts',(17.5747338529472,-13.4556270104065,-15.9723036143074)) ;
#35100=CARTESIAN_POINT('Ctrl Pts',(17.3006525060449,-13.8064465458687,-15.9822520430458)) ;
#35101=CARTESIAN_POINT('Ctrl Pts',(17.0162558032043,-14.1486444484711,-15.992235310962)) ;
#35102=CARTESIAN_POINT('Ctrl Pts',(16.7318118404237,-14.4908992161926,-16.0022202378589)) ;
#35103=CARTESIAN_POINT('Ctrl Pts',(16.4370489379124,-14.8245293621743,-16.0122401910037)) ;
#35104=CARTESIAN_POINT('Ctrl Pts',(16.1324924733015,-15.1488883002968,-16.0223697147375)) ;
#35105=CARTESIAN_POINT('Ctrl Pts',(16.0894287103524,-15.1947520991151,-16.0238020120602)) ;
#35106=CARTESIAN_POINT('Ctrl Pts',(16.0461692040839,-15.2404305689993,-16.0252365287142)) ;
#35107=CARTESIAN_POINT('Ctrl Pts',(16.0027155036575,-15.2859219169845,-16.0266735029158)) ;
#35108=CARTESIAN_POINT('Ctrl Pts',(15.6871772801474,-15.6162564796911,-16.0371080638932)) ;
#35109=CARTESIAN_POINT('Ctrl Pts',(15.3613149608306,-15.9368054596001,-16.0476725338348)) ;
#35110=CARTESIAN_POINT('Ctrl Pts',(15.025797168888,-16.2469674928623,-16.0582816268791)) ;
#35111=CARTESIAN_POINT('Ctrl Pts',(14.6990716395051,-16.5490017126434,-16.068612708045)) ;
#35112=CARTESIAN_POINT('Ctrl Pts',(14.3631902466487,-16.8411865507727,-16.0789860332267)) ;
#35113=CARTESIAN_POINT('Ctrl Pts',(14.0187921791655,-17.1230027213753,-16.0893432763632)) ;
#35114=CARTESIAN_POINT('Ctrl Pts',(13.6744295246733,-17.4047899140176,-16.0996994545084)) ;
#35115=CARTESIAN_POINT('Ctrl Pts',(13.3215519837295,-17.67621067911,-16.1100394591926)) ;
#35116=CARTESIAN_POINT('Ctrl Pts',(12.9608190451236,-17.9367794839549,-16.120327026772)) ;
#35117=CARTESIAN_POINT('Ctrl Pts',(12.6001076278555,-18.1973327432572,-16.1306139805949)) ;
#35118=CARTESIAN_POINT('Ctrl Pts',(12.2315416550019,-18.4470354531436,-16.1408484628769)) ;
#35119=CARTESIAN_POINT('Ctrl Pts',(11.8557982474563,-18.6854299218368,-16.151014256314)) ;
#35120=CARTESIAN_POINT('Ctrl Pts',(11.4622711235392,-18.935107461718,-16.1616611908266)) ;
#35121=CARTESIAN_POINT('Ctrl Pts',(11.0608821915056,-19.1723994457757,-16.1722452198653)) ;
#35122=CARTESIAN_POINT('Ctrl Pts',(10.6524224217679,-19.3967999123517,-16.1827630554936)) ;
#35123=CARTESIAN_POINT('Ctrl Pts',(10.2623833845461,-19.6110803590934,-16.1928065574148)) ;
#35124=CARTESIAN_POINT('Ctrl Pts',(9.86590213146238,-19.8136143204186,-16.2027955777705)) ;
#35125=CARTESIAN_POINT('Ctrl Pts',(9.4637016064469,-20.0040140565321,-16.2127640220214)) ;
#35126=CARTESIAN_POINT('Ctrl Pts',(9.06148307321215,-20.1944223176474,-16.2227329126018)) ;
#35127=CARTESIAN_POINT('Ctrl Pts',(8.65354467893047,-20.3726951538725,-16.2326813415289)) ;
#35128=CARTESIAN_POINT('Ctrl Pts',(8.2406319926359,-20.5384781721711,-16.2426646096125)) ;
#35129=CARTESIAN_POINT('Ctrl Pts',(7.82765069020417,-20.704288739612,-16.2526495366748)) ;
#35130=CARTESIAN_POINT('Ctrl Pts',(7.40969336449929,-20.8576051555763,-16.2626694899634)) ;
#35131=CARTESIAN_POINT('Ctrl Pts',(6.98752966814416,-20.9981084684307,-16.2727990138138)) ;
#35132=CARTESIAN_POINT('Ctrl Pts',(6.92783648149656,-21.0179753839217,-16.2742313102502)) ;
#35133=CARTESIAN_POINT('Ctrl Pts',(6.86805923479046,-21.0375861822736,-16.2756658260145)) ;
#35134=CARTESIAN_POINT('Ctrl Pts',(6.80820014344603,-21.0569400229394,-16.2771027993227)) ;
#35135=CARTESIAN_POINT('Ctrl Pts',(6.3840662249976,-21.1940724132621,-16.2872845295527)) ;
#35136=CARTESIAN_POINT('Ctrl Pts',(5.95571662068674,-21.3183340351005,-16.2975900166844)) ;
#35137=CARTESIAN_POINT('Ctrl Pts',(5.52396187406269,-21.4295287131257,-16.3079398138918)) ;
#35138=CARTESIAN_POINT('Ctrl Pts',(5.07349743468953,-21.5455419097137,-16.318738109992)) ;
#35139=CARTESIAN_POINT('Ctrl Pts',(4.6193263349758,-21.6473310109628,-16.3295842934684)) ;
#35140=CARTESIAN_POINT('Ctrl Pts',(4.16237135896441,-21.734721310978,-16.3404117032938)) ;
#35141=CARTESIAN_POINT('Ctrl Pts',(3.72451307507802,-21.81845946638,-16.3507866227802)) ;
#35142=CARTESIAN_POINT('Ctrl Pts',(3.28409872649029,-21.8889775702143,-16.3611443679875)) ;
#35143=CARTESIAN_POINT('Ctrl Pts',(2.84194227547393,-21.9461619586397,-16.3714489886679)) ;
#35144=CARTESIAN_POINT('Ctrl Pts',(2.39982355247863,-22.003341467675,-16.3817527300827)) ;
#35145=CARTESIAN_POINT('Ctrl Pts',(1.95596293810181,-22.0471895885666,-16.3920033160626)) ;
#35146=CARTESIAN_POINT('Ctrl Pts',(1.51117670721767,-22.0776282696489,-16.4021866747302)) ;
#35147=CARTESIAN_POINT('Ctrl Pts',(1.06639929112509,-22.1080663474962,-16.4123698315837)) ;
#35148=CARTESIAN_POINT('Ctrl Pts',(0.620696708842184,-22.1251049600064,
-16.4224912401162)) ;
#35149=CARTESIAN_POINT('Ctrl Pts',(0.174887699130083,-22.1286943106416,
-16.4325548170702)) ;
#35150=CARTESIAN_POINT('Ctrl Pts',(0.116466280787281,-22.1291646801283,
-16.4338736070149)) ;
#35151=CARTESIAN_POINT('Ctrl Pts',(0.0580430444652074,-22.1294042197614,
-16.4351914834666)) ;
#35152=CARTESIAN_POINT('Ctrl Pts',(-0.000380161200413355,-22.1294128925051,
-16.4365085000897)) ;
#35153=CARTESIAN_POINT('Origin',(0.,0.,-10.)) ;
#35154=CARTESIAN_POINT('',(-2.71011275034311E-15,-22.12975,-20.)) ;
#35155=CARTESIAN_POINT('',(0.00050934658643668,-22.1297499941383,-19.6109246391395)) ;
#35156=CARTESIAN_POINT('',(-2.71011275034311E-15,-22.12975,-10.)) ;
#35157=CARTESIAN_POINT('',(3.34070509846219,-21.8761405304411,-20.)) ;
#35158=CARTESIAN_POINT('Origin',(0.,0.,-20.)) ;
#35159=CARTESIAN_POINT('Ctrl Pts',(3.3407050984622,-21.8761405304411,-20.)) ;
#35160=CARTESIAN_POINT('Ctrl Pts',(3.79243697068971,-21.8071565628812,-19.9895654460161)) ;
#35161=CARTESIAN_POINT('Ctrl Pts',(4.24205501176312,-21.7241722534374,-19.9791308920322)) ;
#35162=CARTESIAN_POINT('Ctrl Pts',(4.6886871030314,-21.6273449205483,-19.9686963380483)) ;
#35163=CARTESIAN_POINT('Ctrl Pts',(5.12615421837869,-21.5325045030461,-19.9584759031075)) ;
#35164=CARTESIAN_POINT('Ctrl Pts',(5.56075648282984,-21.4243835827313,-19.9482554681667)) ;
#35165=CARTESIAN_POINT('Ctrl Pts',(5.99168520350615,-21.3031815343292,-19.9380350332259)) ;
#35166=CARTESIAN_POINT('Ctrl Pts',(6.42260071072155,-21.1819832023156,-19.9278149116718)) ;
#35167=CARTESIAN_POINT('Ctrl Pts',(6.84984268386217,-21.0477046044914,-19.9175947901176)) ;
#35168=CARTESIAN_POINT('Ctrl Pts',(7.27261650517739,-20.9005953080557,-19.9073746685635)) ;
#35169=CARTESIAN_POINT('Ctrl Pts',(7.69539013295677,-20.7534860789633,-19.8971545516879)) ;
#35170=CARTESIAN_POINT('Ctrl Pts',(8.11369540181686,-20.5935462370468,-19.8869344348123)) ;
#35171=CARTESIAN_POINT('Ctrl Pts',(8.52675489776927,-20.4210745548776,-19.8767143179368)) ;
#35172=CARTESIAN_POINT('Ctrl Pts',(8.9549779599098,-20.2422713737505,-19.8661190168075)) ;
#35173=CARTESIAN_POINT('Ctrl Pts',(9.37756266132238,-20.0499991455787,-19.8555237156783)) ;
#35174=CARTESIAN_POINT('Ctrl Pts',(9.79366589611002,-19.8446452066514,-19.8449284145491)) ;
#35175=CARTESIAN_POINT('Ctrl Pts',(10.1951078639102,-19.646526849363,-19.8347064355325)) ;
#35176=CARTESIAN_POINT('Ctrl Pts',(10.5905169982379,-19.4362327966258,-19.8244844565158)) ;
#35177=CARTESIAN_POINT('Ctrl Pts',(10.9791601023046,-19.2141582826431,-19.8142624774992)) ;
#35178=CARTESIAN_POINT('Ctrl Pts',(11.3678262810571,-18.9920705835567,-19.8040398915789)) ;
#35179=CARTESIAN_POINT('Ctrl Pts',(11.7497254337773,-18.7582011388228,-19.7938173056585)) ;
#35180=CARTESIAN_POINT('Ctrl Pts',(12.1241506717191,-18.5129901839749,-19.7835947197381)) ;
#35181=CARTESIAN_POINT('Ctrl Pts',(12.498637489504,-18.2677389005099,-19.7733704525603)) ;
#35182=CARTESIAN_POINT('Ctrl Pts',(12.8656477491244,-18.0111425023592,-19.7631461853824)) ;
#35183=CARTESIAN_POINT('Ctrl Pts',(13.2245034898344,-17.7436845809955,-19.7529219182046)) ;
#35184=CARTESIAN_POINT('Ctrl Pts',(13.2637109393324,-17.7144629697599,-19.7518048469318)) ;
#35185=CARTESIAN_POINT('Ctrl Pts',(13.3028210782212,-17.6851117451297,-19.7506877756589)) ;
#35186=CARTESIAN_POINT('Ctrl Pts',(13.3418330449212,-17.6556315679714,-19.7495707043861)) ;
#35187=CARTESIAN_POINT('Ctrl Pts',(13.7062435193986,-17.3802574647239,-19.7391361504022)) ;
#35188=CARTESIAN_POINT('Ctrl Pts',(14.0621855564206,-17.093551993444,-19.7287015964183)) ;
#35189=CARTESIAN_POINT('Ctrl Pts',(14.4089555524661,-16.7960660557631,-19.7182670424344)) ;
#35190=CARTESIAN_POINT('Ctrl Pts',(14.7456256827497,-16.5072445586938,-19.7081364005413)) ;
#35191=CARTESIAN_POINT('Ctrl Pts',(15.07365025053,-16.2082617802615,-19.6980057586482)) ;
#35192=CARTESIAN_POINT('Ctrl Pts',(15.3924188474478,-15.8996627979097,-19.6878751167551)) ;
#35193=CARTESIAN_POINT('Ctrl Pts',(15.7111459282296,-15.5911040072124,-19.6777457942677)) ;
#35194=CARTESIAN_POINT('Ctrl Pts',(16.0206192789643,-15.2729316755362,-19.6676164717803)) ;
#35195=CARTESIAN_POINT('Ctrl Pts',(16.320264375849,-14.9457286796226,-19.6574871492929)) ;
#35196=CARTESIAN_POINT('Ctrl Pts',(16.6198851681435,-14.618552223555,-19.6473586484075)) ;
#35197=CARTESIAN_POINT('Ctrl Pts',(16.9096791421221,-14.2823467377391,-19.6372301475222)) ;
#35198=CARTESIAN_POINT('Ctrl Pts',(17.1891100231423,-13.9377305066072,-19.6271016466369)) ;
#35199=CARTESIAN_POINT('Ctrl Pts',(17.4685319635363,-13.5931253017616,-19.6169734698214)) ;
#35200=CARTESIAN_POINT('Ctrl Pts',(17.7375913273382,-13.2401100698593,-19.606845293006)) ;
#35201=CARTESIAN_POINT('Ctrl Pts',(17.9957922924994,-12.8793359622194,-19.5967171161906)) ;
#35202=CARTESIAN_POINT('Ctrl Pts',(18.2540199317834,-12.5185245838713,-19.5865878930575)) ;
#35203=CARTESIAN_POINT('Ctrl Pts',(18.5013867940576,-12.1499529159039,-19.5764586699244)) ;
#35204=CARTESIAN_POINT('Ctrl Pts',(18.7374394273198,-11.7743024748823,-19.5663294467913)) ;
#35205=CARTESIAN_POINT('Ctrl Pts',(18.9735016270929,-11.3986368098661,-19.556199813151)) ;
#35206=CARTESIAN_POINT('Ctrl Pts',(19.1982485601447,-11.0158919966168,-19.5460701795106)) ;
#35207=CARTESIAN_POINT('Ctrl Pts',(19.411271159721,-10.6267768879508,-19.5359405458703)) ;
#35208=CARTESIAN_POINT('Ctrl Pts',(19.6243313335516,-10.2375931447357,-19.525809125502)) ;
#35209=CARTESIAN_POINT('Ctrl Pts',(19.8256629301047,-9.84203706470778,-19.5156777051336)) ;
#35210=CARTESIAN_POINT('Ctrl Pts',(20.0149028339713,-9.4408421027569,-19.5055462847653)) ;
#35211=CARTESIAN_POINT('Ctrl Pts',(20.054780694894,-9.35629969616782,-19.503411326101)) ;
#35212=CARTESIAN_POINT('Ctrl Pts',(20.0941217827245,-9.27150697063714,-19.5012763674367)) ;
#35213=CARTESIAN_POINT('Ctrl Pts',(20.1329229677406,-9.18647091311582,-19.4991414087723)) ;
#35214=CARTESIAN_POINT('Ctrl Pts',(20.322562732882,-8.77085943191464,-19.4887068547884)) ;
#35215=CARTESIAN_POINT('Ctrl Pts',(20.4993499633938,-8.34932714801769,-19.4782723008045)) ;
#35216=CARTESIAN_POINT('Ctrl Pts',(20.6629329963277,-7.92269114958888,-19.4678377468206)) ;
#35217=CARTESIAN_POINT('Ctrl Pts',(20.8224877607088,-7.50656115746839,-19.4576601460483)) ;
#35218=CARTESIAN_POINT('Ctrl Pts',(20.9694807490619,-7.0855760176988,-19.447482545276)) ;
#35219=CARTESIAN_POINT('Ctrl Pts',(21.1036346104306,-6.66051359070265,-19.4373049445037)) ;
#35220=CARTESIAN_POINT('Ctrl Pts',(21.2377764380265,-6.23548929234978,-19.4271282566752)) ;
#35221=CARTESIAN_POINT('Ctrl Pts',(21.359081370659,-5.80638865474412,-19.4169515688467)) ;
#35222=CARTESIAN_POINT('Ctrl Pts',(21.467321673352,-5.37400551128574,-19.4067748810181)) ;
#35223=CARTESIAN_POINT('Ctrl Pts',(21.5755565743006,-4.94164394595661,-19.3965987010584)) ;
#35224=CARTESIAN_POINT('Ctrl Pts',(21.670728092663,-4.5060004232084,-19.3864225210986)) ;
#35225=CARTESIAN_POINT('Ctrl Pts',(21.7526590257418,-4.06788155829462,-19.3762463411389)) ;
#35226=CARTESIAN_POINT('Ctrl Pts',(21.8382264844152,-3.61031667457137,-19.3656184888072)) ;
#35227=CARTESIAN_POINT('Ctrl Pts',(21.9093514285122,-3.15005201733719,-19.3549906364754)) ;
#35228=CARTESIAN_POINT('Ctrl Pts',(21.9658916693059,-2.68801752874067,-19.3443627841437)) ;
#35229=CARTESIAN_POINT('Ctrl Pts',(22.0200346956006,-2.24557255302133,-19.3341855355121)) ;
#35230=CARTESIAN_POINT('Ctrl Pts',(22.0608038992464,-1.80150492822418,-19.3240082868804)) ;
#35231=CARTESIAN_POINT('Ctrl Pts',(22.0881273500749,-1.35663747160816,-19.3138310382488)) ;
#35232=CARTESIAN_POINT('Ctrl Pts',(22.1154519954715,-0.911750565602043,
-19.3036533446727)) ;
#35233=CARTESIAN_POINT('Ctrl Pts',(22.1293297018622,-0.466063985600068,
-19.2934756510967)) ;
#35234=CARTESIAN_POINT('Ctrl Pts',(22.1297405942435,-0.0204032838767659,
-19.2832979575206)) ;
#35235=CARTESIAN_POINT('Ctrl Pts',(22.1301515519295,0.425328248427631,-19.2731186463643)) ;
#35236=CARTESIAN_POINT('Ctrl Pts',(22.1170914187326,0.871033666252579,-19.262939335208)) ;
#35237=CARTESIAN_POINT('Ctrl Pts',(22.0905924393186,1.31588781528603,-19.2527600240517)) ;
#35238=CARTESIAN_POINT('Ctrl Pts',(22.0870799060446,1.374854803266,-19.2514107204206)) ;
#35239=CARTESIAN_POINT('Ctrl Pts',(22.0833313212298,1.43380683812886,-19.2500614167895)) ;
#35240=CARTESIAN_POINT('Ctrl Pts',(22.0793468285778,1.49274200244797,-19.2487121131585)) ;
#35241=CARTESIAN_POINT('Ctrl Pts',(22.0485335981691,1.94850461915425,-19.2382775591745)) ;
#35242=CARTESIAN_POINT('Ctrl Pts',(22.0035995302651,2.40337505914454,-19.2278430051906)) ;
#35243=CARTESIAN_POINT('Ctrl Pts',(21.9446221721438,2.85646508544292,-19.2174084512067)) ;
#35244=CARTESIAN_POINT('Ctrl Pts',(21.8872306192117,3.29737225822284,-19.2072544653999)) ;
#35245=CARTESIAN_POINT('Ctrl Pts',(21.8165410911735,3.73659326317763,-19.197100479593)) ;
#35246=CARTESIAN_POINT('Ctrl Pts',(21.7326775496694,4.17331541877621,-19.1869464937861)) ;
#35247=CARTESIAN_POINT('Ctrl Pts',(21.6488230510757,4.60999048312111,-19.176793602872)) ;
#35248=CARTESIAN_POINT('Ctrl Pts',(21.5517974198474,5.04416701032279,-19.1666407119579)) ;
#35249=CARTESIAN_POINT('Ctrl Pts',(21.4417758771208,5.47504176219896,-19.1564878210438)) ;
#35250=CARTESIAN_POINT('Ctrl Pts',(21.3317612926476,5.90588926363242,-19.1463355722438)) ;
#35251=CARTESIAN_POINT('Ctrl Pts',(21.2087524956298,6.33343518393133,-19.1361833234439)) ;
#35252=CARTESIAN_POINT('Ctrl Pts',(21.0729752571866,6.75688899364948,-19.1260310746439)) ;
#35253=CARTESIAN_POINT('Ctrl Pts',(20.9305987099914,7.20092432693188,-19.1153853865523)) ;
#35254=CARTESIAN_POINT('Ctrl Pts',(20.7741819950338,7.64045969298141,-19.1047396984607)) ;
#35255=CARTESIAN_POINT('Ctrl Pts',(20.6040440446311,8.07460240936996,-19.0940940103691)) ;
#35256=CARTESIAN_POINT('Ctrl Pts',(20.4417767872506,8.48866139934446,-19.0839407987813)) ;
#35257=CARTESIAN_POINT('Ctrl Pts',(20.2670289301901,8.89781506380064,-19.0737875871935)) ;
#35258=CARTESIAN_POINT('Ctrl Pts',(20.0801267919074,9.30130867584889,-19.0636343756057)) ;
#35259=CARTESIAN_POINT('Ctrl Pts',(19.8932161178159,9.70482071542506,-19.0534807003214)) ;
#35260=CARTESIAN_POINT('Ctrl Pts',(19.694150152377,10.1026719782809,-19.043327025037)) ;
#35261=CARTESIAN_POINT('Ctrl Pts',(19.4833023080315,10.4941300847833,-19.0331733497527)) ;
#35262=CARTESIAN_POINT('Ctrl Pts',(19.2724186442316,10.8856546933449,-19.023017949532)) ;
#35263=CARTESIAN_POINT('Ctrl Pts',(19.0497492113925,11.2707837727805,-19.0128625493114)) ;
#35264=CARTESIAN_POINT('Ctrl Pts',(18.8157130769916,11.6488100880231,-19.0027071490907)) ;
#35265=CARTESIAN_POINT('Ctrl Pts',(18.7817261199756,11.7037074403484,-19.0012323719087)) ;
#35266=CARTESIAN_POINT('Ctrl Pts',(18.747499525508,11.7584550484515,-18.9997575947267)) ;
#35267=CARTESIAN_POINT('Ctrl Pts',(18.7130346544292,11.8130507949738,-18.9982828175446)) ;
#35268=CARTESIAN_POINT('Ctrl Pts',(18.4691838800839,12.1993344121385,-18.9878482635607)) ;
#35269=CARTESIAN_POINT('Ctrl Pts',(18.2133371812781,12.5781141300808,-18.9774137095768)) ;
#35270=CARTESIAN_POINT('Ctrl Pts',(17.9459852961038,12.9486465244259,-18.9669791555929)) ;
#35271=CARTESIAN_POINT('Ctrl Pts',(17.6855825221689,13.3095479007423,-18.9568158204797)) ;
#35272=CARTESIAN_POINT('Ctrl Pts',(17.4142652102917,13.6626250534368,-18.9466524853664)) ;
#35273=CARTESIAN_POINT('Ctrl Pts',(17.1325301821108,14.0072211598719,-18.9364891502532)) ;
#35274=CARTESIAN_POINT('Ctrl Pts',(16.8508237559169,14.3517822826082,-18.9263268469306)) ;
#35275=CARTESIAN_POINT('Ctrl Pts',(16.5587018711189,14.6878639014468,-18.9161645436081)) ;
#35276=CARTESIAN_POINT('Ctrl Pts',(16.2567019280894,15.0148419067187,-18.9060022402855)) ;
#35277=CARTESIAN_POINT('Ctrl Pts',(15.954719742825,15.3418006855013,-18.8958405345121)) ;
#35278=CARTESIAN_POINT('Ctrl Pts',(15.6428608153228,15.6596567517417,-18.8856788287386)) ;
#35279=CARTESIAN_POINT('Ctrl Pts',(15.3217009513977,15.9678212357992,-18.8755171229652)) ;
#35280=CARTESIAN_POINT('Ctrl Pts',(14.985467828973,16.2904490555668,-18.8648784895456)) ;
#35281=CARTESIAN_POINT('Ctrl Pts',(14.6390401032639,16.6024537021538,-18.8542398561261)) ;
#35282=CARTESIAN_POINT('Ctrl Pts',(14.2831208788024,16.9032036319752,-18.8436012227066)) ;
#35283=CARTESIAN_POINT('Ctrl Pts',(13.9431244897694,17.1904988470508,-18.8334385321344)) ;
#35284=CARTESIAN_POINT('Ctrl Pts',(13.5944673083247,17.467523991423,-18.8232758415622)) ;
#35285=CARTESIAN_POINT('Ctrl Pts',(13.2377964855047,17.7337694602941,-18.8131131509901)) ;
#35286=CARTESIAN_POINT('Ctrl Pts',(12.8811098745721,18.0000267145796,-18.8029500105642)) ;
#35287=CARTESIAN_POINT('Ctrl Pts',(12.5164090986917,18.2555032047083,-18.7927868701383)) ;
#35288=CARTESIAN_POINT('Ctrl Pts',(12.1443721118082,18.4997313783859,-18.7826237297123)) ;
#35289=CARTESIAN_POINT('Ctrl Pts',(11.7722738496555,18.7439997769541,-18.772458915396)) ;
#35290=CARTESIAN_POINT('Ctrl Pts',(11.3928371539001,18.9770160314776,-18.7622941010796)) ;
#35291=CARTESIAN_POINT('Ctrl Pts',(11.0067681889689,19.1983564165478,-18.7521292867632)) ;
#35292=CARTESIAN_POINT('Ctrl Pts',(10.9526356997833,19.2293915607565,-18.7507040318191)) ;
#35293=CARTESIAN_POINT('Ctrl Pts',(10.8983728613506,19.2601972283926,-18.7492787768749)) ;
#35294=CARTESIAN_POINT('Ctrl Pts',(10.8439816606655,19.2907723226845,-18.7478535219308)) ;
#35295=CARTESIAN_POINT('Ctrl Pts',(10.4457736613714,19.5146182200516,-18.7374189679468)) ;
#35296=CARTESIAN_POINT('Ctrl Pts',(10.0405806954128,19.726158913574,-18.7269844139629)) ;
#35297=CARTESIAN_POINT('Ctrl Pts',(9.62918811115828,19.9249735603947,-18.716549859979)) ;
#35298=CARTESIAN_POINT('Ctrl Pts',(9.22858174703272,20.1185755256369,-18.7063888874852)) ;
#35299=CARTESIAN_POINT('Ctrl Pts',(8.82209691497259,20.3001101209105,-18.6962279149914)) ;
#35300=CARTESIAN_POINT('Ctrl Pts',(8.41048263201501,20.4692358665162,-18.6860669424976)) ;
#35301=CARTESIAN_POINT('Ctrl Pts',(7.99891062035745,20.6383442435188,-18.675907013499)) ;
#35302=CARTESIAN_POINT('Ctrl Pts',(7.58221042228983,20.7950462291208,-18.6657470845003)) ;
#35303=CARTESIAN_POINT('Ctrl Pts',(7.16115120186113,20.9390484150207,-18.6555871555017)) ;
#35304=CARTESIAN_POINT('Ctrl Pts',(6.74011703542317,21.0830420324599,-18.6454278310422)) ;
#35305=CARTESIAN_POINT('Ctrl Pts',(6.31472458195684,21.2143372856418,-18.6352685065827)) ;
#35306=CARTESIAN_POINT('Ctrl Pts',(5.88576003712376,21.3326900284024,-18.6251091821232)) ;
#35307=CARTESIAN_POINT('Ctrl Pts',(5.43648214166529,21.4566472920729,-18.6144687691393)) ;
#35308=CARTESIAN_POINT('Ctrl Pts',(4.98328597402742,21.5664067363189,-18.6038283561555)) ;
#35309=CARTESIAN_POINT('Ctrl Pts',(4.52709106641022,21.6617469641515,-18.5931879431716)) ;
#35310=CARTESIAN_POINT('Ctrl Pts',(4.09147980422567,21.7527854134847,-18.5830276286818)) ;
#35311=CARTESIAN_POINT('Ctrl Pts',(3.65313463063065,21.8306768528102,-18.5728673141919)) ;
#35312=CARTESIAN_POINT('Ctrl Pts',(3.21286681761231,21.8952808128781,-18.5627069997021)) ;
#35313=CARTESIAN_POINT('Ctrl Pts',(2.77257919737902,21.9598876794144,-18.5525462281097)) ;
#35314=CARTESIAN_POINT('Ctrl Pts',(2.33036899234188,22.011205841337,-18.5423854565173)) ;
#35315=CARTESIAN_POINT('Ctrl Pts',(1.88705457087286,22.049146471214,-18.5322246849249)) ;
#35316=CARTESIAN_POINT('Ctrl Pts',(1.4436663280189,22.0870934190217,-18.5220622213455)) ;
#35317=CARTESIAN_POINT('Ctrl Pts',(0.999173730027711,22.1116583641229,-18.5118997577662)) ;
#35318=CARTESIAN_POINT('Ctrl Pts',(0.554399116588597,22.1228044488493,-18.5017372941868)) ;
#35319=CARTESIAN_POINT('Ctrl Pts',(0.491476608361625,22.1243812915618,-18.5002996048968)) ;
#35320=CARTESIAN_POINT('Ctrl Pts',(0.42854845840298,22.1256896554998,-18.4988619156069)) ;
#35321=CARTESIAN_POINT('Ctrl Pts',(0.365616996697635,22.1267295205194,-18.497424226317)) ;
#35322=CARTESIAN_POINT('Ctrl Pts',(-0.0911310218380175,22.1342767198753,
-18.486989672333)) ;
#35323=CARTESIAN_POINT('Ctrl Pts',(-0.548172161965109,22.1276775334204,
-18.4765551183491)) ;
#35324=CARTESIAN_POINT('Ctrl Pts',(-1.00461540528293,22.106935177676,-18.4661205643652)) ;
#35325=CARTESIAN_POINT('Ctrl Pts',(-1.44907797800853,22.0867372649376,-18.4559598953733)) ;
#35326=CARTESIAN_POINT('Ctrl Pts',(-1.8929733966678,22.0531291368785,-18.4457992263815)) ;
#35327=CARTESIAN_POINT('Ctrl Pts',(-2.33548041515253,22.0061665515132,-18.4356385573896)) ;
#35328=CARTESIAN_POINT('Ctrl Pts',(-2.77794173212602,21.9592088163786,-18.4254789377775)) ;
#35329=CARTESIAN_POINT('Ctrl Pts',(-3.21901470712191,21.8988994031436,-18.4153193181654)) ;
#35330=CARTESIAN_POINT('Ctrl Pts',(-3.65788322850045,21.8253459388197,-18.4051596985533)) ;
#35331=CARTESIAN_POINT('Ctrl Pts',(-4.09672540761267,21.7517968894057,-18.3950006887535)) ;
#35332=CARTESIAN_POINT('Ctrl Pts',(-4.53336317109265,21.6650054150248,-18.3848416789537)) ;
#35333=CARTESIAN_POINT('Ctrl Pts',(-4.96698884890711,21.5651305777946,-18.3746826691539)) ;
#35334=CARTESIAN_POINT('Ctrl Pts',(-5.42117256714812,21.4605207097616,-18.364042024283)) ;
#35335=CARTESIAN_POINT('Ctrl Pts',(-5.87205145844143,21.3415571265267,-18.3534013794121)) ;
#35336=CARTESIAN_POINT('Ctrl Pts',(-6.31871123447953,21.2084823454617,-18.3427607345412)) ;
#35337=CARTESIAN_POINT('Ctrl Pts',(-6.74519466056983,21.0814187691124,-18.3326007449388)) ;
#35338=CARTESIAN_POINT('Ctrl Pts',(-7.16783141749581,20.9414905278016,-18.3224407553364)) ;
#35339=CARTESIAN_POINT('Ctrl Pts',(-7.58584107653467,20.7889598158268,-18.312280765734)) ;
#35340=CARTESIAN_POINT('Ctrl Pts',(-8.00386942639121,20.6364222836178,-18.3021203218394)) ;
#35341=CARTESIAN_POINT('Ctrl Pts',(-8.41727005014962,20.4712812357829,-18.2919598779449)) ;
#35342=CARTESIAN_POINT('Ctrl Pts',(-8.82528083322448,20.2938476705927,-18.2817994340503)) ;
#35343=CARTESIAN_POINT('Ctrl Pts',(-9.2333594473503,20.1163846073949,-18.2716373010005)) ;
#35344=CARTESIAN_POINT('Ctrl Pts',(-9.63604621986356,19.9266250350328,-18.2614751679506)) ;
#35345=CARTESIAN_POINT('Ctrl Pts',(-10.0326002557977,19.7249275580385,-18.2513130349007)) ;
#35346=CARTESIAN_POINT('Ctrl Pts',(-10.088768307615,19.6963590571215,-18.2498736668348)) ;
#35347=CARTESIAN_POINT('Ctrl Pts',(-10.1448133629315,19.6675511343935,-18.2484342987689)) ;
#35348=CARTESIAN_POINT('Ctrl Pts',(-10.2007333551877,19.6385048839992,-18.246994930703)) ;
#35349=CARTESIAN_POINT('Ctrl Pts',(-10.6061197131374,19.427937014006,-18.2365603767191)) ;
#35350=CARTESIAN_POINT('Ctrl Pts',(-11.0050361639793,19.204785476768,-18.2261258227352)) ;
#35351=CARTESIAN_POINT('Ctrl Pts',(-11.3967005232772,18.9694768574474,-18.2156912687513)) ;
#35352=CARTESIAN_POINT('Ctrl Pts',(-11.7781177315545,18.7403246393959,-18.2055297149727)) ;
#35353=CARTESIAN_POINT('Ctrl Pts',(-12.1526572685521,18.4996434734602,-18.1953681611942)) ;
#35354=CARTESIAN_POINT('Ctrl Pts',(-12.519623122867,18.2478730794543,-18.1852066074156)) ;
#35355=CARTESIAN_POINT('Ctrl Pts',(-12.8865513804556,17.9961284800625,-18.1750460947179)) ;
#35356=CARTESIAN_POINT('Ctrl Pts',(-13.2459073161222,17.7332970517887,-18.1648855820203)) ;
#35357=CARTESIAN_POINT('Ctrl Pts',(-13.5970241052032,17.4598616989088,-18.1547250693226)) ;
#35358=CARTESIAN_POINT('Ctrl Pts',(-13.9481200466894,17.1864425812806,-18.1445651599065)) ;
#35359=CARTESIAN_POINT('Ctrl Pts',(-14.290977637916,16.9024209378865,-18.1344052504903)) ;
#35360=CARTESIAN_POINT('Ctrl Pts',(-14.6249619430466,16.6083209032984,-18.1242453410741)) ;
#35361=CARTESIAN_POINT('Ctrl Pts',(-14.9747273472437,16.3003243421072,-18.1136053655754)) ;
#35362=CARTESIAN_POINT('Ctrl Pts',(-15.314760603478,15.9812742923543,-18.1029653900766)) ;
#35363=CARTESIAN_POINT('Ctrl Pts',(-15.6443729734733,15.6518187227351,-18.0923254145779)) ;
#35364=CARTESIAN_POINT('Ctrl Pts',(-15.9591441257327,15.3371973107145,-18.0821645175588)) ;
#35365=CARTESIAN_POINT('Ctrl Pts',(-16.2644118172505,15.0130867972284,-18.0720036205397)) ;
#35366=CARTESIAN_POINT('Ctrl Pts',(-16.559614118049,14.6800890775162,-18.0618427235205)) ;
#35367=CARTESIAN_POINT('Ctrl Pts',(-16.8548296358653,14.3470764485816,-18.0516813715702)) ;
#35368=CARTESIAN_POINT('Ctrl Pts',(-17.1399787121037,14.0051759916967,-18.0415200196198)) ;
#35369=CARTESIAN_POINT('Ctrl Pts',(-17.4145387367278,13.6550238245675,-18.0313586676694)) ;
#35370=CARTESIAN_POINT('Ctrl Pts',(-17.6891443441964,13.3048135246792,-18.0211956287169)) ;
#35371=CARTESIAN_POINT('Ctrl Pts',(-17.9531572457499,12.9463489577964,-18.0110325897645)) ;
#35372=CARTESIAN_POINT('Ctrl Pts',(-18.2060961372532,12.5802980292039,-18.0008695508121)) ;
#35373=CARTESIAN_POINT('Ctrl Pts',(-18.2418015883866,12.5286254158486,-17.9994349122378)) ;
#35374=CARTESIAN_POINT('Ctrl Pts',(-18.2772864393892,12.4768016790243,-17.9980002736635)) ;
#35375=CARTESIAN_POINT('Ctrl Pts',(-18.3125494054851,12.4248287446615,-17.9965656350893)) ;
#35376=CARTESIAN_POINT('Ctrl Pts',(-18.5690274689917,12.046814101087,-17.9861310811053)) ;
#35377=CARTESIAN_POINT('Ctrl Pts',(-18.8138301175145,11.6608062419235,-17.9756965271214)) ;
#35378=CARTESIAN_POINT('Ctrl Pts',(-19.0464720509751,11.2675524171811,-17.9652619731375)) ;
#35379=CARTESIAN_POINT('Ctrl Pts',(-19.2730114206556,10.8846142587141,-17.9551011339146)) ;
#35380=CARTESIAN_POINT('Ctrl Pts',(-19.4880197714198,10.4948056214014,-17.9449402946916)) ;
#35381=CARTESIAN_POINT('Ctrl Pts',(-19.6910939541567,10.0988441888701,-17.9347794554686)) ;
#35382=CARTESIAN_POINT('Ctrl Pts',(-19.8941472116954,9.70292355705174,-17.9246196632403)) ;
#35383=CARTESIAN_POINT('Ctrl Pts',(-20.085268652827,9.30085160061508,-17.9144598710119)) ;
#35384=CARTESIAN_POINT('Ctrl Pts',(-20.2641013384807,8.89337011521972,-17.9043000787835)) ;
#35385=CARTESIAN_POINT('Ctrl Pts',(-20.4429233261946,8.48591300575116,-17.8941408943235)) ;
#35386=CARTESIAN_POINT('Ctrl Pts',(-20.6094579348632,8.07304722399147,-17.8839817098635)) ;
#35387=CARTESIAN_POINT('Ctrl Pts',(-20.763395883629,7.655535673106,-17.8738225254035)) ;
#35388=CARTESIAN_POINT('Ctrl Pts',(-20.9246272438241,7.21824288217204,-17.8631820099095)) ;
#35389=CARTESIAN_POINT('Ctrl Pts',(-21.0720395086345,6.77585376433237,-17.8525414944155)) ;
#35390=CARTESIAN_POINT('Ctrl Pts',(-21.2053348525127,6.3292660597663,-17.8419009789215)) ;
#35391=CARTESIAN_POINT('Ctrl Pts',(-21.3326128073726,5.90283878894843,-17.8317408111967)) ;
#35392=CARTESIAN_POINT('Ctrl Pts',(-21.4470199752717,5.47258380592941,-17.821580643472)) ;
#35393=CARTESIAN_POINT('Ctrl Pts',(-21.5483482822266,5.03929770606615,-17.8114204757472)) ;
#35394=CARTESIAN_POINT('Ctrl Pts',(-21.6496811278202,4.60599219870317,-17.8012598529341)) ;
#35395=CARTESIAN_POINT('Ctrl Pts',(-21.7379338920429,4.16965552728269,-17.791099230121)) ;
#35396=CARTESIAN_POINT('Ctrl Pts',(-21.8129493646537,3.73109569396881,-17.7809386073079)) ;
#35397=CARTESIAN_POINT('Ctrl Pts',(-21.8879773120214,3.29246293000324,-17.770776294826)) ;
#35398=CARTESIAN_POINT('Ctrl Pts',(-21.9497635306201,2.85160649169889,-17.7606139823442)) ;
#35399=CARTESIAN_POINT('Ctrl Pts',(-21.9982022631477,2.40934270126547,-17.7504516698623)) ;
#35400=CARTESIAN_POINT('Ctrl Pts',(-22.005058613831,2.34674164868904,-17.7490132264)) ;
#35401=CARTESIAN_POINT('Ctrl Pts',(-22.0116476255083,2.28411240874201,-17.7475747829376)) ;
#35402=CARTESIAN_POINT('Ctrl Pts',(-22.017969082177,2.22145730519318,-17.7461363394753)) ;
#35403=CARTESIAN_POINT('Ctrl Pts',(-22.0638253028726,1.76695347694492,-17.7357017854914)) ;
#35404=CARTESIAN_POINT('Ctrl Pts',(-22.0956095704889,1.31097053574373,-17.7252672315075)) ;
#35405=CARTESIAN_POINT('Ctrl Pts',(-22.1132503614142,0.854396579998724,
-17.7148326775236)) ;
#35406=CARTESIAN_POINT('Ctrl Pts',(-22.1304291012946,0.409781298569257,
-17.7046714274177)) ;
#35407=CARTESIAN_POINT('Ctrl Pts',(-22.1341957795088,-0.0353941912238496,
-17.6945101773119)) ;
#35408=CARTESIAN_POINT('Ctrl Pts',(-22.1245370679452,-0.480306768243701,
-17.684348927206)) ;
#35409=CARTESIAN_POINT('Ctrl Pts',(-22.1148793486058,-0.925173640091113,
-17.6741887209494)) ;
#35410=CARTESIAN_POINT('Ctrl Pts',(-22.0917989993386,-1.36977742371452,
-17.6640285146929)) ;
#35411=CARTESIAN_POINT('Ctrl Pts',(-22.0553348089614,-1.81329576382731,
-17.6538683084363)) ;
#35412=CARTESIAN_POINT('Ctrl Pts',(-22.0188727914712,-2.25678767485438,
-17.6437087076225)) ;
#35413=CARTESIAN_POINT('Ctrl Pts',(-21.969028545034,-2.69919404289627,-17.6335491068087)) ;
#35414=CARTESIAN_POINT('Ctrl Pts',(-21.9058928204378,-3.13969660986405,
-17.6233895059949)) ;
#35415=CARTESIAN_POINT('Ctrl Pts',(-21.8397704327511,-3.60103734359781,
-17.6127493008171)) ;
#35416=CARTESIAN_POINT('Ctrl Pts',(-21.7590688864884,-4.06028956270628,
-17.6021090956393)) ;
#35417=CARTESIAN_POINT('Ctrl Pts',(-21.6639530976092,-4.51652202995732,
-17.5914688904615)) ;
#35418=CARTESIAN_POINT('Ctrl Pts',(-21.5731247600813,-4.9521893047067,-17.5813083045205)) ;
#35419=CARTESIAN_POINT('Ctrl Pts',(-21.4691528313875,-5.38510277625743,
-17.5711477185795)) ;
#35420=CARTESIAN_POINT('Ctrl Pts',(-21.3522331111678,-5.81446267756954,
-17.5609871326385)) ;
#35421=CARTESIAN_POINT('Ctrl Pts',(-21.2353081576933,-6.24384179676661,
-17.5508260919159)) ;
#35422=CARTESIAN_POINT('Ctrl Pts',(-21.1054343173727,-6.66966680711632,
-17.5406650511934)) ;
#35423=CARTESIAN_POINT('Ctrl Pts',(-20.9628575586059,-7.09115209540037,
-17.5305040104708)) ;
#35424=CARTESIAN_POINT('Ctrl Pts',(-20.8202571165975,-7.51270739606229,
-17.5203412819108)) ;
#35425=CARTESIAN_POINT('Ctrl Pts',(-20.6649496135383,-7.9299213168805,-17.5101785533509)) ;
#35426=CARTESIAN_POINT('Ctrl Pts',(-20.4972302370595,-8.34202539384011,
-17.5000158247909)) ;
#35427=CARTESIAN_POINT('Ctrl Pts',(-20.4735270866502,-8.40026651734974,
-17.4985795644811)) ;
#35428=CARTESIAN_POINT('Ctrl Pts',(-20.4495761114447,-8.45840561310341,
-17.4971433041712)) ;
#35429=CARTESIAN_POINT('Ctrl Pts',(-20.4253782222638,-8.51644054402846,
-17.4957070438614)) ;
#35430=CARTESIAN_POINT('Ctrl Pts',(-20.2495784878933,-8.93806928050909,
-17.4852724898775)) ;
#35431=CARTESIAN_POINT('Ctrl Pts',(-20.060696399042,-9.35430734868467,-17.4748379358936)) ;
#35432=CARTESIAN_POINT('Ctrl Pts',(-19.859091365861,-9.76433946485292,-17.4644033819097)) ;
#35433=CARTESIAN_POINT('Ctrl Pts',(-19.6627703438885,-10.1636247545978,
-17.4542423146505)) ;
#35434=CARTESIAN_POINT('Ctrl Pts',(-19.4543848809506,-10.5570250251441,
-17.4440812473913)) ;
#35435=CARTESIAN_POINT('Ctrl Pts',(-19.2343146647519,-10.9438098685882,
-17.433920180132)) ;
#35436=CARTESIAN_POINT('Ctrl Pts',(-19.0142670842641,-11.3305549285941,
-17.4237601580074)) ;
#35437=CARTESIAN_POINT('Ctrl Pts',(-18.7825372646835,-11.7106857212213,
-17.4136001358827)) ;
#35438=CARTESIAN_POINT('Ctrl Pts',(-18.5395503765572,-12.0834972957996,
-17.403440113758)) ;
#35439=CARTESIAN_POINT('Ctrl Pts',(-18.2965779902041,-12.4562866204988,
-17.3932806979966)) ;
#35440=CARTESIAN_POINT('Ctrl Pts',(-18.0423500028385,-12.8217574075939,
-17.3831212822352)) ;
#35441=CARTESIAN_POINT('Ctrl Pts',(-17.777335347269,-13.1792330206746,-17.3729618664738)) ;
#35442=CARTESIAN_POINT('Ctrl Pts',(-17.4997754018268,-13.5536308495433,
-17.3623215232883)) ;
#35443=CARTESIAN_POINT('Ctrl Pts',(-17.2103831657475,-13.9192581433289,
-17.3516811801028)) ;
#35444=CARTESIAN_POINT('Ctrl Pts',(-16.9097465941923,-14.2753740820583,
-17.3410408369173)) ;
#35445=CARTESIAN_POINT('Ctrl Pts',(-16.6226705222947,-14.6154270712928,
-17.3308804365723)) ;
#35446=CARTESIAN_POINT('Ctrl Pts',(-16.325342090823,-14.9468074772167,-17.3207200362273)) ;
#35447=CARTESIAN_POINT('Ctrl Pts',(-16.0183138511908,-15.2689048863122,
-17.3105596358824)) ;
#35448=CARTESIAN_POINT('Ctrl Pts',(-15.7112718618294,-15.5910167199836,
-17.3003987805214)) ;
#35449=CARTESIAN_POINT('Ctrl Pts',(-15.3945293564791,-15.9038445617162,
-17.2902379251605)) ;
#35450=CARTESIAN_POINT('Ctrl Pts',(-15.0686762885948,-16.2068143067057,
-17.2800770697995)) ;
#35451=CARTESIAN_POINT('Ctrl Pts',(-14.7427690622244,-16.5098344068532,
-17.2699145256512)) ;
#35452=CARTESIAN_POINT('Ctrl Pts',(-14.4077484158269,-16.8029929801262,
-17.2597519815029)) ;
#35453=CARTESIAN_POINT('Ctrl Pts',(-14.064239445091,-17.0857544139452,-17.2495894373546)) ;
#35454=CARTESIAN_POINT('Ctrl Pts',(-14.0156589628267,-17.1257437242425,
-17.2481522076522)) ;
#35455=CARTESIAN_POINT('Ctrl Pts',(-13.9669087616435,-17.1655251488869,
-17.2467149779499)) ;
#35456=CARTESIAN_POINT('Ctrl Pts',(-13.9179906627924,-17.205097238113,-17.2452777482476)) ;
#35457=CARTESIAN_POINT('Ctrl Pts',(-13.562836199713,-17.4923979393284,-17.2348431942637)) ;
#35458=CARTESIAN_POINT('Ctrl Pts',(-13.1987368800248,-17.7687352045356,
-17.2244086402798)) ;
#35459=CARTESIAN_POINT('Ctrl Pts',(-12.8263965789861,-18.0335627611705,
-17.2139740862959)) ;
#35460=CARTESIAN_POINT('Ctrl Pts',(-12.4638131708609,-18.2914507141593,
-17.2038129618213)) ;
#35461=CARTESIAN_POINT('Ctrl Pts',(-12.0934153512721,-18.5384243082068,
-17.1936518373467)) ;
#35462=CARTESIAN_POINT('Ctrl Pts',(-11.7158844814942,-18.7740215691466,
-17.1834907128721)) ;
#35463=CARTESIAN_POINT('Ctrl Pts',(-11.338392430653,-19.0095946052194,-17.173330633197)) ;
#35464=CARTESIAN_POINT('Ctrl Pts',(-10.9537689893333,-19.2337935232605,
-17.1631705535219)) ;
#35465=CARTESIAN_POINT('Ctrl Pts',(-10.5627234232182,-19.446200373006,-17.1530104738468)) ;
#35466=CARTESIAN_POINT('Ctrl Pts',(-10.1717011865675,-19.6585945507294,
-17.1428510003139)) ;
#35467=CARTESIAN_POINT('Ctrl Pts',(-9.77425779222756,-19.8591979561205,
-17.132691526781)) ;
#35468=CARTESIAN_POINT('Ctrl Pts',(-9.37112753809439,-20.0476383578533,
-17.1225320532481)) ;
#35469=CARTESIAN_POINT('Ctrl Pts',(-8.9489179767631,-20.2449972475346,-17.1118917531969)) ;
#35470=CARTESIAN_POINT('Ctrl Pts',(-8.52047057261104,-20.4290140579446,
-17.1012514531457)) ;
#35471=CARTESIAN_POINT('Ctrl Pts',(-8.0866548242917,-20.5993167074847,-17.0906111530945)) ;
#35472=CARTESIAN_POINT('Ctrl Pts',(-7.67240271472477,-20.7619392773433,
-17.0804506949744)) ;
#35473=CARTESIAN_POINT('Ctrl Pts',(-7.25325591364203,-20.912057024724,-17.0702902368543)) ;
#35474=CARTESIAN_POINT('Ctrl Pts',(-6.8299907847078,-21.0493957381989,-17.0601297787342)) ;
#35475=CARTESIAN_POINT('Ctrl Pts',(-6.40670670611673,-21.186740600353,-17.0499688657286)) ;
#35476=CARTESIAN_POINT('Ctrl Pts',(-5.97930415032894,-21.311305216929,-17.0398079527229)) ;
#35477=CARTESIAN_POINT('Ctrl Pts',(-5.54857511661993,-21.4228651033826,
-17.0296470397173)) ;
#35478=CARTESIAN_POINT('Ctrl Pts',(-5.1177745098352,-21.53444352744,-17.0194844383003)) ;
#35479=CARTESIAN_POINT('Ctrl Pts',(-4.6836465428587,-21.6330128459855,-17.0093218368833)) ;
#35480=CARTESIAN_POINT('Ctrl Pts',(-4.24699582430295,-21.7183991475167,
-16.9991592354663)) ;
#35481=CARTESIAN_POINT('Ctrl Pts',(-4.18525617241255,-21.730472230896,-16.9977223078554)) ;
#35482=CARTESIAN_POINT('Ctrl Pts',(-4.12346610193498,-21.7422818405832,
-16.9962853802446)) ;
#35483=CARTESIAN_POINT('Ctrl Pts',(-4.06162790298059,-21.7538275675852,
-16.9948484526338)) ;
#35484=CARTESIAN_POINT('Ctrl Pts',(-3.61186926570409,-21.8378013981717,
-16.984397459315)) ;
#35485=CARTESIAN_POINT('Ctrl Pts',(-3.15947745055909,-21.9078281300336,
-16.9739464659962)) ;
#35486=CARTESIAN_POINT('Ctrl Pts',(-2.70531145384119,-21.9637684608133,
-16.9634954726774)) ;
#35487=CARTESIAN_POINT('Ctrl Pts',(-2.25124847500317,-22.0196961027208,
-16.9530468499438)) ;
#35488=CARTESIAN_POINT('Ctrl Pts',(-1.7954123174551,-22.0615437046833,-16.9425982272102)) ;
#35489=CARTESIAN_POINT('Ctrl Pts',(-1.33866864577018,-22.0892236468223,
-16.9321496044766)) ;
#35490=CARTESIAN_POINT('Ctrl Pts',(-0.893168431085587,-22.1162222040653,
-16.9219581908686)) ;
#35491=CARTESIAN_POINT('Ctrl Pts',(-0.44680503136645,-22.1297422163973,
-16.9117667772605)) ;
#35492=CARTESIAN_POINT('Ctrl Pts',(-0.000385679535181172,-22.1297499966392,
-16.9015753636525)) ;
#35493=CARTESIAN_POINT('Ctrl Pts',(-0.000394050632519626,-22.1297499964917,
-16.4359246717926)) ;
#35494=CARTESIAN_POINT('Ctrl Pts',(-0.458270040802388,-22.12974184338,-16.4463776769714)) ;
#35495=CARTESIAN_POINT('Ctrl Pts',(-0.91608658402974,-22.1155188134193,
-16.4568306821502)) ;
#35496=CARTESIAN_POINT('Ctrl Pts',(-1.37297316201532,-22.0871179595457,
-16.467283687329)) ;
#35497=CARTESIAN_POINT('Ctrl Pts',(-1.82999981297473,-22.0587083984956,
-16.4777398972058)) ;
#35498=CARTESIAN_POINT('Ctrl Pts',(-2.28609572932389,-22.016112336254,-16.4881961070826)) ;
#35499=CARTESIAN_POINT('Ctrl Pts',(-2.74039394844152,-21.9594188463594,
-16.4986523169594)) ;
#35500=CARTESIAN_POINT('Ctrl Pts',(-3.17025376482808,-21.9057751116256,
-16.5085460481444)) ;
#35501=CARTESIAN_POINT('Ctrl Pts',(-3.59850398566261,-21.8395102898116,
-16.5184397793293)) ;
#35502=CARTESIAN_POINT('Ctrl Pts',(-4.02441617112775,-21.7607423941387,
-16.5283335105142)) ;
#35503=CARTESIAN_POINT('Ctrl Pts',(-4.47361007063524,-21.6776687948833,
-16.5387680644981)) ;
#35504=CARTESIAN_POINT('Ctrl Pts',(-4.92028896367183,-21.5806710394323,
-16.5492026184821)) ;
#35505=CARTESIAN_POINT('Ctrl Pts',(-5.36358016922639,-21.4699288035797,
-16.559637172466)) ;
#35506=CARTESIAN_POINT('Ctrl Pts',(-5.79525488918246,-21.3620885778997,
-16.5697982880316)) ;
#35507=CARTESIAN_POINT('Ctrl Pts',(-6.22371696461821,-21.2412150662447,
-16.5799594035972)) ;
#35508=CARTESIAN_POINT('Ctrl Pts',(-6.64817240571008,-21.1075256419708,
-16.5901205191629)) ;
#35509=CARTESIAN_POINT('Ctrl Pts',(-7.07258420181503,-20.9738499644242,
-16.6002805899033)) ;
#35510=CARTESIAN_POINT('Ctrl Pts',(-7.49298996764377,-20.827361075493,-16.6104406606437)) ;
#35511=CARTESIAN_POINT('Ctrl Pts',(-7.90861102244079,-20.6683261721463,
-16.6206007313841)) ;
#35512=CARTESIAN_POINT('Ctrl Pts',(-8.32420728126773,-20.5093007568288,
-16.6307601959742)) ;
#35513=CARTESIAN_POINT('Ctrl Pts',(-8.73501918503367,-20.3377309044873,
-16.6409196605643)) ;
#35514=CARTESIAN_POINT('Ctrl Pts',(-9.14028651728225,-20.1539325553225,
-16.6510791251545)) ;
#35515=CARTESIAN_POINT('Ctrl Pts',(-9.56473494089009,-19.9614351262012,
-16.6617194319023)) ;
#35516=CARTESIAN_POINT('Ctrl Pts',(-9.98310109258281,-19.7555239619668,
-16.6723597386501)) ;
#35517=CARTESIAN_POINT('Ctrl Pts',(-10.3945369683939,-19.5366178310165,
-16.6830000453979)) ;
#35518=CARTESIAN_POINT('Ctrl Pts',(-10.7874178722743,-19.3275839483412,
-16.6931604946402)) ;
#35519=CARTESIAN_POINT('Ctrl Pts',(-11.1739794721254,-19.1067012528695,
-16.7033209438824)) ;
#35520=CARTESIAN_POINT('Ctrl Pts',(-11.5535086814804,-18.8743813728942,
-16.7134813931247)) ;
#35521=CARTESIAN_POINT('Ctrl Pts',(-11.9330548840379,-18.6420510909297,
-16.7236422972953)) ;
#35522=CARTESIAN_POINT('Ctrl Pts',(-12.3055678724736,-18.3982827231497,
-16.7338032014659)) ;
#35523=CARTESIAN_POINT('Ctrl Pts',(-12.6703621789704,-18.1435321069581,
-16.7439641056365)) ;
#35524=CARTESIAN_POINT('Ctrl Pts',(-13.0352171056192,-17.8887391572628,
-16.7541266983081)) ;
#35525=CARTESIAN_POINT('Ctrl Pts',(-13.3923505992489,-17.6229604440359,
-16.7642892909797)) ;
#35526=CARTESIAN_POINT('Ctrl Pts',(-13.7411074210875,-17.3466942644596,
-16.7744518836513)) ;
#35527=CARTESIAN_POINT('Ctrl Pts',(-13.7904210713462,-17.3076306737142,
-16.7758888578102)) ;
#35528=CARTESIAN_POINT('Ctrl Pts',(-13.8395672951608,-17.2683574687375,
-16.7773258319691)) ;
#35529=CARTESIAN_POINT('Ctrl Pts',(-13.8885442927298,-17.228876123862,-16.778762806128)) ;
#35530=CARTESIAN_POINT('Ctrl Pts',(-14.2441896061347,-16.9421832686685,
-16.7891973601119)) ;
#35531=CARTESIAN_POINT('Ctrl Pts',(-14.5910008705382,-16.6444374970597,
-16.7996319140958)) ;
#35532=CARTESIAN_POINT('Ctrl Pts',(-14.9282958429325,-16.3362118708219,
-16.8100664680797)) ;
#35533=CARTESIAN_POINT('Ctrl Pts',(-15.2567520107339,-16.0360632878367,
-16.8202275848908)) ;
#35534=CARTESIAN_POINT('Ctrl Pts',(-15.5761840758257,-15.7259772360805,
-16.8303887017018)) ;
#35535=CARTESIAN_POINT('Ctrl Pts',(-15.8859969457872,-15.406522518107,-16.8405498185128)) ;
#35536=CARTESIAN_POINT('Ctrl Pts',(-16.1957779590629,-15.0871006482479,
-16.8507098905012)) ;
#35537=CARTESIAN_POINT('Ctrl Pts',(-16.4959415931659,-14.7583122011488,
-16.8608699624896)) ;
#35538=CARTESIAN_POINT('Ctrl Pts',(-16.7859299164886,-14.4207625284252,
-16.8710300344779)) ;
#35539=CARTESIAN_POINT('Ctrl Pts',(-17.075900939101,-14.0832329939231,-16.8811895003162)) ;
#35540=CARTESIAN_POINT('Ctrl Pts',(-17.3556977142044,-13.7369434521286,
-16.8913489661544)) ;
#35541=CARTESIAN_POINT('Ctrl Pts',(-17.6248017328512,-13.3825333528516,
-16.9015084319926)) ;
#35542=CARTESIAN_POINT('Ctrl Pts',(-17.9066422448772,-13.0113492867431,
-16.912148737805)) ;
#35543=CARTESIAN_POINT('Ctrl Pts',(-18.1767533565653,-12.6312577288267,
-16.9227890436175)) ;
#35544=CARTESIAN_POINT('Ctrl Pts',(-18.4345882334818,-12.24303033258,-16.9334293494299)) ;
#35545=CARTESIAN_POINT('Ctrl Pts',(-18.6807953016649,-11.8723111724674,
-16.9435897999089)) ;
#35546=CARTESIAN_POINT('Ctrl Pts',(-18.9158086482927,-11.4941738823983,
-16.9537502503878)) ;
#35547=CARTESIAN_POINT('Ctrl Pts',(-19.1391967285628,-11.1093196752938,
-16.9639107008667)) ;
#35548=CARTESIAN_POINT('Ctrl Pts',(-19.3625948107562,-10.7244482368212,
-16.9740716062672)) ;
#35549=CARTESIAN_POINT('Ctrl Pts',(-19.5743664734542,-10.3328594801228,
-16.9842325116676)) ;
#35550=CARTESIAN_POINT('Ctrl Pts',(-19.7741254912944,-9.93528037435493,
-16.9943934170681)) ;
#35551=CARTESIAN_POINT('Ctrl Pts',(-19.973917704069,-9.53763520091962,-17.0045560109559)) ;
#35552=CARTESIAN_POINT('Ctrl Pts',(-20.161693180309,-9.13399789449304,-17.0147186048438)) ;
#35553=CARTESIAN_POINT('Ctrl Pts',(-20.3371124785335,-8.72511840022681,
-17.0248811987317)) ;
#35554=CARTESIAN_POINT('Ctrl Pts',(-20.361916368469,-8.66730376936636,-17.0263181664017)) ;
#35555=CARTESIAN_POINT('Ctrl Pts',(-20.3864732954977,-8.6093843636827,-17.0277551340718)) ;
#35556=CARTESIAN_POINT('Ctrl Pts',(-20.4107823774842,-8.55136233599528,
-17.0291921017419)) ;
#35557=CARTESIAN_POINT('Ctrl Pts',(-20.587303000441,-8.13003484702398,-17.0396266557258)) ;
#35558=CARTESIAN_POINT('Ctrl Pts',(-20.7507961995129,-7.70318525587862,
-17.0500612097097)) ;
#35559=CARTESIAN_POINT('Ctrl Pts',(-20.9009343320342,-7.27164211925304,
-17.0604957636936)) ;
#35560=CARTESIAN_POINT('Ctrl Pts',(-21.0471380495211,-6.85140770064717,
-17.070656877044)) ;
#35561=CARTESIAN_POINT('Ctrl Pts',(-21.180677613898,-6.42672281012036,-17.0808179903944)) ;
#35562=CARTESIAN_POINT('Ctrl Pts',(-21.3013000227658,-5.99837081236371,
-17.0909791037448)) ;
#35563=CARTESIAN_POINT('Ctrl Pts',(-21.4219100285112,-5.57006286033871,
-17.1011391722683)) ;
#35564=CARTESIAN_POINT('Ctrl Pts',(-21.5296054696472,-5.13808877515966,
-17.1112992407919)) ;
#35565=CARTESIAN_POINT('Ctrl Pts',(-21.6241834146182,-4.70324640152428,
-17.1214593093154)) ;
#35566=CARTESIAN_POINT('Ctrl Pts',(-21.718755717089,-4.26842997049313,-17.1316187716914)) ;
#35567=CARTESIAN_POINT('Ctrl Pts',(-21.8002120381128,-3.8307458171197,-17.1417782340674)) ;
#35568=CARTESIAN_POINT('Ctrl Pts',(-21.8684003411913,-3.3910030344847,-17.1519376964434)) ;
#35569=CARTESIAN_POINT('Ctrl Pts',(-21.9398159877889,-2.93044728312142,
-17.1625780048527)) ;
#35570=CARTESIAN_POINT('Ctrl Pts',(-21.9966774498719,-2.46763361794661,
-17.1732183132621)) ;
#35571=CARTESIAN_POINT('Ctrl Pts',(-22.0388706425406,-2.00350090188735,
-17.1838586216715)) ;
#35572=CARTESIAN_POINT('Ctrl Pts',(-22.0791609878698,-1.56029984916074,
-17.1940190687272)) ;
#35573=CARTESIAN_POINT('Ctrl Pts',(-22.1060766607646,-1.1158963185534,-17.204179515783)) ;
#35574=CARTESIAN_POINT('Ctrl Pts',(-22.119571497574,-0.671112379720387,
-17.2143399628387)) ;
#35575=CARTESIAN_POINT('Ctrl Pts',(-22.1330669386263,-0.226308525301396,
-17.2245008648373)) ;
#35576=CARTESIAN_POINT('Ctrl Pts',(-22.133140338349,0.218875541893517,-17.2346617668358)) ;
#35577=CARTESIAN_POINT('Ctrl Pts',(-22.1197976484675,0.663616646378586,
-17.2448226688344)) ;
#35578=CARTESIAN_POINT('Ctrl Pts',(-22.1064527413112,1.10843165749302,-17.2549852593614)) ;
#35579=CARTESIAN_POINT('Ctrl Pts',(-22.0796872966979,1.55280332939547,-17.2651478498885)) ;
#35580=CARTESIAN_POINT('Ctrl Pts',(-22.0395593478398,1.99591052293076,-17.2753104404155)) ;
#35581=CARTESIAN_POINT('Ctrl Pts',(-22.0338852742473,2.05856567718201,-17.2767474260622)) ;
#35582=CARTESIAN_POINT('Ctrl Pts',(-22.0279441178173,2.12119555697544,-17.2781844117089)) ;
#35583=CARTESIAN_POINT('Ctrl Pts',(-22.0217361263272,2.18379784891302,-17.2796213973557)) ;
#35584=CARTESIAN_POINT('Ctrl Pts',(-21.9766573028303,2.63837928209217,-17.2900559513396)) ;
#35585=CARTESIAN_POINT('Ctrl Pts',(-21.9174923657914,3.09162326122403,-17.3004905053235)) ;
#35586=CARTESIAN_POINT('Ctrl Pts',(-21.8443471114585,3.54264510452476,-17.3109250593074)) ;
#35587=CARTESIAN_POINT('Ctrl Pts',(-21.7731186004249,3.98184809363163,-17.3210861798114)) ;
#35588=CARTESIAN_POINT('Ctrl Pts',(-21.688633135833,4.41894367839406,-17.3312473003155)) ;
#35589=CARTESIAN_POINT('Ctrl Pts',(-21.5910406832882,4.8531224253148,-17.3414084208195)) ;
#35590=CARTESIAN_POINT('Ctrl Pts',(-21.493458265736,5.2872565275897,-17.3515684965013)) ;
#35591=CARTESIAN_POINT('Ctrl Pts',(-21.3827716026278,5.71847416723885,-17.361728572183)) ;
#35592=CARTESIAN_POINT('Ctrl Pts',(-21.2591815922954,6.1459769840366,-17.3718886478648)) ;
#35593=CARTESIAN_POINT('Ctrl Pts',(-21.1355989554263,6.57345429572838,-17.3820481173896)) ;
#35594=CARTESIAN_POINT('Ctrl Pts',(-20.9991145730536,6.99721700689574,-17.3922075869144)) ;
#35595=CARTESIAN_POINT('Ctrl Pts',(-20.8499794644913,7.41648106535637,-17.4023670564392)) ;
#35596=CARTESIAN_POINT('Ctrl Pts',(-20.6937859992954,7.85558830679939,-17.4130073594834)) ;
#35597=CARTESIAN_POINT('Ctrl Pts',(-20.5237156435815,8.28976057934957,-17.4236476625276)) ;
#35598=CARTESIAN_POINT('Ctrl Pts',(-20.3401145130157,8.71811772459553,-17.4342879655718)) ;
#35599=CARTESIAN_POINT('Ctrl Pts',(-20.164793297579,9.12715711947368,-17.4444484196854)) ;
#35600=CARTESIAN_POINT('Ctrl Pts',(-19.9771346756949,9.53089399517996,-17.454608873799)) ;
#35601=CARTESIAN_POINT('Ctrl Pts',(-19.7774889727994,9.92858323192686,-17.4647693279127)) ;
#35602=CARTESIAN_POINT('Ctrl Pts',(-19.5778343315327,10.326290273685,-17.4749302369217)) ;
#35603=CARTESIAN_POINT('Ctrl Pts',(-19.3661916420715,10.7179489314522,-17.4850911459307)) ;
#35604=CARTESIAN_POINT('Ctrl Pts',(-19.14295760106,11.1028378960751,-17.4952520549397)) ;
#35605=CARTESIAN_POINT('Ctrl Pts',(-18.9196864652342,11.4877908177207,-17.5054146523876)) ;
#35606=CARTESIAN_POINT('Ctrl Pts',(-18.6848202443778,11.8659715999616,-17.5155772498355)) ;
#35607=CARTESIAN_POINT('Ctrl Pts',(-18.4388004822799,12.2366854922881,-17.5257398472834)) ;
#35608=CARTESIAN_POINT('Ctrl Pts',(-18.4040143220296,12.289102878418,-17.5271767958455)) ;
#35609=CARTESIAN_POINT('Ctrl Pts',(-18.369005242705,12.3413710274821,-17.5286137444075)) ;
#35610=CARTESIAN_POINT('Ctrl Pts',(-18.3337745623043,12.3934880223892,-17.5300506929695)) ;
#35611=CARTESIAN_POINT('Ctrl Pts',(-18.0779432498685,12.7719410938493,-17.5404852469535)) ;
#35612=CARTESIAN_POINT('Ctrl Pts',(-17.810356562303,13.1425189796053,-17.5509198009374)) ;
#35613=CARTESIAN_POINT('Ctrl Pts',(-17.5315282776837,13.5044937450937,-17.5613543549213)) ;
#35614=CARTESIAN_POINT('Ctrl Pts',(-17.2600068850294,13.8569827064104,-17.5715154640545)) ;
#35615=CARTESIAN_POINT('Ctrl Pts',(-16.9778256938762,14.2013134889568,-17.5816765731877)) ;
#35616=CARTESIAN_POINT('Ctrl Pts',(-16.6855015517371,14.5368453603069,-17.5918376823209)) ;
#35617=CARTESIAN_POINT('Ctrl Pts',(-16.3932074679945,14.8723427304013,-17.6019977466322)) ;
#35618=CARTESIAN_POINT('Ctrl Pts',(-16.0907726672864,15.1990428235145,-17.6121578109436)) ;
#35619=CARTESIAN_POINT('Ctrl Pts',(-15.7787535362038,15.516338869277,-17.6223178752549)) ;
#35620=CARTESIAN_POINT('Ctrl Pts',(-15.4667530197208,15.833615985627,-17.6324773334319)) ;
#35621=CARTESIAN_POINT('Ctrl Pts',(-15.1451694761089,16.1414900118586,-17.6426367916089)) ;
#35622=CARTESIAN_POINT('Ctrl Pts',(-14.8145965786543,16.4393905992352,-17.6527962497858)) ;
#35623=CARTESIAN_POINT('Ctrl Pts',(-14.4683774631192,16.7513910042083,-17.6634365613523)) ;
#35624=CARTESIAN_POINT('Ctrl Pts',(-14.1122978043987,17.0524510061868,-17.6740768729187)) ;
#35625=CARTESIAN_POINT('Ctrl Pts',(-13.7470806382558,17.341960932599,-17.6847171844852)) ;
#35626=CARTESIAN_POINT('Ctrl Pts',(-13.3983344431678,17.6184142174838,-17.6948776274144)) ;
#35627=CARTESIAN_POINT('Ctrl Pts',(-13.0412567961562,17.8843359100162,-17.7050380703436)) ;
#35628=CARTESIAN_POINT('Ctrl Pts',(-12.6765102147787,18.1392371349269,-17.7151985132728)) ;
#35629=CARTESIAN_POINT('Ctrl Pts',(-12.3117473003179,18.3941497741267,-17.7253594111791)) ;
#35630=CARTESIAN_POINT('Ctrl Pts',(-11.9393149548486,18.6380408301885,-17.7355203090854)) ;
#35631=CARTESIAN_POINT('Ctrl Pts',(-11.5599051650042,18.8704644256205,-17.7456812069918)) ;
#35632=CARTESIAN_POINT('Ctrl Pts',(-11.1804323228982,19.1029266463957,-17.7558437934882)) ;
#35633=CARTESIAN_POINT('Ctrl Pts',(-10.7939799152298,19.3239174788007,-17.7660063799845)) ;
#35634=CARTESIAN_POINT('Ctrl Pts',(-10.4012667501909,19.5330357357445,-17.7761689664809)) ;
#35635=CARTESIAN_POINT('Ctrl Pts',(-10.3457364271116,19.5626054201954,-17.7776059738484)) ;
#35636=CARTESIAN_POINT('Ctrl Pts',(-10.290080963963,19.5919377939813,-17.7790429812159)) ;
#35637=CARTESIAN_POINT('Ctrl Pts',(-10.234302432103,19.6210317973024,-17.7804799885833)) ;
#35638=CARTESIAN_POINT('Ctrl Pts',(-9.82927729791871,19.8322923343968,-17.7909145425673)) ;
#35639=CARTESIAN_POINT('Ctrl Pts',(-9.41765613265564,20.0310348947837,-17.8013490965512)) ;
#35640=CARTESIAN_POINT('Ctrl Pts',(-9.00023706922651,20.2168634501057,-17.8117836505351)) ;
#35641=CARTESIAN_POINT('Ctrl Pts',(-8.59375629880124,20.3978224453988,-17.8219447713703)) ;
#35642=CARTESIAN_POINT('Ctrl Pts',(-8.18177782754204,20.5665354915101,-17.8321058922055)) ;
#35643=CARTESIAN_POINT('Ctrl Pts',(-7.76506102216589,20.7226847291691,-17.8422670130407)) ;
#35644=CARTESIAN_POINT('Ctrl Pts',(-7.34838706667009,20.8788179104175,-17.8524270890349)) ;
#35645=CARTESIAN_POINT('Ctrl Pts',(-6.9269759651681,21.0223897832525,-17.8625871650291)) ;
#35646=CARTESIAN_POINT('Ctrl Pts',(-6.50160571582377,21.1531311672402,-17.8727472410233)) ;
#35647=CARTESIAN_POINT('Ctrl Pts',(-6.07626084515955,21.2838647508616,-17.8829067108413)) ;
#35648=CARTESIAN_POINT('Ctrl Pts',(-5.64695751792443,21.4017693075676,-17.8930661806593)) ;
#35649=CARTESIAN_POINT('Ctrl Pts',(-5.21448921269231,21.5066254283004,-17.9032256504773)) ;
#35650=CARTESIAN_POINT('Ctrl Pts',(-4.76155280893994,21.6164442373588,-17.9138659532873)) ;
#35651=CARTESIAN_POINT('Ctrl Pts',(-4.30514490389635,21.7119497426604,-17.9245062560973)) ;
#35652=CARTESIAN_POINT('Ctrl Pts',(-3.84619147011417,21.7929494616429,-17.9351465589073)) ;
#35653=CARTESIAN_POINT('Ctrl Pts',(-3.4079355765569,21.8702963156102,-17.9453070132638)) ;
#35654=CARTESIAN_POINT('Ctrl Pts',(-2.96735888389062,21.9344165972658,-17.9554674676203)) ;
#35655=CARTESIAN_POINT('Ctrl Pts',(-2.52527668758332,21.9851953076075,-17.9656279219769)) ;
#35656=CARTESIAN_POINT('Ctrl Pts',(-2.08317469951773,22.035976291282,-17.9757888312109)) ;
#35657=CARTESIAN_POINT('Ctrl Pts',(-1.63956730143142,22.0734144864172,-17.985949740445)) ;
#35658=CARTESIAN_POINT('Ctrl Pts',(-1.19527526488837,22.0974467326804,-17.996110649679)) ;
#35659=CARTESIAN_POINT('Ctrl Pts',(-0.750909401426862,22.121482972323,-18.0062732473265)) ;
#35660=CARTESIAN_POINT('Ctrl Pts',(-0.305858901380434,22.1321087996347,
-18.0164358449739)) ;
#35661=CARTESIAN_POINT('Ctrl Pts',(0.139053121511222,22.1293131229123,-18.0265984426213)) ;
#35662=CARTESIAN_POINT('Ctrl Pts',(0.201961750205417,22.1289178263596,-18.0280353898133)) ;
#35663=CARTESIAN_POINT('Ctrl Pts',(0.264867610527304,22.1282542823854,-18.0294723370053)) ;
#35664=CARTESIAN_POINT('Ctrl Pts',(0.327768376633555,22.1273225437191,-18.0309092841973)) ;
#35665=CARTESIAN_POINT('Ctrl Pts',(0.784529378868009,22.1205566183833,-18.0413438381812)) ;
#35666=CARTESIAN_POINT('Ctrl Pts',(1.24113991677261,22.0996420266961,-18.0517783921651)) ;
#35667=CARTESIAN_POINT('Ctrl Pts',(1.69670955080554,22.0646099390564,-18.062212946149)) ;
#35668=CARTESIAN_POINT('Ctrl Pts',(2.14034132093769,22.0304958412544,-18.0723740703957)) ;
#35669=CARTESIAN_POINT('Ctrl Pts',(2.58298580001337,21.9829946786199,-18.0825351946423)) ;
#35670=CARTESIAN_POINT('Ctrl Pts',(3.02382382315773,21.9221879507727,-18.092696318889)) ;
#35671=CARTESIAN_POINT('Ctrl Pts',(3.46461651891799,21.861387475131,-18.1028563983592)) ;
#35672=CARTESIAN_POINT('Ctrl Pts',(3.90360290244921,21.7872841983707,-18.1130164778295)) ;
#35673=CARTESIAN_POINT('Ctrl Pts',(4.3399705682238,21.700011302519,-18.1231765572997)) ;
#35674=CARTESIAN_POINT('Ctrl Pts',(4.7763122016556,21.6127436130978,-18.1333360306511)) ;
#35675=CARTESIAN_POINT('Ctrl Pts',(5.21003520441906,21.5123079192163,-18.1434955040024)) ;
#35676=CARTESIAN_POINT('Ctrl Pts',(5.64033722181922,21.3988885479284,-18.1536549773538)) ;
#35677=CARTESIAN_POINT('Ctrl Pts',(6.09100454339223,21.2801012724663,-18.1642952775586)) ;
#35678=CARTESIAN_POINT('Ctrl Pts',(6.53791902154512,21.1470718784239,-18.1749355777633)) ;
#35679=CARTESIAN_POINT('Ctrl Pts',(6.98017455454659,21.0000713867968,-18.1855758779681)) ;
#35680=CARTESIAN_POINT('Ctrl Pts',(7.40248583158888,20.8597001292037,-18.1957363359664)) ;
#35681=CARTESIAN_POINT('Ctrl Pts',(7.82054879569433,20.7065899384987,-18.2058967939648)) ;
#35682=CARTESIAN_POINT('Ctrl Pts',(8.23359155226314,20.5410273650809,-18.2160572519631)) ;
#35683=CARTESIAN_POINT('Ctrl Pts',(8.64665280167992,20.3754573790564,-18.2262181648679)) ;
#35684=CARTESIAN_POINT('Ctrl Pts',(9.0546931823239,20.1974339839893,-18.2363790777726)) ;
#35685=CARTESIAN_POINT('Ctrl Pts',(9.45696063420162,20.0072919363331,-18.2465399906774)) ;
#35686=CARTESIAN_POINT('Ctrl Pts',(9.85929493094365,19.8171182927343,-18.2567025920231)) ;
#35687=CARTESIAN_POINT('Ctrl Pts',(10.2558541746451,19.614822070914,-18.2668651933688)) ;
#35688=CARTESIAN_POINT('Ctrl Pts',(10.6459090061464,19.4007849453405,-18.2770277947145)) ;
#35689=CARTESIAN_POINT('Ctrl Pts',(10.7010603234539,19.3705214324322,-18.27846472308)) ;
#35690=CARTESIAN_POINT('Ctrl Pts',(10.7560816439118,19.3400232678949,-18.2799016514455)) ;
#35691=CARTESIAN_POINT('Ctrl Pts',(10.8109709466575,19.3092916041223,-18.281338579811)) ;
#35692=CARTESIAN_POINT('Ctrl Pts',(11.2095610269893,19.0861272402275,-18.291773133795)) ;
#35693=CARTESIAN_POINT('Ctrl Pts',(11.6012903702668,18.8505879952913,-18.3022076877789)) ;
#35694=CARTESIAN_POINT('Ctrl Pts',(11.9853904837859,18.6031247378948,-18.3126422417628)) ;
#35695=CARTESIAN_POINT('Ctrl Pts',(12.3594234447549,18.362147420687,-18.3228033091138)) ;
#35696=CARTESIAN_POINT('Ctrl Pts',(12.7262217752393,18.1098632747737,-18.3329643764648)) ;
#35697=CARTESIAN_POINT('Ctrl Pts',(13.0851036283453,17.8467335414065,-18.3431254438158)) ;
#35698=CARTESIAN_POINT('Ctrl Pts',(13.4439485754045,17.5836308673018,-18.3532854662412)) ;
#35699=CARTESIAN_POINT('Ctrl Pts',(13.794878486179,17.309684969259,-18.3634454886666)) ;
#35700=CARTESIAN_POINT('Ctrl Pts',(14.1372420373358,17.0253993386436,-18.373605511092)) ;
#35701=CARTESIAN_POINT('Ctrl Pts',(14.4795851627889,16.7411306687532,-18.3837649273618)) ;
#35702=CARTESIAN_POINT('Ctrl Pts',(14.8133627731231,16.4465236453209,-18.3939243436315)) ;
#35703=CARTESIAN_POINT('Ctrl Pts',(15.1379567085441,16.1421219718085,-18.4040837599013)) ;
#35704=CARTESIAN_POINT('Ctrl Pts',(15.4779162794496,15.8233105245892,-18.4147241028616)) ;
#35705=CARTESIAN_POINT('Ctrl Pts',(15.8078016088646,15.4937550079356,-18.4253644458219)) ;
#35706=CARTESIAN_POINT('Ctrl Pts',(16.1269444809372,15.1541247444803,-18.4360047887822)) ;
#35707=CARTESIAN_POINT('Ctrl Pts',(16.4316921460637,14.8298137889445,-18.446165190148)) ;
#35708=CARTESIAN_POINT('Ctrl Pts',(16.7266447332537,14.4963169159911,-18.4563255915139)) ;
#35709=CARTESIAN_POINT('Ctrl Pts',(17.0112594907531,14.154253268921,-18.4664859928797)) ;
#35710=CARTESIAN_POINT('Ctrl Pts',(17.2958869991246,13.8121742972422,-18.4766468494362)) ;
#35711=CARTESIAN_POINT('Ctrl Pts',(17.5701756074771,13.4615279625757,-18.4868077059926)) ;
#35712=CARTESIAN_POINT('Ctrl Pts',(17.8336229367823,13.1029663821279,-18.4969685625491)) ;
#35713=CARTESIAN_POINT('Ctrl Pts',(18.0971140586121,12.7443451984307,-18.5071311081322)) ;
#35714=CARTESIAN_POINT('Ctrl Pts',(18.34976016463,12.3778063249207,-18.5172936537154)) ;
#35715=CARTESIAN_POINT('Ctrl Pts',(18.5911011573929,12.004032356591,-18.5274561992985)) ;
#35716=CARTESIAN_POINT('Ctrl Pts',(18.6252325072704,11.9511718377786,-18.528893424674)) ;
#35717=CARTESIAN_POINT('Ctrl Pts',(18.6591378185395,11.8981666586563,-18.5303306500495)) ;
#35718=CARTESIAN_POINT('Ctrl Pts',(18.6928158607279,11.8450187952329,-18.5317678754249)) ;
#35719=CARTESIAN_POINT('Ctrl Pts',(18.937325424281,11.4591542958431,-18.5422024294089)) ;
#35720=CARTESIAN_POINT('Ctrl Pts',(19.1699147805733,11.0656664148644,-18.5526369833928)) ;
#35721=CARTESIAN_POINT('Ctrl Pts',(19.3901223208208,10.6653172220102,-18.5630715373767)) ;
#35722=CARTESIAN_POINT('Ctrl Pts',(19.6045621556333,10.2754540289221,-18.5732327881228)) ;
#35723=CARTESIAN_POINT('Ctrl Pts',(19.8072603769393,9.87908456548571,-18.583394038869)) ;
#35724=CARTESIAN_POINT('Ctrl Pts',(19.9978365056969,9.47693885988061,-18.5935552896152)) ;
#35725=CARTESIAN_POINT('Ctrl Pts',(20.188393041677,9.07483449812786,-18.603715495702)) ;
#35726=CARTESIAN_POINT('Ctrl Pts',(20.3668298762112,8.6669552877514,-18.6138757017889)) ;
#35727=CARTESIAN_POINT('Ctrl Pts',(20.5328134736599,8.25405390813451,-18.6240359078758)) ;
#35728=CARTESIAN_POINT('Ctrl Pts',(20.698787167029,7.84117716594067,-18.634195507713)) ;
#35729=CARTESIAN_POINT('Ctrl Pts',(20.8523090222703,7.42327906610788,-18.6443551075503)) ;
#35730=CARTESIAN_POINT('Ctrl Pts',(20.9930938002441,7.00113189110542,-18.6545147073876)) ;
#35731=CARTESIAN_POINT('Ctrl Pts',(21.140538479695,6.55901481143818,-18.6651549126918)) ;
#35732=CARTESIAN_POINT('Ctrl Pts',(21.2740119866376,6.1122372486611,-18.6757951179961)) ;
#35733=CARTESIAN_POINT('Ctrl Pts',(21.3932448091053,5.66170571472859,-18.6864353233004)) ;
#35734=CARTESIAN_POINT('Ctrl Pts',(21.5071030430424,5.23148252848763,-18.696595906264)) ;
#35735=CARTESIAN_POINT('Ctrl Pts',(21.6079758403492,4.79783651864598,-18.7067564892277)) ;
#35736=CARTESIAN_POINT('Ctrl Pts',(21.6956801712193,4.36157047067479,-18.7169170721913)) ;
#35737=CARTESIAN_POINT('Ctrl Pts',(21.7833884217748,3.92528492508412,-18.7270781092521)) ;
#35738=CARTESIAN_POINT('Ctrl Pts',(21.8579269871129,3.48637933287732,-18.7372391463129)) ;
#35739=CARTESIAN_POINT('Ctrl Pts',(21.9191640334981,3.04566628754737,-18.7474001833738)) ;
#35740=CARTESIAN_POINT('Ctrl Pts',(21.9804112462253,2.60488007671033,-18.7575629073314)) ;
#35741=CARTESIAN_POINT('Ctrl Pts',(22.028352496046,2.16228604050916,-18.767725631289)) ;
#35742=CARTESIAN_POINT('Ctrl Pts',(22.0629076375027,1.7187034769044,-18.7778883552466)) ;
#35743=CARTESIAN_POINT('Ctrl Pts',(22.0677912277629,1.65601308132613,-18.7793246271773)) ;
#35744=CARTESIAN_POINT('Ctrl Pts',(22.0724075360066,1.59330294842003,-18.780760899108)) ;
#35745=CARTESIAN_POINT('Ctrl Pts',(22.0767564197453,1.53057539694607,-18.7821971710388)) ;
#35746=CARTESIAN_POINT('Ctrl Pts',(22.1083511764002,1.07485805809132,-18.7926317250227)) ;
#35747=CARTESIAN_POINT('Ctrl Pts',(22.1258345572466,0.618103055261106,-18.8030662790066)) ;
#35748=CARTESIAN_POINT('Ctrl Pts',(22.1291628742813,0.161200328877062,-18.8135008329905)) ;
#35749=CARTESIAN_POINT('Ctrl Pts',(22.1324038834859,-0.283717005133503,
-18.82366166958)) ;
#35750=CARTESIAN_POINT('Ctrl Pts',(22.1222229435832,-0.728774169492671,
-18.8338225061696)) ;
#35751=CARTESIAN_POINT('Ctrl Pts',(22.0986325054952,-1.17314809362323,-18.8439833427592)) ;
#35752=CARTESIAN_POINT('Ctrl Pts',(22.0750444935956,-1.61747631555604,-18.8541431343446)) ;
#35753=CARTESIAN_POINT('Ctrl Pts',(22.0380497504388,-2.0611212084516,-18.8643029259301)) ;
#35754=CARTESIAN_POINT('Ctrl Pts',(21.987712794336,-2.50326209900041,-18.8744627175156)) ;
#35755=CARTESIAN_POINT('Ctrl Pts',(21.9373788396031,-2.94537662664519,-18.8846219033177)) ;
#35756=CARTESIAN_POINT('Ctrl Pts',(21.873704287247,-3.38598710307002,-18.8947810891198)) ;
#35757=CARTESIAN_POINT('Ctrl Pts',(21.7968054637468,-3.82427857746736,-18.9049402749218)) ;
#35758=CARTESIAN_POINT('Ctrl Pts',(21.7162632651838,-4.28333578215012,-18.9155807908994)) ;
#35759=CARTESIAN_POINT('Ctrl Pts',(21.6212136012674,-4.7398486899698,-18.926221306877)) ;
#35760=CARTESIAN_POINT('Ctrl Pts',(21.5118505074808,-5.19289156504341,-18.9368618228545)) ;
#35761=CARTESIAN_POINT('Ctrl Pts',(21.4074243627027,-5.62548284629804,-18.947021996854)) ;
#35762=CARTESIAN_POINT('Ctrl Pts',(21.2899483818142,-6.05491017847042,-18.9571821708534)) ;
#35763=CARTESIAN_POINT('Ctrl Pts',(21.1596433130348,-6.48038038448689,-18.9673423448528)) ;
#35764=CARTESIAN_POINT('Ctrl Pts',(21.0293323860427,-6.90586971865379,-18.97750297563)) ;
#35765=CARTESIAN_POINT('Ctrl Pts',(20.8861912882732,-7.32740135243248,-18.9876636064072)) ;
#35766=CARTESIAN_POINT('Ctrl Pts',(20.7304904684155,-7.74419782814426,-18.9978242371844)) ;
#35767=CARTESIAN_POINT('Ctrl Pts',(20.5747637205468,-8.16106371070696,-19.0079865599562)) ;
#35768=CARTESIAN_POINT('Ctrl Pts',(20.4064731518633,-8.57319264461813,-19.018148882728)) ;
#35769=CARTESIAN_POINT('Ctrl Pts',(20.2259378685435,-8.9798258557902,-19.0283112054998)) ;
#35770=CARTESIAN_POINT('Ctrl Pts',(20.200384101217,-9.0373825298899,-19.0297496258841)) ;
#35771=CARTESIAN_POINT('Ctrl Pts',(20.1745850912025,-9.09482913238595,-19.0311880462684)) ;
#35772=CARTESIAN_POINT('Ctrl Pts',(20.1485418203396,-9.15216354620723,-19.0326264666527)) ;
#35773=CARTESIAN_POINT('Ctrl Pts',(19.9596193615738,-9.56807744919059,-19.0430610206366)) ;
#35774=CARTESIAN_POINT('Ctrl Pts',(19.7577899213315,-9.97819337166521,-19.0534955746205)) ;
#35775=CARTESIAN_POINT('Ctrl Pts',(19.5434382712976,-10.3817077399857,-19.0639301286044)) ;
#35776=CARTESIAN_POINT('Ctrl Pts',(19.334694588316,-10.7746651786894,-19.0740916889587)) ;
#35777=CARTESIAN_POINT('Ctrl Pts',(19.1140756649796,-11.1613618636978,-19.0842532493131)) ;
#35778=CARTESIAN_POINT('Ctrl Pts',(18.8819839317268,-11.5410795796802,-19.0944148096674)) ;
#35779=CARTESIAN_POINT('Ctrl Pts',(18.6499160627817,-11.9207582520469,-19.1045753251823)) ;
#35780=CARTESIAN_POINT('Ctrl Pts',(18.406377859936,-12.2934591930215,-19.1147358406971)) ;
#35781=CARTESIAN_POINT('Ctrl Pts',(18.1518164162402,-12.6584910575318,-19.124896356212)) ;
#35782=CARTESIAN_POINT('Ctrl Pts',(17.897270181131,-13.0235011134814,-19.1350562646943)) ;
#35783=CARTESIAN_POINT('Ctrl Pts',(17.6317021521492,-13.3808428201497,-19.1452161731766)) ;
#35784=CARTESIAN_POINT('Ctrl Pts',(17.3556022759239,-13.7298545040522,-19.155376081659)) ;
#35785=CARTESIAN_POINT('Ctrl Pts',(17.066456429831,-14.0953573069438,-19.1660160550429)) ;
#35786=CARTESIAN_POINT('Ctrl Pts',(16.7657597501494,-14.4517237890874,-19.1766560284269)) ;
#35787=CARTESIAN_POINT('Ctrl Pts',(16.4541230109498,-14.7982320228814,-19.1872960018108)) ;
#35788=CARTESIAN_POINT('Ctrl Pts',(16.1565183554016,-15.1291380124246,-19.1974568885603)) ;
#35789=CARTESIAN_POINT('Ctrl Pts',(15.8489371338289,-15.4510536424285,-19.2076177753097)) ;
#35790=CARTESIAN_POINT('Ctrl Pts',(15.531950792724,-15.7633860459896,-19.2177786620592)) ;
#35791=CARTESIAN_POINT('Ctrl Pts',(15.2149503591327,-16.0757323351338,-19.2279400005384)) ;
#35792=CARTESIAN_POINT('Ctrl Pts',(14.8885441357062,-16.3784943872188,-19.2381013390176)) ;
#35793=CARTESIAN_POINT('Ctrl Pts',(14.5533398161578,-16.6711167969616,-19.2482626774968)) ;
#35794=CARTESIAN_POINT('Ctrl Pts',(14.2180799909986,-16.9637876612877,-19.2584256985656)) ;
#35795=CARTESIAN_POINT('Ctrl Pts',(13.8740193316362,-17.2463153775312,-19.2685887196343)) ;
#35796=CARTESIAN_POINT('Ctrl Pts',(13.5217994519541,-17.5181841137612,-19.2787517407031)) ;
#35797=CARTESIAN_POINT('Ctrl Pts',(13.4720779519223,-17.5565627577755,-19.2801864145576)) ;
#35798=CARTESIAN_POINT('Ctrl Pts',(13.4221939082105,-17.5947290580384,-19.281621088412)) ;
#35799=CARTESIAN_POINT('Ctrl Pts',(13.3721491765175,-17.6326816299581,-19.2830557622665)) ;
#35800=CARTESIAN_POINT('Ctrl Pts',(13.0081678766255,-17.908715210202,-19.2934903162504)) ;
#35801=CARTESIAN_POINT('Ctrl Pts',(12.6355894894932,-18.1735105277762,-19.3039248702343)) ;
#35802=CARTESIAN_POINT('Ctrl Pts',(12.2551346890656,-18.4265435938312,-19.3143594242182)) ;
#35803=CARTESIAN_POINT('Ctrl Pts',(11.8846664628094,-18.6729347842174,-19.3245200811526)) ;
#35804=CARTESIAN_POINT('Ctrl Pts',(11.506730223014,-18.908173171776,-19.334680738087)) ;
#35805=CARTESIAN_POINT('Ctrl Pts',(11.122021406894,-19.1318183894551,-19.3448413950214)) ;
#35806=CARTESIAN_POINT('Ctrl Pts',(10.7373521223267,-19.3554406260058,-19.3550010078765)) ;
#35807=CARTESIAN_POINT('Ctrl Pts',(10.3459118499595,-19.5674719568917,-19.3651606207315)) ;
#35808=CARTESIAN_POINT('Ctrl Pts',(9.94842253873426,-19.7675168914384,-19.3753202335865)) ;
#35809=CARTESIAN_POINT('Ctrl Pts',(9.55095687890385,-19.9675499229186,-19.3854792419246)) ;
#35810=CARTESIAN_POINT('Ctrl Pts',(9.14744310432309,-20.1555978797707,-19.3956382502627)) ;
#35811=CARTESIAN_POINT('Ctrl Pts',(8.73862675140959,-20.3313117521238,-19.4057972586008)) ;
#35812=CARTESIAN_POINT('Ctrl Pts',(8.31042829381307,-20.5153562713406,-19.4164379085408)) ;
#35813=CARTESIAN_POINT('Ctrl Pts',(7.87641261126653,-20.6858689254489,-19.4270785584807)) ;
#35814=CARTESIAN_POINT('Ctrl Pts',(7.43746056803071,-20.8425050164679,-19.4377192084207)) ;
#35815=CARTESIAN_POINT('Ctrl Pts',(7.01833641904422,-20.992065701651,-19.4478792097682)) ;
#35816=CARTESIAN_POINT('Ctrl Pts',(6.59471216982767,-21.1289754616445,-19.4580392111156)) ;
#35817=CARTESIAN_POINT('Ctrl Pts',(6.16737233137084,-21.2529845807299,-19.4681992124631)) ;
#35818=CARTESIAN_POINT('Ctrl Pts',(5.74001319418937,-21.3769993000837,-19.4783596726376)) ;
#35819=CARTESIAN_POINT('Ctrl Pts',(5.30893835363587,-21.4881121528177,-19.4885201328121)) ;
#35820=CARTESIAN_POINT('Ctrl Pts',(4.87494638901349,-21.586123616035,-19.4986805929866)) ;
#35821=CARTESIAN_POINT('Ctrl Pts',(4.4408820067301,-21.6841514338429,-19.5088427485767)) ;
#35822=CARTESIAN_POINT('Ctrl Pts',(4.0038997516947,-21.7690734433896,-19.5190049041668)) ;
#35823=CARTESIAN_POINT('Ctrl Pts',(3.56480922029008,-21.8407410653905,-19.529167059757)) ;
#35824=CARTESIAN_POINT('Ctrl Pts',(3.50261795014775,-21.8508918204661,-19.5306063924648)) ;
#35825=CARTESIAN_POINT('Ctrl Pts',(3.44038440017182,-21.860776764644,-19.5320457251726)) ;
#35826=CARTESIAN_POINT('Ctrl Pts',(3.37811088385319,-21.870395559269,-19.5334850578803)) ;
#35827=CARTESIAN_POINT('Ctrl Pts',(2.92127077503222,-21.94095928271,-19.5440440394463)) ;
#35828=CARTESIAN_POINT('Ctrl Pts',(2.46219788517309,-21.997207914348,-19.5546030210123)) ;
#35829=CARTESIAN_POINT('Ctrl Pts',(2.00177361950542,-22.0390275973953,-19.5651620025783)) ;
#35830=CARTESIAN_POINT('Ctrl Pts',(1.54146658847117,-22.0808366321871,-19.5757182955842)) ;
#35831=CARTESIAN_POINT('Ctrl Pts',(1.07980905639184,-22.1082240440806,-19.58627458859)) ;
#35832=CARTESIAN_POINT('Ctrl Pts',(0.617687415648591,-22.1211278491638,
-19.5968308815959)) ;
#35833=CARTESIAN_POINT('Ctrl Pts',(0.412027140883022,-22.1268704932318,
-19.6015288007771)) ;
#35834=CARTESIAN_POINT('Ctrl Pts',(0.206275004551934,-22.1297452581592,
-19.6062267199583)) ;
#35835=CARTESIAN_POINT('Ctrl Pts',(0.00050934658643668,-22.1297499941383,
-19.6109246391395)) ;
#35836=CARTESIAN_POINT('Origin',(0.,0.,5.8748638224677)) ;
#35837=CARTESIAN_POINT('',(18.1314964472961,-9.20710716996868,-2.14394731085456)) ;
#35838=CARTESIAN_POINT('',(18.1314964405175,-9.2071071833178,-1.50729947444597)) ;
#35839=CARTESIAN_POINT('',(18.1314964405232,-9.20710718330643,5.8748638224677)) ;
#35840=CARTESIAN_POINT('',(-16.4382148282779,-11.9710934804213,1.74782063822043E-13)) ;
#35841=CARTESIAN_POINT('Ctrl Pts',(18.1314964473001,-9.20710716996079,-2.14394731121824)) ;
#35842=CARTESIAN_POINT('Ctrl Pts',(18.4070604988656,-8.66444067007858,-2.12914163381511)) ;
#35843=CARTESIAN_POINT('Ctrl Pts',(18.6581480245163,-8.10962743636976,-2.11424200137709)) ;
#35844=CARTESIAN_POINT('Ctrl Pts',(19.1103747290994,-6.97767300525182,-2.08402031193033)) ;
#35845=CARTESIAN_POINT('Ctrl Pts',(19.311139015107,-6.40111261666378,-2.0687139103353)) ;
#35846=CARTESIAN_POINT('Ctrl Pts',(19.6449050680122,-5.28295493835131,-2.03918173204836)) ;
#35847=CARTESIAN_POINT('Ctrl Pts',(19.7821641775101,-4.74319360546866,-2.0249931683764)) ;
#35848=CARTESIAN_POINT('Ctrl Pts',(20.0076220225193,-3.67472276012286,-1.99722483133982)) ;
#35849=CARTESIAN_POINT('Ctrl Pts',(20.097417547488,-3.14679846711533,-1.98365443331201)) ;
#35850=CARTESIAN_POINT('Ctrl Pts',(20.215535744351,-2.23622729969757,-1.9607817254437)) ;
#35851=CARTESIAN_POINT('Ctrl Pts',(20.25405783991,-1.8551927740339,-1.95138198287428)) ;
#35852=CARTESIAN_POINT('Ctrl Pts',(20.328558793268,-0.829593349802003,-1.92629447398207)) ;
#35853=CARTESIAN_POINT('Ctrl Pts',(20.3446471041896,-0.184026714065221,
-1.91071628859271)) ;
#35854=CARTESIAN_POINT('Ctrl Pts',(20.3147745984406,1.13274267984035,-1.87868818779915)) ;
#35855=CARTESIAN_POINT('Ctrl Pts',(20.2662770572425,1.80310203072013,-1.86224593843474)) ;
#35856=CARTESIAN_POINT('Ctrl Pts',(20.1059766817548,3.1131594358071,-1.8294707549246)) ;
#35857=CARTESIAN_POINT('Ctrl Pts',(19.9965465099027,3.75235604437061,-1.81317389417271)) ;
#35858=CARTESIAN_POINT('Ctrl Pts',(19.6850285228298,5.16294251539185,-1.77654689194309)) ;
#35859=CARTESIAN_POINT('Ctrl Pts',(19.4677347381169,5.92989250164944,-1.75616931465371)) ;
#35860=CARTESIAN_POINT('Ctrl Pts',(19.0969913292527,6.99549883656332,-1.72772363405256)) ;
#35861=CARTESIAN_POINT('Ctrl Pts',(18.9803055255759,7.30616789254893,-1.71942424390114)) ;
#35862=CARTESIAN_POINT('Ctrl Pts',(18.6270344095751,8.18106127797865,-1.69610832322852)) ;
#35863=CARTESIAN_POINT('Ctrl Pts',(18.3725214965132,8.73765636526242,-1.68128119906307)) ;
#35864=CARTESIAN_POINT('Ctrl Pts',(17.692629506754,10.0629722209494,-1.64515670408829)) ;
#35865=CARTESIAN_POINT('Ctrl Pts',(17.2418041688731,10.8172420572401,-1.62386139796713)) ;
#35866=CARTESIAN_POINT('Ctrl Pts',(16.4142942665253,12.0178940801389,-1.58777800121821)) ;
#35867=CARTESIAN_POINT('Ctrl Pts',(16.064626498684,12.481450277972,-1.57325807757352)) ;
#35868=CARTESIAN_POINT('Ctrl Pts',(15.2355192782029,13.4879420754917,-1.54032775643703)) ;
#35869=CARTESIAN_POINT('Ctrl Pts',(14.7459402570254,14.0215144549308,-1.52185763212307)) ;
#35870=CARTESIAN_POINT('Ctrl Pts',(13.9156141079229,14.8347582832945,-1.49234182989152)) ;
#35871=CARTESIAN_POINT('Ctrl Pts',(13.5924101608993,15.1314493493459,-1.48125018949377)) ;
#35872=CARTESIAN_POINT('Ctrl Pts',(12.9806406249973,15.6576049047881,-1.4611340156327)) ;
#35873=CARTESIAN_POINT('Ctrl Pts',(12.6949446197056,15.8901228458011,-1.45208134364914)) ;
#35874=CARTESIAN_POINT('Ctrl Pts',(11.9365412565554,16.473845482997,-1.428711200507)) ;
#35875=CARTESIAN_POINT('Ctrl Pts',(11.4546150392463,16.8125072556577,-1.41448677511618)) ;
#35876=CARTESIAN_POINT('Ctrl Pts',(10.3614203648338,17.5118719554038,-1.38297106473484)) ;
#35877=CARTESIAN_POINT('Ctrl Pts',(9.74459614002155,17.8624613848042,-1.36566102265593)) ;
#35878=CARTESIAN_POINT('Ctrl Pts',(8.56695497260617,18.4526208173196,-1.33300576935575)) ;
#35879=CARTESIAN_POINT('Ctrl Pts',(8.01123497730341,18.7005892071007,-1.31775132822014)) ;
#35880=CARTESIAN_POINT('Ctrl Pts',(7.05069167603135,19.0785088641159,-1.29163120878163)) ;
#35881=CARTESIAN_POINT('Ctrl Pts',(6.65138332692506,19.2213644644102,-1.28084508721137)) ;
#35882=CARTESIAN_POINT('Ctrl Pts',(5.6476362773152,19.5454360459507,-1.25400172155765)) ;
#35883=CARTESIAN_POINT('Ctrl Pts',(5.03867446859198,19.7112057522894,-1.23794767112378)) ;
#35884=CARTESIAN_POINT('Ctrl Pts',(4.09048204034264,19.9224997528993,-1.21368061529707)) ;
#35885=CARTESIAN_POINT('Ctrl Pts',(3.75616222978537,19.9882286622897,-1.20527986520689)) ;
#35886=CARTESIAN_POINT('Ctrl Pts',(2.94049161212025,20.1274057392257,-1.18502727560605)) ;
#35887=CARTESIAN_POINT('Ctrl Pts',(2.45784751184561,20.1920266813045,-1.17323622308097)) ;
#35888=CARTESIAN_POINT('Ctrl Pts',(1.16539400332144,20.3180422333094,-1.1417423316886)) ;
#35889=CARTESIAN_POINT('Ctrl Pts',(0.353452242653345,20.3483670971419,-1.12201771310095)) ;
#35890=CARTESIAN_POINT('Ctrl Pts',(-1.03452166985655,20.3170902643203,-1.08767445272038)) ;
#35891=CARTESIAN_POINT('Ctrl Pts',(-1.61010437925601,20.2795943532478,-1.07325669585217)) ;
#35892=CARTESIAN_POINT('Ctrl Pts',(-2.887436311421,20.1416551426706,-1.04082413410225)) ;
#35893=CARTESIAN_POINT('Ctrl Pts',(-3.58710714495018,20.0288845241005,-1.02275548667019)) ;
#35894=CARTESIAN_POINT('Ctrl Pts',(-4.728583451408,19.783163105859,-0.993087957827959)) ;
#35895=CARTESIAN_POINT('Ctrl Pts',(-5.17430308148158,19.6712896363558,-0.981459861869672)) ;
#35896=CARTESIAN_POINT('Ctrl Pts',(-5.96207971388486,19.4449315258678,-0.96101602464987)) ;
#35897=CARTESIAN_POINT('Ctrl Pts',(-6.30560267918617,19.3362646781196,-0.952154263379939)) ;
#35898=CARTESIAN_POINT('Ctrl Pts',(-7.17410015107353,19.0359251514032,-0.929701075255005)) ;
#35899=CARTESIAN_POINT('Ctrl Pts',(-7.69439392225628,18.8316346910951,-0.916193587012207)) ;
#35900=CARTESIAN_POINT('Ctrl Pts',(-8.84950855944488,18.3222111373546,-0.885552539775624)) ;
#35901=CARTESIAN_POINT('Ctrl Pts',(-9.47822329441879,18.0050130882924,-0.8684000658019)) ;
#35902=CARTESIAN_POINT('Ctrl Pts',(-10.5924135477188,17.3683229020488,-0.836647666386695)) ;
#35903=CARTESIAN_POINT('Ctrl Pts',(-11.083076537831,17.0594041772199,-0.822150128390012)) ;
#35904=CARTESIAN_POINT('Ctrl Pts',(-12.1523009529982,16.3206037883209,-0.789333034621653)) ;
#35905=CARTESIAN_POINT('Ctrl Pts',(-12.7225679017549,15.8800750951574,-0.770955141014419)) ;
#35906=CARTESIAN_POINT('Ctrl Pts',(-13.6042674086005,15.1209289036687,-0.741404424010633)) ;
#35907=CARTESIAN_POINT('Ctrl Pts',(-13.9307242687187,14.8207121330741,-0.730189714768981)) ;
#35908=CARTESIAN_POINT('Ctrl Pts',(-14.5090111905555,14.2529051111629,-0.709983274671964)) ;
#35909=CARTESIAN_POINT('Ctrl Pts',(-14.7639050642147,13.9887032134202,-0.700959695861528)) ;
#35910=CARTESIAN_POINT('Ctrl Pts',(-15.4053784238701,13.2867306178644,-0.677735911140703)) ;
#35911=CARTESIAN_POINT('Ctrl Pts',(-15.7805031862737,12.8389492488045,-0.663627217392614)) ;
#35912=CARTESIAN_POINT('Ctrl Pts',(-16.5678199913945,11.8124156469433,-0.632212178287984)) ;
#35913=CARTESIAN_POINT('Ctrl Pts',(-16.9700105384739,11.2269565957541,-0.614886334466801)) ;
#35914=CARTESIAN_POINT('Ctrl Pts',(-17.6564842816621,10.1062311654097,-0.582311719678745)) ;
#35915=CARTESIAN_POINT('Ctrl Pts',(-17.9490644994335,9.57697339141689,-0.567156569360043)) ;
#35916=CARTESIAN_POINT('Ctrl Pts',(-18.5826511492801,8.29951432464586,-0.531081318129922)) ;
#35917=CARTESIAN_POINT('Ctrl Pts',(-18.9027344600243,7.54211406716008,-0.51006273235971)) ;
#35918=CARTESIAN_POINT('Ctrl Pts',(-19.2952777119488,6.42980821109379,-0.480241768079931)) ;
#35919=CARTESIAN_POINT('Ctrl Pts',(-19.4054935741367,6.08908865801761,-0.471249831683759)) ;
#35920=CARTESIAN_POINT('Ctrl Pts',(-19.6860582950359,5.1365600894882,-0.446641306907111)) ;
#35921=CARTESIAN_POINT('Ctrl Pts',(-19.8368358112422,4.51941352605139,-0.431244421412695)) ;
#35922=CARTESIAN_POINT('Ctrl Pts',(-20.1315721908958,3.00961929385165,-0.393939392305378)) ;
#35923=CARTESIAN_POINT('Ctrl Pts',(-20.2453808210544,2.11247495945526,-0.372041340353589)) ;
#35924=CARTESIAN_POINT('Ctrl Pts',(-20.3337181638462,0.631424936674302,
-0.335325976267399)) ;
#35925=CARTESIAN_POINT('Ctrl Pts',(-20.3434557697033,0.0508955018989362,
-0.320806137541027)) ;
#35926=CARTESIAN_POINT('Ctrl Pts',(-20.3094700081703,-1.25448810626689,
-0.287828656960079)) ;
#35927=CARTESIAN_POINT('Ctrl Pts',(-20.2517912924953,-1.97819474295732,
-0.269310323623449)) ;
#35928=CARTESIAN_POINT('Ctrl Pts',(-20.0942908791518,-3.15513204026942,
-0.239157653214394)) ;
#35929=CARTESIAN_POINT('Ctrl Pts',(-20.0174332880666,-3.61078296201057,
-0.227480522918781)) ;
#35930=CARTESIAN_POINT('Ctrl Pts',(-19.8421665466511,-4.47020919927205,
-0.205656060245955)) ;
#35931=CARTESIAN_POINT('Ctrl Pts',(-19.7467703008463,-4.8743624684055,-0.195485321582215)) ;
#35932=CARTESIAN_POINT('Ctrl Pts',(-19.3421533093001,-6.38068085310552,
-0.157484461189357)) ;
#35933=CARTESIAN_POINT('Ctrl Pts',(-18.9524467025526,-7.45900487226203,
-0.129970419011596)) ;
#35934=CARTESIAN_POINT('Ctrl Pts',(-18.33406171794,-8.80320602529759,-0.0933871600585856)) ;
#35935=CARTESIAN_POINT('Ctrl Pts',(-18.1865243033531,-9.10409728854879,
-0.085051792049178)) ;
#35936=CARTESIAN_POINT('Ctrl Pts',(-17.5649938141278,-10.2962000708724,
-0.0513967240819126)) ;
#35937=CARTESIAN_POINT('Ctrl Pts',(-17.0323873926875,-11.1552000722871,
-0.025624345594017)) ;
#35938=CARTESIAN_POINT('Ctrl Pts',(-16.4382148282779,-11.9710934804213,
1.86183533867901E-13)) ;
#35939=CARTESIAN_POINT('',(-16.4251684725406,11.9889877181628,1.11022302462516E-15)) ;
#35940=CARTESIAN_POINT('Origin',(0.,0.,1.11022302462516E-15)) ;
#35941=CARTESIAN_POINT('Ctrl Pts',(-16.4251684725406,11.9889877181628,9.19403442267708E-16)) ;
#35942=CARTESIAN_POINT('Ctrl Pts',(-15.7219712149796,12.952382935206,-0.0296386565568351)) ;
#35943=CARTESIAN_POINT('Ctrl Pts',(-14.9353782007936,13.8520448586411,-0.0582115199547762)) ;
#35944=CARTESIAN_POINT('Ctrl Pts',(-13.6865165338504,15.0495895201416,-0.100707837078664)) ;
#35945=CARTESIAN_POINT('Ctrl Pts',(-13.2839741547818,15.4060671066688,-0.114015439948085)) ;
#35946=CARTESIAN_POINT('Ctrl Pts',(-12.235534047229,16.2628530497365,-0.147905859106198)) ;
#35947=CARTESIAN_POINT('Ctrl Pts',(-11.5727423153889,16.7409765741639,-0.168668796287312)) ;
#35948=CARTESIAN_POINT('Ctrl Pts',(-10.4504160352174,17.4520211923301,-0.202612219255183)) ;
#35949=CARTESIAN_POINT('Ctrl Pts',(-10.0076207859949,17.709651808454,-0.21571277353598)) ;
#35950=CARTESIAN_POINT('Ctrl Pts',(-9.25245913876061,18.1116509552783,-0.237390996457211)) ;
#35951=CARTESIAN_POINT('Ctrl Pts',(-8.94530316347661,18.2653074811295,-0.246030364109235)) ;
#35952=CARTESIAN_POINT('Ctrl Pts',(-8.21650025089806,18.6070997266183,-0.266015168510672)) ;
#35953=CARTESIAN_POINT('Ctrl Pts',(-7.79204552560557,18.7888016920705,-0.277285765206995)) ;
#35954=CARTESIAN_POINT('Ctrl Pts',(-6.69110876728485,19.216364933913,-0.306000207822587)) ;
#35955=CARTESIAN_POINT('Ctrl Pts',(-6.00709437540987,19.441050264074,-0.323367849376024)) ;
#35956=CARTESIAN_POINT('Ctrl Pts',(-4.75371597153538,19.7802785394849,-0.355098077817085)) ;
#35957=CARTESIAN_POINT('Ctrl Pts',(-4.18861647154059,19.9076045446856,-0.369366498788469)) ;
#35958=CARTESIAN_POINT('Ctrl Pts',(-2.81094533615709,20.1567518224348,-0.404281146988823)) ;
#35959=CARTESIAN_POINT('Ctrl Pts',(-1.99493103026704,20.2537968393659,-0.425087477408961)) ;
#35960=CARTESIAN_POINT('Ctrl Pts',(-0.697887529780475,20.3288864237583,
-0.458140229404543)) ;
#35961=CARTESIAN_POINT('Ctrl Pts',(-0.21964999526929,20.3396761523728,-0.470314421784974)) ;
#35962=CARTESIAN_POINT('Ctrl Pts',(0.59746849952955,20.3292872467944,-0.490928594759438)) ;
#35963=CARTESIAN_POINT('Ctrl Pts',(0.936256696337432,20.3165035783119,-0.49941434113361)) ;
#35964=CARTESIAN_POINT('Ctrl Pts',(1.88052753388487,20.2572019990012,-0.522807492740379)) ;
#35965=CARTESIAN_POINT('Ctrl Pts',(2.48447960409391,20.1920278333657,-0.537532244683842)) ;
#35966=CARTESIAN_POINT('Ctrl Pts',(3.51328878711502,20.0341428410562,-0.562781070047226)) ;
#35967=CARTESIAN_POINT('Ctrl Pts',(3.93975081945725,19.9546596075592,-0.573294782305604)) ;
#35968=CARTESIAN_POINT('Ctrl Pts',(4.96485395431136,19.7294573611182,-0.59888790002866)) ;
#35969=CARTESIAN_POINT('Ctrl Pts',(5.56004610352606,19.5700572545556,-0.614023173627694)) ;
#35970=CARTESIAN_POINT('Ctrl Pts',(6.82786080761857,19.168003838611,-0.64713199168191)) ;
#35971=CARTESIAN_POINT('Ctrl Pts',(7.49678808185005,18.9164005021167,-0.665155449979463)) ;
#35972=CARTESIAN_POINT('Ctrl Pts',(8.68573499721003,18.3962105785484,-0.698126809632371)) ;
#35973=CARTESIAN_POINT('Ctrl Pts',(9.21006803657225,18.1393826657444,-0.713013891681812)) ;
#35974=CARTESIAN_POINT('Ctrl Pts',(10.0456123870918,17.684538166588,-0.737065327508699)) ;
#35975=CARTESIAN_POINT('Ctrl Pts',(10.3637717111078,17.4999845891053,-0.746301370099693)) ;
#35976=CARTESIAN_POINT('Ctrl Pts',(11.1369487134599,17.0230060573996,-0.768809774521529)) ;
#35977=CARTESIAN_POINT('Ctrl Pts',(11.58563980657,16.7208648253939,-0.781961505553171)) ;
#35978=CARTESIAN_POINT('Ctrl Pts',(12.5577503102278,16.0083269080645,-0.811211874784397)) ;
#35979=CARTESIAN_POINT('Ctrl Pts',(13.0741611450178,15.5894172898652,-0.827284196837257)) ;
#35980=CARTESIAN_POINT('Ctrl Pts',(13.9886805663289,14.7701083375025,-0.857329854589425)) ;
#35981=CARTESIAN_POINT('Ctrl Pts',(14.3924270211163,14.3769719035031,-0.87123408282866)) ;
#35982=CARTESIAN_POINT('Ctrl Pts',(15.4110846311364,13.2991137050321,-0.908266919871303)) ;
#35983=CARTESIAN_POINT('Ctrl Pts',(15.9967555779025,12.5885557748925,-0.931658915679869)) ;
#35984=CARTESIAN_POINT('Ctrl Pts',(16.878451015568,11.3575200483428,-0.970199293705423)) ;
#35985=CARTESIAN_POINT('Ctrl Pts',(17.2032376720091,10.8592813464447,-0.985303589678979)) ;
#35986=CARTESIAN_POINT('Ctrl Pts',(17.694621029346,10.0279694223595,-1.00937345260218)) ;
#35987=CARTESIAN_POINT('Ctrl Pts',(17.8747258531264,9.7032963799115,-1.0184949619102)) ;
#35988=CARTESIAN_POINT('Ctrl Pts',(18.4048995851386,8.68264789894119,-1.04657461776846)) ;
#35989=CARTESIAN_POINT('Ctrl Pts',(18.7239452244203,7.97136031257796,-1.06533766762343)) ;
#35990=CARTESIAN_POINT('Ctrl Pts',(19.2209235455291,6.66767422753229,-1.09934704103421)) ;
#35991=CARTESIAN_POINT('Ctrl Pts',(19.4141517981003,6.08214457079392,-1.11448617868724)) ;
#35992=CARTESIAN_POINT('Ctrl Pts',(19.7718753841205,4.80600620762275,-1.14746669668622)) ;
#35993=CARTESIAN_POINT('Ctrl Pts',(19.927418170574,4.11372607210993,-1.16535440325119)) ;
#35994=CARTESIAN_POINT('Ctrl Pts',(20.145793450775,2.83173967860662,-1.19839064679211)) ;
#35995=CARTESIAN_POINT('Ctrl Pts',(20.2196230506528,2.24467981957297,-1.21348053536974)) ;
#35996=CARTESIAN_POINT('Ctrl Pts',(20.2978287413328,1.28708130193953,-1.23777705679103)) ;
#35997=CARTESIAN_POINT('Ctrl Pts',(20.3178592037096,0.918168610825223,-1.24705709300463)) ;
#35998=CARTESIAN_POINT('Ctrl Pts',(20.3398770536836,0.102781692689801,-1.26727135936445)) ;
#35999=CARTESIAN_POINT('Ctrl Pts',(20.3372340397449,-0.343626683938318,
-1.2781632442229)) ;
#36000=CARTESIAN_POINT('Ctrl Pts',(20.2920426930773,-1.50661779239668,-1.30645425721975)) ;
#36001=CARTESIAN_POINT('Ctrl Pts',(20.2262473093586,-2.2216691251496,-1.32377799590472)) ;
#36002=CARTESIAN_POINT('Ctrl Pts',(20.03940846552,-3.5040868038042,-1.35544979326474)) ;
#36003=CARTESIAN_POINT('Ctrl Pts',(19.9316425617138,-4.07260761472665,-1.36970457180588)) ;
#36004=CARTESIAN_POINT('Ctrl Pts',(19.6427688522322,-5.30641667700451,-1.40131018670499)) ;
#36005=CARTESIAN_POINT('Ctrl Pts',(19.4517739557115,-5.96866006951631,-1.4187176908526)) ;
#36006=CARTESIAN_POINT('Ctrl Pts',(19.0422020257174,-7.15825970678939,-1.45070432997864)) ;
#36007=CARTESIAN_POINT('Ctrl Pts',(18.8343309265916,-7.6885707034895,-1.4652318784316)) ;
#36008=CARTESIAN_POINT('Ctrl Pts',(18.4579742636463,-8.5414796265195,-1.4888054269677)) ;
#36009=CARTESIAN_POINT('Ctrl Pts',(18.3026026643531,-8.86952253996998,-1.49792082093674)) ;
#36010=CARTESIAN_POINT('Ctrl Pts',(18.13618981682,-9.19786016798943,-1.50704257034263)) ;
#36011=CARTESIAN_POINT('Ctrl Pts',(18.1338440092164,-9.20248413150992,-1.50717103379489)) ;
#36012=CARTESIAN_POINT('Ctrl Pts',(18.1314964405117,-9.20710718332916,-1.50729947444597)) ;
#36013=CARTESIAN_POINT('Origin',(0.,0.,5.8748638224677)) ;
#36014=CARTESIAN_POINT('',(18.1314964416892,-9.20710718101026,-5.31929120111857)) ;
#36015=CARTESIAN_POINT('',(18.1314964277575,-9.20710720844602,-4.68087293510305)) ;
#36016=CARTESIAN_POINT('',(18.1314964405232,-9.20710718330643,5.8748638224677)) ;
#36017=CARTESIAN_POINT('Ctrl Pts',(18.1314964428552,-9.20710717871412,-5.31929120111857)) ;
#36018=CARTESIAN_POINT('Ctrl Pts',(18.1559821510112,-9.15888763247507,-5.31792774964532)) ;
#36019=CARTESIAN_POINT('Ctrl Pts',(18.1802763413727,-9.1105687599884,-5.3165631336081)) ;
#36020=CARTESIAN_POINT('Ctrl Pts',(18.5257542087327,-8.41656031266548,-5.29698693603004)) ;
#36021=CARTESIAN_POINT('Ctrl Pts',(18.812559440899,-7.75433145747545,-5.27858124043252)) ;
#36022=CARTESIAN_POINT('Ctrl Pts',(19.2173957433681,-6.66400522939126,-5.24904220623317)) ;
#36023=CARTESIAN_POINT('Ctrl Pts',(19.3576696079644,-6.24482956744858,-5.23786576038616)) ;
#36024=CARTESIAN_POINT('Ctrl Pts',(19.5891884193155,-5.46994018417184,-5.21770239003431)) ;
#36025=CARTESIAN_POINT('Ctrl Pts',(19.6846715106068,-5.11568730207103,-5.20868442153962)) ;
#36026=CARTESIAN_POINT('Ctrl Pts',(19.9070235798934,-4.1919693321225,-5.18548127515127)) ;
#36027=CARTESIAN_POINT('Ctrl Pts',(20.01906597078,-3.61928115521873,-5.17138750943531)) ;
#36028=CARTESIAN_POINT('Ctrl Pts',(20.2125403282271,-2.34073661212831,-5.1399886145783)) ;
#36029=CARTESIAN_POINT('Ctrl Pts',(20.2819235790346,-1.63382978160729,-5.12266394850667)) ;
#36030=CARTESIAN_POINT('Ctrl Pts',(20.341628685311,-0.322271658271764,-5.0901250649481)) ;
#36031=CARTESIAN_POINT('Ctrl Pts',(20.3422387413483,0.281122441438539,-5.07500528495166)) ;
#36032=CARTESIAN_POINT('Ctrl Pts',(20.2805486881811,1.69944790969356,-5.03909214548146)) ;
#36033=CARTESIAN_POINT('Ctrl Pts',(20.1959593676048,2.51236867865972,-5.01820225209204)) ;
#36034=CARTESIAN_POINT('Ctrl Pts',(20.003033753051,3.67892060385428,-4.98830116649707)) ;
#36035=CARTESIAN_POINT('Ctrl Pts',(19.9336141555108,4.03817398281195,-4.97911105857734)) ;
#36036=CARTESIAN_POINT('Ctrl Pts',(19.7169315789473,5.01696301556774,-4.95426715437512)) ;
#36037=CARTESIAN_POINT('Ctrl Pts',(19.5502062721511,5.6317631709054,-4.93882867315064)) ;
#36038=CARTESIAN_POINT('Ctrl Pts',(19.0789827810852,7.0939118971983,-4.90157021711408)) ;
#36039=CARTESIAN_POINT('Ctrl Pts',(18.7465469335426,7.9308345030986,-4.87975936640964)) ;
#36040=CARTESIAN_POINT('Ctrl Pts',(18.1096423233854,9.26829907880833,-4.8430982931057)) ;
#36041=CARTESIAN_POINT('Ctrl Pts',(17.8370604409887,9.78262637817891,-4.82854004079058)) ;
#36042=CARTESIAN_POINT('Ctrl Pts',(17.1739178738523,10.9137770434637,-4.79542382251435)) ;
#36043=CARTESIAN_POINT('Ctrl Pts',(16.7714468156124,11.522697112974,-4.77680392585817)) ;
#36044=CARTESIAN_POINT('Ctrl Pts',(16.0652550039059,12.4754979401561,-4.74669152458499)) ;
#36045=CARTESIAN_POINT('Ctrl Pts',(15.7810933767637,12.8330652546081,-4.7351519394572)) ;
#36046=CARTESIAN_POINT('Ctrl Pts',(15.2189472597664,13.4934904143528,-4.71357318973011)) ;
#36047=CARTESIAN_POINT('Ctrl Pts',(14.9433454287944,13.7980821014407,-4.70351182668701)) ;
#36048=CARTESIAN_POINT('Ctrl Pts',(13.7819594721497,15.005991399071,-4.66268786995385)) ;
#36049=CARTESIAN_POINT('Ctrl Pts',(12.822039094026,15.8340616479812,-4.63230648977514)) ;
#36050=CARTESIAN_POINT('Ctrl Pts',(11.2705226606738,16.9383022133271,-4.5850307035503)) ;
#36051=CARTESIAN_POINT('Ctrl Pts',(10.7324344207221,17.284258819552,-4.56896247581451)) ;
#36052=CARTESIAN_POINT('Ctrl Pts',(9.49726269523084,17.99844555663,-4.53279983291788)) ;
#36053=CARTESIAN_POINT('Ctrl Pts',(8.79325973576812,18.3526734065808,-4.51265608620187)) ;
#36054=CARTESIAN_POINT('Ctrl Pts',(7.75698817238502,18.8007388644242,-4.48416089966032)) ;
#36055=CARTESIAN_POINT('Ctrl Pts',(7.44011275310201,18.9283748749947,-4.47560413940647)) ;
#36056=CARTESIAN_POINT('Ctrl Pts',(6.52246470706421,19.2713935114325,-4.45136992208235)) ;
#36057=CARTESIAN_POINT('Ctrl Pts',(5.9145711602534,19.4665614275168,-4.43590902175634)) ;
#36058=CARTESIAN_POINT('Ctrl Pts',(4.46238337407389,19.8584778008896,-4.39943068161008)) ;
#36059=CARTESIAN_POINT('Ctrl Pts',(3.61270560573872,20.0304855698857,-4.37841506745215)) ;
#36060=CARTESIAN_POINT('Ctrl Pts',(2.18029147518007,20.2263288514101,-4.34264201396965)) ;
#36061=CARTESIAN_POINT('Ctrl Pts',(1.60283395315019,20.2802604584607,-4.3281401286249)) ;
#36062=CARTESIAN_POINT('Ctrl Pts',(0.303975372320136,20.3457402264736,-4.29530039101204)) ;
#36063=CARTESIAN_POINT('Ctrl Pts',(-0.417335032413373,20.3437304944877,
-4.27690391106356)) ;
#36064=CARTESIAN_POINT('Ctrl Pts',(-1.57868926258423,20.2786937551661,-4.24736157726332)) ;
#36065=CARTESIAN_POINT('Ctrl Pts',(-2.01944860790256,20.2395531485828,-4.23617301754538)) ;
#36066=CARTESIAN_POINT('Ctrl Pts',(-2.82252969581127,20.1417411123703,-4.21600245294478)) ;
#36067=CARTESIAN_POINT('Ctrl Pts',(-3.18521255936294,20.0875790072685,-4.20698899832239)) ;
#36068=CARTESIAN_POINT('Ctrl Pts',(-4.1198644264802,19.9220500231144,-4.18380767998688)) ;
#36069=CARTESIAN_POINT('Ctrl Pts',(-4.68886700872009,19.7958553722445,-4.16973101253819)) ;
#36070=CARTESIAN_POINT('Ctrl Pts',(-5.93742480729189,19.462087328627,-4.1383495640242)) ;
#36071=CARTESIAN_POINT('Ctrl Pts',(-6.61310926607348,19.242989159634,-4.12102518045135)) ;
#36072=CARTESIAN_POINT('Ctrl Pts',(-7.83847800144446,18.7734692246094,-4.08850431681238)) ;
#36073=CARTESIAN_POINT('Ctrl Pts',(-8.39114766142448,18.5330384800905,-4.07340268560286)) ;
#36074=CARTESIAN_POINT('Ctrl Pts',(-9.66340846286822,17.9109683531498,-4.03757887817461)) ;
#36075=CARTESIAN_POINT('Ctrl Pts',(-10.3723728449488,17.5099435998261,-4.01676128458584)) ;
#36076=CARTESIAN_POINT('Ctrl Pts',(-11.3644555938423,16.8673273129995,-3.986864930243)) ;
#36077=CARTESIAN_POINT('Ctrl Pts',(-11.6680254241961,16.6587745831404,-3.97761235817111)) ;
#36078=CARTESIAN_POINT('Ctrl Pts',(-12.4761743375731,16.0706424584172,-3.95283884329037)) ;
#36079=CARTESIAN_POINT('Ctrl Pts',(-12.969012009516,15.6756248780064,-3.93752735238435)) ;
#36080=CARTESIAN_POINT('Ctrl Pts',(-14.124125878444,14.6579622040014,-3.90018900818199)) ;
#36081=CARTESIAN_POINT('Ctrl Pts',(-14.7645845484479,14.0126306882734,-3.87817348869706)) ;
#36082=CARTESIAN_POINT('Ctrl Pts',(-15.7414024152423,12.8867905911197,-3.84128411561408)) ;
#36083=CARTESIAN_POINT('Ctrl Pts',(-16.103972501381,12.430735397658,-3.82671197625354)) ;
#36084=CARTESIAN_POINT('Ctrl Pts',(-16.8766837623956,11.3681406801463,-3.79352754605739)) ;
#36085=CARTESIAN_POINT('Ctrl Pts',(-17.274663788893,10.7537463644558,-3.77485250637854)) ;
#36086=CARTESIAN_POINT('Ctrl Pts',(-17.8643813866559,9.72582113497613,-3.74476532263966)) ;
#36087=CARTESIAN_POINT('Ctrl Pts',(-18.0768666610458,9.32494587308614,-3.73330351633081)) ;
#36088=CARTESIAN_POINT('Ctrl Pts',(-18.4564949196336,8.54690779082685,-3.7117648017382)) ;
#36089=CARTESIAN_POINT('Ctrl Pts',(-18.6259193753762,8.17110568143938,-3.70166870844146)) ;
#36090=CARTESIAN_POINT('Ctrl Pts',(-19.2656157557448,6.62870580523238,-3.6609904811159)) ;
#36091=CARTESIAN_POINT('Ctrl Pts',(-19.6386135852726,5.42480940085267,-3.63078223882926)) ;
#36092=CARTESIAN_POINT('Ctrl Pts',(-20.0288419676727,3.57349332928095,-3.58382219019039)) ;
#36093=CARTESIAN_POINT('Ctrl Pts',(-20.1305592892701,2.94702166548093,-3.56788497202938)) ;
#36094=CARTESIAN_POINT('Ctrl Pts',(-20.2919301335513,1.53986115124165,-3.53199399658883)) ;
#36095=CARTESIAN_POINT('Ctrl Pts',(-20.336135819065,0.758404399295824,-3.51198995184768)) ;
#36096=CARTESIAN_POINT('Ctrl Pts',(-20.3348212719647,-0.371850029604857,
-3.48344537174236)) ;
#36097=CARTESIAN_POINT('Ctrl Pts',(-20.3254730830073,-0.719985144308301,
-3.47471456322468)) ;
#36098=CARTESIAN_POINT('Ctrl Pts',(-20.2760620399025,-1.65975043878857,
-3.45142170283921)) ;
#36099=CARTESIAN_POINT('Ctrl Pts',(-20.2190580112873,-2.2501481542125,-3.4370326667016)) ;
#36100=CARTESIAN_POINT('Ctrl Pts',(-20.0068234580975,-3.75642445874931,
-3.40013501711456)) ;
#36101=CARTESIAN_POINT('Ctrl Pts',(-19.8145176404088,-4.66568197339976,
-3.37764394821454)) ;
#36102=CARTESIAN_POINT('Ctrl Pts',(-19.4012900804551,-6.11983084814863,
-3.34022694617133)) ;
#36103=CARTESIAN_POINT('Ctrl Pts',(-19.2177301737652,-6.67392121870762,
-3.32562601743648)) ;
#36104=CARTESIAN_POINT('Ctrl Pts',(-18.7493477397926,-7.90730586690761,
-3.29230002823761)) ;
#36105=CARTESIAN_POINT('Ctrl Pts',(-18.4509419304834,-8.58057464067465,
-3.2735105166438)) ;
#36106=CARTESIAN_POINT('Ctrl Pts',(-17.9246075092757,-9.61297600972349,
-3.24409445403031)) ;
#36107=CARTESIAN_POINT('Ctrl Pts',(-17.7208015771778,-9.98368956859351,
-3.23340709515066)) ;
#36108=CARTESIAN_POINT('Ctrl Pts',(-17.3144346144009,-10.6711501975291,
-3.21350673853816)) ;
#36109=CARTESIAN_POINT('Ctrl Pts',(-17.114361987694,-10.989163170545,-3.20427955772466)) ;
#36110=CARTESIAN_POINT('Ctrl Pts',(-16.562748791522,-11.8143093382929,-3.18005395100237)) ;
#36111=CARTESIAN_POINT('Ctrl Pts',(-16.1967411976689,-12.3113009502041,
-3.16515691186729)) ;
#36112=CARTESIAN_POINT('Ctrl Pts',(-15.3773813481496,-13.3239768187198,
-3.133503402729)) ;
#36113=CARTESIAN_POINT('Ctrl Pts',(-14.9193693249711,-13.8349059995625,
-3.11674068766792)) ;
#36114=CARTESIAN_POINT('Ctrl Pts',(-13.9983046704741,-14.7633478698724,
-3.08429713304078)) ;
#36115=CARTESIAN_POINT('Ctrl Pts',(-13.5401522683127,-15.1846382880166,
-3.06867986646868)) ;
#36116=CARTESIAN_POINT('Ctrl Pts',(-12.273494607637,-16.246406544396,-3.02682294982442)) ;
#36117=CARTESIAN_POINT('Ctrl Pts',(-11.4343779880079,-16.847533591618,-3.00035128809016)) ;
#36118=CARTESIAN_POINT('Ctrl Pts',(-10.2573202563203,-17.5621546356799,
-2.96597026664429)) ;
#36119=CARTESIAN_POINT('Ctrl Pts',(-9.95678235336474,-17.7342713265434,
-2.95743783011756)) ;
#36120=CARTESIAN_POINT('Ctrl Pts',(-9.20534756741494,-18.1394892450863,
-2.9365538209568)) ;
#36121=CARTESIAN_POINT('Ctrl Pts',(-8.74983841907269,-18.3635460865105,
-2.92426988918525)) ;
#36122=CARTESIAN_POINT('Ctrl Pts',(-7.57919642304287,-18.8859082291014,
-2.89317653789288)) ;
#36123=CARTESIAN_POINT('Ctrl Pts',(-6.85452267548015,-19.1608260831607,
-2.874342072748)) ;
#36124=CARTESIAN_POINT('Ctrl Pts',(-5.56729315337474,-19.5667622311266,
-2.84095791844988)) ;
#36125=CARTESIAN_POINT('Ctrl Pts',(-5.01155363446369,-19.7164210453311,
-2.82657401849589)) ;
#36126=CARTESIAN_POINT('Ctrl Pts',(-3.76434522106229,-19.9961441505205,
-2.79431156345238)) ;
#36127=CARTESIAN_POINT('Ctrl Pts',(-3.07095541609495,-20.1143058864918,
-2.77638121592286)) ;
#36128=CARTESIAN_POINT('Ctrl Pts',(-1.9109392768459,-20.2505950739922,-2.74669961807585)) ;
#36129=CARTESIAN_POINT('Ctrl Pts',(-1.44730307479802,-20.2890021451473,
-2.73492410963611)) ;
#36130=CARTESIAN_POINT('Ctrl Pts',(-0.626954948110609,-20.3286941224461,
-2.71443328580762)) ;
#36131=CARTESIAN_POINT('Ctrl Pts',(-0.270762259295128,-20.3365573588638,
-2.70566650212191)) ;
#36132=CARTESIAN_POINT('Ctrl Pts',(0.629321581591579,-20.3327749817555,
-2.6836673689249)) ;
#36133=CARTESIAN_POINT('Ctrl Pts',(1.17288107122135,-20.3086714890162,-2.67051431989398)) ;
#36134=CARTESIAN_POINT('Ctrl Pts',(2.43130969904529,-20.2021719751195,-2.63986861127068)) ;
#36135=CARTESIAN_POINT('Ctrl Pts',(3.14407350940222,-20.1035770788437,-2.62235408269805)) ;
#36136=CARTESIAN_POINT('Ctrl Pts',(4.41601894790743,-19.8583211785809,-2.59031105777517)) ;
#36137=CARTESIAN_POINT('Ctrl Pts',(4.97702696327167,-19.7251954957874,-2.57589920033517)) ;
#36138=CARTESIAN_POINT('Ctrl Pts',(6.21209824809652,-19.376064520588,-2.54350015905168)) ;
#36139=CARTESIAN_POINT('Ctrl Pts',(6.88207995319268,-19.1483422019311,-2.52545957319964)) ;
#36140=CARTESIAN_POINT('Ctrl Pts',(7.96696701704833,-18.7152859913309,-2.49577841572246)) ;
#36141=CARTESIAN_POINT('Ctrl Pts',(8.38917057033345,-18.5298762748669,-2.48410975236042)) ;
#36142=CARTESIAN_POINT('Ctrl Pts',(9.12911082110965,-18.1744556599384,-2.46363482643909)) ;
#36143=CARTESIAN_POINT('Ctrl Pts',(9.44931891438479,-18.0100492850482,-2.45478133249999)) ;
#36144=CARTESIAN_POINT('Ctrl Pts',(10.25391352465,-17.5695738505339,-2.43236865412459)) ;
#36145=CARTESIAN_POINT('Ctrl Pts',(10.7316215597439,-17.2819261129632,-2.41889297829457)) ;
#36146=CARTESIAN_POINT('Ctrl Pts',(11.7856830911829,-16.5866554654144,-2.38824614270176)) ;
#36147=CARTESIAN_POINT('Ctrl Pts',(12.3538488586625,-16.1679273323465,-2.37105567099732)) ;
#36148=CARTESIAN_POINT('Ctrl Pts',(13.3470239570827,-15.3530011744314,-2.33926772330736)) ;
#36149=CARTESIAN_POINT('Ctrl Pts',(13.7790261411589,-14.9665000387234,-2.32477401215987)) ;
#36150=CARTESIAN_POINT('Ctrl Pts',(14.7092110958243,-14.0598316175406,-2.29197434772223)) ;
#36151=CARTESIAN_POINT('Ctrl Pts',(15.1974680285817,-13.5305844023817,-2.27361024388068)) ;
#36152=CARTESIAN_POINT('Ctrl Pts',(15.9399896757244,-12.6347091686847,-2.24405621502609)) ;
#36153=CARTESIAN_POINT('Ctrl Pts',(16.2120666867259,-12.2836494797824,-2.23282498533318)) ;
#36154=CARTESIAN_POINT('Ctrl Pts',(16.6870212631333,-11.6275205233157,-2.21262927117704)) ;
#36155=CARTESIAN_POINT('Ctrl Pts',(16.893567392919,-11.3253385544376,-2.20363190181635)) ;
#36156=CARTESIAN_POINT('Ctrl Pts',(17.4061026073839,-10.5302419978033,-2.18052815892107)) ;
#36157=CARTESIAN_POINT('Ctrl Pts',(17.6993580095662,-10.0295131625774,-2.16651221541519)) ;
#36158=CARTESIAN_POINT('Ctrl Pts',(18.0252615792884,-9.41411009224698,-2.1496040846359)) ;
#36159=CARTESIAN_POINT('Ctrl Pts',(18.078826114347,-9.31083051511026,-2.14677721575038)) ;
#36160=CARTESIAN_POINT('Ctrl Pts',(18.1314964473001,-9.2071071699608,-2.14394731121824)) ;
#36161=CARTESIAN_POINT('Ctrl Pts',(18.1314964405117,-9.20710718332915,-1.50729947444597)) ;
#36162=CARTESIAN_POINT('Ctrl Pts',(17.931679960588,-9.60060448083557,-1.51823187387938)) ;
#36163=CARTESIAN_POINT('Ctrl Pts',(17.7191046873647,-9.98749663233832,-1.5290015688187)) ;
#36164=CARTESIAN_POINT('Ctrl Pts',(17.1281981947186,-10.9846234998532,-1.55717469977094)) ;
#36165=CARTESIAN_POINT('Ctrl Pts',(16.7298560809444,-11.5822727656112,-1.57450204871407)) ;
#36166=CARTESIAN_POINT('Ctrl Pts',(15.9545411699598,-12.6218042253867,-1.60619443826675)) ;
#36167=CARTESIAN_POINT('Ctrl Pts',(15.5886620159045,-13.0709959220834,-1.62046639596972)) ;
#36168=CARTESIAN_POINT('Ctrl Pts',(14.7558371702652,-14.0086739984771,-1.65174617509447)) ;
#36169=CARTESIAN_POINT('Ctrl Pts',(14.2827086477002,-14.4907521949825,-1.66880058980069)) ;
#36170=CARTESIAN_POINT('Ctrl Pts',(13.3631368055728,-15.3388471891994,-1.70059535045569)) ;
#36171=CARTESIAN_POINT('Ctrl Pts',(12.9233906504269,-15.7111308707512,-1.71528951228431)) ;
#36172=CARTESIAN_POINT('Ctrl Pts',(12.1801583387756,-16.28799860044,-1.73907935903575)) ;
#36173=CARTESIAN_POINT('Ctrl Pts',(11.8859047649343,-16.5039519441112,-1.748245547445)) ;
#36174=CARTESIAN_POINT('Ctrl Pts',(11.2171270537096,-16.9676017320783,-1.76841089369576)) ;
#36175=CARTESIAN_POINT('Ctrl Pts',(10.8398896254436,-17.2110501102726,-1.7793635901593)) ;
#36176=CARTESIAN_POINT('Ctrl Pts',(9.84075242908301,-17.8099489333762,-1.80767708616042)) ;
#36177=CARTESIAN_POINT('Ctrl Pts',(9.20758678954942,-18.1453860492822,-1.82496471288984)) ;
#36178=CARTESIAN_POINT('Ctrl Pts',(8.03323387083179,-18.6902074591705,-1.85660421164305)) ;
#36179=CARTESIAN_POINT('Ctrl Pts',(7.49826929292229,-18.911177935506,-1.87086378527517)) ;
#36180=CARTESIAN_POINT('Ctrl Pts',(6.32063693777119,-19.3397699396133,-1.90212207100057)) ;
#36181=CARTESIAN_POINT('Ctrl Pts',(5.67557303286072,-19.5388078214488,-1.91916746525642)) ;
#36182=CARTESIAN_POINT('Ctrl Pts',(4.46336522351739,-19.8477323571006,-1.95096385584129)) ;
#36183=CARTESIAN_POINT('Ctrl Pts',(3.89911576652593,-19.966246663739,-1.96566886219092)) ;
#36184=CARTESIAN_POINT('Ctrl Pts',(2.97056623354441,-20.1204104515116,-1.98947076388529)) ;
#36185=CARTESIAN_POINT('Ctrl Pts',(2.60898812358905,-20.1704825854934,-1.99863835351361)) ;
#36186=CARTESIAN_POINT('Ctrl Pts',(1.7704147312209,-20.2636827344797,-2.01954710877414)) ;
#36187=CARTESIAN_POINT('Ctrl Pts',(1.29285219851626,-20.2997474260199,-2.03121840685039)) ;
#36188=CARTESIAN_POINT('Ctrl Pts',(0.114827243913788,-20.3469671807111,
-2.0598584861084)) ;
#36189=CARTESIAN_POINT('Ctrl Pts',(-0.585785981426001,-20.3388572127459,
-2.07677256901841)) ;
#36190=CARTESIAN_POINT('Ctrl Pts',(-1.85799711370025,-20.2583305087049,
-2.10793922852146)) ;
#36191=CARTESIAN_POINT('Ctrl Pts',(-2.42961215087073,-20.1977495076431,
-2.12210708924134)) ;
#36192=CARTESIAN_POINT('Ctrl Pts',(-3.72189028244642,-20.0051328435108,
-2.15470718588174)) ;
#36193=CARTESIAN_POINT('Ctrl Pts',(-4.43953009968398,-19.8582064770843,
-2.17322951128812)) ;
#36194=CARTESIAN_POINT('Ctrl Pts',(-5.6633056996895,-19.5379894415735,-2.20540541298524)) ;
#36195=CARTESIAN_POINT('Ctrl Pts',(-6.17343150103331,-19.3828482896351,
-2.21899493987718)) ;
#36196=CARTESIAN_POINT('Ctrl Pts',(-7.01052651262709,-19.0918642557179,
-2.2413860423993)) ;
#36197=CARTESIAN_POINT('Ctrl Pts',(-7.3411057299747,-18.9672068466635,-2.25024848035673)) ;
#36198=CARTESIAN_POINT('Ctrl Pts',(-8.09973310493635,-18.658331277792,-2.27053048643341)) ;
#36199=CARTESIAN_POINT('Ctrl Pts',(-8.52503137253512,-18.4678869402404,
-2.28188655391473)) ;
#36200=CARTESIAN_POINT('Ctrl Pts',(-9.57283390191909,-17.9547767688043,
-2.31022903436473)) ;
#36201=CARTESIAN_POINT('Ctrl Pts',(-10.1858964435259,-17.6142178533954,
-2.32715837737893)) ;
#36202=CARTESIAN_POINT('Ctrl Pts',(-11.2675460356486,-16.937969215499,-2.35834655001133)) ;
#36203=CARTESIAN_POINT('Ctrl Pts',(-11.7417986043157,-16.6127226077643,
-2.37252040053138)) ;
#36204=CARTESIAN_POINT('Ctrl Pts',(-12.7896829377169,-15.826760197692,-2.40520335689515)) ;
#36205=CARTESIAN_POINT('Ctrl Pts',(-13.353381014675,-15.3541371600193,-2.42380469731094)) ;
#36206=CARTESIAN_POINT('Ctrl Pts',(-14.2781528882038,-14.4892519524119,
-2.45601194955388)) ;
#36207=CARTESIAN_POINT('Ctrl Pts',(-14.651698515326,-14.111406879844,-2.46955314804877)) ;
#36208=CARTESIAN_POINT('Ctrl Pts',(-15.2480086758211,-13.4589988018858,
-2.49188352326496)) ;
#36209=CARTESIAN_POINT('Ctrl Pts',(-15.4791814507536,-13.1924738048849,
-2.50073309925654)) ;
#36210=CARTESIAN_POINT('Ctrl Pts',(-15.9993633374509,-12.560234379475,-2.52100504250987)) ;
#36211=CARTESIAN_POINT('Ctrl Pts',(-16.2829661866801,-12.1903294675225,
-2.53236368367608)) ;
#36212=CARTESIAN_POINT('Ctrl Pts',(-16.9603847076335,-11.2408995733523,
-2.56069677309593)) ;
#36213=CARTESIAN_POINT('Ctrl Pts',(-17.3374327804186,-10.6501594554693,
-2.57761453501714)) ;
#36214=CARTESIAN_POINT('Ctrl Pts',(-17.9669902824396,-9.54145913085048,
-2.60878651550773)) ;
#36215=CARTESIAN_POINT('Ctrl Pts',(-18.229420337493,-9.0299727804122,-2.62295595904236)) ;
#36216=CARTESIAN_POINT('Ctrl Pts',(-18.7768009261932,-7.84168486601956,
-2.655599681445)) ;
#36217=CARTESIAN_POINT('Ctrl Pts',(-19.0474751251439,-7.15918643759163,
-2.67416527045035)) ;
#36218=CARTESIAN_POINT('Ctrl Pts',(-19.4497598633974,-5.95917948995069,
-2.706358581822)) ;
#36219=CARTESIAN_POINT('Ctrl Pts',(-19.5989900371501,-5.44835479055282,
-2.71992188893821)) ;
#36220=CARTESIAN_POINT('Ctrl Pts',(-19.8136287671889,-4.58984561078642,
-2.74227980842077)) ;
#36221=CARTESIAN_POINT('Ctrl Pts',(-19.8903100757725,-4.2452489795954,-2.75113504185427)) ;
#36222=CARTESIAN_POINT('Ctrl Pts',(-20.0473124236452,-3.44155844627817,
-2.77141131862243)) ;
#36223=CARTESIAN_POINT('Ctrl Pts',(-20.1208997509695,-2.98135181708414,
-2.78276871851628)) ;
#36224=CARTESIAN_POINT('Ctrl Pts',(-20.2654039335711,-1.82380183773396,
-2.81110713779146)) ;
#36225=CARTESIAN_POINT('Ctrl Pts',(-20.3162055848214,-1.12456194766157,
-2.82803125954087)) ;
#36226=CARTESIAN_POINT('Ctrl Pts',(-20.3428032991933,0.150504483196495,
-2.85921209444023)) ;
#36227=CARTESIAN_POINT('Ctrl Pts',(-20.3304243301488,0.725352551259077,
-2.87338391920243)) ;
#36228=CARTESIAN_POINT('Ctrl Pts',(-20.2468210857837,2.03155072083549,-2.90604166894579)) ;
#36229=CARTESIAN_POINT('Ctrl Pts',(-20.1602868809396,2.7611193008484,-2.9246191867066)) ;
#36230=CARTESIAN_POINT('Ctrl Pts',(-19.9433911357388,4.00821911015401,-2.95681697117818)) ;
#36231=CARTESIAN_POINT('Ctrl Pts',(-19.8317802280077,4.5282628989769,-2.97037272203585)) ;
#36232=CARTESIAN_POINT('Ctrl Pts',(-19.6123967152931,5.38520338436748,-2.9927213559517)) ;
#36233=CARTESIAN_POINT('Ctrl Pts',(-19.5159902179828,5.72474037613498,-3.00157477901812)) ;
#36234=CARTESIAN_POINT('Ctrl Pts',(-19.2719081461799,6.50635360558748,-3.02184972770117)) ;
#36235=CARTESIAN_POINT('Ctrl Pts',(-19.1177750820932,6.946204880368,-3.03320759258375)) ;
#36236=CARTESIAN_POINT('Ctrl Pts',(-18.6944326197623,8.03311120996374,-3.0615436430039)) ;
#36237=CARTESIAN_POINT('Ctrl Pts',(-18.4066389319981,8.67227358385617,-3.07846502264682)) ;
#36238=CARTESIAN_POINT('Ctrl Pts',(-17.8237475696155,9.80644029831512,-3.10964206395009)) ;
#36239=CARTESIAN_POINT('Ctrl Pts',(-17.5395098600439,10.3062037006224,-3.12381288683432)) ;
#36240=CARTESIAN_POINT('Ctrl Pts',(-16.8452234401258,11.4148288191342,-3.15645108432189)) ;
#36241=CARTESIAN_POINT('Ctrl Pts',(-16.4226182843025,12.0148850578971,-3.17500951984659)) ;
#36242=CARTESIAN_POINT('Ctrl Pts',(-15.6390393910186,13.0086748133683,-3.20720028692804)) ;
#36243=CARTESIAN_POINT('Ctrl Pts',(-15.2932736843599,13.4134617064196,-3.22076826265459)) ;
#36244=CARTESIAN_POINT('Ctrl Pts',(-14.6923896364129,14.0634382065645,-3.24313224922067)) ;
#36245=CARTESIAN_POINT('Ctrl Pts',(-14.4460376142167,14.3163756175292,-3.25198891965484)) ;
#36246=CARTESIAN_POINT('Ctrl Pts',(-13.8595737623538,14.8879570933692,-3.27226638233046)) ;
#36247=CARTESIAN_POINT('Ctrl Pts',(-13.5148453314719,15.2015792748605,-3.28362356535633)) ;
#36248=CARTESIAN_POINT('Ctrl Pts',(-12.625512279075,15.956481271788,-3.31196185955175)) ;
#36249=CARTESIAN_POINT('Ctrl Pts',(-12.0683028909577,16.381969338984,-3.32888606359975)) ;
#36250=CARTESIAN_POINT('Ctrl Pts',(-11.0160689380441,17.1025878764741,-3.36006674941463)) ;
#36251=CARTESIAN_POINT('Ctrl Pts',(-10.5283403566255,17.4070769617992,-3.37423833645923)) ;
#36252=CARTESIAN_POINT('Ctrl Pts',(-9.39716893216085,18.0483144709618,-3.40668178234294)) ;
#36253=CARTESIAN_POINT('Ctrl Pts',(-8.74727002565604,18.3720900088539,-3.42503881544016)) ;
#36254=CARTESIAN_POINT('Ctrl Pts',(-7.58854779621848,18.8739097072096,-3.45715533181558)) ;
#36255=CARTESIAN_POINT('Ctrl Pts',(-7.08736400983769,19.067768565847,-3.47085224169067)) ;
#36256=CARTESIAN_POINT('Ctrl Pts',(-6.24376845983031,19.3562116692087,-3.49337962385169)) ;
#36257=CARTESIAN_POINT('Ctrl Pts',(-5.90549928457571,19.4620826003385,-3.5022719485616)) ;
#36258=CARTESIAN_POINT('Ctrl Pts',(-5.1168192141225,19.6864652854163,-3.52257739844244)) ;
#36259=CARTESIAN_POINT('Ctrl Pts',(-4.66475971933943,19.7984538934229,-3.53392759252148)) ;
#36260=CARTESIAN_POINT('Ctrl Pts',(-3.52285661358665,20.0400523410299,-3.56228262981554)) ;
#36261=CARTESIAN_POINT('Ctrl Pts',(-2.82940544657397,20.1496570844654,-3.57922972254332)) ;
#36262=CARTESIAN_POINT('Ctrl Pts',(-1.55988901236768,20.2834738028633,-3.61043926899561)) ;
#36263=CARTESIAN_POINT('Ctrl Pts',(-0.985803598136994,20.3194671830052,
-3.62461636408733)) ;
#36264=CARTESIAN_POINT('Ctrl Pts',(0.34907381416042,20.3464501795615,-3.65792906066143)) ;
#36265=CARTESIAN_POINT('Ctrl Pts',(1.10937474094696,20.3191820208798,-3.67717624096812)) ;
#36266=CARTESIAN_POINT('Ctrl Pts',(2.56050338015072,20.1854339997927,-3.71425133826466)) ;
#36267=CARTESIAN_POINT('Ctrl Pts',(3.25090648785058,20.0858043470427,-3.73203484978193)) ;
#36268=CARTESIAN_POINT('Ctrl Pts',(4.24844578666855,19.8890642328277,-3.75748739774337)) ;
#36269=CARTESIAN_POINT('Ctrl Pts',(4.56055729021179,19.8198255676919,-3.76539766653791)) ;
#36270=CARTESIAN_POINT('Ctrl Pts',(5.65433088606337,19.5499777724197,-3.7930408743695)) ;
#36271=CARTESIAN_POINT('Ctrl Pts',(6.42555507314387,19.3102393688022,-3.81246499702841)) ;
#36272=CARTESIAN_POINT('Ctrl Pts',(7.79738916061737,18.7924845669388,-3.84813547191183)) ;
#36273=CARTESIAN_POINT('Ctrl Pts',(8.40259026412085,18.5297927888828,-3.86428651998511)) ;
#36274=CARTESIAN_POINT('Ctrl Pts',(9.58503196085372,17.946684428984,-3.89703783010886)) ;
#36275=CARTESIAN_POINT('Ctrl Pts',(10.1615843856654,17.6266420549615,-3.91361863943306)) ;
#36276=CARTESIAN_POINT('Ctrl Pts',(11.4240029594834,16.8433226018647,-3.95130391409726)) ;
#36277=CARTESIAN_POINT('Ctrl Pts',(12.0992007970443,16.3650450229797,-3.97246317545991)) ;
#36278=CARTESIAN_POINT('Ctrl Pts',(12.8553587923976,15.7569785546575,-3.99687002616268)) ;
#36279=CARTESIAN_POINT('Ctrl Pts',(12.9663512222465,15.6657702985513,-4.00047068462399)) ;
#36280=CARTESIAN_POINT('Ctrl Pts',(13.3504290834985,15.3432751705168,-4.01298161554906)) ;
#36281=CARTESIAN_POINT('Ctrl Pts',(13.618367782473,15.1059626914056,-4.02178721215786)) ;
#36282=CARTESIAN_POINT('Ctrl Pts',(14.4833505067786,14.2981227520694,-4.05071069258373)) ;
#36283=CARTESIAN_POINT('Ctrl Pts',(15.051911897898,13.6983106067469,-4.0705832408216)) ;
#36284=CARTESIAN_POINT('Ctrl Pts',(15.9716005878999,12.6014615600297,-4.10549367227418)) ;
#36285=CARTESIAN_POINT('Ctrl Pts',(16.3398350154851,12.1201749904149,-4.12038340043091)) ;
#36286=CARTESIAN_POINT('Ctrl Pts',(17.0915947667932,11.0409612257292,-4.15312801458585)) ;
#36287=CARTESIAN_POINT('Ctrl Pts',(17.4664003687829,10.4379250757297,-4.17103695047986)) ;
#36288=CARTESIAN_POINT('Ctrl Pts',(18.0918294018035,9.30328775361926,-4.20396119083834)) ;
#36289=CARTESIAN_POINT('Ctrl Pts',(18.3524219535583,8.77804437935544,-4.21891726249764)) ;
#36290=CARTESIAN_POINT('Ctrl Pts',(18.7389458071928,7.90626329195108,-4.24303579536137)) ;
#36291=CARTESIAN_POINT('Ctrl Pts',(18.878790832447,7.56626408438369,-4.25227098886652)) ;
#36292=CARTESIAN_POINT('Ctrl Pts',(19.165662910752,6.81124419867061,-4.2722892913204)) ;
#36293=CARTESIAN_POINT('Ctrl Pts',(19.3085844787189,6.39486142599375,-4.28303329335084)) ;
#36294=CARTESIAN_POINT('Ctrl Pts',(19.6501461161649,5.28353754798832,-4.31129854211033)) ;
#36295=CARTESIAN_POINT('Ctrl Pts',(19.8254506778058,4.5820865525839,-4.3287387600465)) ;
#36296=CARTESIAN_POINT('Ctrl Pts',(20.0735365754715,3.30328165574474,-4.36057039461972)) ;
#36297=CARTESIAN_POINT('Ctrl Pts',(20.1595990429213,2.72930371006243,-4.37486635117816)) ;
#36298=CARTESIAN_POINT('Ctrl Pts',(20.2941852977256,1.46493687931805,-4.40657679710737)) ;
#36299=CARTESIAN_POINT('Ctrl Pts',(20.3322567287544,0.774157649557999,-4.42404857398858)) ;
#36300=CARTESIAN_POINT('Ctrl Pts',(20.3373822022035,-0.484781177569453,
-4.45605319658284)) ;
#36301=CARTESIAN_POINT('Ctrl Pts',(20.3159298056552,-1.05219992621706,-4.47053345588276)) ;
#36302=CARTESIAN_POINT('Ctrl Pts',(20.2419180649595,-1.97945371830992,-4.49405182864441)) ;
#36303=CARTESIAN_POINT('Ctrl Pts',(20.20340142889,-2.34009849004814,-4.50315872875805)) ;
#36304=CARTESIAN_POINT('Ctrl Pts',(20.09513401912,-3.1484475524981,-4.52336630592519)) ;
#36305=CARTESIAN_POINT('Ctrl Pts',(20.0200247136739,-3.59523975853926,-4.53441644919468)) ;
#36306=CARTESIAN_POINT('Ctrl Pts',(19.7884420576793,-4.73791899084519,-4.56275156300918)) ;
#36307=CARTESIAN_POINT('Ctrl Pts',(19.610174850103,-5.42875285913641,-4.57996688218247)) ;
#36308=CARTESIAN_POINT('Ctrl Pts',(19.2224294398213,-6.65988090871565,-4.61151468807607)) ;
#36309=CARTESIAN_POINT('Ctrl Pts',(19.0254576747953,-7.20331587378892,-4.6257563455703)) ;
#36310=CARTESIAN_POINT('Ctrl Pts',(18.6004501997403,-8.23625949884474,-4.65361808332889)) ;
#36311=CARTESIAN_POINT('Ctrl Pts',(18.3755607890832,-8.72647284682466,-4.66720239419565)) ;
#36312=CARTESIAN_POINT('Ctrl Pts',(18.1314964277493,-9.20710720846217,-4.68087293438847)) ;
#36313=CARTESIAN_POINT('Origin',(0.,0.,5.8748638224677)) ;
#36314=CARTESIAN_POINT('',(18.1314964426296,-9.20710717915839,-8.49264489791374)) ;
#36315=CARTESIAN_POINT('',(18.1314964397986,-9.2071071847335,-7.85560087779543)) ;
#36316=CARTESIAN_POINT('',(18.1314964405232,-9.20710718330643,5.8748638224677)) ;
#36317=CARTESIAN_POINT('Ctrl Pts',(18.131496444736,-9.20710717501038,-8.49264489791374)) ;
#36318=CARTESIAN_POINT('Ctrl Pts',(18.1932674928183,-9.08546185065345,-8.48921597676009)) ;
#36319=CARTESIAN_POINT('Ctrl Pts',(18.2538163712279,-8.96319091114333,-8.48579881785955)) ;
#36320=CARTESIAN_POINT('Ctrl Pts',(18.4728147531323,-8.50952521834696,-8.4732394955958)) ;
#36321=CARTESIAN_POINT('Ctrl Pts',(18.6235044093928,-8.17447174954134,-8.46421003414079)) ;
#36322=CARTESIAN_POINT('Ctrl Pts',(18.9904852834932,-7.29560107995186,-8.44095127109311)) ;
#36323=CARTESIAN_POINT('Ctrl Pts',(19.1925271143377,-6.74620138477858,-8.42681393123442)) ;
#36324=CARTESIAN_POINT('Ctrl Pts',(19.5865814277305,-5.5128443631374,-8.39537318257033)) ;
#36325=CARTESIAN_POINT('Ctrl Pts',(19.7670274914648,-4.82599611654746,-8.37805044530867)) ;
#36326=CARTESIAN_POINT('Ctrl Pts',(20.0340665331976,-3.53892179136578,-8.3454695286419)) ;
#36327=CARTESIAN_POINT('Ctrl Pts',(20.1304533551351,-2.941534835654,-8.33030467021252)) ;
#36328=CARTESIAN_POINT('Ctrl Pts',(20.2948600824927,-1.52274471572167,-8.29416956240355)) ;
#36329=CARTESIAN_POINT('Ctrl Pts',(20.3398733544353,-0.699744311822382,
-8.27309999793224)) ;
#36330=CARTESIAN_POINT('Ctrl Pts',(20.3326732563183,0.483760817714732,-8.2431822172196)) ;
#36331=CARTESIAN_POINT('Ctrl Pts',(20.3209206250887,0.843692761431439,-8.23414218048783)) ;
#36332=CARTESIAN_POINT('Ctrl Pts',(20.2619672669607,1.83837644347612,-8.20945746357235)) ;
#36333=CARTESIAN_POINT('Ctrl Pts',(20.1945184988773,2.47151386605704,-8.19402822491205)) ;
#36334=CARTESIAN_POINT('Ctrl Pts',(19.9612492075238,3.9835945910032,-8.15692170200691)) ;
#36335=CARTESIAN_POINT('Ctrl Pts',(19.7669429729029,4.85679412600449,-8.13525196739468)) ;
#36336=CARTESIAN_POINT('Ctrl Pts',(19.3524424112644,6.27240414608569,-8.09874849696558)) ;
#36337=CARTESIAN_POINT('Ctrl Pts',(19.1651896699438,6.82316474363552,-8.08420010532792)) ;
#36338=CARTESIAN_POINT('Ctrl Pts',(18.690967904662,8.04360082058764,-8.05113229623419)) ;
#36339=CARTESIAN_POINT('Ctrl Pts',(18.3911030964677,8.70741723048133,-8.03255152790795)) ;
#36340=CARTESIAN_POINT('Ctrl Pts',(17.8452784204912,9.7610699717966,-8.00242067816574)) ;
#36341=CARTESIAN_POINT('Ctrl Pts',(17.620533104815,10.1611646401539,-7.99082532445382)) ;
#36342=CARTESIAN_POINT('Ctrl Pts',(17.1698355381235,10.9035120098911,-7.96921656654375)) ;
#36343=CARTESIAN_POINT('Ctrl Pts',(16.9466879673368,11.2472039390264,-7.95917882762995)) ;
#36344=CARTESIAN_POINT('Ctrl Pts',(15.9898515385722,12.6277299165048,-7.9182548591709)) ;
#36345=CARTESIAN_POINT('Ctrl Pts',(15.1702019484581,13.6014667716605,-7.88775489658032)) ;
#36346=CARTESIAN_POINT('Ctrl Pts',(13.8068741521705,14.9434136805402,-7.84025866223606)) ;
#36347=CARTESIAN_POINT('Ctrl Pts',(13.327522494099,15.3724597544759,-7.82409645369742)) ;
#36348=CARTESIAN_POINT('Ctrl Pts',(12.2147766604731,16.277198542221,-7.78774176398343)) ;
#36349=CARTESIAN_POINT('Ctrl Pts',(11.5722923534326,16.7400719244327,-7.76750070324327)) ;
#36350=CARTESIAN_POINT('Ctrl Pts',(10.6197969596022,17.345191026119,-7.73903165503595)) ;
#36351=CARTESIAN_POINT('Ctrl Pts',(10.3306569328559,17.5189403838093,-7.73058763602346)) ;
#36352=CARTESIAN_POINT('Ctrl Pts',(9.90571895203523,17.7601130953422,-7.71850594637521)) ;
#36353=CARTESIAN_POINT('Ctrl Pts',(9.77328262245036,17.8333348573003,-7.71478237534946)) ;
#36354=CARTESIAN_POINT('Ctrl Pts',(9.2597694124691,18.1098089481559,-7.70048200028835)) ;
#36355=CARTESIAN_POINT('Ctrl Pts',(8.8730704250491,18.3023805470242,-7.68999991658958)) ;
#36356=CARTESIAN_POINT('Ctrl Pts',(7.64276566526082,18.866895267784,-7.65716672155101)) ;
#36357=CARTESIAN_POINT('Ctrl Pts',(6.77983813774774,19.1938893097623,-7.63483030379097)) ;
#36358=CARTESIAN_POINT('Ctrl Pts',(5.33966402241091,19.6303335366024,-7.59758426882942)) ;
#36359=CARTESIAN_POINT('Ctrl Pts',(4.77460210253822,19.7753678214987,-7.58299197760067)) ;
#36360=CARTESIAN_POINT('Ctrl Pts',(3.48538919668097,20.0477841143969,-7.54970849235954)) ;
#36361=CARTESIAN_POINT('Ctrl Pts',(2.75898443028803,20.1605948129092,-7.53095335906623)) ;
#36362=CARTESIAN_POINT('Ctrl Pts',(1.60749515412967,20.2760107404773,-7.50157565350564)) ;
#36363=CARTESIAN_POINT('Ctrl Pts',(1.18569852694703,20.3050430929132,-7.49089351167923)) ;
#36364=CARTESIAN_POINT('Ctrl Pts',(0.391163179234408,20.334887761987,-7.47107658945271)) ;
#36365=CARTESIAN_POINT('Ctrl Pts',(0.0187096304971401,20.3386410462601,
-7.46192636134628)) ;
#36366=CARTESIAN_POINT('Ctrl Pts',(-0.957969681235675,20.3216536893527,
-7.43807945923731)) ;
#36367=CARTESIAN_POINT('Ctrl Pts',(-1.56153474184536,20.2842038945325,-7.42348050899772)) ;
#36368=CARTESIAN_POINT('Ctrl Pts',(-2.84926844815383,20.14647991131,-7.39201967694105)) ;
#36369=CARTESIAN_POINT('Ctrl Pts',(-3.53180938168843,20.0380961108315,-7.37514712359831)) ;
#36370=CARTESIAN_POINT('Ctrl Pts',(-4.80589160842951,19.7686486728442,-7.34285740243697)) ;
#36371=CARTESIAN_POINT('Ctrl Pts',(-5.39825754073355,19.6151693824441,-7.32751406300869)) ;
#36372=CARTESIAN_POINT('Ctrl Pts',(-6.79895095392575,19.1839900707252,-7.29042060741557)) ;
#36373=CARTESIAN_POINT('Ctrl Pts',(-7.59846294567933,18.881593238979,-7.26855803393727)) ;
#36374=CARTESIAN_POINT('Ctrl Pts',(-8.68544689161686,18.3902116635167,-7.2384580283756)) ;
#36375=CARTESIAN_POINT('Ctrl Pts',(-8.99076791818554,18.2428882224929,-7.22996984157808)) ;
#36376=CARTESIAN_POINT('Ctrl Pts',(-9.42613706030807,18.0192279668962,-7.21786500247111)) ;
#36377=CARTESIAN_POINT('Ctrl Pts',(-9.55923899426645,17.9489717389519,-7.21416106077178)) ;
#36378=CARTESIAN_POINT('Ctrl Pts',(-10.0674837841138,17.6734438538954,-7.19998303249942)) ;
#36379=CARTESIAN_POINT('Ctrl Pts',(-10.4368979716341,17.4578352277467,-7.18960248119923)) ;
#36380=CARTESIAN_POINT('Ctrl Pts',(-11.5875986240165,16.7366420037633,-7.15666140785297)) ;
#36381=CARTESIAN_POINT('Ctrl Pts',(-12.3411126403601,16.1890257351276,-7.13412054761323)) ;
#36382=CARTESIAN_POINT('Ctrl Pts',(-13.501895699122,15.2171388177069,-7.09664864954409)) ;
#36383=CARTESIAN_POINT('Ctrl Pts',(-13.9329787510482,14.8234474888726,-7.08204510994786)) ;
#36384=CARTESIAN_POINT('Ctrl Pts',(-14.8683485479531,13.8923117024224,-7.0487062932591)) ;
#36385=CARTESIAN_POINT('Ctrl Pts',(-15.3615675319116,13.3448997181919,-7.02990641066344)) ;
#36386=CARTESIAN_POINT('Ctrl Pts',(-16.0892022183127,12.4433854765112,-7.00049846000239)) ;
#36387=CARTESIAN_POINT('Ctrl Pts',(-16.3441004827617,12.1066367480222,-6.98982903363529)) ;
#36388=CARTESIAN_POINT('Ctrl Pts',(-16.8056078946816,11.4557686780552,-6.96994612776944)) ;
#36389=CARTESIAN_POINT('Ctrl Pts',(-17.0143525322356,11.1433792677009,-6.96071894253681)) ;
#36390=CARTESIAN_POINT('Ctrl Pts',(-17.5427302432451,10.3031630980202,-6.93649330215191)) ;
#36391=CARTESIAN_POINT('Ctrl Pts',(-17.8472025903495,9.7662642678522,-6.9215962342594)) ;
#36392=CARTESIAN_POINT('Ctrl Pts',(-18.4375850322338,8.60509571756327,-6.88994271837802)) ;
#36393=CARTESIAN_POINT('Ctrl Pts',(-18.7172530796746,7.97851119947298,-6.87318002593854)) ;
#36394=CARTESIAN_POINT('Ctrl Pts',(-19.189241589446,6.75884458700106,-6.84073651545719)) ;
#36395=CARTESIAN_POINT('Ctrl Pts',(-19.3870100099025,6.16869558480859,-6.82511927024866)) ;
#36396=CARTESIAN_POINT('Ctrl Pts',(-19.8397625058855,4.57910718211882,-6.78326233391622)) ;
#36397=CARTESIAN_POINT('Ctrl Pts',(-20.0463315664789,3.5677699205246,-6.75679062883414)) ;
#36398=CARTESIAN_POINT('Ctrl Pts',(-20.218677211945,2.20158745389991,-6.72240952422769)) ;
#36399=CARTESIAN_POINT('Ctrl Pts',(-20.2532348093798,1.85698015649438,-6.71387704507936)) ;
#36400=CARTESIAN_POINT('Ctrl Pts',(-20.3166990478875,1.00560412832394,-6.69299285041195)) ;
#36401=CARTESIAN_POINT('Ctrl Pts',(-20.3354662319348,0.498313472598733,
-6.68070877754043)) ;
#36402=CARTESIAN_POINT('Ctrl Pts',(-20.334889551072,-0.783581673061414,
-6.64961551101604)) ;
#36403=CARTESIAN_POINT('Ctrl Pts',(-20.2903021214652,-1.55735749048991,
-6.63078127140845)) ;
#36404=CARTESIAN_POINT('Ctrl Pts',(-20.1358720522922,-2.89820559516594,
-6.59739731442196)) ;
#36405=CARTESIAN_POINT('Ctrl Pts',(-20.0458278439741,-3.4666578185139,-6.58301337638405)) ;
#36406=CARTESIAN_POINT('Ctrl Pts',(-19.7924843776348,-4.71949604009386,
-6.5507507945064)) ;
#36407=CARTESIAN_POINT('Ctrl Pts',(-19.6175340056101,-5.40078076590417,
-6.53282035727844)) ;
#36408=CARTESIAN_POINT('Ctrl Pts',(-19.2687971071472,-6.51550049506038,
-6.5031387050621)) ;
#36409=CARTESIAN_POINT('Ctrl Pts',(-19.1147465052204,-6.95447763417581,
-6.49136322954928)) ;
#36410=CARTESIAN_POINT('Ctrl Pts',(-18.8163646253583,-7.71966982779728,
-6.47087234604565)) ;
#36411=CARTESIAN_POINT('Ctrl Pts',(-18.6782510680693,-8.04809400935234,
-6.46210547202084)) ;
#36412=CARTESIAN_POINT('Ctrl Pts',(-18.3076446776743,-8.86836772680735,
-6.44010590062631)) ;
#36413=CARTESIAN_POINT('Ctrl Pts',(-18.063911901196,-9.3548324491682,-6.42695250827293)) ;
#36414=CARTESIAN_POINT('Ctrl Pts',(-17.4533573106967,-10.4603689719171,
-6.39630676388711)) ;
#36415=CARTESIAN_POINT('Ctrl Pts',(-17.0726065157728,-11.0709122222924,
-6.37879254438756)) ;
#36416=CARTESIAN_POINT('Ctrl Pts',(-16.3298588994978,-12.1321826127183,
-6.34674976342576)) ;
#36417=CARTESIAN_POINT('Ctrl Pts',(-15.9794738373463,-12.590097452661,-6.3323378287567)) ;
#36418=CARTESIAN_POINT('Ctrl Pts',(-15.1569095298164,-13.5753509782339,
-6.29993835103382)) ;
#36419=CARTESIAN_POINT('Ctrl Pts',(-14.6756963033449,-14.0941828888234,
-6.28189740023685)) ;
#36420=CARTESIAN_POINT('Ctrl Pts',(-13.8377803886648,-14.9080618490359,
-6.25221642321969)) ;
#36421=CARTESIAN_POINT('Ctrl Pts',(-13.4962940054707,-15.2179015218636,
-6.240548290746)) ;
#36422=CARTESIAN_POINT('Ctrl Pts',(-12.8699771114681,-15.7484981462581,
-6.22007382416863)) ;
#36423=CARTESIAN_POINT('Ctrl Pts',(-12.5892545875132,-15.9737964779749,
-6.21122027333049)) ;
#36424=CARTESIAN_POINT('Ctrl Pts',(-11.8588835448729,-16.5287495145717,
-6.18880728908166)) ;
#36425=CARTESIAN_POINT('Ctrl Pts',(-11.4013871290171,-16.8475830490838,
-6.17533136794391)) ;
#36426=CARTESIAN_POINT('Ctrl Pts',(-10.3366323470895,-17.5263653729688,
-6.14468452283959)) ;
#36427=CARTESIAN_POINT('Ctrl Pts',(-9.72257543638125,-17.8743103011633,
-6.12749428948782)) ;
#36428=CARTESIAN_POINT('Ctrl Pts',(-8.57341777328908,-18.4486910524161,
-6.09570658249754)) ;
#36429=CARTESIAN_POINT('Ctrl Pts',(-8.04431764871778,-18.6854659739644,
-6.08121286554617)) ;
#36430=CARTESIAN_POINT('Ctrl Pts',(-6.83707999963106,-19.1649183674483,
-6.04841314798866)) ;
#36431=CARTESIAN_POINT('Ctrl Pts',(-6.15470096420743,-19.3948294029144,
-6.03004899612453)) ;
#36432=CARTESIAN_POINT('Ctrl Pts',(-5.03386769216678,-19.7073418079305,
-6.00049496899895)) ;
#36433=CARTESIAN_POINT('Ctrl Pts',(-4.60236216404437,-19.8125569209369,
-5.98926378685334)) ;
#36434=CARTESIAN_POINT('Ctrl Pts',(-3.80954984437051,-19.9785698825362,
-5.9690676990184)) ;
#36435=CARTESIAN_POINT('Ctrl Pts',(-3.44938261443551,-20.0438939486088,
-5.9600699193788)) ;
#36436=CARTESIAN_POINT('Ctrl Pts',(-2.51429977879769,-20.1875399508006,
-5.93696433519843)) ;
#36437=CARTESIAN_POINT('Ctrl Pts',(-1.93744315322656,-20.2510441802163,
-5.92294697681138)) ;
#36438=CARTESIAN_POINT('Ctrl Pts',(-0.635491093403947,-20.3382264991574,
-5.89126431651432)) ;
#36439=CARTESIAN_POINT('Ctrl Pts',(0.0897453550806687,-20.3479542121509,
-5.8735748440604)) ;
#36440=CARTESIAN_POINT('Ctrl Pts',(1.42352942581411,-20.2945248130426,-5.84047966504807)) ;
#36441=CARTESIAN_POINT('Ctrl Pts',(2.0316997923572,-20.2426865635556,-5.8251769070561)) ;
#36442=CARTESIAN_POINT('Ctrl Pts',(3.19842593928037,-20.0901241217493,-5.79539823306841)) ;
#36443=CARTESIAN_POINT('Ctrl Pts',(3.7569215023495,-19.9932126866801,-5.78095573007756)) ;
#36444=CARTESIAN_POINT('Ctrl Pts',(4.8247207349255,-19.7615984010064,-5.75317452714807)) ;
#36445=CARTESIAN_POINT('Ctrl Pts',(5.33428659815078,-19.6301832425762,-5.73984266301656)) ;
#36446=CARTESIAN_POINT('Ctrl Pts',(6.20531554825694,-19.3691233047096,-5.71719187551594)) ;
#36447=CARTESIAN_POINT('Ctrl Pts',(6.56926329430078,-19.2487313784905,-5.70778343914778)) ;
#36448=CARTESIAN_POINT('Ctrl Pts',(7.5377477943781,-18.8976926946415,-5.68265164402447)) ;
#36449=CARTESIAN_POINT('Ctrl Pts',(8.13504068305113,-18.6483658256576,-5.66703828743495)) ;
#36450=CARTESIAN_POINT('Ctrl Pts',(9.32515255716397,-18.0835025278383,-5.63500288632133)) ;
#36451=CARTESIAN_POINT('Ctrl Pts',(9.91627795033413,-17.7662307555444,-5.61858951222894)) ;
#36452=CARTESIAN_POINT('Ctrl Pts',(11.0466583143976,-17.0855081643718,-5.58582086193217)) ;
#36453=CARTESIAN_POINT('Ctrl Pts',(11.5863165201075,-16.7242490655957,-5.56950011778613)) ;
#36454=CARTESIAN_POINT('Ctrl Pts',(12.7483411379843,-15.8630853188755,-5.53282697474644)) ;
#36455=CARTESIAN_POINT('Ctrl Pts',(13.3604378352449,-15.3511034160689,-5.51242739080587)) ;
#36456=CARTESIAN_POINT('Ctrl Pts',(14.1818258335732,-14.5776310115413,-5.48398528020362)) ;
#36457=CARTESIAN_POINT('Ctrl Pts',(14.4171882564254,-14.3449014606328,-5.47570885832489)) ;
#36458=CARTESIAN_POINT('Ctrl Pts',(15.0760440458305,-13.660813311538,-5.45224112912472)) ;
#36459=CARTESIAN_POINT('Ctrl Pts',(15.4847529342396,-13.1957327042059,-5.43724555280852)) ;
#36460=CARTESIAN_POINT('Ctrl Pts',(16.4138990550934,-12.0357109092044,-5.40120091548751)) ;
#36461=CARTESIAN_POINT('Ctrl Pts',(16.9123007715931,-11.3246849799612,-5.38015222413626)) ;
#36462=CARTESIAN_POINT('Ctrl Pts',(17.6373946762965,-10.1351205510364,-5.34568057294485)) ;
#36463=CARTESIAN_POINT('Ctrl Pts',(17.893492917947,-9.67580597644696,-5.33254408539732)) ;
#36464=CARTESIAN_POINT('Ctrl Pts',(18.1314964428552,-9.20710717871412,-5.31929120111857)) ;
#36465=CARTESIAN_POINT('Ctrl Pts',(18.1314964277493,-9.20710720846216,-4.68087293438847)) ;
#36466=CARTESIAN_POINT('Ctrl Pts',(18.0523186452368,-9.36303150132383,-4.68530784267373)) ;
#36467=CARTESIAN_POINT('Ctrl Pts',(17.9711228049512,-9.51794767764142,-4.6897511590617)) ;
#36468=CARTESIAN_POINT('Ctrl Pts',(17.6266893201308,-10.1549739633927,-4.70816687118514)) ;
#36469=CARTESIAN_POINT('Ctrl Pts',(17.3459827772761,-10.6273494016093,-4.7221755114788)) ;
#36470=CARTESIAN_POINT('Ctrl Pts',(16.8514746170197,-11.3876126790035,-4.74509759838492)) ;
#36471=CARTESIAN_POINT('Ctrl Pts',(16.6485719905417,-11.6822504765265,-4.75407572346182)) ;
#36472=CARTESIAN_POINT('Ctrl Pts',(16.1645160437808,-12.3469113555224,-4.7744420263802)) ;
#36473=CARTESIAN_POINT('Ctrl Pts',(15.8782408678854,-12.7129568319709,-4.78576912166363)) ;
#36474=CARTESIAN_POINT('Ctrl Pts',(15.1272276196611,-13.6082552580042,-4.81416040569896)) ;
#36475=CARTESIAN_POINT('Ctrl Pts',(14.6470714677209,-14.1237715717995,-4.83116467092485)) ;
#36476=CARTESIAN_POINT('Ctrl Pts',(13.7275412161976,-15.0135893299879,-4.86244627437124)) ;
#36477=CARTESIAN_POINT('Ctrl Pts',(13.2971302422379,-15.3960894973893,-4.87663709220211)) ;
#36478=CARTESIAN_POINT('Ctrl Pts',(12.2923176824295,-16.2154471370018,-4.90898445864983)) ;
#36479=CARTESIAN_POINT('Ctrl Pts',(11.7097251327719,-16.6410373002128,-4.92722230095032)) ;
#36480=CARTESIAN_POINT('Ctrl Pts',(10.6522173054578,-17.3304759122839,-4.95932864520367)) ;
#36481=CARTESIAN_POINT('Ctrl Pts',(10.1870366082399,-17.6079361468506,-4.97313551388248)) ;
#36482=CARTESIAN_POINT('Ctrl Pts',(9.39895532900243,-18.0362978148204,-4.99580215751323)) ;
#36483=CARTESIAN_POINT('Ctrl Pts',(9.08216866487118,-18.1978740154346,-5.00472479228085)) ;
#36484=CARTESIAN_POINT('Ctrl Pts',(8.34142296047336,-18.5515264932037,-5.0250532362406)) ;
#36485=CARTESIAN_POINT('Ctrl Pts',(7.91478173495953,-18.7375213898214,-5.03639671589767)) ;
#36486=CARTESIAN_POINT('Ctrl Pts',(6.82898138842262,-19.1671699920706,-5.06476550979927)) ;
#36487=CARTESIAN_POINT('Ctrl Pts',(6.16287660469016,-19.3916049762649,-5.08173233593433)) ;
#36488=CARTESIAN_POINT('Ctrl Pts',(4.93266189503718,-19.7363027731233,-5.11296674033377)) ;
#36489=CARTESIAN_POINT('Ctrl Pts',(4.37249641020224,-19.8679155362104,-5.12714855901422)) ;
#36490=CARTESIAN_POINT('Ctrl Pts',(3.09846408611006,-20.1107562768848,-5.15950800860268)) ;
#36491=CARTESIAN_POINT('Ctrl Pts',(2.3827303204123,-20.2080572831549,-5.17776777172363)) ;
#36492=CARTESIAN_POINT('Ctrl Pts',(1.12488481625565,-20.3112903407755,-5.20986644447541)) ;
#36493=CARTESIAN_POINT('Ctrl Pts',(0.584874102586749,-20.3340061177622,
-5.22364359864288)) ;
#36494=CARTESIAN_POINT('Ctrl Pts',(-0.310632077300816,-20.3359702145692,
-5.24627261087276)) ;
#36495=CARTESIAN_POINT('Ctrl Pts',(-0.665828451570617,-20.3274409486539,
-5.25518705775032)) ;
#36496=CARTESIAN_POINT('Ctrl Pts',(-1.48540360645998,-20.2862546658499,
-5.27550939406321)) ;
#36497=CARTESIAN_POINT('Ctrl Pts',(-1.94924850372538,-20.2469500918845,
-5.28685478750299)) ;
#36498=CARTESIAN_POINT('Ctrl Pts',(-3.10858582711033,-20.1084998925431,
-5.31521995017413)) ;
#36499=CARTESIAN_POINT('Ctrl Pts',(-3.80105142593879,-19.9891740977748,
-5.33218143203738)) ;
#36500=CARTESIAN_POINT('Ctrl Pts',(-5.04689461541006,-19.7073993924063,
-5.36340910001509)) ;
#36501=CARTESIAN_POINT('Ctrl Pts',(-5.60219651994496,-19.5567922296115,
-5.37758963507189)) ;
#36502=CARTESIAN_POINT('Ctrl Pts',(-6.88185689440415,-19.1507438043911,
-5.41108617195795)) ;
#36503=CARTESIAN_POINT('Ctrl Pts',(-7.59961829259005,-18.8774131380579,
-5.43051941813763)) ;
#36504=CARTESIAN_POINT('Ctrl Pts',(-8.76716071463369,-18.3553947435915,
-5.46305851184877)) ;
#36505=CARTESIAN_POINT('Ctrl Pts',(-9.22607405494234,-18.1290700920658,
-5.47609430972741)) ;
#36506=CARTESIAN_POINT('Ctrl Pts',(-9.98149972271132,-17.7203928156439,
-5.49778391185284)) ;
#36507=CARTESIAN_POINT('Ctrl Pts',(-10.2827520333698,-17.5472982222961,
-5.5064932719995)) ;
#36508=CARTESIAN_POINT('Ctrl Pts',(-11.4618939357414,-16.8289845265552,
-5.54066571611911)) ;
#36509=CARTESIAN_POINT('Ctrl Pts',(-12.3021110078318,-16.2249142478387,
-5.56541565375218)) ;
#36510=CARTESIAN_POINT('Ctrl Pts',(-13.5683529946967,-15.1594227991939,
-5.6057400748679)) ;
#36511=CARTESIAN_POINT('Ctrl Pts',(-14.0253292971861,-14.7376535327089,
-5.62100081478672)) ;
#36512=CARTESIAN_POINT('Ctrl Pts',(-14.944566972909,-13.8077001509719,-5.653529486803)) ;
#36513=CARTESIAN_POINT('Ctrl Pts',(-15.4018613095405,-13.2956880269988,
-5.67082389327669)) ;
#36514=CARTESIAN_POINT('Ctrl Pts',(-16.2191211190515,-12.2817686118603,
-5.7038957899571)) ;
#36515=CARTESIAN_POINT('Ctrl Pts',(-16.5838349768186,-11.7846572875102,
-5.71962798801488)) ;
#36516=CARTESIAN_POINT('Ctrl Pts',(-17.1335305179989,-10.9592468818078,
-5.74472164879162)) ;
#36517=CARTESIAN_POINT('Ctrl Pts',(-17.3329570886999,-10.6410321419026,
-5.75416185539592)) ;
#36518=CARTESIAN_POINT('Ctrl Pts',(-17.7374233266058,-9.95407646846906,
-5.77392877806474)) ;
#36519=CARTESIAN_POINT('Ctrl Pts',(-17.9400311561078,-9.58410721721756,
-5.78423300381752)) ;
#36520=CARTESIAN_POINT('Ctrl Pts',(-18.4644945166908,-8.5514256546696,-5.81240688096996)) ;
#36521=CARTESIAN_POINT('Ctrl Pts',(-18.7620766322954,-7.87711369197664,
-5.83017715348359)) ;
#36522=CARTESIAN_POINT('Ctrl Pts',(-19.2287110709534,-6.64223127829799,
-5.86242550382837)) ;
#36523=CARTESIAN_POINT('Ctrl Pts',(-19.4114029600428,-6.08769191180265,
-5.87680124775349)) ;
#36524=CARTESIAN_POINT('Ctrl Pts',(-19.8231473315249,-4.62954228969047,
-5.914577844863)) ;
#36525=CARTESIAN_POINT('Ctrl Pts',(-20.0143957853065,-3.71668696132871,
-5.93824202395825)) ;
#36526=CARTESIAN_POINT('Ctrl Pts',(-20.2234612532234,-2.20947709836345,
-5.97696244300309)) ;
#36527=CARTESIAN_POINT('Ctrl Pts',(-20.2790564039257,-1.62174353473886,
-5.99196018620084)) ;
#36528=CARTESIAN_POINT('Ctrl Pts',(-20.3267009554494,-0.684518342453904,
-6.01538700183379)) ;
#36529=CARTESIAN_POINT('Ctrl Pts',(-20.3354443265445,-0.336215972824135,
-6.02396830376446)) ;
#36530=CARTESIAN_POINT('Ctrl Pts',(-20.3347696017134,0.794075410618914,
-6.05161225316834)) ;
#36531=CARTESIAN_POINT('Ctrl Pts',(-20.2892024562884,1.57533590928818,-6.07044353448938)) ;
#36532=CARTESIAN_POINT('Ctrl Pts',(-20.125404454939,2.98200010873307,-6.10492983665134)) ;
#36533=CARTESIAN_POINT('Ctrl Pts',(-20.0226171098174,3.60818844230698,-6.12048853700425)) ;
#36534=CARTESIAN_POINT('Ctrl Pts',(-19.6292478759167,5.45856606542675,-6.16752322739209)) ;
#36535=CARTESIAN_POINT('Ctrl Pts',(-19.2542282705926,6.6616758845014,-6.1996678371757)) ;
#36536=CARTESIAN_POINT('Ctrl Pts',(-18.61196560671,8.20284094613253,-6.24199141751562)) ;
#36537=CARTESIAN_POINT('Ctrl Pts',(-18.4418872135962,8.57838358101396,-6.25238086663229)) ;
#36538=CARTESIAN_POINT('Ctrl Pts',(-18.0609437410463,9.35574548362379,-6.27388110292608)) ;
#36539=CARTESIAN_POINT('Ctrl Pts',(-17.847805435031,9.75620362594056,-6.28496129213293)) ;
#36540=CARTESIAN_POINT('Ctrl Pts',(-17.2563467729632,10.7831180846691,-6.31378211727741)) ;
#36541=CARTESIAN_POINT('Ctrl Pts',(-16.8572979835043,11.3968699716414,-6.33143517742053)) ;
#36542=CARTESIAN_POINT('Ctrl Pts',(-16.0827391690205,12.4581955234338,-6.36353552931055)) ;
#36543=CARTESIAN_POINT('Ctrl Pts',(-15.7193838906015,12.913639955258,-6.37788293923393)) ;
#36544=CARTESIAN_POINT('Ctrl Pts',(-14.7405317272159,14.0379416997429,-6.41505324288756)) ;
#36545=CARTESIAN_POINT('Ctrl Pts',(-14.0988491451116,14.6822854666767,-6.43811631393356)) ;
#36546=CARTESIAN_POINT('Ctrl Pts',(-12.9467303015985,15.6937736613283,-6.47713198858411)) ;
#36547=CARTESIAN_POINT('Ctrl Pts',(-12.458456000942,16.0841300303486,-6.49302121782243)) ;
#36548=CARTESIAN_POINT('Ctrl Pts',(-11.6606791644631,16.6637659195397,-6.51761543908738)) ;
#36549=CARTESIAN_POINT('Ctrl Pts',(-11.3627651222621,16.8683165221969,-6.52650274465454)) ;
#36550=CARTESIAN_POINT('Ctrl Pts',(-10.3698062090231,17.5118444081389,-6.55541133735499)) ;
#36551=CARTESIAN_POINT('Ctrl Pts',(-9.65358337859131,17.9166378537394,-6.5751955799527)) ;
#36552=CARTESIAN_POINT('Ctrl Pts',(-8.37157240397254,18.541955280397,-6.60998648575256)) ;
#36553=CARTESIAN_POINT('Ctrl Pts',(-7.81677440872748,18.7825812750195,-6.62484670724638)) ;
#36554=CARTESIAN_POINT('Ctrl Pts',(-6.58903079019188,19.2512432320273,-6.65756666678475)) ;
#36555=CARTESIAN_POINT('Ctrl Pts',(-5.91318352347607,19.4694616933211,-6.67548142331575)) ;
#36556=CARTESIAN_POINT('Ctrl Pts',(-4.66227799181143,19.8021971452917,-6.7083763207331)) ;
#36557=CARTESIAN_POINT('Ctrl Pts',(-4.09101684857812,19.9280563423746,-6.72329708712856)) ;
#36558=CARTESIAN_POINT('Ctrl Pts',(-3.15345603968111,20.0925990500634,-6.747371142373)) ;
#36559=CARTESIAN_POINT('Ctrl Pts',(-2.79012676745793,20.146265670974,-6.75659687764503)) ;
#36560=CARTESIAN_POINT('Ctrl Pts',(-1.9877004539964,20.2426654098935,-6.77662748053633)) ;
#36561=CARTESIAN_POINT('Ctrl Pts',(-1.54826285545236,20.2810094184567,-6.78739245042025)) ;
#36562=CARTESIAN_POINT('Ctrl Pts',(-0.38714765283173,20.344364544381,-6.81566218836829)) ;
#36563=CARTESIAN_POINT('Ctrl Pts',(0.335211131801346,20.3452865751508,-6.83308674848994)) ;
#36564=CARTESIAN_POINT('Ctrl Pts',(1.63527276899067,20.2776781940589,-6.86489862269561)) ;
#36565=CARTESIAN_POINT('Ctrl Pts',(2.21290108733795,20.2227943351447,-6.87919080054629)) ;
#36566=CARTESIAN_POINT('Ctrl Pts',(3.47797413104281,20.0477360726295,-6.91104179026425)) ;
#36567=CARTESIAN_POINT('Ctrl Pts',(4.16318287476264,19.9167246434693,-6.92866206780184)) ;
#36568=CARTESIAN_POINT('Ctrl Pts',(5.38764960139512,19.6166459994107,-6.96071356446155)) ;
#36569=CARTESIAN_POINT('Ctrl Pts',(5.92918512910822,19.459813287763,-6.9750900514938)) ;
#36570=CARTESIAN_POINT('Ctrl Pts',(6.80629938240583,19.1657764570306,-6.99847733107374)) ;
#36571=CARTESIAN_POINT('Ctrl Pts',(7.14597084944364,19.0417385068789,-7.00755602325346)) ;
#36572=CARTESIAN_POINT('Ctrl Pts',(7.9061950747109,18.7409184964848,-7.02781200001761)) ;
#36573=CARTESIAN_POINT('Ctrl Pts',(8.32447040222371,18.5589101101451,-7.03893602336652)) ;
#36574=CARTESIAN_POINT('Ctrl Pts',(9.3780620912044,18.0576592430295,-7.06728932490813)) ;
#36575=CARTESIAN_POINT('Ctrl Pts',(10.0034004445994,17.7188906304676,-7.08445150867794)) ;
#36576=CARTESIAN_POINT('Ctrl Pts',(11.1021413708814,17.046924060357,-7.11593227583205)) ;
#36577=CARTESIAN_POINT('Ctrl Pts',(11.5815164450668,16.7249404127619,-7.13016111803944)) ;
#36578=CARTESIAN_POINT('Ctrl Pts',(12.7094391931464,15.8955706239743,-7.16508529626908)) ;
#36579=CARTESIAN_POINT('Ctrl Pts',(13.3421363363681,15.3683566612708,-7.18594311988888)) ;
#36580=CARTESIAN_POINT('Ctrl Pts',(14.4143475351795,14.3586581388065,-7.22342331023085)) ;
#36581=CARTESIAN_POINT('Ctrl Pts',(14.8659146446333,13.8906107296394,-7.23998367067229)) ;
#36582=CARTESIAN_POINT('Ctrl Pts',(15.510166803466,13.1553794517549,-7.26444036775844)) ;
#36583=CARTESIAN_POINT('Ctrl Pts',(15.7200563570076,12.9038409519787,-7.27253713703068)) ;
#36584=CARTESIAN_POINT('Ctrl Pts',(16.4219456576386,12.020118921661,-7.3002052098067)) ;
#36585=CARTESIAN_POINT('Ctrl Pts',(16.8826186394949,11.3640115498233,-7.31948819747828)) ;
#36586=CARTESIAN_POINT('Ctrl Pts',(17.6463459583452,10.1269282207857,-7.35486440420772)) ;
#36587=CARTESIAN_POINT('Ctrl Pts',(17.9623464898602,9.5552236829556,-7.37086172866693)) ;
#36588=CARTESIAN_POINT('Ctrl Pts',(18.5440448238941,8.371614000146,-7.40363032436401)) ;
#36589=CARTESIAN_POINT('Ctrl Pts',(18.8082497509511,7.75984845441656,-7.42039169249166)) ;
#36590=CARTESIAN_POINT('Ctrl Pts',(19.3308247553459,6.36543532668595,-7.45817300001808)) ;
#36591=CARTESIAN_POINT('Ctrl Pts',(19.5726222530227,5.57781409248115,-7.47924057867345)) ;
#36592=CARTESIAN_POINT('Ctrl Pts',(19.7993282149357,4.63990184905076,-7.50350100928927)) ;
#36593=CARTESIAN_POINT('Ctrl Pts',(19.8311966017323,4.50174726995194,-7.50705295132518)) ;
#36594=CARTESIAN_POINT('Ctrl Pts',(19.9399615148408,4.00664911744195,-7.51969236259956)) ;
#36595=CARTESIAN_POINT('Ctrl Pts',(20.0086863129187,3.64798229709993,-7.52866996891407)) ;
#36596=CARTESIAN_POINT('Ctrl Pts',(20.199868287735,2.48101672171897,-7.55755264345226)) ;
#36597=CARTESIAN_POINT('Ctrl Pts',(20.2832635636153,1.66713831158843,-7.57722974781153)) ;
#36598=CARTESIAN_POINT('Ctrl Pts',(20.3426798402346,0.247673027358125,-7.61188471003829)) ;
#36599=CARTESIAN_POINT('Ctrl Pts',(20.3410735553585,-0.355925594235231,
-7.62671854096718)) ;
#36600=CARTESIAN_POINT('Ctrl Pts',(20.2791764547102,-1.66758078837585,-7.65941473943478)) ;
#36601=CARTESIAN_POINT('Ctrl Pts',(20.2086171861824,-2.3743630890629,-7.6773329384659)) ;
#36602=CARTESIAN_POINT('Ctrl Pts',(20.0129875733312,-3.65277631698287,-7.71020049598997)) ;
#36603=CARTESIAN_POINT('Ctrl Pts',(19.8999425410213,-4.22548623332871,-7.72509039010834)) ;
#36604=CARTESIAN_POINT('Ctrl Pts',(19.6759621555885,-5.14908738348592,-7.74912554701932)) ;
#36605=CARTESIAN_POINT('Ctrl Pts',(19.5798626614912,-5.50323287449455,-7.75834300526929)) ;
#36606=CARTESIAN_POINT('Ctrl Pts',(19.3470476572957,-6.27765007180376,-7.77838462815951)) ;
#36607=CARTESIAN_POINT('Ctrl Pts',(19.2061083955231,-6.69645792239567,-7.78916819527272)) ;
#36608=CARTESIAN_POINT('Ctrl Pts',(18.7994464817941,-7.78607832377935,-7.81744195033205)) ;
#36609=CARTESIAN_POINT('Ctrl Pts',(18.5114810466438,-8.44791532986397,-7.83485265313227)) ;
#36610=CARTESIAN_POINT('Ctrl Pts',(18.1699267787802,-9.13113132033814,-7.85351834323284)) ;
#36611=CARTESIAN_POINT('Ctrl Pts',(18.1507709233616,-9.16915006932015,-7.85455929226164)) ;
#36612=CARTESIAN_POINT('Ctrl Pts',(18.1314964390739,-9.20710718616059,-7.85560087779543)) ;
#36613=CARTESIAN_POINT('Origin',(0.,0.,5.8748638224677)) ;
#36614=CARTESIAN_POINT('',(18.1314964616813,-9.20710714163998,-11.6687558734427)) ;
#36615=CARTESIAN_POINT('',(18.1314964420815,-9.20710718023772,-11.0322347276753)) ;
#36616=CARTESIAN_POINT('',(18.1314964405232,-9.20710718330643,5.8748638224677)) ;
#36617=CARTESIAN_POINT('Ctrl Pts',(18.1314964616938,-9.20710714161542,-11.6687558745767)) ;
#36618=CARTESIAN_POINT('Ctrl Pts',(18.2644739001709,-8.94523553328637,-11.6616247551653)) ;
#36619=CARTESIAN_POINT('Ctrl Pts',(18.391785753033,-8.68046790628738,-11.6544792653389)) ;
#36620=CARTESIAN_POINT('Ctrl Pts',(18.7543475034272,-7.88262674001481,-11.6330691624918)) ;
#36621=CARTESIAN_POINT('Ctrl Pts',(18.9724551492615,-7.34215854648363,-11.6187174011085)) ;
#36622=CARTESIAN_POINT('Ctrl Pts',(19.471581392229,-5.93384513506377,-11.5814618845947)) ;
#36623=CARTESIAN_POINT('Ctrl Pts',(19.7179811697906,-5.0551151568954,-11.5583147733356)) ;
#36624=CARTESIAN_POINT('Ctrl Pts',(20.0250982014908,-3.58663586093282,-11.5201361262327)) ;
#36625=CARTESIAN_POINT('Ctrl Pts',(20.1205283548207,-3.00547161251361,-11.5051669123351)) ;
#36626=CARTESIAN_POINT('Ctrl Pts',(20.2305155847466,-2.08819683527602,-11.4820760342017)) ;
#36627=CARTESIAN_POINT('Ctrl Pts',(20.2621849322976,-1.75447676518937,-11.4738035306207)) ;
#36628=CARTESIAN_POINT('Ctrl Pts',(20.3409804622817,-0.628929714393546,
-11.4461703104481)) ;
#36629=CARTESIAN_POINT('Ctrl Pts',(20.3500339446608,0.164827882851609,-11.4270738833638)) ;
#36630=CARTESIAN_POINT('Ctrl Pts',(20.2823537764486,1.60123956804531,-11.3920719691454)) ;
#36631=CARTESIAN_POINT('Ctrl Pts',(20.2213791806036,2.24358135100497,-11.3762627454793)) ;
#36632=CARTESIAN_POINT('Ctrl Pts',(19.9496333159388,4.14169546660323,-11.3286069890023)) ;
#36633=CARTESIAN_POINT('Ctrl Pts',(19.651419904358,5.38173937783459,-11.2960738940596)) ;
#36634=CARTESIAN_POINT('Ctrl Pts',(19.1067732956969,6.97284908097476,-11.2534486205041)) ;
#36635=CARTESIAN_POINT('Ctrl Pts',(18.9626035307604,7.35588764401761,-11.2431363222837)) ;
#36636=CARTESIAN_POINT('Ctrl Pts',(18.6320535515641,8.15966182634198,-11.2215538952151)) ;
#36637=CARTESIAN_POINT('Ctrl Pts',(18.4427515604126,8.57895223271918,-11.2103208887694)) ;
#36638=CARTESIAN_POINT('Ctrl Pts',(17.9179044953875,9.64361666003351,-11.181458000497)) ;
#36639=CARTESIAN_POINT('Ctrl Pts',(17.5616689415133,10.2780556717329,-11.1639099260452)) ;
#36640=CARTESIAN_POINT('Ctrl Pts',(16.8608830349276,11.3829028430115,-11.131942139304)) ;
#36641=CARTESIAN_POINT('Ctrl Pts',(16.528643529125,11.860176595648,-11.1176201230084)) ;
#36642=CARTESIAN_POINT('Ctrl Pts',(15.636803814885,13.030937675594,-11.0809191550807)) ;
#36643=CARTESIAN_POINT('Ctrl Pts',(15.0512450284891,13.7031005982243,-11.0583171485039)) ;
#36644=CARTESIAN_POINT('Ctrl Pts',(13.9984070067423,14.762462134288,-11.020307225313)) ;
#36645=CARTESIAN_POINT('Ctrl Pts',(13.5544664991448,15.1710952507671,-11.0049643258568)) ;
#36646=CARTESIAN_POINT('Ctrl Pts',(12.8382133778352,15.7738126559706,-10.9815614086281)) ;
#36647=CARTESIAN_POINT('Ctrl Pts',(12.5781798297473,15.9819360770221,-10.9733388808027)) ;
#36648=CARTESIAN_POINT('Ctrl Pts',(11.6802940609545,16.6650852530905,-10.9457000993399)) ;
#36649=CARTESIAN_POINT('Ctrl Pts',(11.0197383572832,17.1090535624009,-10.9265544041125)) ;
#36650=CARTESIAN_POINT('Ctrl Pts',(9.77772819691337,17.8419881207972,-10.8914546721904)) ;
#36651=CARTESIAN_POINT('Ctrl Pts',(9.20520540511956,18.1439988032286,-10.8755968305895)) ;
#36652=CARTESIAN_POINT('Ctrl Pts',(7.46415502869361,18.9587675303416,-10.8278252742946)) ;
#36653=CARTESIAN_POINT('Ctrl Pts',(6.26075656118646,19.3894640284856,-10.7952218245531)) ;
#36654=CARTESIAN_POINT('Ctrl Pts',(4.62903477404356,19.8055802561647,-10.7525417888207)) ;
#36655=CARTESIAN_POINT('Ctrl Pts',(4.23011053522662,19.8946008433138,-10.7422433212736)) ;
#36656=CARTESIAN_POINT('Ctrl Pts',(3.37587394598267,20.0583677539779,-10.720643854053)) ;
#36657=CARTESIAN_POINT('Ctrl Pts',(2.92014939149677,20.1297634184969,-10.7093812246527)) ;
#36658=CARTESIAN_POINT('Ctrl Pts',(1.74149529091752,20.273544401591,-10.6805098312542)) ;
#36659=CARTESIAN_POINT('Ctrl Pts',(1.01640818719418,20.3228030401721,-10.662981794902)) ;
#36660=CARTESIAN_POINT('Ctrl Pts',(-0.2907517079791,20.3414619205923,-10.6310393061773)) ;
#36661=CARTESIAN_POINT('Ctrl Pts',(-0.871830604109229,20.3248496419359,
-10.6167221336598)) ;
#36662=CARTESIAN_POINT('Ctrl Pts',(-2.33631900803327,20.2200568250381,-10.5801083433041)) ;
#36663=CARTESIAN_POINT('Ctrl Pts',(-3.21614306287666,20.0988925386872,-10.5575917884417)) ;
#36664=CARTESIAN_POINT('Ctrl Pts',(-4.69316381036904,19.79599277279,-10.5192202809965)) ;
#36665=CARTESIAN_POINT('Ctrl Pts',(-5.29507781997509,19.6435555360137,-10.5034304755838)) ;
#36666=CARTESIAN_POINT('Ctrl Pts',(-6.21642563714968,19.3647877362269,-10.4793874238207)) ;
#36667=CARTESIAN_POINT('Ctrl Pts',(-6.54122155327408,19.2575017170481,-10.470955337764)) ;
#36668=CARTESIAN_POINT('Ctrl Pts',(-7.6040364769991,18.8764424028527,-10.4433245169478)) ;
#36669=CARTESIAN_POINT('Ctrl Pts',(-8.32887114586476,18.5680199236532,-10.42437196776)) ;
#36670=CARTESIAN_POINT('Ctrl Pts',(-9.60648786267476,17.9344835961022,-10.389651975235)) ;
#36671=CARTESIAN_POINT('Ctrl Pts',(-10.1652682088097,17.6237800621291,-10.373980887929)) ;
#36672=CARTESIAN_POINT('Ctrl Pts',(-11.7834581811822,16.6214036752975,-10.326662299053)) ;
#36673=CARTESIAN_POINT('Ctrl Pts',(-12.7939709280014,15.8567073858111,-10.2943377863863)) ;
#36674=CARTESIAN_POINT('Ctrl Pts',(-14.0299467657592,14.7258722452353,-10.2518746451638)) ;
#36675=CARTESIAN_POINT('Ctrl Pts',(-14.3245421419475,14.4394673595353,-10.2415210919698)) ;
#36676=CARTESIAN_POINT('Ctrl Pts',(-14.927704807478,13.816435948504,-10.2199852021186)) ;
#36677=CARTESIAN_POINT('Ctrl Pts',(-15.2340207895599,13.4779408469831,-10.2088364118082)) ;
#36678=CARTESIAN_POINT('Ctrl Pts',(-15.9997083995505,12.5723318606258,-10.1799970917707)) ;
#36679=CARTESIAN_POINT('Ctrl Pts',(-16.440407115086,11.9902965739383,-10.1623915064785)) ;
#36680=CARTESIAN_POINT('Ctrl Pts',(-17.174666673047,10.9037323775427,-10.1303511097546)) ;
#36681=CARTESIAN_POINT('Ctrl Pts',(-17.4796130868513,10.4078659365241,-10.1160151906014)) ;
#36682=CARTESIAN_POINT('Ctrl Pts',(-18.2010772685386,9.11334243900613,-10.0790607033173)) ;
#36683=CARTESIAN_POINT('Ctrl Pts',(-18.5865874435017,8.29885312023002,-10.0562099047307)) ;
#36684=CARTESIAN_POINT('Ctrl Pts',(-19.0792013177351,7.04995072791319,-10.0220436999903)) ;
#36685=CARTESIAN_POINT('Ctrl Pts',(-19.2280650107008,6.6331927567273,-10.0107900395202)) ;
#36686=CARTESIAN_POINT('Ctrl Pts',(-19.4637722789977,5.89846700872934,-9.99134313324307)) ;
#36687=CARTESIAN_POINT('Ctrl Pts',(-19.5567033174411,5.58262526534466,-9.98311377696789)) ;
#36688=CARTESIAN_POINT('Ctrl Pts',(-19.8060872175668,4.65219891399434,-9.95931814270051)) ;
#36689=CARTESIAN_POINT('Ctrl Pts',(-19.9415120356514,4.03238819383098,-9.94396128563841)) ;
#36690=CARTESIAN_POINT('Ctrl Pts',(-20.1893981051791,2.57386814890178,-9.90808249181154)) ;
#36691=CARTESIAN_POINT('Ctrl Pts',(-20.2789340505529,1.73245925534119,-9.88755883477629)) ;
#36692=CARTESIAN_POINT('Ctrl Pts',(-20.341103048006,0.310028945555236,-9.85233272823169)) ;
#36693=CARTESIAN_POINT('Ctrl Pts',(-20.341691015884,-0.268680190415014,
-9.83786436388446)) ;
#36694=CARTESIAN_POINT('Ctrl Pts',(-20.2878109996761,-1.5617167766763,-9.80518880033128)) ;
#36695=CARTESIAN_POINT('Ctrl Pts',(-20.2202816950277,-2.27473849227552,
-9.78692492533925)) ;
#36696=CARTESIAN_POINT('Ctrl Pts',(-20.0494162186243,-3.42705074382047,
-9.75733344824936)) ;
#36697=CARTESIAN_POINT('Ctrl Pts',(-19.9688233781693,-3.86909093217934,
-9.74596878888194)) ;
#36698=CARTESIAN_POINT('Ctrl Pts',(-19.7965447233957,-4.66382796933867,
-9.72569073895414)) ;
#36699=CARTESIAN_POINT('Ctrl Pts',(-19.7098949742089,-5.01742113284066,
-9.71674004681931)) ;
#36700=CARTESIAN_POINT('Ctrl Pts',(-19.4626251649724,-5.92082112187331,
-9.69386137694853)) ;
#36701=CARTESIAN_POINT('Ctrl Pts',(-19.2881857050826,-6.46651350902452,
-9.68002158856314)) ;
#36702=CARTESIAN_POINT('Ctrl Pts',(-18.8557880747323,-7.64508921402875,
-9.64954447393179)) ;
#36703=CARTESIAN_POINT('Ctrl Pts',(-18.5884971782981,-8.27380786498699,
-9.6328941190496)) ;
#36704=CARTESIAN_POINT('Ctrl Pts',(-18.0367165696884,-9.40929921359298,
-9.60165612086801)) ;
#36705=CARTESIAN_POINT('Ctrl Pts',(-17.7611625135032,-9.91963475623672,
-9.58715408442755)) ;
#36706=CARTESIAN_POINT('Ctrl Pts',(-17.0949133576442,-11.0365536664555,
-9.55431360555433)) ;
#36707=CARTESIAN_POINT('Ctrl Pts',(-16.6929876720756,-11.6355375762919,
-9.53591652660456)) ;
#36708=CARTESIAN_POINT('Ctrl Pts',(-15.9944720974617,-12.5656084408824,
-9.50637440803287)) ;
#36709=CARTESIAN_POINT('Ctrl Pts',(-15.7173605405647,-12.9105474296837,
-9.49518663648372)) ;
#36710=CARTESIAN_POINT('Ctrl Pts',(-15.1903875197806,-13.5243685608157,
-9.47501654108906)) ;
#36711=CARTESIAN_POINT('Ctrl Pts',(-14.9440750967618,-13.7960515355945,
-9.46600279388126)) ;
#36712=CARTESIAN_POINT('Ctrl Pts',(-14.2877067459067,-14.48181100612,-9.44282006096143)) ;
#36713=CARTESIAN_POINT('Ctrl Pts',(-13.866958795232,-14.8851896720789,-9.42874228551097)) ;
#36714=CARTESIAN_POINT('Ctrl Pts',(-12.8964473607371,-15.7387261769407,
-9.39735968761845)) ;
#36715=CARTESIAN_POINT('Ctrl Pts',(-12.3392466279428,-16.1792718713767,
-9.38003526662975)) ;
#36716=CARTESIAN_POINT('Ctrl Pts',(-11.2686649084898,-16.9381855459576,
-9.34751320716504)) ;
#36717=CARTESIAN_POINT('Ctrl Pts',(-10.7619369014238,-17.2645776899066,
-9.33241039137698)) ;
#36718=CARTESIAN_POINT('Ctrl Pts',(-9.53826119513563,-17.977934220112,-9.29658075444099)) ;
#36719=CARTESIAN_POINT('Ctrl Pts',(-8.81107458198392,-18.3452855796188,
-9.27575844311755)) ;
#36720=CARTESIAN_POINT('Ctrl Pts',(-7.72593619808643,-18.814020699806,-9.24586181420824)) ;
#36721=CARTESIAN_POINT('Ctrl Pts',(-7.38413331996738,-18.950779573039,-9.23661335380016)) ;
#36722=CARTESIAN_POINT('Ctrl Pts',(-6.90643315141013,-19.1270247024386,
-9.22399311644376)) ;
#36723=CARTESIAN_POINT('Ctrl Pts',(-6.77355780482382,-19.1744832450379,
-9.22051295894036)) ;
#36724=CARTESIAN_POINT('Ctrl Pts',(-5.86184569907663,-19.4894559273203,
-9.19680703527173)) ;
#36725=CARTESIAN_POINT('Ctrl Pts',(-5.06787299617498,-19.7108296906015,
-9.17698849863006)) ;
#36726=CARTESIAN_POINT('Ctrl Pts',(-3.60983258549382,-20.0234081213887,
-9.14072306887849)) ;
#36727=CARTESIAN_POINT('Ctrl Pts',(-2.95050835202995,-20.1311265055259,
-9.12437621116661)) ;
#36728=CARTESIAN_POINT('Ctrl Pts',(-1.63982801643752,-20.2794787868767,
-9.09161677954966)) ;
#36729=CARTESIAN_POINT('Ctrl Pts',(-0.989429106004565,-20.3215972276946,
-9.0752350353492)) ;
#36730=CARTESIAN_POINT('Ctrl Pts',(0.461336783687866,-20.3457241267949,
-9.03844123722084)) ;
#36731=CARTESIAN_POINT('Ctrl Pts',(1.26089775150676,-20.3118550747804,-9.01798257693822)) ;
#36732=CARTESIAN_POINT('Ctrl Pts',(2.38350328160935,-20.1977476850636,-8.98954519437575)) ;
#36733=CARTESIAN_POINT('Ctrl Pts',(2.70977206246689,-20.156568157791,-8.98132578441109)) ;
#36734=CARTESIAN_POINT('Ctrl Pts',(3.66532035197343,-20.0123434835586,-8.95745472300499)) ;
#36735=CARTESIAN_POINT('Ctrl Pts',(4.29091813027024,-19.8875965850159,-8.94201562076869)) ;
#36736=CARTESIAN_POINT('Ctrl Pts',(5.72513655220656,-19.5307712539944,-8.90617302810925)) ;
#36737=CARTESIAN_POINT('Ctrl Pts',(6.52728271107211,-19.2775201460758,-8.88576762481878)) ;
#36738=CARTESIAN_POINT('Ctrl Pts',(7.85095262762428,-18.7674932266274,-8.85067246468831)) ;
#36739=CARTESIAN_POINT('Ctrl Pts',(8.38133805824009,-18.5367047452253,-8.83621174535561)) ;
#36740=CARTESIAN_POINT('Ctrl Pts',(9.54362907206953,-17.9708575065631,-8.80357360389728)) ;
#36741=CARTESIAN_POINT('Ctrl Pts',(10.1691599024166,-17.6244362989125,-8.78533994997957)) ;
#36742=CARTESIAN_POINT('Ctrl Pts',(11.1574434898248,-17.006958540734,-8.75573684021118)) ;
#36743=CARTESIAN_POINT('Ctrl Pts',(11.5316890688778,-16.7554568878551,-8.74433158094691)) ;
#36744=CARTESIAN_POINT('Ctrl Pts',(12.1919900283931,-16.2791102680347,-8.72402802510731)) ;
#36745=CARTESIAN_POINT('Ctrl Pts',(12.4809596929103,-16.0586331143493,-8.71509108914202)) ;
#36746=CARTESIAN_POINT('Ctrl Pts',(13.2079663950725,-15.4724609853883,-8.6922785529023)) ;
#36747=CARTESIAN_POINT('Ctrl Pts',(13.6368036721768,-15.0958608406856,-8.67849048156248)) ;
#36748=CARTESIAN_POINT('Ctrl Pts',(14.5457142325556,-14.2272893979939,-8.64797083023692)) ;
#36749=CARTESIAN_POINT('Ctrl Pts',(15.0178340127291,-13.7280085420308,-8.6312250250989)) ;
#36750=CARTESIAN_POINT('Ctrl Pts',(15.8404540417171,-12.7647335753372,-8.59988057389655)) ;
#36751=CARTESIAN_POINT('Ctrl Pts',(16.1980747562379,-12.3077525526816,-8.58537048257343)) ;
#36752=CARTESIAN_POINT('Ctrl Pts',(16.9559401947958,-11.2489749761785,-8.55249052851208)) ;
#36753=CARTESIAN_POINT('Ctrl Pts',(17.3446396883675,-10.6398690101613,-8.53406155890164)) ;
#36754=CARTESIAN_POINT('Ctrl Pts',(17.849916193536,-9.74654099798349,-8.5079960712815)) ;
#36755=CARTESIAN_POINT('Ctrl Pts',(17.9937452640463,-9.4783796817226,-8.50029148886646)) ;
#36756=CARTESIAN_POINT('Ctrl Pts',(18.131496444736,-9.20710717501038,-8.49264489791374)) ;
#36757=CARTESIAN_POINT('Ctrl Pts',(18.1314964390739,-9.20710718616059,-7.85560087779543)) ;
#36758=CARTESIAN_POINT('Ctrl Pts',(17.8882630500469,-9.68610512089045,-7.86874511426699)) ;
#36759=CARTESIAN_POINT('Ctrl Pts',(17.6261380674114,-10.155287974147,-7.88199762182294)) ;
#36760=CARTESIAN_POINT('Ctrl Pts',(16.8927925656504,-11.353795088599,-7.91703979929467)) ;
#36761=CARTESIAN_POINT('Ctrl Pts',(16.3929324675541,-12.0642796468869,-7.93905694544084)) ;
#36762=CARTESIAN_POINT('Ctrl Pts',(15.4616803202276,-13.2227469724641,-7.97688440688327)) ;
#36763=CARTESIAN_POINT('Ctrl Pts',(15.0523404040361,-13.6869153000442,-7.9926288318601)) ;
#36764=CARTESIAN_POINT('Ctrl Pts',(14.392468270309,-14.3697039890772,-8.01637363824206)) ;
#36765=CARTESIAN_POINT('Ctrl Pts',(14.1566830725011,-14.6020498649752,-8.02454904267831)) ;
#36766=CARTESIAN_POINT('Ctrl Pts',(13.3339607992616,-15.3741049928171,-8.05219587890495)) ;
#36767=CARTESIAN_POINT('Ctrl Pts',(12.721009972887,-15.8850096636789,-8.07139047604844)) ;
#36768=CARTESIAN_POINT('Ctrl Pts',(11.5575522247841,-16.7441389836427,-8.10658802442379)) ;
#36769=CARTESIAN_POINT('Ctrl Pts',(11.0173028737393,-17.104450631235,-8.12249486882939)) ;
#36770=CARTESIAN_POINT('Ctrl Pts',(9.88574650823828,-17.7832396516569,-8.15528524128576)) ;
#36771=CARTESIAN_POINT('Ctrl Pts',(9.29403528847779,-18.0995163386267,-8.17216480123747)) ;
#36772=CARTESIAN_POINT('Ctrl Pts',(8.10296931623272,-18.6623216988528,-8.20559292514709)) ;
#36773=CARTESIAN_POINT('Ctrl Pts',(7.505299583517,-18.9106012583172,-8.2221112926014)) ;
#36774=CARTESIAN_POINT('Ctrl Pts',(6.53628245870715,-19.2599552824999,-8.24818725338983)) ;
#36775=CARTESIAN_POINT('Ctrl Pts',(6.17214191829832,-19.3797197136801,-8.25782913399017)) ;
#36776=CARTESIAN_POINT('Ctrl Pts',(5.3010425589228,-19.6391764789149,-8.28037563349866)) ;
#36777=CARTESIAN_POINT('Ctrl Pts',(4.7916210027444,-19.7696403915504,-8.29317666213022)) ;
#36778=CARTESIAN_POINT('Ctrl Pts',(3.72434227071597,-19.9992914861906,-8.31968347802475)) ;
#36779=CARTESIAN_POINT('Ctrl Pts',(3.166239957531,-20.0952061271093,-8.33337343160315)) ;
#36780=CARTESIAN_POINT('Ctrl Pts',(1.99943603469413,-20.245910715939,-8.36205869249268)) ;
#36781=CARTESIAN_POINT('Ctrl Pts',(1.39079739999137,-20.2968056351824,-8.37705966539734)) ;
#36782=CARTESIAN_POINT('Ctrl Pts',(0.0731679175983439,-20.3474349678555,
-8.40987972686049)) ;
#36783=CARTESIAN_POINT('Ctrl Pts',(-0.635392167642173,-20.3376430638463,
-8.42774866955298)) ;
#36784=CARTESIAN_POINT('Ctrl Pts',(-1.9322415329278,-20.2518727712336,-8.4607730069592)) ;
#36785=CARTESIAN_POINT('Ctrl Pts',(-2.52050965974613,-20.1870983445915,
-8.47587010111979)) ;
#36786=CARTESIAN_POINT('Ctrl Pts',(-3.4698024662583,-20.0404248556819,-8.50016618382197)) ;
#36787=CARTESIAN_POINT('Ctrl Pts',(-3.83289241839446,-19.9741607969628,
-8.50943903624526)) ;
#36788=CARTESIAN_POINT('Ctrl Pts',(-4.62128767800484,-19.8079879854046,
-8.52941035018297)) ;
#36789=CARTESIAN_POINT('Ctrl Pts',(-5.04558441927441,-19.7041815486263,
-8.54007279093563)) ;
#36790=CARTESIAN_POINT('Ctrl Pts',(-6.16463724853136,-19.3918803534568,
-8.56832103602392)) ;
#36791=CARTESIAN_POINT('Ctrl Pts',(-6.85213693819959,-19.1597493700807,
-8.58582255801348)) ;
#36792=CARTESIAN_POINT('Ctrl Pts',(-8.06530669699869,-18.6764588466243,
-8.61773158692266)) ;
#36793=CARTESIAN_POINT('Ctrl Pts',(-8.59538714632041,-18.4385085873238,
-8.63204236425467)) ;
#36794=CARTESIAN_POINT('Ctrl Pts',(-9.90371777134193,-17.7825113919991,
-8.66854091206945)) ;
#36795=CARTESIAN_POINT('Ctrl Pts',(-10.666273023241,-17.3358567790004,-8.69094452336418)) ;
#36796=CARTESIAN_POINT('Ctrl Pts',(-11.9295889440631,-16.4808941328367,
-8.72976584349847)) ;
#36797=CARTESIAN_POINT('Ctrl Pts',(-12.4444299033452,-16.0956868694347,
-8.74611852443698)) ;
#36798=CARTESIAN_POINT('Ctrl Pts',(-13.2156213361805,-15.4595228040943,
-8.77105907575097)) ;
#36799=CARTESIAN_POINT('Ctrl Pts',(-13.4850431837754,-15.2250813845003,
-8.77984625120089)) ;
#36800=CARTESIAN_POINT('Ctrl Pts',(-14.3577672892834,-14.4243199046883,
-8.80879282232597)) ;
#36801=CARTESIAN_POINT('Ctrl Pts',(-14.9326795648082,-13.8282889946704,
-8.82870442177622)) ;
#36802=CARTESIAN_POINT('Ctrl Pts',(-15.8628051567735,-12.7381410546666,
-8.86365451420733)) ;
#36803=CARTESIAN_POINT('Ctrl Pts',(-16.2351418589337,-12.2600564898606,
-8.87854358941128)) ;
#36804=CARTESIAN_POINT('Ctrl Pts',(-16.9961301333448,-11.1873590729252,
-8.91128766448158)) ;
#36805=CARTESIAN_POINT('Ctrl Pts',(-17.3761038082093,-10.5875608263402,
-8.92919673598262)) ;
#36806=CARTESIAN_POINT('Ctrl Pts',(-18.0112429628168,-9.4583585864117,-8.96212037160191)) ;
#36807=CARTESIAN_POINT('Ctrl Pts',(-18.2763251760578,-8.93539919819827,
-8.97707569962068)) ;
#36808=CARTESIAN_POINT('Ctrl Pts',(-18.6703109372152,-8.06700520554083,
-9.00119329305808)) ;
#36809=CARTESIAN_POINT('Ctrl Pts',(-18.813069633418,-7.72822752835531,-9.01042828487)) ;
#36810=CARTESIAN_POINT('Ctrl Pts',(-19.1064229585065,-6.97569337953957,
-9.03044678180629)) ;
#36811=CARTESIAN_POINT('Ctrl Pts',(-19.2529225977215,-6.56053905774759,
-9.04119116502603)) ;
#36812=CARTESIAN_POINT('Ctrl Pts',(-19.6040212792152,-5.45218706636591,
-9.06945649809231)) ;
#36813=CARTESIAN_POINT('Ctrl Pts',(-19.785343815118,-4.75227993549421,-9.08689643411367)) ;
#36814=CARTESIAN_POINT('Ctrl Pts',(-20.0444073099992,-3.47566867337971,
-9.11872771758462)) ;
#36815=CARTESIAN_POINT('Ctrl Pts',(-20.1353988861546,-2.90245427197672,
-9.13302361087297)) ;
#36816=CARTESIAN_POINT('Ctrl Pts',(-20.2809206309282,-1.63864521514933,
-9.16475027109484)) ;
#36817=CARTESIAN_POINT('Ctrl Pts',(-20.3249356444628,-0.947564026151293,
-9.18223878548889)) ;
#36818=CARTESIAN_POINT('Ctrl Pts',(-20.3407620441901,0.311505017826325,
-9.21424923645223)) ;
#36819=CARTESIAN_POINT('Ctrl Pts',(-20.3241631270323,0.87865239574256,-9.22871833912442)) ;
#36820=CARTESIAN_POINT('Ctrl Pts',(-20.2581321205381,1.80595751199905,-9.25222262260541)) ;
#36821=CARTESIAN_POINT('Ctrl Pts',(-20.2227191460455,2.1668032112663,-9.26132649509985)) ;
#36822=CARTESIAN_POINT('Ctrl Pts',(-20.1213641475515,2.97626209251346,-9.28153918339051)) ;
#36823=CARTESIAN_POINT('Ctrl Pts',(-20.0500280028594,3.42400547827348,-9.29259717550828)) ;
#36824=CARTESIAN_POINT('Ctrl Pts',(-19.8281845624787,4.56870547157898,-9.32093419742774)) ;
#36825=CARTESIAN_POINT('Ctrl Pts',(-19.65588745088,5.26080422166608,-9.33814385087967)) ;
#36826=CARTESIAN_POINT('Ctrl Pts',(-19.2787896693064,6.49492165951928,-9.36968450652277)) ;
#36827=CARTESIAN_POINT('Ctrl Pts',(-19.0865023884051,7.039968542636,-9.38392479558484)) ;
#36828=CARTESIAN_POINT('Ctrl Pts',(-18.5165439765595,8.45967814926106,-9.42208579428037)) ;
#36829=CARTESIAN_POINT('Ctrl Pts',(-18.1001983586443,9.31726041477277,-9.44629458698304)) ;
#36830=CARTESIAN_POINT('Ctrl Pts',(-17.4213223148545,10.4969895559092,-9.48092347259129)) ;
#36831=CARTESIAN_POINT('Ctrl Pts',(-17.2066824248624,10.8452451730826,-9.49131344937297)) ;
#36832=CARTESIAN_POINT('Ctrl Pts',(-16.9009117351543,11.3094088237495,-9.50530414680677)) ;
#36833=CARTESIAN_POINT('Ctrl Pts',(-16.8188109755505,11.4311479306215,-9.50898713664741)) ;
#36834=CARTESIAN_POINT('Ctrl Pts',(-16.5378009552827,11.8382479874688,-9.52133641073563)) ;
#36835=CARTESIAN_POINT('Ctrl Pts',(-16.3328911758984,12.1193911449966,-9.52990549974328)) ;
#36836=CARTESIAN_POINT('Ctrl Pts',(-15.6440036891357,13.0153444164916,-9.55754793652415)) ;
#36837=CARTESIAN_POINT('Ctrl Pts',(-15.1317416105862,13.6075143443474,-9.57638876339137)) ;
#36838=CARTESIAN_POINT('Ctrl Pts',(-14.1444780986719,14.6238995865002,-9.61089334243074)) ;
#36839=CARTESIAN_POINT('Ctrl Pts',(-13.6812563590108,15.0581511105426,-9.62646076785511)) ;
#36840=CARTESIAN_POINT('Ctrl Pts',(-12.2414192402371,16.286570208368,-9.67351781771797)) ;
#36841=CARTESIAN_POINT('Ctrl Pts',(-11.2106400565273,17.0125300812806,-9.70567673375053)) ;
#36842=CARTESIAN_POINT('Ctrl Pts',(-9.76202827405727,17.8436144297636,-9.74801140413763)) ;
#36843=CARTESIAN_POINT('Ctrl Pts',(-9.39846678293497,18.0377548382297,-9.75839798939039)) ;
#36844=CARTESIAN_POINT('Ctrl Pts',(-8.62269824640536,18.4221860797962,-9.77990093242946)) ;
#36845=CARTESIAN_POINT('Ctrl Pts',(-8.20950819024049,18.6099931744824,-9.79098646168336)) ;
#36846=CARTESIAN_POINT('Ctrl Pts',(-7.11479442787982,19.0640134639661,-9.819808705586)) ;
#36847=CARTESIAN_POINT('Ctrl Pts',(-6.42458537360321,19.3075532564698,-9.83745805170337)) ;
#36848=CARTESIAN_POINT('Ctrl Pts',(-5.16396854351254,19.6772589158637,-9.8695537141949)) ;
#36849=CARTESIAN_POINT('Ctrl Pts',(-4.59840029468319,19.8170582127219,-9.88390022624317)) ;
#36850=CARTESIAN_POINT('Ctrl Pts',(-3.13790738370902,20.1121711054945,-9.92105328838455)) ;
#36851=CARTESIAN_POINT('Ctrl Pts',(-2.23716577128077,20.2321760983763,-9.94409937575324)) ;
#36852=CARTESIAN_POINT('Ctrl Pts',(-0.893628586157868,20.3203325810586,
-9.97836380789294)) ;
#36853=CARTESIAN_POINT('Ctrl Pts',(-0.455002842144645,20.3348829031922,
-9.98952252649341)) ;
#36854=CARTESIAN_POINT('Ctrl Pts',(0.312038583452749,20.3354958401899,-10.0088518552467)) ;
#36855=CARTESIAN_POINT('Ctrl Pts',(0.640287622543884,20.3278084393698,-10.0170574121269)) ;
#36856=CARTESIAN_POINT('Ctrl Pts',(1.61005161874381,20.2815831365506,-10.0410377290103)) ;
#36857=CARTESIAN_POINT('Ctrl Pts',(2.25008566363119,20.2205837399273,-10.0565954211858)) ;
#36858=CARTESIAN_POINT('Ctrl Pts',(3.710976709445,20.0111206217978,-10.092387039232)) ;
#36859=CARTESIAN_POINT('Ctrl Pts',(4.52774025422039,19.8422743960425,-10.112622977512)) ;
#36860=CARTESIAN_POINT('Ctrl Pts',(5.88938842104761,19.4723112323457,-10.1475309433996)) ;
#36861=CARTESIAN_POINT('Ctrl Pts',(6.44022823999945,19.2971306732805,-10.161981094038)) ;
#36862=CARTESIAN_POINT('Ctrl Pts',(7.65245535823624,18.8539176608413,-10.194567462467)) ;
#36863=CARTESIAN_POINT('Ctrl Pts',(8.30871451488158,18.5740555581093,-10.2127592979663)) ;
#36864=CARTESIAN_POINT('Ctrl Pts',(9.35565962503226,18.0609743923566,-10.2423787910021)) ;
#36865=CARTESIAN_POINT('Ctrl Pts',(9.75563420448104,17.8481026608384,-10.2538405372012)) ;
#36866=CARTESIAN_POINT('Ctrl Pts',(10.4624052872712,17.4410881150172,-10.2741800335069)) ;
#36867=CARTESIAN_POINT('Ctrl Pts',(10.7717467628711,17.251752115875,-10.2830982771922)) ;
#36868=CARTESIAN_POINT('Ctrl Pts',(11.5518246233472,16.7451314666697,-10.3058210329773)) ;
#36869=CARTESIAN_POINT('Ctrl Pts',(12.0146412124843,16.4162261242857,-10.3195389147573)) ;
#36870=CARTESIAN_POINT('Ctrl Pts',(13.0094560927125,15.6446199438071,-10.3501003655355)) ;
#36871=CARTESIAN_POINT('Ctrl Pts',(13.5338446630016,15.1932590429419,-10.3669595559333)) ;
#36872=CARTESIAN_POINT('Ctrl Pts',(14.4540468431467,14.3156931744071,-10.3984241293179)) ;
#36873=CARTESIAN_POINT('Ctrl Pts',(14.8565455233173,13.8975389017678,-10.4129372843635)) ;
#36874=CARTESIAN_POINT('Ctrl Pts',(15.7189478185064,12.9212497599537,-10.4458322055585)) ;
#36875=CARTESIAN_POINT('Ctrl Pts',(16.1680825384402,12.3546394313075,-10.4642732566595)) ;
#36876=CARTESIAN_POINT('Ctrl Pts',(16.8407381506725,11.406367521265,-10.4937997989432)) ;
#36877=CARTESIAN_POINT('Ctrl Pts',(17.0836521290077,11.0392262191932,-10.5049299472697)) ;
#36878=CARTESIAN_POINT('Ctrl Pts',(17.5072273679419,10.351525566645,-10.525066114738)) ;
#36879=CARTESIAN_POINT('Ctrl Pts',(17.6914714713784,10.0333907221002,-10.5341016220387)) ;
#36880=CARTESIAN_POINT('Ctrl Pts',(18.1468451329918,9.19551315903772,-10.5573896433154)) ;
#36881=CARTESIAN_POINT('Ctrl Pts',(18.4043082986069,8.6687306066441,-10.5715499068541)) ;
#36882=CARTESIAN_POINT('Ctrl Pts',(18.9223882860589,7.48122025175797,-10.6030113120323)) ;
#36883=CARTESIAN_POINT('Ctrl Pts',(19.1718821335937,6.81647707442332,-10.6203316499522)) ;
#36884=CARTESIAN_POINT('Ctrl Pts',(19.5690055468501,5.56263222914312,-10.6529326694459)) ;
#36885=CARTESIAN_POINT('Ctrl Pts',(19.7259997231188,4.97732663842603,-10.6681206536517)) ;
#36886=CARTESIAN_POINT('Ctrl Pts',(20.0347610418548,3.57944455740328,-10.7043410416274)) ;
#36887=CARTESIAN_POINT('Ctrl Pts',(20.1635925341505,2.7628974755857,-10.7254734698459)) ;
#36888=CARTESIAN_POINT('Ctrl Pts',(20.2765593789294,1.58465221010846,-10.7553893357962)) ;
#36889=CARTESIAN_POINT('Ctrl Pts',(20.3013005026288,1.22767544682827,-10.7643697752945)) ;
#36890=CARTESIAN_POINT('Ctrl Pts',(20.3418306564613,0.281445753206663,-10.7878287519677)) ;
#36891=CARTESIAN_POINT('Ctrl Pts',(20.3414437677678,-0.308158963865643,
-10.8021384712817)) ;
#36892=CARTESIAN_POINT('Ctrl Pts',(20.2737845864534,-1.84066206873555,-10.8393508987583)) ;
#36893=CARTESIAN_POINT('Ctrl Pts',(20.166408049051,-2.78035121329638,-10.8622289185661)) ;
#36894=CARTESIAN_POINT('Ctrl Pts',(19.8874994093046,-4.2837976432321,-10.9000789076202)) ;
#36895=CARTESIAN_POINT('Ctrl Pts',(19.7561750138368,-4.85356516943185,-10.9147063704701)) ;
#36896=CARTESIAN_POINT('Ctrl Pts',(19.403387817664,-6.13009396921374,-10.948162918131)) ;
#36897=CARTESIAN_POINT('Ctrl Pts',(19.1674998270474,-6.83201681768048,-10.9670580286776)) ;
#36898=CARTESIAN_POINT('Ctrl Pts',(18.7415600003681,-7.90225327399103,-10.9962932662791)) ;
#36899=CARTESIAN_POINT('Ctrl Pts',(18.5776393121558,-8.28027772460641,-11.0067007695699)) ;
#36900=CARTESIAN_POINT('Ctrl Pts',(18.3148670791874,-8.83911176884274,-11.0220934427904)) ;
#36901=CARTESIAN_POINT('Ctrl Pts',(18.2245720180128,-9.02381405227549,-11.0271783889829)) ;
#36902=CARTESIAN_POINT('Ctrl Pts',(18.1314964436398,-9.20710717716895,-11.0322347276753)) ;
#36903=CARTESIAN_POINT('Origin',(0.,0.,5.8748638224677)) ;
#36904=CARTESIAN_POINT('',(18.1314964553944,-9.20710715402079,-14.8444016786038)) ;
#36905=CARTESIAN_POINT('',(18.1314964185968,-9.20710722648607,-14.2060611031549)) ;
#36906=CARTESIAN_POINT('',(18.1314964405232,-9.20710718330643,5.8748638224677)) ;
#36907=CARTESIAN_POINT('Ctrl Pts',(18.1314964554037,-9.20710715400241,-14.8444016794283)) ;
#36908=CARTESIAN_POINT('Ctrl Pts',(18.3793175840612,-8.71907461124281,-14.8306536571053)) ;
#36909=CARTESIAN_POINT('Ctrl Pts',(18.6073666963369,-8.22117033262147,-14.816774955725)) ;
#36910=CARTESIAN_POINT('Ctrl Pts',(19.0167898114644,-7.22263228758697,-14.7893236747267)) ;
#36911=CARTESIAN_POINT('Ctrl Pts',(19.1991357427948,-6.722938352433,-14.775766890081)) ;
#36912=CARTESIAN_POINT('Ctrl Pts',(19.4695729787702,-5.88066771931294,-14.7534170506565)) ;
#36913=CARTESIAN_POINT('Ctrl Pts',(19.5686943715667,-5.54190685110016,-14.7445634423528)) ;
#36914=CARTESIAN_POINT('Ctrl Pts',(19.7781124555335,-4.7502994045236,-14.7242883946986)) ;
#36915=CARTESIAN_POINT('Ctrl Pts',(19.881758767847,-4.2958992688073,-14.712930618706)) ;
#36916=CARTESIAN_POINT('Ctrl Pts',(20.1019323774357,-3.15040311145857,-14.6845939920956)) ;
#36917=CARTESIAN_POINT('Ctrl Pts',(20.1985226533667,-2.45609586418258,-14.6676719691478)) ;
#36918=CARTESIAN_POINT('Ctrl Pts',(20.3087787733636,-1.18564937864585,-14.6364940506944)) ;
#36919=CARTESIAN_POINT('Ctrl Pts',(20.3341734607863,-0.6112622026835,-14.6223230058526)) ;
#36920=CARTESIAN_POINT('Ctrl Pts',(20.3365274559342,0.697512022562245,-14.5896675549361)) ;
#36921=CARTESIAN_POINT('Ctrl Pts',(20.2980967610298,1.43112695980136,-14.5710915794615)) ;
#36922=CARTESIAN_POINT('Ctrl Pts',(20.1635790872482,2.68975644455828,-14.5388943302587)) ;
#36923=CARTESIAN_POINT('Ctrl Pts',(20.0863576339816,3.21604567820772,-14.5253375590982)) ;
#36924=CARTESIAN_POINT('Ctrl Pts',(19.9237170107269,4.08558749479809,-14.5029877367147)) ;
#36925=CARTESIAN_POINT('Ctrl Pts',(19.8498154701953,4.43072868203372,-14.4941341320922)) ;
#36926=CARTESIAN_POINT('Ctrl Pts',(19.6575897469739,5.22668557556732,-14.4738590873597)) ;
#36927=CARTESIAN_POINT('Ctrl Pts',(19.5326764966984,5.67570534257694,-14.4625013106784)) ;
#36928=CARTESIAN_POINT('Ctrl Pts',(19.1816206861132,6.78808903594647,-14.434164686282)) ;
#36929=CARTESIAN_POINT('Ctrl Pts',(18.9364126651438,7.44479680596961,-14.4172426661441)) ;
#36930=CARTESIAN_POINT('Ctrl Pts',(18.4292436451885,8.61482665690823,-14.386064751637)) ;
#36931=CARTESIAN_POINT('Ctrl Pts',(18.1784335648506,9.13218511036002,-14.3718937078825)) ;
#36932=CARTESIAN_POINT('Ctrl Pts',(17.5581176850556,10.2846183525344,-14.3392382697389)) ;
#36933=CARTESIAN_POINT('Ctrl Pts',(17.1754406882582,10.9116952381982,-14.3206623062712)) ;
#36934=CARTESIAN_POINT('Ctrl Pts',(16.4585665486567,11.9549278042565,-14.288465061813)) ;
#36935=CARTESIAN_POINT('Ctrl Pts',(16.1403589644349,12.3811762610222,-14.2749082832902)) ;
#36936=CARTESIAN_POINT('Ctrl Pts',(15.5837754330599,13.0687592373938,-14.2525584516795)) ;
#36937=CARTESIAN_POINT('Ctrl Pts',(15.3546333075434,13.3372323552268,-14.2437048451206)) ;
#36938=CARTESIAN_POINT('Ctrl Pts',(14.8070175421818,13.9460140633165,-14.2234297988823)) ;
#36939=CARTESIAN_POINT('Ctrl Pts',(14.4836016339789,14.2816093613836,-14.2120720225994)) ;
#36940=CARTESIAN_POINT('Ctrl Pts',(13.6457881896671,15.0932166783478,-14.183735396665)) ;
#36941=CARTESIAN_POINT('Ctrl Pts',(13.1177843029926,15.5543067732995,-14.1668133746529)) ;
#36942=CARTESIAN_POINT('Ctrl Pts',(12.115226137486,16.3423852400491,-14.1356354575289)) ;
#36943=CARTESIAN_POINT('Ctrl Pts',(11.6485617076652,16.6782271821253,-14.1214644130649)) ;
#36944=CARTESIAN_POINT('Ctrl Pts',(10.5548374496442,17.3970192273679,-14.0888089693573)) ;
#36945=CARTESIAN_POINT('Ctrl Pts',(9.91999445320359,17.7666700915468,-14.0702330009091)) ;
#36946=CARTESIAN_POINT('Ctrl Pts',(8.79325938757738,18.3434811542774,-14.0380357545278)) ;
#36947=CARTESIAN_POINT('Ctrl Pts',(8.31063355588396,18.5671237104765,-14.024478979104)) ;
#36948=CARTESIAN_POINT('Ctrl Pts',(7.49403356605316,18.9072997977826,-14.0021291513409)) ;
#36949=CARTESIAN_POINT('Ctrl Pts',(7.16478753904079,19.0345042069972,-13.9932755455622)) ;
#36950=CARTESIAN_POINT('Ctrl Pts',(6.39355018054793,19.3096243579578,-13.9730004999153)) ;
#36951=CARTESIAN_POINT('Ctrl Pts',(5.94945259307183,19.4510435733835,-13.9616427234541)) ;
#36952=CARTESIAN_POINT('Ctrl Pts',(4.82647793343027,19.7665838150784,-13.9333060983236)) ;
#36953=CARTESIAN_POINT('Ctrl Pts',(4.14272761925487,19.921107700979,-13.916384077262)) ;
#36954=CARTESIAN_POINT('Ctrl Pts',(2.88601800327718,20.1376056114963,-13.8852061614592)) ;
#36955=CARTESIAN_POINT('Ctrl Pts',(2.31578900329025,20.211120035043,-13.8710351173489)) ;
#36956=CARTESIAN_POINT('Ctrl Pts',(1.01183071483298,20.3233134629898,-13.8383796752688)) ;
#36957=CARTESIAN_POINT('Ctrl Pts',(0.277579105510846,20.346591996161,-13.8198037081226)) ;
#36958=CARTESIAN_POINT('Ctrl Pts',(-0.987899490826792,20.3181880625369,
-13.7876064622164)) ;
#36959=CARTESIAN_POINT('Ctrl Pts',(-1.51881324726421,20.2854114903864,-13.7740496859548)) ;
#36960=CARTESIAN_POINT('Ctrl Pts',(-2.39893785524069,20.1963269409041,-13.7516998571747)) ;
#36961=CARTESIAN_POINT('Ctrl Pts',(-2.74906395265028,20.1516544798401,-13.7428462512073)) ;
#36962=CARTESIAN_POINT('Ctrl Pts',(-3.55834620266862,20.0269131185032,-13.7225712054274)) ;
#36963=CARTESIAN_POINT('Ctrl Pts',(-4.0162657858277,19.9401276672434,-13.7112134290212)) ;
#36964=CARTESIAN_POINT('Ctrl Pts',(-5.15418922315739,19.6836749219689,-13.6828768035733)) ;
#36965=CARTESIAN_POINT('Ctrl Pts',(-5.82916060428898,19.4944507702114,-13.6659547821514)) ;
#36966=CARTESIAN_POINT('Ctrl Pts',(-7.03762968589347,19.0872739826849,-13.6347768658501)) ;
#36967=CARTESIAN_POINT('Ctrl Pts',(-7.57421360100202,18.8807717032836,-13.6206058216082)) ;
#36968=CARTESIAN_POINT('Ctrl Pts',(-8.77464479071782,18.3593703648678,-13.5879503813168)) ;
#36969=CARTESIAN_POINT('Ctrl Pts',(-9.43162786276003,18.0306752997138,-13.5693744161529)) ;
#36970=CARTESIAN_POINT('Ctrl Pts',(-10.531347936492,17.4038910086251,-13.5371771710166)) ;
#36971=CARTESIAN_POINT('Ctrl Pts',(-10.982800075023,17.1225820359373,-13.523620393526)) ;
#36972=CARTESIAN_POINT('Ctrl Pts',(-11.7146719300653,16.6256725072387,-13.5012705631693)) ;
#36973=CARTESIAN_POINT('Ctrl Pts',(-12.0014300436204,16.4198723444649,-13.4924169568436)) ;
#36974=CARTESIAN_POINT('Ctrl Pts',(-12.654026035905,15.9252849843984,-13.4721419107723)) ;
#36975=CARTESIAN_POINT('Ctrl Pts',(-13.0155820663386,15.6311773619367,-13.4607841344249)) ;
#36976=CARTESIAN_POINT('Ctrl Pts',(-13.8946448012753,14.8644398090299,-13.4324475088949)) ;
#36977=CARTESIAN_POINT('Ctrl Pts',(-14.3984242406956,14.3769991158017,-13.4155254873372)) ;
#36978=CARTESIAN_POINT('Ctrl Pts',(-15.2678684628203,13.4441233365775,-13.3843475708726)) ;
#36979=CARTESIAN_POINT('Ctrl Pts',(-15.6416933658884,13.0072933554173,-13.370176526606)) ;
#36980=CARTESIAN_POINT('Ctrl Pts',(-16.44974914612,11.9777555821607,-13.3375210122179)) ;
#36981=CARTESIAN_POINT('Ctrl Pts',(-16.8713807195268,11.3761756702548,-13.3189449707417)) ;
#36982=CARTESIAN_POINT('Ctrl Pts',(-17.5407255078541,10.3018279088841,-13.2867476969551)) ;
#36983=CARTESIAN_POINT('Ctrl Pts',(-17.8040855733151,9.83967722895478,-13.2731909677616)) ;
#36984=CARTESIAN_POINT('Ctrl Pts',(-18.2115988808362,9.05451216737767,-13.2508411986072)) ;
#36985=CARTESIAN_POINT('Ctrl Pts',(-18.3659884079632,8.73710480294482,-13.2419876056377)) ;
#36986=CARTESIAN_POINT('Ctrl Pts',(-18.7048689174683,7.99168040154145,-13.2217125701352)) ;
#36987=CARTESIAN_POINT('Ctrl Pts',(-18.8830630479746,7.56101926201225,-13.2103547912493)) ;
#36988=CARTESIAN_POINT('Ctrl Pts',(-19.2917429981322,6.46849105799463,-13.1820181721876)) ;
#36989=CARTESIAN_POINT('Ctrl Pts',(-19.503109886224,5.80012314008325,-13.1650961593188)) ;
#36990=CARTESIAN_POINT('Ctrl Pts',(-19.8243216146061,4.56601928410968,-13.1339182538095)) ;
#36991=CARTESIAN_POINT('Ctrl Pts',(-19.9454369469548,4.00397261185963,-13.1197472116332)) ;
#36992=CARTESIAN_POINT('Ctrl Pts',(-20.1666572808306,2.71415284203437,-13.0870948303192)) ;
#36993=CARTESIAN_POINT('Ctrl Pts',(-20.2514731144785,1.98456865362528,-13.0685220144798)) ;
#36994=CARTESIAN_POINT('Ctrl Pts',(-20.329403307692,0.721217768220855,-13.0363259505766)) ;
#36995=CARTESIAN_POINT('Ctrl Pts',(-20.3413112248757,0.189348972981878,
-13.0227671787657)) ;
#36996=CARTESIAN_POINT('Ctrl Pts',(-20.3264156435255,-0.695245817713759,
-13.0004148214405)) ;
#36997=CARTESIAN_POINT('Ctrl Pts',(-20.3112883989533,-1.04790714701697,
-12.9915606638422)) ;
#36998=CARTESIAN_POINT('Ctrl Pts',(-20.2549134348881,-1.8648201028368,-12.9712851816854)) ;
#36999=CARTESIAN_POINT('Ctrl Pts',(-20.2068705024629,-2.32840337181275,
-12.9599275102734)) ;
#37000=CARTESIAN_POINT('Ctrl Pts',(-20.0468340372782,-3.48384722064875,
-12.9315906168136)) ;
#37001=CARTESIAN_POINT('Ctrl Pts',(-19.9149283673365,-4.17233432271597,
-12.9146682355612)) ;
#37002=CARTESIAN_POINT('Ctrl Pts',(-19.6106151643196,-5.4107334898701,-12.8834898657631)) ;
#37003=CARTESIAN_POINT('Ctrl Pts',(-19.4498778512491,-5.96276007333131,
-12.8693187351503)) ;
#37004=CARTESIAN_POINT('Ctrl Pts',(-19.0324601571692,-7.19860943130656,
-12.836771516659)) ;
#37005=CARTESIAN_POINT('Ctrl Pts',(-18.7618976180403,-7.87690928700065,
-12.8183071257014)) ;
#37006=CARTESIAN_POINT('Ctrl Pts',(-18.2310278865844,-9.02426027681257,
-12.786151369651)) ;
#37007=CARTESIAN_POINT('Ctrl Pts',(-17.9875531216752,-9.50029396764206,
-12.7725235508096)) ;
#37008=CARTESIAN_POINT('Ctrl Pts',(-17.5522851400165,-10.2744509724509,
-12.7500837103629)) ;
#37009=CARTESIAN_POINT('Ctrl Pts',(-17.3709475889917,-10.5781492922524,
-12.7412104741872)) ;
#37010=CARTESIAN_POINT('Ctrl Pts',(-16.9326544202609,-11.2704982178444,
-12.720919941201)) ;
#37011=CARTESIAN_POINT('Ctrl Pts',(-16.6700805757201,-11.6553564893335,
-12.7095659404388)) ;
#37012=CARTESIAN_POINT('Ctrl Pts',(-15.9797519222731,-12.5960713068128,
-12.6812198625451)) ;
#37013=CARTESIAN_POINT('Ctrl Pts',(-15.5360304497324,-13.1394536018569,
-12.6642850815589)) ;
#37014=CARTESIAN_POINT('Ctrl Pts',(-14.6790323109405,-14.0846875676049,
-12.6330910835965)) ;
#37015=CARTESIAN_POINT('Ctrl Pts',(-14.2750497206702,-14.4939767155589,
-12.6189169760098)) ;
#37016=CARTESIAN_POINT('Ctrl Pts',(-13.3035522912369,-15.3981655343969,
-12.5858031408785)) ;
#37017=CARTESIAN_POINT('Ctrl Pts',(-12.724813319516,-15.8797706140345,-12.566757921796)) ;
#37018=CARTESIAN_POINT('Ctrl Pts',(-11.5653282938198,-16.7404783152019,
-12.53002185721)) ;
#37019=CARTESIAN_POINT('Ctrl Pts',(-10.9892530655328,-17.1241570683089,
-12.5123742754328)) ;
#37020=CARTESIAN_POINT('Ctrl Pts',(-10.1196035711132,-17.6413744453928,
-12.4870257394034)) ;
#37021=CARTESIAN_POINT('Ctrl Pts',(-9.84063600884161,-17.7984929912793,
-12.4790957632584)) ;
#37022=CARTESIAN_POINT('Ctrl Pts',(-8.76973875852369,-18.368760611688,-12.4493068271358)) ;
#37023=CARTESIAN_POINT('Ctrl Pts',(-7.95460237524104,-18.736168344006,-12.4278452409879)) ;
#37024=CARTESIAN_POINT('Ctrl Pts',(-6.53507870208474,-19.2666010060396,
-12.3909211991686)) ;
#37025=CARTESIAN_POINT('Ctrl Pts',(-5.94251788476641,-19.4575342757416,
-12.3756441334639)) ;
#37026=CARTESIAN_POINT('Ctrl Pts',(-4.68058609153175,-19.8011160500778,
-12.3431097415594)) ;
#37027=CARTESIAN_POINT('Ctrl Pts',(-4.01035082367705,-19.9476604071713,
-12.3258267224519)) ;
#37028=CARTESIAN_POINT('Ctrl Pts',(-2.72525323735467,-20.1612448052724,
-12.2927443248325)) ;
#37029=CARTESIAN_POINT('Ctrl Pts',(-2.11221498516215,-20.2346570257772,
-12.2769898775049)) ;
#37030=CARTESIAN_POINT('Ctrl Pts',(-1.12212018118544,-20.3077318824365,
-12.2518683441286)) ;
#37031=CARTESIAN_POINT('Ctrl Pts',(-0.746751946405798,-20.3249968190638,
-12.2424223496793)) ;
#37032=CARTESIAN_POINT('Ctrl Pts',(0.0513961026171948,-20.3395654194972,
-12.2226279674806)) ;
#37033=CARTESIAN_POINT('Ctrl Pts',(0.474050221572415,-20.3341054352808,
-12.2123026061609)) ;
#37034=CARTESIAN_POINT('Ctrl Pts',(1.63162959178368,-20.2830381752318,-12.1841175910848)) ;
#37035=CARTESIAN_POINT('Ctrl Pts',(2.36472561101066,-20.2106884269275,-12.1663566960149)) ;
#37036=CARTESIAN_POINT('Ctrl Pts',(3.66898964405881,-20.01002163033,-12.1341201998595)) ;
#37037=CARTESIAN_POINT('Ctrl Pts',(4.24160694275495,-19.8965125860197,-12.1197467362106)) ;
#37038=CARTESIAN_POINT('Ctrl Pts',(5.7116274166498,-19.5387603669351,-12.0820257340898)) ;
#37039=CARTESIAN_POINT('Ctrl Pts',(6.59857169675064,-19.2573275633482,-12.0584170482112)) ;
#37040=CARTESIAN_POINT('Ctrl Pts',(8.0167078703821,-18.6978212513221,-12.0196230613945)) ;
#37041=CARTESIAN_POINT('Ctrl Pts',(8.56042598330759,-18.455222523287,-12.0044969377431)) ;
#37042=CARTESIAN_POINT('Ctrl Pts',(9.40661172232529,-18.0322153377766,-11.980885384834)) ;
#37043=CARTESIAN_POINT('Ctrl Pts',(9.7163864692485,-17.8672037023283,-11.9722435455832)) ;
#37044=CARTESIAN_POINT('Ctrl Pts',(10.7004117119079,-17.3098680515347,-11.9445910995291)) ;
#37045=CARTESIAN_POINT('Ctrl Pts',(11.3564116163775,-16.8867482559813,-11.9258062681128)) ;
#37046=CARTESIAN_POINT('Ctrl Pts',(12.4973696507733,-16.0542115421019,-11.8914086492038)) ;
#37047=CARTESIAN_POINT('Ctrl Pts',(12.9905817363718,-15.6578010352562,-11.8758921440458)) ;
#37048=CARTESIAN_POINT('Ctrl Pts',(14.404844553611,-14.4082246461022,-11.8289663288442)) ;
#37049=CARTESIAN_POINT('Ctrl Pts',(15.2662510313588,-13.4921451386782,-11.7968916949704)) ;
#37050=CARTESIAN_POINT('Ctrl Pts',(16.2914439660495,-12.1770753735735,-11.7546223485855)) ;
#37051=CARTESIAN_POINT('Ctrl Pts',(16.5352189102869,-11.843937362808,-11.7442188775614)) ;
#37052=CARTESIAN_POINT('Ctrl Pts',(17.0246289195859,-11.1305296550288,-11.722731659385)) ;
#37053=CARTESIAN_POINT('Ctrl Pts',(17.2680485320547,-10.749008595165,-11.711677389608)) ;
#37054=CARTESIAN_POINT('Ctrl Pts',(17.7219347600441,-9.98234945919308,-11.6900089439147)) ;
#37055=CARTESIAN_POINT('Ctrl Pts',(17.9330259355545,-9.59795386329417,-11.6793991614211)) ;
#37056=CARTESIAN_POINT('Ctrl Pts',(18.1314964616938,-9.20710714161543,-11.6687558745767)) ;
#37057=CARTESIAN_POINT('Ctrl Pts',(18.1314964436398,-9.20710717716894,-11.0322347276753)) ;
#37058=CARTESIAN_POINT('Ctrl Pts',(18.0566892618479,-9.35442447504745,-11.036298634348)) ;
#37059=CARTESIAN_POINT('Ctrl Pts',(17.9800859455993,-9.50083148223316,-11.0403445448935)) ;
#37060=CARTESIAN_POINT('Ctrl Pts',(17.6178387460248,-10.1730938980304,-11.0589891313672)) ;
#37061=CARTESIAN_POINT('Ctrl Pts',(17.3108587948471,-10.6871068634057,-11.0734444332431)) ;
#37062=CARTESIAN_POINT('Ctrl Pts',(16.6197502037577,-11.736212507307,-11.103958900449)) ;
#37063=CARTESIAN_POINT('Ctrl Pts',(16.231397660812,-12.2677015846865,-11.1200202695315)) ;
#37064=CARTESIAN_POINT('Ctrl Pts',(15.4495771182218,-13.2354142166768,-11.150819029114)) ;
#37065=CARTESIAN_POINT('Ctrl Pts',(15.0616417406918,-13.675253622841,-11.1654932884422)) ;
#37066=CARTESIAN_POINT('Ctrl Pts',(14.1372967015666,-14.6361545773828,-11.1991806525867)) ;
#37067=CARTESIAN_POINT('Ctrl Pts',(13.5900626531215,-15.1456385955681,-11.2182625805862)) ;
#37068=CARTESIAN_POINT('Ctrl Pts',(12.6791180873017,-15.9045356018542,-11.2483461517184)) ;
#37069=CARTESIAN_POINT('Ctrl Pts',(12.3332013899885,-16.1742522617928,-11.2594161431569)) ;
#37070=CARTESIAN_POINT('Ctrl Pts',(11.6232535875375,-16.6917820379748,-11.281254883196)) ;
#37071=CARTESIAN_POINT('Ctrl Pts',(11.2593507949114,-16.9393812344377,-11.2920166697651)) ;
#37072=CARTESIAN_POINT('Ctrl Pts',(9.84050989198713,-17.8388241530597,-11.3328969405192)) ;
#37073=CARTESIAN_POINT('Ctrl Pts',(8.73480518989878,-18.405500877718,-11.3627229914717)) ;
#37074=CARTESIAN_POINT('Ctrl Pts',(6.97323581450083,-19.1136033118688,-11.4098859154353)) ;
#37075=CARTESIAN_POINT('Ctrl Pts',(6.35051016463328,-19.3294298320257,-11.4264574366206)) ;
#37076=CARTESIAN_POINT('Ctrl Pts',(4.94453393834806,-19.741425701259,-11.4636197508681)) ;
#37077=CARTESIAN_POINT('Ctrl Pts',(4.15784919182704,-19.9219625841466,-11.4842552003682)) ;
#37078=CARTESIAN_POINT('Ctrl Pts',(3.04686803574372,-20.1082327192256,-11.5126185028616)) ;
#37079=CARTESIAN_POINT('Ctrl Pts',(2.73000102682804,-20.1536975950115,-11.5206094675228)) ;
#37080=CARTESIAN_POINT('Ctrl Pts',(1.72661538515555,-20.2735666118176,-11.5455533565328)) ;
#37081=CARTESIAN_POINT('Ctrl Pts',(1.03731127826029,-20.320499567124,-11.5622429886949)) ;
#37082=CARTESIAN_POINT('Ctrl Pts',(-0.421549536565036,-20.3453938772391,
-11.5976348281654)) ;
#37083=CARTESIAN_POINT('Ctrl Pts',(-1.19017337345049,-20.3149263527762,
-11.6163302770035)) ;
#37084=CARTESIAN_POINT('Ctrl Pts',(-2.52769396458766,-20.1857259512756,
-11.6495662217085)) ;
#37085=CARTESIAN_POINT('Ctrl Pts',(-3.09755859930884,-20.1061654994494,
-11.6639462101679)) ;
#37086=CARTESIAN_POINT('Ctrl Pts',(-4.35410842691338,-19.8760402791194,
-11.6961894305837)) ;
#37087=CARTESIAN_POINT('Ctrl Pts',(-5.03791746861582,-19.7138179352369,
-11.7141042275286)) ;
#37088=CARTESIAN_POINT('Ctrl Pts',(-6.15854630799884,-19.3858407094886,
-11.7437772690061)) ;
#37089=CARTESIAN_POINT('Ctrl Pts',(-6.60052142164793,-19.2398449594205,
-11.7555593040985)) ;
#37090=CARTESIAN_POINT('Ctrl Pts',(-7.37053878020162,-18.955828948767,-11.7760368056274)) ;
#37091=CARTESIAN_POINT('Ctrl Pts',(-7.70069597317297,-18.8241221504686,
-11.7847841930272)) ;
#37092=CARTESIAN_POINT('Ctrl Pts',(-8.52416630073965,-18.4703302904785,
-11.8066909854947)) ;
#37093=CARTESIAN_POINT('Ctrl Pts',(-9.01238660192301,-18.2370886773914,
-11.8197720375566)) ;
#37094=CARTESIAN_POINT('Ctrl Pts',(-10.1287370561163,-17.647976763951,-11.8504001826418)) ;
#37095=CARTESIAN_POINT('Ctrl Pts',(-10.748373671431,-17.2775823501562,-11.8679693700332)) ;
#37096=CARTESIAN_POINT('Ctrl Pts',(-11.8244770083481,-16.5539957724781,
-11.9000437433199)) ;
#37097=CARTESIAN_POINT('Ctrl Pts',(-12.2880960828762,-16.212825744257,-11.9144298521117)) ;
#37098=CARTESIAN_POINT('Ctrl Pts',(-13.2848401305551,-15.4119941257301,
-11.9467029966208)) ;
#37099=CARTESIAN_POINT('Ctrl Pts',(-13.809840482815,-14.9433877917634,-11.9646419497777)) ;
#37100=CARTESIAN_POINT('Ctrl Pts',(-14.6398529273788,-14.1213619056663,
-11.9943279910468)) ;
#37101=CARTESIAN_POINT('Ctrl Pts',(-14.9588854111087,-13.7829571403322,
-12.006099598405)) ;
#37102=CARTESIAN_POINT('Ctrl Pts',(-15.5016595812026,-13.1661591149811,
-12.026597334191)) ;
#37103=CARTESIAN_POINT('Ctrl Pts',(-15.7301951048606,-12.8922518501087,
-12.0353746730684)) ;
#37104=CARTESIAN_POINT('Ctrl Pts',(-16.2897519376653,-12.1845621239422,
-12.0574240567864)) ;
#37105=CARTESIAN_POINT('Ctrl Pts',(-16.6107403448509,-11.7432057417062,
-12.0706162868542)) ;
#37106=CARTESIAN_POINT('Ctrl Pts',(-17.3120051469498,-10.692589484698,-12.1012683055797)) ;
#37107=CARTESIAN_POINT('Ctrl Pts',(-17.6785369989615,-10.0750340898224,
-12.1187497834374)) ;
#37108=CARTESIAN_POINT('Ctrl Pts',(-18.2794016099887,-8.92850312041314,
-12.1507710190593)) ;
#37109=CARTESIAN_POINT('Ctrl Pts',(-18.5252882686476,-8.40644854232918,
-12.165195550606)) ;
#37110=CARTESIAN_POINT('Ctrl Pts',(-19.0232288734611,-7.22090883673879,
-12.1976565854428)) ;
#37111=CARTESIAN_POINT('Ctrl Pts',(-19.2634274811846,-6.55325228302571,
-12.2157472232844)) ;
#37112=CARTESIAN_POINT('Ctrl Pts',(-19.6006573210983,-5.43564802233724,
-12.2454075447318)) ;
#37113=CARTESIAN_POINT('Ctrl Pts',(-19.7181837034024,-4.9925216744397,-12.2570072690369)) ;
#37114=CARTESIAN_POINT('Ctrl Pts',(-19.9012846902632,-4.19416345328748,
-12.2774363918178)) ;
#37115=CARTESIAN_POINT('Ctrl Pts',(-19.9725599621307,-3.84044115399536,
-12.2863107869349)) ;
#37116=CARTESIAN_POINT('Ctrl Pts',(-20.1304720784916,-2.93264680309043,
-12.3088234309956)) ;
#37117=CARTESIAN_POINT('Ctrl Pts',(-20.2036720143247,-2.37654458057251,
-12.3223771615009)) ;
#37118=CARTESIAN_POINT('Ctrl Pts',(-20.3164784164307,-1.11989077530671,
-12.353001183084)) ;
#37119=CARTESIAN_POINT('Ctrl Pts',(-20.3430080730884,-0.41888376827425,
-12.3700897316749)) ;
#37120=CARTESIAN_POINT('Ctrl Pts',(-20.3252414322484,0.861762165061094,
-12.4017808313418)) ;
#37121=CARTESIAN_POINT('Ctrl Pts',(-20.2924146577997,1.44082333602945,-12.4162832564512)) ;
#37122=CARTESIAN_POINT('Ctrl Pts',(-20.163366808376,2.7350138593994,-12.4491255895736)) ;
#37123=CARTESIAN_POINT('Ctrl Pts',(-20.0537463860115,3.44802991823574,-12.4675241558239)) ;
#37124=CARTESIAN_POINT('Ctrl Pts',(-19.8161596500103,4.58665495070952,-12.4970657655909)) ;
#37125=CARTESIAN_POINT('Ctrl Pts',(-19.7117206798026,5.01653853587843,-12.5082516052741)) ;
#37126=CARTESIAN_POINT('Ctrl Pts',(-19.4952060723064,5.79597976929068,-12.5284205887677)) ;
#37127=CARTESIAN_POINT('Ctrl Pts',(-19.3875264678072,6.14656483326287,-12.5374350903917)) ;
#37128=CARTESIAN_POINT('Ctrl Pts',(-19.08433431817,7.04625688323722,-12.5606214490273)) ;
#37129=CARTESIAN_POINT('Ctrl Pts',(-18.8745914461672,7.59021435148052,-12.5747020599811)) ;
#37130=CARTESIAN_POINT('Ctrl Pts',(-18.3581811583187,8.77513761122839,-12.6060876021864)) ;
#37131=CARTESIAN_POINT('Ctrl Pts',(-18.0407087789179,9.41056171121832,-12.6234121218039)) ;
#37132=CARTESIAN_POINT('Ctrl Pts',(-17.3935133449375,10.5522875409961,-12.6559372739215)) ;
#37133=CARTESIAN_POINT('Ctrl Pts',(-17.0732115187385,11.0630247912466,-12.6710431513239)) ;
#37134=CARTESIAN_POINT('Ctrl Pts',(-16.267768063359,12.2288604308801,-12.7068878086331)) ;
#37135=CARTESIAN_POINT('Ctrl Pts',(-15.7649931234071,12.8705201861648,-12.7277222660458)) ;
#37136=CARTESIAN_POINT('Ctrl Pts',(-14.9813695185047,13.7555710024903,-12.7576196422071)) ;
#37137=CARTESIAN_POINT('Ctrl Pts',(-14.7302170631559,14.0241890250451,-12.7668575576336)) ;
#37138=CARTESIAN_POINT('Ctrl Pts',(-14.0270899450958,14.7364739457685,-12.7916641107128)) ;
#37139=CARTESIAN_POINT('Ctrl Pts',(-13.5614545576104,15.1660766100367,-12.8070212246478)) ;
#37140=CARTESIAN_POINT('Ctrl Pts',(-12.3831480523363,16.1554756381271,-12.8443386486679)) ;
#37141=CARTESIAN_POINT('Ctrl Pts',(-11.6516583014095,16.6907338212634,-12.8662883651654)) ;
#37142=CARTESIAN_POINT('Ctrl Pts',(-10.3952162257203,17.4871498557438,-12.9031044217192)) ;
#37143=CARTESIAN_POINT('Ctrl Pts',(-9.89033530316382,17.7775754580964,-12.9176721986956)) ;
#37144=CARTESIAN_POINT('Ctrl Pts',(-8.7251378485802,18.3828200002772,-12.9508351460039)) ;
#37145=CARTESIAN_POINT('Ctrl Pts',(-8.0588928922872,18.6844946290157,-12.9694928070031)) ;
#37146=CARTESIAN_POINT('Ctrl Pts',(-6.95430589570256,19.1145549278497,-12.9995878687193)) ;
#37147=CARTESIAN_POINT('Ctrl Pts',(-6.52533673009241,19.2652164768086,-13.011074113294)) ;
#37148=CARTESIAN_POINT('Ctrl Pts',(-5.69891768599815,19.52469696654,-13.0326252262983)) ;
#37149=CARTESIAN_POINT('Ctrl Pts',(-5.30250099061949,19.636062252115,-13.0427102296833)) ;
#37150=CARTESIAN_POINT('Ctrl Pts',(-3.68015293350261,20.0391129708792,-13.0834348842783)) ;
#37151=CARTESIAN_POINT('Ctrl Pts',(-2.43174476311662,20.2285986005478,-13.1136983174551)) ;
#37152=CARTESIAN_POINT('Ctrl Pts',(-0.5390004985823,20.3380392674615,-13.1607582867672)) ;
#37153=CARTESIAN_POINT('Ctrl Pts',(0.0972128450064538,20.3449478059646,
-13.1767365319779)) ;
#37154=CARTESIAN_POINT('Ctrl Pts',(1.51594820637505,20.2937962450181,-13.2127130412846)) ;
#37155=CARTESIAN_POINT('Ctrl Pts',(2.29690909705949,20.2202984671873,-13.2327613045522)) ;
#37156=CARTESIAN_POINT('Ctrl Pts',(3.41373945141306,20.0496411437315,-13.2612887840401)) ;
#37157=CARTESIAN_POINT('Ctrl Pts',(3.75441923683923,19.9886485090049,-13.2699629951663)) ;
#37158=CARTESIAN_POINT('Ctrl Pts',(4.71173751112913,19.7919182468557,-13.2941489981447)) ;
#37159=CARTESIAN_POINT('Ctrl Pts',(5.32384633183264,19.636119027211,-13.3094505388668)) ;
#37160=CARTESIAN_POINT('Ctrl Pts',(6.77058710057535,19.1952477725674,-13.3461305114116)) ;
#37161=CARTESIAN_POINT('Ctrl Pts',(7.59586505908332,18.8838875411011,-13.3675047001487)) ;
#37162=CARTESIAN_POINT('Ctrl Pts',(8.9271745921226,18.2801727861172,-13.4036779926435)) ;
#37163=CARTESIAN_POINT('Ctrl Pts',(9.4454915734253,18.0178201624902,-13.4182053964112)) ;
#37164=CARTESIAN_POINT('Ctrl Pts',(10.5838377577577,17.3789968142754,-13.4511701813564)) ;
#37165=CARTESIAN_POINT('Ctrl Pts',(11.1963977951298,16.990815781739,-13.469667681205)) ;
#37166=CARTESIAN_POINT('Ctrl Pts',(12.1432377407707,16.3173208458749,-13.499174706412)) ;
#37167=CARTESIAN_POINT('Ctrl Pts',(12.4912868324381,16.0524434194065,-13.5102313986805)) ;
#37168=CARTESIAN_POINT('Ctrl Pts',(13.1166301935421,15.5438731394018,-13.5303252021079)) ;
#37169=CARTESIAN_POINT('Ctrl Pts',(13.3963512900077,15.3034555739844,-13.5393893199704)) ;
#37170=CARTESIAN_POINT('Ctrl Pts',(14.1066521035878,14.6585530485366,-13.5628161249132)) ;
#37171=CARTESIAN_POINT('Ctrl Pts',(14.5264213884448,14.2426786965329,-13.5770851948431)) ;
#37172=CARTESIAN_POINT('Ctrl Pts',(15.4085840839167,13.2890716189011,-13.6086336472594)) ;
#37173=CARTESIAN_POINT('Ctrl Pts',(15.862165002764,12.7442378610308,-13.6259314045786)) ;
#37174=CARTESIAN_POINT('Ctrl Pts',(16.651465025194,11.688558941956,-13.6586111460248)) ;
#37175=CARTESIAN_POINT('Ctrl Pts',(16.9943985513127,11.1841005657229,-13.6739036739568)) ;
#37176=CARTESIAN_POINT('Ctrl Pts',(17.5382164045228,10.3012370006598,-13.7001450491441)) ;
#37177=CARTESIAN_POINT('Ctrl Pts',(17.7507653702497,9.93050077307125,-13.7110148847182)) ;
#37178=CARTESIAN_POINT('Ctrl Pts',(18.2429496488048,9.00564838391378,-13.7376773902474)) ;
#37179=CARTESIAN_POINT('Ctrl Pts',(18.5092046976381,8.44489566614177,-13.7534651184153)) ;
#37180=CARTESIAN_POINT('Ctrl Pts',(18.8804332177875,7.56080461403457,-13.7774231923831)) ;
#37181=CARTESIAN_POINT('Ctrl Pts',(19.0036491510871,7.24553958597785,-13.7857718418013)) ;
#37182=CARTESIAN_POINT('Ctrl Pts',(19.2819199811741,6.47753359224639,-13.805770076588)) ;
#37183=CARTESIAN_POINT('Ctrl Pts',(19.4289757211978,6.02210803125775,-13.8173617184285)) ;
#37184=CARTESIAN_POINT('Ctrl Pts',(19.786245072644,4.76568414680968,-13.8490404295854)) ;
#37185=CARTESIAN_POINT('Ctrl Pts',(19.9638259441646,3.95637227027586,-13.8691465634733)) ;
#37186=CARTESIAN_POINT('Ctrl Pts',(20.1807119036668,2.56794258003691,-13.9039114855573)) ;
#37187=CARTESIAN_POINT('Ctrl Pts',(20.2454932410903,1.99385475191587,-13.91835382311)) ;
#37188=CARTESIAN_POINT('Ctrl Pts',(20.3353798108998,0.707759959603777,-13.9509019621734)) ;
#37189=CARTESIAN_POINT('Ctrl Pts',(20.3476919958434,-0.00438795168989717,
-13.969062928623)) ;
#37190=CARTESIAN_POINT('Ctrl Pts',(20.3066418432188,-1.17001440531332,-13.9986946904666)) ;
#37191=CARTESIAN_POINT('Ctrl Pts',(20.2754129431107,-1.62365974657679,-14.0101983246054)) ;
#37192=CARTESIAN_POINT('Ctrl Pts',(20.192048098113,-2.43603301316927,-14.0305647493857)) ;
#37193=CARTESIAN_POINT('Ctrl Pts',(20.1454777829067,-2.7951365758985,-14.0394694047063)) ;
#37194=CARTESIAN_POINT('Ctrl Pts',(20.0016850960595,-3.71136854291113,-14.0621269840593)) ;
#37195=CARTESIAN_POINT('Ctrl Pts',(19.8907671598969,-4.26603429286399,-14.0757939315026)) ;
#37196=CARTESIAN_POINT('Ctrl Pts',(19.5924066585068,-5.49017466750817,-14.1063783939317)) ;
#37197=CARTESIAN_POINT('Ctrl Pts',(19.3934684693106,-6.15611792462093,-14.1233124246089)) ;
#37198=CARTESIAN_POINT('Ctrl Pts',(18.9665715038959,-7.35714903919237,-14.1548528757879)) ;
#37199=CARTESIAN_POINT('Ctrl Pts',(18.7489979705012,-7.89515946049258,-14.1693645498328)) ;
#37200=CARTESIAN_POINT('Ctrl Pts',(18.388566797702,-8.6871599391645,-14.1913380652936)) ;
#37201=CARTESIAN_POINT('Ctrl Pts',(18.2627932302902,-8.94854526859602,-14.1986920259333)) ;
#37202=CARTESIAN_POINT('Ctrl Pts',(18.1314964185826,-9.20710722651393,-14.2060611019251)) ;
#37203=CARTESIAN_POINT('Origin',(0.,0.,5.8748638224677)) ;
#37204=CARTESIAN_POINT('',(18.13149644046,-9.20710718343108,-18.0177676543358)) ;
#37205=CARTESIAN_POINT('',(18.1314964193088,-9.20710722508389,-17.3804829809499)) ;
#37206=CARTESIAN_POINT('',(18.1314964405232,-9.20710718330643,5.8748638224677)) ;
#37207=CARTESIAN_POINT('Ctrl Pts',(18.1314964403967,-9.20710718355568,-18.0177676543358)) ;
#37208=CARTESIAN_POINT('Ctrl Pts',(18.2848468652002,-8.90511518693541,-18.0092111172447)) ;
#37209=CARTESIAN_POINT('Ctrl Pts',(18.4306320472352,-8.59933220051178,-18.0007113518994)) ;
#37210=CARTESIAN_POINT('Ctrl Pts',(18.7638970465689,-7.85285814102169,-17.9804530256096)) ;
#37211=CARTESIAN_POINT('Ctrl Pts',(18.9435802765869,-7.40891258858516,-17.9687815480159)) ;
#37212=CARTESIAN_POINT('Ctrl Pts',(19.3470444774742,-6.30112102115447,-17.9401413350593)) ;
#37213=CARTESIAN_POINT('Ctrl Pts',(19.552520645194,-5.63126910593042,-17.9232272954833)) ;
#37214=CARTESIAN_POINT('Ctrl Pts',(19.8629563074807,-4.39489182516919,-17.8920606974358)) ;
#37215=CARTESIAN_POINT('Ctrl Pts',(19.9791952998858,-3.83195181331826,-17.8778928539826)) ;
#37216=CARTESIAN_POINT('Ctrl Pts',(20.188971113737,-2.5423051834774,-17.845291702278)) ;
#37217=CARTESIAN_POINT('Ctrl Pts',(20.2673987781289,-1.81394643648051,-17.8267682718461)) ;
#37218=CARTESIAN_POINT('Ctrl Pts',(20.3347660057942,-0.550749519922652,
-17.7945919644321)) ;
#37219=CARTESIAN_POINT('Ctrl Pts',(20.3422153178882,-0.0176339134709528,
-17.7810031462317)) ;
#37220=CARTESIAN_POINT('Ctrl Pts',(20.3197651828203,0.868274262940604,-17.7586129470385)) ;
#37221=CARTESIAN_POINT('Ctrl Pts',(20.3016175165226,1.2211018192908,-17.7497507102282)) ;
#37222=CARTESIAN_POINT('Ctrl Pts',(20.2382467390559,2.03773712335482,-17.7294688738315)) ;
#37223=CARTESIAN_POINT('Ctrl Pts',(20.1862554309954,2.50082003081712,-17.718112778665)) ;
#37224=CARTESIAN_POINT('Ctrl Pts',(20.0163339745423,3.6550682917691,-17.6897704054366)) ;
#37225=CARTESIAN_POINT('Ctrl Pts',(19.878486812409,4.34268479864119,-17.6728411930499)) ;
#37226=CARTESIAN_POINT('Ctrl Pts',(19.563466074364,5.57881594977015,-17.6416532069444)) ;
#37227=CARTESIAN_POINT('Ctrl Pts',(19.3979640233866,6.12954941964333,-17.6274794100156)) ;
#37228=CARTESIAN_POINT('Ctrl Pts',(18.9681516648124,7.36692435238321,-17.5947961003701)) ;
#37229=CARTESIAN_POINT('Ctrl Pts',(18.6894740988052,8.04772603605271,-17.5761943392817)) ;
#37230=CARTESIAN_POINT('Ctrl Pts',(18.1470175588704,9.19183408402059,-17.543986951799)) ;
#37231=CARTESIAN_POINT('Ctrl Pts',(17.9007695949262,9.66263470761095,-17.5304460421146)) ;
#37232=CARTESIAN_POINT('Ctrl Pts',(17.4607713559866,10.4291839844668,-17.5081160409011)) ;
#37233=CARTESIAN_POINT('Ctrl Pts',(17.2772359495011,10.7304957492154,-17.4992665526856)) ;
#37234=CARTESIAN_POINT('Ctrl Pts',(16.833278221658,11.4184000387083,-17.4789946898218)) ;
#37235=CARTESIAN_POINT('Ctrl Pts',(16.5672188229569,11.8011177901146,-17.4676360429288)) ;
#37236=CARTESIAN_POINT('Ctrl Pts',(15.8689611111785,12.7353266029941,-17.4393029863442)) ;
#37237=CARTESIAN_POINT('Ctrl Pts',(15.4209771907138,13.274258250832,-17.4223852617783)) ;
#37238=CARTESIAN_POINT('Ctrl Pts',(14.5564391609998,14.2113426630041,-17.3912133366882)) ;
#37239=CARTESIAN_POINT('Ctrl Pts',(14.1490707226599,14.6169754436214,-17.3770439105198)) ;
#37240=CARTESIAN_POINT('Ctrl Pts',(13.1836889780527,15.5000214367709,-17.3443994401186)) ;
#37241=CARTESIAN_POINT('Ctrl Pts',(12.6159023526168,15.9655664468605,-17.3258330622126)) ;
#37242=CARTESIAN_POINT('Ctrl Pts',(11.5952137037948,16.7139455775033,-17.2936394725038)) ;
#37243=CARTESIAN_POINT('Ctrl Pts',(11.1540431690795,17.0115337359609,-17.2800766824873)) ;
#37244=CARTESIAN_POINT('Ctrl Pts',(10.4015872509112,17.4772293666899,-17.2577194222446)) ;
#37245=CARTESIAN_POINT('Ctrl Pts',(10.0966729479995,17.6551342450156,-17.2488643357817)) ;
#37246=CARTESIAN_POINT('Ctrl Pts',(9.37887939602634,18.0492571050063,-17.2285881849787)) ;
#37247=CARTESIAN_POINT('Ctrl Pts',(8.96289090314646,18.2593990295814,-17.217230766666)) ;
#37248=CARTESIAN_POINT('Ctrl Pts',(7.90421558549184,18.7492991810976,-17.1888924321946)) ;
#37249=CARTESIAN_POINT('Ctrl Pts',(7.2536011695045,19.0104737732274,-17.1719684103905)) ;
#37250=CARTESIAN_POINT('Ctrl Pts',(6.04710580231004,19.4238206106951,-17.1407877182251)) ;
#37251=CARTESIAN_POINT('Ctrl Pts',(5.49575524182426,19.5869589809446,-17.1266159344591)) ;
#37252=CARTESIAN_POINT('Ctrl Pts',(4.22605273264442,19.9048099806835,-17.0939578919097)) ;
#37253=CARTESIAN_POINT('Ctrl Pts',(3.50473852120334,20.0443950885938,-17.0753800291579)) ;
#37254=CARTESIAN_POINT('Ctrl Pts',(2.25077640559223,20.2172863225218,-17.0431821328598)) ;
#37255=CARTESIAN_POINT('Ctrl Pts',(1.72144134674525,20.2692205531145,-17.0296266179625)) ;
#37256=CARTESIAN_POINT('Ctrl Pts',(0.83839413705373,20.3210140914646,-17.007278290098)) ;
#37257=CARTESIAN_POINT('Ctrl Pts',(0.485625654000585,20.3325033459276,-16.9984249392236)) ;
#37258=CARTESIAN_POINT('Ctrl Pts',(-0.333192031165951,20.3378480682913,
-16.9781500585281)) ;
#37259=CARTESIAN_POINT('Ctrl Pts',(-0.799086858003867,20.3248750713429,
-16.9667921908016)) ;
#37260=CARTESIAN_POINT('Ctrl Pts',(-1.96327042406237,20.2523641561014,-16.9384561726787)) ;
#37261=CARTESIAN_POINT('Ctrl Pts',(-2.65969615688901,20.1727216860304,-16.9215348272028)) ;
#37262=CARTESIAN_POINT('Ctrl Pts',(-3.91744974358327,19.9626109331623,-16.8903578417404)) ;
#37263=CARTESIAN_POINT('Ctrl Pts',(-4.48000617322129,19.8439357121956,-16.8761870400015)) ;
#37264=CARTESIAN_POINT('Ctrl Pts',(-5.74801992083268,19.5197638994597,-16.8435310805167)) ;
#37265=CARTESIAN_POINT('Ctrl Pts',(-6.44888974641509,19.299552358675,-16.8249543236513)) ;
#37266=CARTESIAN_POINT('Ctrl Pts',(-7.63419518228278,18.8553376330106,-16.7927567110361)) ;
#37267=CARTESIAN_POINT('Ctrl Pts',(-8.12457243802752,18.6492899999245,-16.7792003641962)) ;
#37268=CARTESIAN_POINT('Ctrl Pts',(-8.92604162034029,18.2749090635845,-16.7568511177691)) ;
#37269=CARTESIAN_POINT('Ctrl Pts',(-9.24183490843041,18.1172573522834,-16.7479976670987)) ;
#37270=CARTESIAN_POINT('Ctrl Pts',(-9.96468169632983,17.7325744260933,-16.7277227606743)) ;
#37271=CARTESIAN_POINT('Ctrl Pts',(-10.3683523476635,17.4996100578037,-16.7163649739773)) ;
#37272=CARTESIAN_POINT('Ctrl Pts',(-11.3580162748056,16.8821857765042,-16.6880282482898)) ;
#37273=CARTESIAN_POINT('Ctrl Pts',(-11.9328080695378,16.4809229434472,-16.6711061399647)) ;
#37274=CARTESIAN_POINT('Ctrl Pts',(-12.9393567353492,15.6979396197025,-16.6399281095113)) ;
#37275=CARTESIAN_POINT('Ctrl Pts',(-13.377803957127,15.3260110404622,-16.6257570397981)) ;
#37276=CARTESIAN_POINT('Ctrl Pts',(-14.3390525641398,14.4378798572536,-16.5931027361268)) ;
#37277=CARTESIAN_POINT('Ctrl Pts',(-14.8508270856633,13.9109209828762,-16.574527968869)) ;
#37278=CARTESIAN_POINT('Ctrl Pts',(-15.6822693853246,12.956510641737,-16.5423312204117)) ;
#37279=CARTESIAN_POINT('Ctrl Pts',(-16.0156937568029,12.5420212101978,-16.5287737317652)) ;
#37280=CARTESIAN_POINT('Ctrl Pts',(-16.5427380143628,11.8314981870084,-16.5064229912819)) ;
#37281=CARTESIAN_POINT('Ctrl Pts',(-16.7455754381747,11.5426270735492,-16.4975691798431)) ;
#37282=CARTESIAN_POINT('Ctrl Pts',(-17.1985274356489,10.8604663528818,-16.4772939663375)) ;
#37283=CARTESIAN_POINT('Ctrl Pts',(-17.442845371727,10.4635666093895,-16.4659362229455)) ;
#37284=CARTESIAN_POINT('Ctrl Pts',(-18.0198263305446,9.44979310335126,-16.4375995299252)) ;
#37285=CARTESIAN_POINT('Ctrl Pts',(-18.3346447889792,8.82346475836924,-16.420677411076)) ;
#37286=CARTESIAN_POINT('Ctrl Pts',(-18.8477487508107,7.65601910921282,-16.3894993556758)) ;
#37287=CARTESIAN_POINT('Ctrl Pts',(-19.0565762035925,7.12033405608312,-16.3753282713825)) ;
#37288=CARTESIAN_POINT('Ctrl Pts',(-19.4798530288185,5.88185746235006,-16.3426719435368)) ;
#37289=CARTESIAN_POINT('Ctrl Pts',(-19.6794787986084,5.17484492062462,-16.3240951064432)) ;
#37290=CARTESIAN_POINT('Ctrl Pts',(-19.9570136934487,3.93983429351838,-16.2918975100239)) ;
#37291=CARTESIAN_POINT('Ctrl Pts',(-20.0532006406604,3.41669948229693,-16.2783412604372)) ;
#37292=CARTESIAN_POINT('Ctrl Pts',(-20.1789347354474,2.54108516131153,-16.2559920971618)) ;
#37293=CARTESIAN_POINT('Ctrl Pts',(-20.219993529437,2.19052246674787,-16.2471386349231)) ;
#37294=CARTESIAN_POINT('Ctrl Pts',(-20.2940468022163,1.37504265726054,-16.226863703197)) ;
#37295=CARTESIAN_POINT('Ctrl Pts',(-20.3202243573513,0.909706260809126,
-16.2155058998852)) ;
#37296=CARTESIAN_POINT('Ctrl Pts',(-20.3456859909393,-0.25647622032154,
-16.1871693611005)) ;
#37297=CARTESIAN_POINT('Ctrl Pts',(-20.3247773694971,-0.957153370477013,
-16.1702474496231)) ;
#37298=CARTESIAN_POINT('Ctrl Pts',(-20.2209709212091,-2.22813658621772,
-16.1390696877212)) ;
#37299=CARTESIAN_POINT('Ctrl Pts',(-20.1499294262565,-2.79867716241515,
-16.1248986860191)) ;
#37300=CARTESIAN_POINT('Ctrl Pts',(-19.9333331497246,-4.0893855548962,-16.0922437421317)) ;
#37301=CARTESIAN_POINT('Ctrl Pts',(-19.7727361782618,-4.80621818148921,
-16.0736682433026)) ;
#37302=CARTESIAN_POINT('Ctrl Pts',(-19.4295863565967,-6.02460765284369,
-16.04147118245)) ;
#37303=CARTESIAN_POINT('Ctrl Pts',(-19.2654172270123,-6.53057607672751,
-16.0279141190136)) ;
#37304=CARTESIAN_POINT('Ctrl Pts',(-18.9596145754748,-7.36067537038867,
-16.0055639303227)) ;
#37305=CARTESIAN_POINT('Ctrl Pts',(-18.8290211989872,-7.68859503422874,
-15.9967102488269)) ;
#37306=CARTESIAN_POINT('Ctrl Pts',(-18.5063625802065,-8.44118594288248,
-15.9764351443152)) ;
#37307=CARTESIAN_POINT('Ctrl Pts',(-18.308101698657,-8.86298447241692,-15.9650773834482)) ;
#37308=CARTESIAN_POINT('Ctrl Pts',(-17.7759216759422,-9.90097661245427,
-15.9367406980118)) ;
#37309=CARTESIAN_POINT('Ctrl Pts',(-17.4243187346176,-10.5074185766589,
-15.9198186034857)) ;
#37310=CARTESIAN_POINT('Ctrl Pts',(-16.7285807071223,-11.5761327112718,
-15.8886405851111)) ;
#37311=CARTESIAN_POINT('Ctrl Pts',(-16.3947644575661,-12.0442497277268,
-15.8744695131932)) ;
#37312=CARTESIAN_POINT('Ctrl Pts',(-15.590413801362,-13.0766922488291,-15.841813854104)) ;
#37313=CARTESIAN_POINT('Ctrl Pts',(-15.1082310161832,-13.6309289022104,
-15.8232376928488)) ;
#37314=CARTESIAN_POINT('Ctrl Pts',(-14.226951014899,-14.5395519675784,-15.7910403720142)) ;
#37315=CARTESIAN_POINT('Ctrl Pts',(-13.8419307099823,-14.9065644024412,
-15.77748371656)) ;
#37316=CARTESIAN_POINT('Ctrl Pts',(-13.1781802256053,-15.4913553272338,
-15.7551340377466)) ;
#37317=CARTESIAN_POINT('Ctrl Pts',(-12.9073594749646,-15.717716165862,-15.7462804621722)) ;
#37318=CARTESIAN_POINT('Ctrl Pts',(-12.2656279341798,-16.2263196210202,
-15.7260054394226)) ;
#37319=CARTESIAN_POINT('Ctrl Pts',(-11.8906328554521,-16.5030885853016,
-15.7146476560595)) ;
#37320=CARTESIAN_POINT('Ctrl Pts',(-10.928865679103,-17.1631179494164,-15.6863110620378)) ;
#37321=CARTESIAN_POINT('Ctrl Pts',(-10.3311750509017,-17.5293908635168,
-15.6693890777624)) ;
#37322=CARTESIAN_POINT('Ctrl Pts',(-9.21092100351927,-18.1386656973709,
-15.6382112130951)) ;
#37323=CARTESIAN_POINT('Ctrl Pts',(-8.69465526530311,-18.3917160953206,
-15.6240401826759)) ;
#37324=CARTESIAN_POINT('Ctrl Pts',(-7.49610980689216,-18.9174312803453,
-15.5913848054304)) ;
#37325=CARTESIAN_POINT('Ctrl Pts',(-6.80838122351373,-19.1756824678193,
-15.5728088905757)) ;
#37326=CARTESIAN_POINT('Ctrl Pts',(-5.60103778724539,-19.5558965179745,
-15.5406116637739)) ;
#37327=CARTESIAN_POINT('Ctrl Pts',(-5.08780149689677,-19.6956591742904,
-15.5270548538831)) ;
#37328=CARTESIAN_POINT('Ctrl Pts',(-4.22580343339836,-19.8944492327781,
-15.5047049842164)) ;
#37329=CARTESIAN_POINT('Ctrl Pts',(-3.8799182677934,-19.9647881361655,-15.4958513706128)) ;
#37330=CARTESIAN_POINT('Ctrl Pts',(-3.07352708276674,-20.1070263322599,
-15.4755763194249)) ;
#37331=CARTESIAN_POINT('Ctrl Pts',(-2.61203116819607,-20.172168334746,-15.4642185452072)) ;
#37332=CARTESIAN_POINT('Ctrl Pts',(-1.45209688915559,-20.2954216622683,
-15.4358819073146)) ;
#37333=CARTESIAN_POINT('Ctrl Pts',(-0.752131972562254,-20.3333967285738,
-15.4189598717337)) ;
#37334=CARTESIAN_POINT('Ctrl Pts',(0.523086470668565,-20.3366329681707,
-15.3877819358679)) ;
#37335=CARTESIAN_POINT('Ctrl Pts',(1.09757853848662,-20.3137286924139,-15.3736108864778)) ;
#37336=CARTESIAN_POINT('Ctrl Pts',(2.4019320821558,-20.2062266049689,-15.3409554422)) ;
#37337=CARTESIAN_POINT('Ctrl Pts',(3.12973246549749,-20.1063579631095,-15.3223794783815)) ;
#37338=CARTESIAN_POINT('Ctrl Pts',(4.37263038854816,-19.866675994929,-15.2901822347595)) ;
#37339=CARTESIAN_POINT('Ctrl Pts',(4.8905815211749,-19.7455545744569,-15.2766254574297)) ;
#37340=CARTESIAN_POINT('Ctrl Pts',(5.74340477639792,-19.5105055379013,-15.2542756265258)) ;
#37341=CARTESIAN_POINT('Ctrl Pts',(6.08112553807109,-19.4078964113495,-15.2454220195245)) ;
#37342=CARTESIAN_POINT('Ctrl Pts',(6.85814013758017,-19.1495428304986,-15.2251469726107)) ;
#37343=CARTESIAN_POINT('Ctrl Pts',(7.29509134239601,-18.9873832995528,-15.2137891960326)) ;
#37344=CARTESIAN_POINT('Ctrl Pts',(8.37408516501341,-18.5442018549637,-15.1854525737386)) ;
#37345=CARTESIAN_POINT('Ctrl Pts',(9.00789491764561,-18.2447404240817,-15.1685305555329)) ;
#37346=CARTESIAN_POINT('Ctrl Pts',(10.1312286204141,-17.6411583030212,-15.1373526435956)) ;
#37347=CARTESIAN_POINT('Ctrl Pts',(10.625710614469,-17.3478103998223,-15.1231816004402)) ;
#37348=CARTESIAN_POINT('Ctrl Pts',(11.7220139194575,-16.6329571072558,-15.0905261431185)) ;
#37349=CARTESIAN_POINT('Ctrl Pts',(12.3147600163876,-16.1989982006957,-15.0719501592592)) ;
#37350=CARTESIAN_POINT('Ctrl Pts',(13.2941431665818,-15.3970928621927,-15.0397529063177)) ;
#37351=CARTESIAN_POINT('Ctrl Pts',(13.6921794945441,-15.0442325592076,-15.0261961398718)) ;
#37352=CARTESIAN_POINT('Ctrl Pts',(14.3306208199668,-14.4319032553308,-15.0038463237411)) ;
#37353=CARTESIAN_POINT('Ctrl Pts',(14.5789142184307,-14.1810363169254,-14.9949927206885)) ;
#37354=CARTESIAN_POINT('Ctrl Pts',(15.1395853811299,-13.584256742991,-14.9747176773215)) ;
#37355=CARTESIAN_POINT('Ctrl Pts',(15.4468516640989,-13.2338148669836,-14.9633599004859)) ;
#37356=CARTESIAN_POINT('Ctrl Pts',(16.1852759965221,-12.3308380024637,-14.9350232755944)) ;
#37357=CARTESIAN_POINT('Ctrl Pts',(16.600422774887,-11.7659971027763,-14.9181012551279)) ;
#37358=CARTESIAN_POINT('Ctrl Pts',(17.3015739403144,-10.7008316898369,-14.8869233402179)) ;
#37359=CARTESIAN_POINT('Ctrl Pts',(17.5970628635087,-10.2076260875571,-14.8727522963968)) ;
#37360=CARTESIAN_POINT('Ctrl Pts',(17.9602893881657,-9.538595533303,-14.8537576929866)) ;
#37361=CARTESIAN_POINT('Ctrl Pts',(18.0470410689725,-9.37342459922203,-14.8490868914772)) ;
#37362=CARTESIAN_POINT('Ctrl Pts',(18.1314964554037,-9.20710715400241,-14.8444016794283)) ;
#37363=CARTESIAN_POINT('Ctrl Pts',(18.1314964185826,-9.20710722651395,-14.2060611019251)) ;
#37364=CARTESIAN_POINT('Ctrl Pts',(17.9358763267721,-9.59234060186247,-14.2170403428017)) ;
#37365=CARTESIAN_POINT('Ctrl Pts',(17.7279956224823,-9.97130655589842,-14.2280546280103)) ;
#37366=CARTESIAN_POINT('Ctrl Pts',(17.284148524616,-10.7226001072057,-14.2502160005134)) ;
#37367=CARTESIAN_POINT('Ctrl Pts',(17.047877993267,-11.0944041437719,-14.2613538164525)) ;
#37368=CARTESIAN_POINT('Ctrl Pts',(16.5926782493387,-11.7618038366014,-14.2814944671437)) ;
#37369=CARTESIAN_POINT('Ctrl Pts',(16.3774457319728,-12.059696215226,-14.290527048049)) ;
#37370=CARTESIAN_POINT('Ctrl Pts',(15.7985717768379,-12.8167872494878,-14.3138008947374)) ;
#37371=CARTESIAN_POINT('Ctrl Pts',(15.4229541086325,-13.2664010149578,-14.3279500499567)) ;
#37372=CARTESIAN_POINT('Ctrl Pts',(14.5504153941473,-14.2236052365707,-14.359401565525)) ;
#37373=CARTESIAN_POINT('Ctrl Pts',(14.0452548052217,-14.7226472103789,-14.3767231881684)) ;
#37374=CARTESIAN_POINT('Ctrl Pts',(13.0627935843752,-15.5965305615437,-14.409314660392)) ;
#37375=CARTESIAN_POINT('Ctrl Pts',(12.5928090209797,-15.9784070825999,-14.4244915076494)) ;
#37376=CARTESIAN_POINT('Ctrl Pts',(11.4225885965584,-16.8455034298845,-14.461340489271)) ;
#37377=CARTESIAN_POINT('Ctrl Pts',(10.7075407047529,-17.3088151129628,-14.4831295564706)) ;
#37378=CARTESIAN_POINT('Ctrl Pts',(9.66356012251429,-17.895743379507,-14.5133717407458)) ;
#37379=CARTESIAN_POINT('Ctrl Pts',(9.35725611455952,-18.0577902677465,-14.5220572295973)) ;
#37380=CARTESIAN_POINT('Ctrl Pts',(8.48808657723682,-18.489558794215,-14.5460753687141)) ;
#37381=CARTESIAN_POINT('Ctrl Pts',(7.91672812828408,-18.7413133345442,-14.5612049193879)) ;
#37382=CARTESIAN_POINT('Ctrl Pts',(6.50440272820335,-19.2874886385148,-14.5979300476961)) ;
#37383=CARTESIAN_POINT('Ctrl Pts',(5.65392662827631,-19.5537099908529,-14.6195197088102)) ;
#37384=CARTESIAN_POINT('Ctrl Pts',(4.22385052510927,-19.900224159471,-14.6559337505174)) ;
#37385=CARTESIAN_POINT('Ctrl Pts',(3.65334484369751,-20.0128183289596,-14.6704765150215)) ;
#37386=CARTESIAN_POINT('Ctrl Pts',(2.36016473251122,-20.2108923170943,-14.7035166569855)) ;
#37387=CARTESIAN_POINT('Ctrl Pts',(1.63613970786653,-20.2823466401737,-14.7220750538599)) ;
#37388=CARTESIAN_POINT('Ctrl Pts',(0.450302395088354,-20.3354572780443,
-14.7522166891377)) ;
#37389=CARTESIAN_POINT('Ctrl Pts',(-0.00981580338987972,-20.3404401002588,
-14.7638441743822)) ;
#37390=CARTESIAN_POINT('Ctrl Pts',(-0.878733626513398,-20.3203642717784,
-14.7854707490982)) ;
#37391=CARTESIAN_POINT('Ctrl Pts',(-1.28738263790034,-20.2985720133255,
-14.7954953941133)) ;
#37392=CARTESIAN_POINT('Ctrl Pts',(-2.96347683346068,-20.1583688742635,
-14.8364751683913)) ;
#37393=CARTESIAN_POINT('Ctrl Pts',(-4.21909058816922,-19.9334220812544,
-14.8670412017991)) ;
#37394=CARTESIAN_POINT('Ctrl Pts',(-6.06689801808748,-19.4198559139412,
-14.9146618712423)) ;
#37395=CARTESIAN_POINT('Ctrl Pts',(-6.67980000883116,-19.217656347121,-14.9308780736159)) ;
#37396=CARTESIAN_POINT('Ctrl Pts',(-8.02273855991015,-18.7025927007995,
-14.9673419798132)) ;
#37397=CARTESIAN_POINT('Ctrl Pts',(-8.74616799484573,-18.3754142924498,
-14.9876378056753)) ;
#37398=CARTESIAN_POINT('Ctrl Pts',(-9.74526611379734,-17.851162276582,-15.0160952926151)) ;
#37399=CARTESIAN_POINT('Ctrl Pts',(-10.0380131877422,-17.6882023680529,
-15.0244790979386)) ;
#37400=CARTESIAN_POINT('Ctrl Pts',(-10.8346760546563,-17.2185834688636,
-15.0473402724233)) ;
#37401=CARTESIAN_POINT('Ctrl Pts',(-11.3294809836519,-16.8971208228581,
-15.0616477938207)) ;
#37402=CARTESIAN_POINT('Ctrl Pts',(-12.5504129673034,-16.0261404239907,
-15.0980235895946)) ;
#37403=CARTESIAN_POINT('Ctrl Pts',(-13.2548979994215,-15.4485503999224,
-15.120081495915)) ;
#37404=CARTESIAN_POINT('Ctrl Pts',(-14.3429776035582,-14.4270662107565,
-15.1570181236818)) ;
#37405=CARTESIAN_POINT('Ctrl Pts',(-14.7503019787096,-14.0103471988409,
-15.1715930934248)) ;
#37406=CARTESIAN_POINT('Ctrl Pts',(-15.627842607075,-13.0318165116084,-15.2047913792323)) ;
#37407=CARTESIAN_POINT('Ctrl Pts',(-16.0867349806377,-12.4609251806071,
-15.2234776101177)) ;
#37408=CARTESIAN_POINT('Ctrl Pts',(-16.7781755725741,-11.4986952782749,
-15.2535598154692)) ;
#37409=CARTESIAN_POINT('Ctrl Pts',(-17.0301419704014,-11.1221148098039,
-15.2650059803411)) ;
#37410=CARTESIAN_POINT('Ctrl Pts',(-17.4870978845055,-10.3871794541201,
-15.2865369525305)) ;
#37411=CARTESIAN_POINT('Ctrl Pts',(-17.6941678523924,-10.0303796837544,
-15.2966403326889)) ;
#37412=CARTESIAN_POINT('Ctrl Pts',(-18.4874191611665,-8.56242856749256,
-15.337288239056)) ;
#37413=CARTESIAN_POINT('Ctrl Pts',(-18.9809131254149,-7.40437684840318,
-15.3674603915569)) ;
#37414=CARTESIAN_POINT('Ctrl Pts',(-19.5577514721686,-5.6051262129008,-15.4143555214567)) ;
#37415=CARTESIAN_POINT('Ctrl Pts',(-19.7228195259651,-4.9933417024841,-15.4302663369936)) ;
#37416=CARTESIAN_POINT('Ctrl Pts',(-20.0270799951898,-3.612193070057,-15.4661019720934)) ;
#37417=CARTESIAN_POINT('Ctrl Pts',(-20.1510176811904,-2.84048492571852,
-15.4860772580447)) ;
#37418=CARTESIAN_POINT('Ctrl Pts',(-20.2657464435653,-1.71573646667443,
-15.514633659491)) ;
#37419=CARTESIAN_POINT('Ctrl Pts',(-20.2922503472445,-1.3670451592217,-15.5234019992902)) ;
#37420=CARTESIAN_POINT('Ctrl Pts',(-20.341497512413,-0.384377930322299,
-15.5477579544355)) ;
#37421=CARTESIAN_POINT('Ctrl Pts',(-20.3435902926221,0.250227276189321,
-15.5631321567441)) ;
#37422=CARTESIAN_POINT('Ctrl Pts',(-20.2776451958704,1.76595391228162,-15.5999271289221)) ;
#37423=CARTESIAN_POINT('Ctrl Pts',(-20.181866006293,2.64457186147614,-15.6213430419292)) ;
#37424=CARTESIAN_POINT('Ctrl Pts',(-19.9289262116076,4.08621997057266,-15.6575629482805)) ;
#37425=CARTESIAN_POINT('Ctrl Pts',(-19.8041002585643,4.65369721003538,-15.6720933342683)) ;
#37426=CARTESIAN_POINT('Ctrl Pts',(-19.4691943455686,5.91593452280017,-15.705072745162)) ;
#37427=CARTESIAN_POINT('Ctrl Pts',(-19.2458740792131,6.60637065508469,-15.7235820634347)) ;
#37428=CARTESIAN_POINT('Ctrl Pts',(-18.8297569377225,7.69109339204809,-15.7530850757679)) ;
#37429=CARTESIAN_POINT('Ctrl Pts',(-18.6602652571632,8.0936498854933,-15.7641264675232)) ;
#37430=CARTESIAN_POINT('Ctrl Pts',(-18.3238657942352,8.82576408561461,-15.7842115842327)) ;
#37431=CARTESIAN_POINT('Ctrl Pts',(-18.1606874541884,9.15683357519549,-15.7932817966719)) ;
#37432=CARTESIAN_POINT('Ctrl Pts',(-17.7127060980746,10.0065979909938,-15.8167382137131)) ;
#37433=CARTESIAN_POINT('Ctrl Pts',(-17.414115835438,10.517629680803,-15.8310305102049)) ;
#37434=CARTESIAN_POINT('Ctrl Pts',(-16.7100989795109,11.6101693347247,-15.862595529692)) ;
#37435=CARTESIAN_POINT('Ctrl Pts',(-16.2956986105653,12.1849758283577,-15.8798864139723)) ;
#37436=CARTESIAN_POINT('Ctrl Pts',(-15.4697779922949,13.2128975311609,-15.9125799145422)) ;
#37437=CARTESIAN_POINT('Ctrl Pts',(-15.0661586634025,13.6713402910528,-15.9278938183899)) ;
#37438=CARTESIAN_POINT('Ctrl Pts',(-14.2176386588299,14.5518268088224,-15.9588410428491)) ;
#37439=CARTESIAN_POINT('Ctrl Pts',(-13.7730493294221,14.9733102931769,-15.9744590929112)) ;
#37440=CARTESIAN_POINT('Ctrl Pts',(-12.9622391298698,15.6752695819456,-16.0017088370085)) ;
#37441=CARTESIAN_POINT('Ctrl Pts',(-12.6042300423405,15.9645579075918,-16.0133558358841)) ;
#37442=CARTESIAN_POINT('Ctrl Pts',(-11.9490623645648,16.4581775406919,-16.0338162517828)) ;
#37443=CARTESIAN_POINT('Ctrl Pts',(-11.6557030213528,16.6672219255522,-16.0426762000691)) ;
#37444=CARTESIAN_POINT('Ctrl Pts',(-10.8937479261421,17.1802226536296,-16.0651197441503)) ;
#37445=CARTESIAN_POINT('Ctrl Pts',(-10.4178990008301,17.4728697796118,-16.0786195188759)) ;
#37446=CARTESIAN_POINT('Ctrl Pts',(-9.31625051688439,18.0893642552714,-16.109259619691)) ;
#37447=CARTESIAN_POINT('Ctrl Pts',(-8.68445642331316,18.4010279577892,-16.1264189439552)) ;
#37448=CARTESIAN_POINT('Ctrl Pts',(-7.50545867371461,18.9083554803841,-16.158177454499)) ;
#37449=CARTESIAN_POINT('Ctrl Pts',(-6.96359604916064,19.114553046566,-16.1726739943814)) ;
#37450=CARTESIAN_POINT('Ctrl Pts',(-5.73042922750216,19.5244091944784,-16.2054874926823)) ;
#37451=CARTESIAN_POINT('Ctrl Pts',(-5.03560946930113,19.7150451019282,-16.2238627660137)) ;
#37452=CARTESIAN_POINT('Ctrl Pts',(-3.89887327313653,19.962901286656,-16.2534127738905)) ;
#37453=CARTESIAN_POINT('Ctrl Pts',(-3.46261862467731,20.0431763198624,-16.2646292945534)) ;
#37454=CARTESIAN_POINT('Ctrl Pts',(-2.66195517821135,20.1635831616703,-16.2848166102783)) ;
#37455=CARTESIAN_POINT('Ctrl Pts',(-2.29841784722897,20.208249977966,-16.2938197889457)) ;
#37456=CARTESIAN_POINT('Ctrl Pts',(-1.35557703796695,20.2983219725844,-16.3169514223199)) ;
#37457=CARTESIAN_POINT('Ctrl Pts',(-0.775178092395972,20.3287620541768,
-16.330989172813)) ;
#37458=CARTESIAN_POINT('Ctrl Pts',(0.525800891148537,20.3411915233625,-16.3625793739936)) ;
#37459=CARTESIAN_POINT('Ctrl Pts',(1.24572608182642,20.3098176921019,-16.3801545596301)) ;
#37460=CARTESIAN_POINT('Ctrl Pts',(2.56729544218104,20.1816808104442,-16.4130698324889)) ;
#37461=CARTESIAN_POINT('Ctrl Pts',(3.16918972236981,20.0959566274744,-16.4283095354248)) ;
#37462=CARTESIAN_POINT('Ctrl Pts',(4.18186173607639,19.9050951551573,-16.4543855016734)) ;
#37463=CARTESIAN_POINT('Ctrl Pts',(4.59484272414636,19.813838585845,-16.465142037111)) ;
#37464=CARTESIAN_POINT('Ctrl Pts',(5.61952630538609,19.5536524456278,-16.4920474314851)) ;
#37465=CARTESIAN_POINT('Ctrl Pts',(6.22673658324856,19.3688450435273,-16.5081937605405)) ;
#37466=CARTESIAN_POINT('Ctrl Pts',(7.14603656153679,19.0413441848069,-16.532570000997)) ;
#37467=CARTESIAN_POINT('Ctrl Pts',(7.46481913699451,18.9186443007041,-16.5409909522811)) ;
#37468=CARTESIAN_POINT('Ctrl Pts',(8.23303242687312,18.6005165280536,-16.5613401997083)) ;
#37469=CARTESIAN_POINT('Ctrl Pts',(8.67878310928617,18.396759633008,-16.5732066521846)) ;
#37470=CARTESIAN_POINT('Ctrl Pts',(9.83717795615027,17.8157657972116,-16.6046367772584)) ;
#37471=CARTESIAN_POINT('Ctrl Pts',(10.5354919712934,17.411920592555,-16.6242230332246)) ;
#37472=CARTESIAN_POINT('Ctrl Pts',(11.6889518512255,16.6500043968405,-16.6584186308077)) ;
#37473=CARTESIAN_POINT('Ctrl Pts',(12.1561838820426,16.3120025311964,-16.6728327672675)) ;
#37474=CARTESIAN_POINT('Ctrl Pts',(13.1635063121564,15.5159476804399,-16.7052429806693)) ;
#37475=CARTESIAN_POINT('Ctrl Pts',(13.6953179463166,15.0486142157575,-16.723292591908)) ;
#37476=CARTESIAN_POINT('Ctrl Pts',(14.5312812685789,14.2329165126168,-16.7529699546142)) ;
#37477=CARTESIAN_POINT('Ctrl Pts',(14.8498581943657,13.9002073291417,-16.76462614677)) ;
#37478=CARTESIAN_POINT('Ctrl Pts',(15.3968959495581,13.2886120721922,-16.7850927101015)) ;
#37479=CARTESIAN_POINT('Ctrl Pts',(15.6297567451281,13.0139279257207,-16.7939499098735)) ;
#37480=CARTESIAN_POINT('Ctrl Pts',(16.2045818323457,12.2981641541507,-16.8163803002743)) ;
#37481=CARTESIAN_POINT('Ctrl Pts',(16.5359090602219,11.8489252294761,-16.8298698029265)) ;
#37482=CARTESIAN_POINT('Ctrl Pts',(17.2428671739373,10.8028674754818,-16.8605128805814)) ;
#37483=CARTESIAN_POINT('Ctrl Pts',(17.606783170301,10.1989995034871,-16.8776855894045)) ;
#37484=CARTESIAN_POINT('Ctrl Pts',(18.2115370599317,9.06629390603653,-16.9094568234527)) ;
#37485=CARTESIAN_POINT('Ctrl Pts',(18.4624773590473,8.54369289445659,-16.9239522237103)) ;
#37486=CARTESIAN_POINT('Ctrl Pts',(18.9743287038201,7.3494878938411,-16.9567600995734)) ;
#37487=CARTESIAN_POINT('Ctrl Pts',(19.2225720434545,6.67329294055859,-16.9751308228226)) ;
#37488=CARTESIAN_POINT('Ctrl Pts',(19.56503125503,5.56133073220388,-17.0046824935636)) ;
#37489=CARTESIAN_POINT('Ctrl Pts',(19.6817127130537,5.13313124283561,-17.0159050304079)) ;
#37490=CARTESIAN_POINT('Ctrl Pts',(19.8689376607649,4.34526619725645,-17.0360959193856)) ;
#37491=CARTESIAN_POINT('Ctrl Pts',(19.943946782144,3.98685456518818,-17.045096856844)) ;
#37492=CARTESIAN_POINT('Ctrl Pts',(20.1127798097398,3.05534630776733,-17.0682176846032)) ;
#37493=CARTESIAN_POINT('Ctrl Pts',(20.1918083544377,2.47990560977458,-17.0822469775228)) ;
#37494=CARTESIAN_POINT('Ctrl Pts',(20.3136472950072,1.18288690624342,-17.1138780036046)) ;
#37495=CARTESIAN_POINT('Ctrl Pts',(20.3428395797298,0.460819480629736,-17.1315030976438)) ;
#37496=CARTESIAN_POINT('Ctrl Pts',(20.3257407620204,-0.869940269848479,
-17.1644971582826)) ;
#37497=CARTESIAN_POINT('Ctrl Pts',(20.2905933221345,-1.47795339420346,-17.1797646295784)) ;
#37498=CARTESIAN_POINT('Ctrl Pts',(20.1846674587742,-2.50637917286517,-17.2059274371778)) ;
#37499=CARTESIAN_POINT('Ctrl Pts',(20.1278565607367,-2.92781927268253,-17.2167434211728)) ;
#37500=CARTESIAN_POINT('Ctrl Pts',(19.9546686600175,-3.96564670157676,-17.2435209473983)) ;
#37501=CARTESIAN_POINT('Ctrl Pts',(19.8229083481296,-4.57902462313986,-17.2594786405501)) ;
#37502=CARTESIAN_POINT('Ctrl Pts',(19.576353644806,-5.51397105890394,-17.2836342401105)) ;
#37503=CARTESIAN_POINT('Ctrl Pts',(19.4814636605641,-5.84038291029885,-17.292016445134)) ;
#37504=CARTESIAN_POINT('Ctrl Pts',(19.2317827409194,-6.62529842866866,-17.3121781252484)) ;
#37505=CARTESIAN_POINT('Ctrl Pts',(19.0687213537764,-7.08095443782718,-17.323897830387)) ;
#37506=CARTESIAN_POINT('Ctrl Pts',(18.6622661199277,-8.10052863368516,-17.3505173436298)) ;
#37507=CARTESIAN_POINT('Ctrl Pts',(18.4093092976805,-8.66001212927637,-17.3654140700582)) ;
#37508=CARTESIAN_POINT('Ctrl Pts',(18.131496419296,-9.20710722510901,-17.3804829797999)) ;
#37509=CARTESIAN_POINT('Origin',(0.,0.,-315.477129595899)) ;
#37510=CARTESIAN_POINT('',(18.5446545942647,-0.888979967106324,-319.159121327694)) ;
#37511=CARTESIAN_POINT('',(18.5446545937445,-0.888979977957671,-318.864005972278)) ;
#37512=CARTESIAN_POINT('',(18.544654593745,-0.888979977948782,-315.477129595899)) ;
#37513=CARTESIAN_POINT('',(-15.1336583262364,-10.7548540235205,-318.25)) ;
#37514=CARTESIAN_POINT('Ctrl Pts',(18.5446545942648,-0.888979967104711,
-319.159121327827)) ;
#37515=CARTESIAN_POINT('Ctrl Pts',(18.5602689642712,-0.563254856088902,
-319.155126550097)) ;
#37516=CARTESIAN_POINT('Ctrl Pts',(18.5673008594752,-0.237133928660758,
-319.151136261858)) ;
#37517=CARTESIAN_POINT('Ctrl Pts',(18.5639848688748,0.454254634712284,-319.142610920134)) ;
#37518=CARTESIAN_POINT('Ctrl Pts',(18.5514574374049,0.819333613877284,-319.13806986498)) ;
#37519=CARTESIAN_POINT('Ctrl Pts',(18.5180763409334,1.34179379210061,-319.131464220557)) ;
#37520=CARTESIAN_POINT('Ctrl Pts',(18.5059617259299,1.49964744098828,-319.129454667652)) ;
#37521=CARTESIAN_POINT('Ctrl Pts',(18.4807422496105,1.78103690751676,-319.125845180896)) ;
#37522=CARTESIAN_POINT('Ctrl Pts',(18.4684136000839,1.90463267002766,-319.124250374317)) ;
#37523=CARTESIAN_POINT('Ctrl Pts',(18.4390218585907,2.17208561171922,-319.120778140491)) ;
#37524=CARTESIAN_POINT('Ctrl Pts',(18.421513417929,2.31588564456462,-319.118897916994)) ;
#37525=CARTESIAN_POINT('Ctrl Pts',(18.3641442814051,2.74513552295158,-319.113245342165)) ;
#37526=CARTESIAN_POINT('Ctrl Pts',(18.3193179528783,3.02987679463541,-319.10944209017)) ;
#37527=CARTESIAN_POINT('Ctrl Pts',(18.1897974753758,3.74395388119465,-319.099785218467)) ;
#37528=CARTESIAN_POINT('Ctrl Pts',(18.0965206139479,4.17155406676792,-319.093890983782)) ;
#37529=CARTESIAN_POINT('Ctrl Pts',(17.8777899404563,5.02774224115309,-319.081988015267)) ;
#37530=CARTESIAN_POINT('Ctrl Pts',(17.751807178305,5.45590580439147,-319.075983307905)) ;
#37531=CARTESIAN_POINT('Ctrl Pts',(17.5739425268451,5.98868833864924,-319.068588741989)) ;
#37532=CARTESIAN_POINT('Ctrl Pts',(17.5363403569636,6.09791857126738,-319.067077126615)) ;
#37533=CARTESIAN_POINT('Ctrl Pts',(17.4768575727714,6.26560799361809,-319.064767119793)) ;
#37534=CARTESIAN_POINT('Ctrl Pts',(17.4556975126237,6.32431960832953,-319.0639603586)) ;
#37535=CARTESIAN_POINT('Ctrl Pts',(17.4098631644016,6.44951100624338,-319.062245298802)) ;
#37536=CARTESIAN_POINT('Ctrl Pts',(17.3851032159711,6.51595839515908,-319.061338165955)) ;
#37537=CARTESIAN_POINT('Ctrl Pts',(17.3158320455551,6.69865317473294,-319.058850804712)) ;
#37538=CARTESIAN_POINT('Ctrl Pts',(17.270531439088,6.81459739623427,-319.057279814005)) ;
#37539=CARTESIAN_POINT('Ctrl Pts',(17.1623822603318,7.08339220602497,-319.053646912958)) ;
#37540=CARTESIAN_POINT('Ctrl Pts',(17.0986519257871,7.23587675668323,-319.051592927197)) ;
#37541=CARTESIAN_POINT('Ctrl Pts',(16.8434926916753,7.82418213797548,-319.043664708043)) ;
#37542=CARTESIAN_POINT('Ctrl Pts',(16.637367043777,8.25342905545798,-319.037867645929)) ;
#37543=CARTESIAN_POINT('Ctrl Pts',(16.2040220929921,9.07347940620958,-319.026477257805)) ;
#37544=CARTESIAN_POINT('Ctrl Pts',(15.9785784620398,9.46485021332613,-319.020892772631)) ;
#37545=CARTESIAN_POINT('Ctrl Pts',(15.6593832850657,9.97500867674571,-319.013312424007)) ;
#37546=CARTESIAN_POINT('Ctrl Pts',(15.5781300400181,10.1014329350564,-319.011408780047)) ;
#37547=CARTESIAN_POINT('Ctrl Pts',(15.4256443411548,10.3324735668653,-319.007880621998)) ;
#37548=CARTESIAN_POINT('Ctrl Pts',(15.3548597489361,10.437374927953,-319.00625960607)) ;
#37549=CARTESIAN_POINT('Ctrl Pts',(15.2063368188461,10.6527017438039,-319.002891498421)) ;
#37550=CARTESIAN_POINT('Ctrl Pts',(15.1284549811114,10.7630192654991,-319.001143340073)) ;
#37551=CARTESIAN_POINT('Ctrl Pts',(14.9155173915696,11.0577614781655,-318.996411003453)) ;
#37552=CARTESIAN_POINT('Ctrl Pts',(14.7782479870054,11.2405575529418,-318.993409718934)) ;
#37553=CARTESIAN_POINT('Ctrl Pts',(14.5397237453007,11.5462664518458,-318.988280019695)) ;
#37554=CARTESIAN_POINT('Ctrl Pts',(14.44019912732,11.6704963325322,-318.986163564225)) ;
#37555=CARTESIAN_POINT('Ctrl Pts',(13.971284365632,12.2406281926226,-318.976309148053)) ;
#37556=CARTESIAN_POINT('Ctrl Pts',(13.5827613493189,12.6703732122854,-318.968462947069)) ;
#37557=CARTESIAN_POINT('Ctrl Pts',(12.9737467394363,13.2837425015678,-318.956878270431)) ;
#37558=CARTESIAN_POINT('Ctrl Pts',(12.7680580198789,13.4815657209763,-318.953078519596)) ;
#37559=CARTESIAN_POINT('Ctrl Pts',(12.4950209821368,13.7323062986608,-318.948221047424)) ;
#37560=CARTESIAN_POINT('Ctrl Pts',(12.431752879163,13.789608623984,-318.947108093075)) ;
#37561=CARTESIAN_POINT('Ctrl Pts',(12.3181165561857,13.8911120546022,-318.945133301297)) ;
#37562=CARTESIAN_POINT('Ctrl Pts',(12.2678999504967,13.9354806321743,-318.944268981605)) ;
#37563=CARTESIAN_POINT('Ctrl Pts',(12.1586034327819,14.0310002704813,-318.942406544563)) ;
#37564=CARTESIAN_POINT('Ctrl Pts',(12.0994386529375,14.082052063953,-318.941409867692)) ;
#37565=CARTESIAN_POINT('Ctrl Pts',(11.9152540704735,14.2389625794178,-318.938339632435)) ;
#37566=CARTESIAN_POINT('Ctrl Pts',(11.789154102652,14.3435414247497,-318.936283455166)) ;
#37567=CARTESIAN_POINT('Ctrl Pts',(11.2685627490624,14.7637815723509,-318.927946438416)) ;
#37568=CARTESIAN_POINT('Ctrl Pts',(10.8626484278794,15.0649468671552,-318.921789813333)) ;
#37569=CARTESIAN_POINT('Ctrl Pts',(10.0116776814233,15.6440235255924,-318.909170967969)) ;
#37570=CARTESIAN_POINT('Ctrl Pts',(9.56610922093536,15.9203867673038,-318.902710439529)) ;
#37571=CARTESIAN_POINT('Ctrl Pts',(8.97854663842178,16.2512389727499,-318.894216439311)) ;
#37572=CARTESIAN_POINT('Ctrl Pts',(8.84675497468873,16.3233573207557,-318.892313406443)) ;
#37573=CARTESIAN_POINT('Ctrl Pts',(8.60236262678938,16.4532632100368,-318.888785868166)) ;
#37574=CARTESIAN_POINT('Ctrl Pts',(8.49001831243035,16.5115142256101,-318.887164852958)) ;
#37575=CARTESIAN_POINT('Ctrl Pts',(8.25654015526587,16.629560740872,-318.883796164784)) ;
#37576=CARTESIAN_POINT('Ctrl Pts',(8.13533149768715,16.6891919255227,-318.88204741897)) ;
#37577=CARTESIAN_POINT('Ctrl Pts',(7.80710937199113,16.8462424234499,-318.877311822209)) ;
#37578=CARTESIAN_POINT('Ctrl Pts',(7.59892846058663,16.9411666211697,-318.87430782646)) ;
#37579=CARTESIAN_POINT('Ctrl Pts',(7.24283356526584,17.0956504179605,-318.869172612588)) ;
#37580=CARTESIAN_POINT('Ctrl Pts',(7.09580967690666,17.1571963389631,-318.867053361369)) ;
#37581=CARTESIAN_POINT('Ctrl Pts',(6.40958256758438,17.4341294800548,-318.857174597596)) ;
#37582=CARTESIAN_POINT('Ctrl Pts',(5.86125825431229,17.6260395130887,-318.849306299)) ;
#37583=CARTESIAN_POINT('Ctrl Pts',(5.03359195347694,17.872816540472,-318.83773199408)) ;
#37584=CARTESIAN_POINT('Ctrl Pts',(4.76052363866778,17.9474798871337,-318.833963135922)) ;
#37585=CARTESIAN_POINT('Ctrl Pts',(4.4029616932434,18.0365108885831,-318.829134705794)) ;
#37586=CARTESIAN_POINT('Ctrl Pts',(4.31992687419947,18.0565785389903,-318.828020888114)) ;
#37587=CARTESIAN_POINT('Ctrl Pts',(4.17150517814051,18.0913663271595,-318.826045092615)) ;
#37588=CARTESIAN_POINT('Ctrl Pts',(4.10617149994144,18.1063068207655,-318.825180623535)) ;
#37589=CARTESIAN_POINT('Ctrl Pts',(3.96454428321469,18.1378881186817,-318.823318787552)) ;
#37590=CARTESIAN_POINT('Ctrl Pts',(3.88822389397825,18.1544019937816,-318.822322851705)) ;
#37591=CARTESIAN_POINT('Ctrl Pts',(3.65176627396126,18.2040061762582,-318.819257085943)) ;
#37592=CARTESIAN_POINT('Ctrl Pts',(3.4912942062205,18.2354627774394,-318.817204572854)) ;
#37593=CARTESIAN_POINT('Ctrl Pts',(2.83382432440572,18.3553467206454,-318.808876413922)) ;
#37594=CARTESIAN_POINT('Ctrl Pts',(2.33373384078386,18.4256072390721,-318.802725003206)) ;
#37595=CARTESIAN_POINT('Ctrl Pts',(1.352420382488,18.5228814337528,-318.790636017191)) ;
#37596=CARTESIAN_POINT('Ctrl Pts',(0.871773872791576,18.5517165397807,-318.784706468524)) ;
#37597=CARTESIAN_POINT('Ctrl Pts',(0.205140700510149,18.5657428971848,-318.77633451)) ;
#37598=CARTESIAN_POINT('Ctrl Pts',(0.0196814447135078,18.5668657698757,
-318.773990293903)) ;
#37599=CARTESIAN_POINT('Ctrl Pts',(-0.292086859466395,18.5640820833563,
-318.770019298556)) ;
#37600=CARTESIAN_POINT('Ctrl Pts',(-0.41839555666227,18.5616648885815,-318.768402192849)) ;
#37601=CARTESIAN_POINT('Ctrl Pts',(-0.677301023370646,18.5540661033441,
-318.765069429211)) ;
#37602=CARTESIAN_POINT('Ctrl Pts',(-0.809886748483699,18.5487516840306,
-318.763353001344)) ;
#37603=CARTESIAN_POINT('Ctrl Pts',(-1.15739072023135,18.5310896824256,-318.758828362998)) ;
#37604=CARTESIAN_POINT('Ctrl Pts',(-1.37217082284677,18.5164247379902,-318.756005663441)) ;
#37605=CARTESIAN_POINT('Ctrl Pts',(-1.85894929379247,18.4746718782548,-318.749552448906)) ;
#37606=CARTESIAN_POINT('Ctrl Pts',(-2.13070226663562,18.4453056610072,-318.745909885078)) ;
#37607=CARTESIAN_POINT('Ctrl Pts',(-2.74944388752091,18.3645864748853,-318.737547411276)) ;
#37608=CARTESIAN_POINT('Ctrl Pts',(-3.09582519599233,18.3093785834638,-318.732815558718)) ;
#37609=CARTESIAN_POINT('Ctrl Pts',(-3.53341348580599,18.2268604295015,-318.726821792608)) ;
#37610=CARTESIAN_POINT('Ctrl Pts',(-3.62625741274178,18.208616343989,-318.725549271372)) ;
#37611=CARTESIAN_POINT('Ctrl Pts',(-4.03422819987566,18.1252048962627,-318.71995834476)) ;
#37612=CARTESIAN_POINT('Ctrl Pts',(-4.34777011644217,18.0525606343029,-318.715662488817)) ;
#37613=CARTESIAN_POINT('Ctrl Pts',(-4.75402736579329,17.947236738845,-318.710158445573)) ;
#37614=CARTESIAN_POINT('Ctrl Pts',(-4.84859346628896,17.9219202150331,-318.708881769034)) ;
#37615=CARTESIAN_POINT('Ctrl Pts',(-5.00695331122746,17.8781801700861,-318.706754024377)) ;
#37616=CARTESIAN_POINT('Ctrl Pts',(-5.07085636005197,17.860160230684,-318.705898284603)) ;
#37617=CARTESIAN_POINT('Ctrl Pts',(-5.21206349339977,17.8195224623743,-318.704014250737)) ;
#37618=CARTESIAN_POINT('Ctrl Pts',(-5.28931968261299,17.7967436337499,-318.702987828093)) ;
#37619=CARTESIAN_POINT('Ctrl Pts',(-5.53741294583378,17.721835667284,-318.699702391115)) ;
#37620=CARTESIAN_POINT('Ctrl Pts',(-5.70764701574402,17.667743695579,-318.697464369429)) ;
#37621=CARTESIAN_POINT('Ctrl Pts',(-6.14563602350867,17.5215814032531,-318.691721530713)) ;
#37622=CARTESIAN_POINT('Ctrl Pts',(-6.41211301018302,17.4258275027864,-318.688242077665)) ;
#37623=CARTESIAN_POINT('Ctrl Pts',(-7.33936226880055,17.0684859878422,-318.67605949018)) ;
#37624=CARTESIAN_POINT('Ctrl Pts',(-7.98721189798678,16.7750975591633,-318.667388752436)) ;
#37625=CARTESIAN_POINT('Ctrl Pts',(-8.75432584874016,16.3731621316589,-318.656491183854)) ;
#37626=CARTESIAN_POINT('Ctrl Pts',(-8.89109464336208,16.2992973838001,-318.654524004584)) ;
#37627=CARTESIAN_POINT('Ctrl Pts',(-9.13737203238803,16.1622680436406,-318.650934540585)) ;
#37628=CARTESIAN_POINT('Ctrl Pts',(-9.2471938514487,16.0996857669079,-318.649316582503)) ;
#37629=CARTESIAN_POINT('Ctrl Pts',(-9.47093178478554,15.9691434791818,-318.645983644309)) ;
#37630=CARTESIAN_POINT('Ctrl Pts',(-9.58477591511213,15.9010742695455,-318.644267910623)) ;
#37631=CARTESIAN_POINT('Ctrl Pts',(-9.8811208305962,15.719545999035,-318.639748975747)) ;
#37632=CARTESIAN_POINT('Ctrl Pts',(-10.0623980895875,15.6041282909349,-318.63693136277)) ;
#37633=CARTESIAN_POINT('Ctrl Pts',(-10.4689874569629,15.3352242246589,-318.630492998658)) ;
#37634=CARTESIAN_POINT('Ctrl Pts',(-10.6930048253221,15.1798698213774,-318.626860292161)) ;
#37635=CARTESIAN_POINT('Ctrl Pts',(-11.1979542227078,14.8129651950213,-318.618495819203)) ;
#37636=CARTESIAN_POINT('Ctrl Pts',(-11.4764600815456,14.5982526456681,-318.61375177208)) ;
#37637=CARTESIAN_POINT('Ctrl Pts',(-11.7911611138096,14.3410608418183,-318.608281240642)) ;
#37638=CARTESIAN_POINT('Ctrl Pts',(-11.8334677611648,14.3061716481852,-318.607543484001)) ;
#37639=CARTESIAN_POINT('Ctrl Pts',(-12.1306642129733,14.058861139532,-318.602345714431)) ;
#37640=CARTESIAN_POINT('Ctrl Pts',(-12.3799744482791,13.8398274609973,-318.59790527827)) ;
#37641=CARTESIAN_POINT('Ctrl Pts',(-12.7060976809789,13.5374420106455,-318.592053327911)) ;
#37642=CARTESIAN_POINT('Ctrl Pts',(-12.7882119762277,13.4598992930987,-318.590576144318)) ;
#37643=CARTESIAN_POINT('Ctrl Pts',(-12.914289658331,13.3386455118696,-318.588305850461)) ;
#37644=CARTESIAN_POINT('Ctrl Pts',(-12.9587502015143,13.2954554153335,-318.587504809431)) ;
#37645=CARTESIAN_POINT('Ctrl Pts',(-13.054107212376,13.2018904784254,-318.585786697686)) ;
#37646=CARTESIAN_POINT('Ctrl Pts',(-13.104930218344,13.1514421759214,-318.58487091452)) ;
#37647=CARTESIAN_POINT('Ctrl Pts',(-13.2457409007182,13.0100429250027,-318.582331393171)) ;
#37648=CARTESIAN_POINT('Ctrl Pts',(-13.3350822610358,12.9184538584369,-318.580717519741)) ;
#37649=CARTESIAN_POINT('Ctrl Pts',(-13.5421371321574,12.7017529407807,-318.576961776424)) ;
#37650=CARTESIAN_POINT('Ctrl Pts',(-13.6590752301625,12.5759162634834,-318.574828574908)) ;
#37651=CARTESIAN_POINT('Ctrl Pts',(-14.1229851451993,12.0625994631588,-318.5662809536)) ;
#37652=CARTESIAN_POINT('Ctrl Pts',(-14.4553511707041,11.6622398838606,-318.55995431712)) ;
#37653=CARTESIAN_POINT('Ctrl Pts',(-14.9505217350408,11.0120260128224,-318.549897637633)) ;
#37654=CARTESIAN_POINT('Ctrl Pts',(-15.1248714250512,10.7713082318509,-318.546219969152)) ;
#37655=CARTESIAN_POINT('Ctrl Pts',(-15.4134301199703,10.3520777089572,-318.539853914446)) ;
#37656=CARTESIAN_POINT('Ctrl Pts',(-15.5304994132162,10.1756045868752,-318.537185705044)) ;
#37657=CARTESIAN_POINT('Ctrl Pts',(-15.7156502983618,9.8858627766046,-318.532815694429)) ;
#37658=CARTESIAN_POINT('Ctrl Pts',(-15.785586519244,9.77380198905806,-318.531128152536)) ;
#37659=CARTESIAN_POINT('Ctrl Pts',(-15.921054578928,9.55149031568692,-318.527784175687)) ;
#37660=CARTESIAN_POINT('Ctrl Pts',(-15.9866517133622,9.44128768204757,-318.526128356935)) ;
#37661=CARTESIAN_POINT('Ctrl Pts',(-16.1462579007195,9.16671733074994,-318.522006849643)) ;
#37662=CARTESIAN_POINT('Ctrl Pts',(-16.2389041643838,9.00157442803382,-318.519531329207)) ;
#37663=CARTESIAN_POINT('Ctrl Pts',(-16.4370412482625,8.63537566324837,-318.514050979254)) ;
#37664=CARTESIAN_POINT('Ctrl Pts',(-16.541402933734,8.43374333079441,-318.511039217987)) ;
#37665=CARTESIAN_POINT('Ctrl Pts',(-16.8886048482437,7.7316808686993,-318.500587796269)) ;
#37666=CARTESIAN_POINT('Ctrl Pts',(-17.1126401192644,7.22228557587834,-318.493056941253)) ;
#37667=CARTESIAN_POINT('Ctrl Pts',(-17.4261477460373,6.41258627639805,-318.481404513876)) ;
#37668=CARTESIAN_POINT('Ctrl Pts',(-17.5314721620727,6.11877214399491,-318.477241434961)) ;
#37669=CARTESIAN_POINT('Ctrl Pts',(-17.6596064516527,5.73080387792469,-318.471884885673)) ;
#37670=CARTESIAN_POINT('Ctrl Pts',(-17.6891571151897,5.63893019176652,-318.470626676888)) ;
#37671=CARTESIAN_POINT('Ctrl Pts',(-17.7377678891916,5.48365498363562,-318.468519914761)) ;
#37672=CARTESIAN_POINT('Ctrl Pts',(-17.7572076253362,5.42037443860558,-318.46766690355)) ;
#37673=CARTESIAN_POINT('Ctrl Pts',(-17.7997355321152,5.27925245645252,-318.465777481868)) ;
#37674=CARTESIAN_POINT('Ctrl Pts',(-17.8226523196749,5.20136095928083,-318.464743068812)) ;
#37675=CARTESIAN_POINT('Ctrl Pts',(-17.8956273485174,4.94718140774883,-318.461391520513)) ;
#37676=CARTESIAN_POINT('Ctrl Pts',(-17.9435866691828,4.77030184957938,-318.459096621088)) ;
#37677=CARTESIAN_POINT('Ctrl Pts',(-18.0619446800004,4.30671535820382,-318.453149528427)) ;
#37678=CARTESIAN_POINT('Ctrl Pts',(-18.1281377124707,4.01898822142204,-318.449524953752)) ;
#37679=CARTESIAN_POINT('Ctrl Pts',(-18.3251680355522,3.05822018577023,-318.437506739991)) ;
#37680=CARTESIAN_POINT('Ctrl Pts',(-18.4255900720567,2.37952180469889,-318.429134787705)) ;
#37681=CARTESIAN_POINT('Ctrl Pts',(-18.5043188370393,1.52171228094436,-318.418302299987)) ;
#37682=CARTESIAN_POINT('Ctrl Pts',(-18.5179020693778,1.34637539465069,-318.416076495061)) ;
#37683=CARTESIAN_POINT('Ctrl Pts',(-18.5369432144629,1.04505026301386,-318.412227400989)) ;
#37684=CARTESIAN_POINT('Ctrl Pts',(-18.5436122629388,0.919150682497201,
-318.410612040555)) ;
#37685=CARTESIAN_POINT('Ctrl Pts',(-18.5540282093306,0.67557142995478,-318.407472122584)) ;
#37686=CARTESIAN_POINT('Ctrl Pts',(-18.557939051304,0.557904717806982,-318.405948705179)) ;
#37687=CARTESIAN_POINT('Ctrl Pts',(-18.5651912253845,0.25212794626181,-318.401972420641)) ;
#37688=CARTESIAN_POINT('Ctrl Pts',(-18.5667929056849,0.0639903423706501,
-318.399508691408)) ;
#37689=CARTESIAN_POINT('Ctrl Pts',(-18.5638984000726,-0.368896367162233,
-318.393802427836)) ;
#37690=CARTESIAN_POINT('Ctrl Pts',(-18.5574218695251,-0.613597248698912,
-318.390549095427)) ;
#37691=CARTESIAN_POINT('Ctrl Pts',(-18.5143817902944,-1.54382427506486,
-318.378099834224)) ;
#37692=CARTESIAN_POINT('Ctrl Pts',(-18.4446477669696,-2.22726109135783,
-318.368764315729)) ;
#37693=CARTESIAN_POINT('Ctrl Pts',(-18.3089863403239,-3.0835194181925,-318.357243022656)) ;
#37694=CARTESIAN_POINT('Ctrl Pts',(-18.27814623129,-3.26135606137891,-318.354861264853)) ;
#37695=CARTESIAN_POINT('Ctrl Pts',(-18.2297458640308,-3.51815288053859,
-318.351451092482)) ;
#37696=CARTESIAN_POINT('Ctrl Pts',(-18.2142549483766,-3.59749227350268,
-318.350401550622)) ;
#37697=CARTESIAN_POINT('Ctrl Pts',(-18.1858442295867,-3.73811329733303,
-318.348550114836)) ;
#37698=CARTESIAN_POINT('Ctrl Pts',(-18.1731316170183,-3.79943529920401,
-318.347745848588)) ;
#37699=CARTESIAN_POINT('Ctrl Pts',(-18.158429225038,-3.8685931205935,-318.346842019715)) ;
#37700=CARTESIAN_POINT('Ctrl Pts',(-18.1567443315294,-3.87649325201482,
-318.346738818546)) ;
#37701=CARTESIAN_POINT('Ctrl Pts',(-18.1539314428153,-3.88964026281774,
-318.346567151481)) ;
#37702=CARTESIAN_POINT('Ctrl Pts',(-18.1528063275652,-3.89488775685342,
-318.3464986523)) ;
#37703=CARTESIAN_POINT('Ctrl Pts',(-18.1508174306041,-3.9041443136841,-318.346377854715)) ;
#37704=CARTESIAN_POINT('Ctrl Pts',(-18.149954595568,-3.9081535793794,-318.346325545485)) ;
#37705=CARTESIAN_POINT('Ctrl Pts',(-18.1483734457119,-3.91548876325583,
-318.346229863474)) ;
#37706=CARTESIAN_POINT('Ctrl Pts',(-18.1476555448736,-3.91881477041541,
-318.346186485996)) ;
#37707=CARTESIAN_POINT('Ctrl Pts',(-18.1463049319,-3.9250637784958,-318.346105001539)) ;
#37708=CARTESIAN_POINT('Ctrl Pts',(-18.1456724277551,-3.92798682423524,
-318.346066892216)) ;
#37709=CARTESIAN_POINT('Ctrl Pts',(-18.1444572512732,-3.93359606649929,
-318.345993772863)) ;
#37710=CARTESIAN_POINT('Ctrl Pts',(-18.1438746886403,-3.93628228669855,
-318.345958761606)) ;
#37711=CARTESIAN_POINT('Ctrl Pts',(-18.1427353884965,-3.94153001977682,
-318.345890374176)) ;
#37712=CARTESIAN_POINT('Ctrl Pts',(-18.1421787049898,-3.94409154432547,
-318.345856997402)) ;
#37713=CARTESIAN_POINT('Ctrl Pts',(-18.1410727097517,-3.9491754843671,-318.345790762332)) ;
#37714=CARTESIAN_POINT('Ctrl Pts',(-18.1405234143736,-3.95169790335584,
-318.345757903857)) ;
#37715=CARTESIAN_POINT('Ctrl Pts',(-18.1394161344572,-3.95677754672119,
-318.345691742188)) ;
#37716=CARTESIAN_POINT('Ctrl Pts',(-18.1388581352217,-3.95933476780442,
-318.345658439159)) ;
#37717=CARTESIAN_POINT('Ctrl Pts',(-18.1377176875766,-3.96455595549308,
-318.345590451913)) ;
#37718=CARTESIAN_POINT('Ctrl Pts',(-18.1371351929829,-3.96721991196936,
-318.345555768203)) ;
#37719=CARTESIAN_POINT('Ctrl Pts',(-18.1359285503817,-3.97273250071204,
-318.345484006164)) ;
#37720=CARTESIAN_POINT('Ctrl Pts',(-18.1353043180758,-3.97558111444687,
-318.345446928757)) ;
#37721=CARTESIAN_POINT('Ctrl Pts',(-18.133993709784,-3.98155519560775,-318.345369181675)) ;
#37722=CARTESIAN_POINT('Ctrl Pts',(-18.1333071968592,-3.98468063293579,
-318.345328513487)) ;
#37723=CARTESIAN_POINT('Ctrl Pts',(-18.1318459158649,-3.99132510197802,
-318.345242069256)) ;
#37724=CARTESIAN_POINT('Ctrl Pts',(-18.1310709312786,-3.99484408598062,
-318.345196295546)) ;
#37725=CARTESIAN_POINT('Ctrl Pts',(-18.1293976485544,-4.00243146873174,
-318.345097618819)) ;
#37726=CARTESIAN_POINT('Ctrl Pts',(-18.1284990052823,-4.00649979118784,
-318.345044719496)) ;
#37727=CARTESIAN_POINT('Ctrl Pts',(-18.1265293287268,-4.01540264694927,
-318.344928981165)) ;
#37728=CARTESIAN_POINT('Ctrl Pts',(-18.1254577305941,-4.02023705504703,
-318.344866148149)) ;
#37729=CARTESIAN_POINT('Ctrl Pts',(-18.1230709949504,-4.03098422284104,
-318.344726499441)) ;
#37730=CARTESIAN_POINT('Ctrl Pts',(-18.1217548976287,-4.03689676894075,
-318.344649693826)) ;
#37731=CARTESIAN_POINT('Ctrl Pts',(-18.1187728395093,-4.05026277199221,
-318.34447611454)) ;
#37732=CARTESIAN_POINT('Ctrl Pts',(-18.117105172565,-4.05771584739041,-318.344379358558)) ;
#37733=CARTESIAN_POINT('Ctrl Pts',(-18.1132570179065,-4.074864213554,-318.344156815123)) ;
#37734=CARTESIAN_POINT('Ctrl Pts',(-18.1110733439094,-4.08455878733749,
-318.344031060171)) ;
#37735=CARTESIAN_POINT('Ctrl Pts',(-18.1059391720616,-4.1072672382508,-318.343736621695)) ;
#37736=CARTESIAN_POINT('Ctrl Pts',(-18.1029824250556,-4.12027969766941,
-318.34356800057)) ;
#37737=CARTESIAN_POINT('Ctrl Pts',(-18.0750185728465,-4.24273570201157,
-318.341982050093)) ;
#37738=CARTESIAN_POINT('Ctrl Pts',(-18.0490332825581,-4.35195361406421,
-318.340574212525)) ;
#37739=CARTESIAN_POINT('Ctrl Pts',(-17.9668517425299,-4.68396528585044,
-318.336306934106)) ;
#37740=CARTESIAN_POINT('Ctrl Pts',(-17.9075088299259,-4.90595761318199,
-318.333470611908)) ;
#37741=CARTESIAN_POINT('Ctrl Pts',(-17.6252202696703,-5.88847745537046,
-318.320903469693)) ;
#37742=CARTESIAN_POINT('Ctrl Pts',(-17.3578351629958,-6.63536862936886,
-318.311275402797)) ;
#37743=CARTESIAN_POINT('Ctrl Pts',(-16.9817878734702,-7.50583971962521,
-318.299342870323)) ;
#37744=CARTESIAN_POINT('Ctrl Pts',(-16.918234904781,-7.64801130293698,-318.297371936375)) ;
#37745=CARTESIAN_POINT('Ctrl Pts',(-16.7997576900633,-7.90434598660228,
-318.293775222344)) ;
#37746=CARTESIAN_POINT('Ctrl Pts',(-16.7454391792276,-8.01877862034104,
-318.292153768767)) ;
#37747=CARTESIAN_POINT('Ctrl Pts',(-16.6389050002422,-8.23740985922531,
-318.289024407353)) ;
#37748=CARTESIAN_POINT('Ctrl Pts',(-16.5868708111661,-8.34169032315824,
-318.287517859778)) ;
#37749=CARTESIAN_POINT('Ctrl Pts',(-16.4739218003158,-8.56281266263802,
-318.2842931734)) ;
#37750=CARTESIAN_POINT('Ctrl Pts',(-16.4127379426994,-8.67950997138908,
-318.282573183366)) ;
#37751=CARTESIAN_POINT('Ctrl Pts',(-15.9857591937404,-9.47323419920945,
-318.270750914775)) ;
#37752=CARTESIAN_POINT('Ctrl Pts',(-15.5794215653148,-10.1275997121318,
-318.260347666216)) ;
#37753=CARTESIAN_POINT('Ctrl Pts',(-15.1336583262364,-10.7548540235205,
-318.25)) ;
#37754=CARTESIAN_POINT('',(-15.1169169700218,10.7783728235744,-318.25)) ;
#37755=CARTESIAN_POINT('Origin',(0.,0.,-318.25)) ;
#37756=CARTESIAN_POINT('Ctrl Pts',(-15.1169169700218,10.7783728235744,-318.25)) ;
#37757=CARTESIAN_POINT('Ctrl Pts',(-15.0804944480825,10.8294562523078,-318.250806729991)) ;
#37758=CARTESIAN_POINT('Ctrl Pts',(-15.0438190603979,10.8803466676463,-318.251609740784)) ;
#37759=CARTESIAN_POINT('Ctrl Pts',(-14.9579853298804,10.998184895247,-318.253468673654)) ;
#37760=CARTESIAN_POINT('Ctrl Pts',(-14.9086402498598,11.0649826949969,-318.254522080836)) ;
#37761=CARTESIAN_POINT('Ctrl Pts',(-14.5784009174709,11.5058037452061,-318.261478585359)) ;
#37762=CARTESIAN_POINT('Ctrl Pts',(-14.2839052146774,11.8694291017734,-318.267243743558)) ;
#37763=CARTESIAN_POINT('Ctrl Pts',(-13.6209747107106,12.6275256931051,-318.279666832644)) ;
#37764=CARTESIAN_POINT('Ctrl Pts',(-13.248436743511,13.0178446772958,-318.286323244042)) ;
#37765=CARTESIAN_POINT('Ctrl Pts',(-12.7598241901181,13.4870478312939,-318.294856579549)) ;
#37766=CARTESIAN_POINT('Ctrl Pts',(-12.6591461570025,13.5815901528953,-318.296604476164)) ;
#37767=CARTESIAN_POINT('Ctrl Pts',(-12.4700111119216,13.7552683005789,-318.299871675423)) ;
#37768=CARTESIAN_POINT('Ctrl Pts',(-12.3818319254856,13.8346962843052,-318.301388458098)) ;
#37769=CARTESIAN_POINT('Ctrl Pts',(-12.1966947945626,13.9982718639443,-318.304561025838)) ;
#37770=CARTESIAN_POINT('Ctrl Pts',(-12.0996133420859,14.0822702716743,-318.306217959224)) ;
#37771=CARTESIAN_POINT('Ctrl Pts',(-11.8645152255382,14.2814597456724,-318.3102157174)) ;
#37772=CARTESIAN_POINT('Ctrl Pts',(-11.7256815267206,14.3956662431381,-318.31256463121)) ;
#37773=CARTESIAN_POINT('Ctrl Pts',(-10.8544872507128,15.09135705424,-318.327232159744)) ;
#37774=CARTESIAN_POINT('Ctrl Pts',(-10.0807227641066,15.6188334184307,-318.340025544145)) ;
#37775=CARTESIAN_POINT('Ctrl Pts',(-9.08320412226288,16.1937225475383,-318.355554114097)) ;
#37776=CARTESIAN_POINT('Ctrl Pts',(-8.89400347550464,16.2984032805629,-318.358455446921)) ;
#37777=CARTESIAN_POINT('Ctrl Pts',(-8.60845672260143,16.4499371486907,-318.362748276585)) ;
#37778=CARTESIAN_POINT('Ctrl Pts',(-8.5134635221799,16.4992999319676,-318.364162380739)) ;
#37779=CARTESIAN_POINT('Ctrl Pts',(-8.39152923399645,16.5613291071284,-318.365957300581)) ;
#37780=CARTESIAN_POINT('Ctrl Pts',(-8.36497743171584,16.5747560237762,-318.366346934525)) ;
#37781=CARTESIAN_POINT('Ctrl Pts',(-8.32742032269198,16.5936349546005,-318.366896285397)) ;
#37782=CARTESIAN_POINT('Ctrl Pts',(-8.31644171426074,16.5991399611761,-318.367056655943)) ;
#37783=CARTESIAN_POINT('Ctrl Pts',(-8.29492316239464,16.6099033071463,-318.367370563337)) ;
#37784=CARTESIAN_POINT('Ctrl Pts',(-8.28438366125306,16.6151625178938,-318.367524111155)) ;
#37785=CARTESIAN_POINT('Ctrl Pts',(-8.26717845326089,16.6237274756253,-318.367774439919)) ;
#37786=CARTESIAN_POINT('Ctrl Pts',(-8.26051575240305,16.6270392513593,-318.367871298751)) ;
#37787=CARTESIAN_POINT('Ctrl Pts',(-8.24983555684862,16.6323399671715,-318.36802643134)) ;
#37788=CARTESIAN_POINT('Ctrl Pts',(-8.24581932980345,16.634331458729,-318.368084738526)) ;
#37789=CARTESIAN_POINT('Ctrl Pts',(-8.18861115537183,16.6626729685035,-318.368914858298)) ;
#37790=CARTESIAN_POINT('Ctrl Pts',(-8.1352937953847,16.6887692176808,-318.369683285192)) ;
#37791=CARTESIAN_POINT('Ctrl Pts',(-8.01968606929195,16.744667893812,-318.371337613913)) ;
#37792=CARTESIAN_POINT('Ctrl Pts',(-7.95735283482998,16.7743793745763,-318.372222345166)) ;
#37793=CARTESIAN_POINT('Ctrl Pts',(-7.79236082525833,16.8518971083591,-318.374546844281)) ;
#37794=CARTESIAN_POINT('Ctrl Pts',(-7.68942784001788,16.8991130812709,-318.375979424839)) ;
#37795=CARTESIAN_POINT('Ctrl Pts',(-7.12736806461566,17.1507346594597,-318.383721888176)) ;
#37796=CARTESIAN_POINT('Ctrl Pts',(-6.66051661901487,17.337375700734,-318.389869841283)) ;
#37797=CARTESIAN_POINT('Ctrl Pts',(-5.81707614590315,17.635469527898,-318.400840395687)) ;
#37798=CARTESIAN_POINT('Ctrl Pts',(-5.44343991918518,17.7543550083848,-318.405652938792)) ;
#37799=CARTESIAN_POINT('Ctrl Pts',(-4.8810697088908,17.9138699693625,-318.412920224449)) ;
#37800=CARTESIAN_POINT('Ctrl Pts',(-4.69501173579473,17.9635309289428,-318.415327935294)) ;
#37801=CARTESIAN_POINT('Ctrl Pts',(-4.38050282546227,18.0422566993248,-318.419411484194)) ;
#37802=CARTESIAN_POINT('Ctrl Pts',(-4.25245416643611,18.0728654428255,-318.421077777132)) ;
#37803=CARTESIAN_POINT('Ctrl Pts',(-4.01051882246542,18.1279840655623,-318.42423499826)) ;
#37804=CARTESIAN_POINT('Ctrl Pts',(-3.89670584611696,18.1527890698395,-318.425723933116)) ;
#37805=CARTESIAN_POINT('Ctrl Pts',(-3.65877194330506,18.2023048557559,-318.428845269554)) ;
#37806=CARTESIAN_POINT('Ctrl Pts',(-3.53461654536178,18.2268208971872,-318.430478870912)) ;
#37807=CARTESIAN_POINT('Ctrl Pts',(-3.22719365502355,18.2842661584178,-318.434536451853)) ;
#37808=CARTESIAN_POINT('Ctrl Pts',(-3.04366311077679,18.3157113577331,-318.436969901929)) ;
#37809=CARTESIAN_POINT('Ctrl Pts',(-2.27776241053797,18.4351069440466,-318.447168610217)) ;
#37810=CARTESIAN_POINT('Ctrl Pts',(-1.69184858502896,18.4980814588032,-318.455086823874)) ;
#37811=CARTESIAN_POINT('Ctrl Pts',(-0.596788143931648,18.5633094174577,
-318.469870661373)) ;
#37812=CARTESIAN_POINT('Ctrl Pts',(-0.0886155740524386,18.5726884753098,
-318.476722158459)) ;
#37813=CARTESIAN_POINT('Ctrl Pts',(0.520446927102541,18.5589296618443,-318.484719967855)) ;
#37814=CARTESIAN_POINT('Ctrl Pts',(0.621572978063025,18.5558180168559,-318.486040563542)) ;
#37815=CARTESIAN_POINT('Ctrl Pts',(0.789256073556296,18.5492861013175,-318.488215355147)) ;
#37816=CARTESIAN_POINT('Ctrl Pts',(0.855829086489303,18.5463337786349,-318.489074790814)) ;
#37817=CARTESIAN_POINT('Ctrl Pts',(1.00110580434746,18.5391072834794,-318.490940999427)) ;
#37818=CARTESIAN_POINT('Ctrl Pts',(1.07980094253777,18.5346902225778,-318.491946199504)) ;
#37819=CARTESIAN_POINT('Ctrl Pts',(1.32423476406868,18.5194084275355,-318.495053688154)) ;
#37820=CARTESIAN_POINT('Ctrl Pts',(1.48985763389259,18.5068206510279,-318.49713821824)) ;
#37821=CARTESIAN_POINT('Ctrl Pts',(2.29840258448145,18.4344447563835,-318.507253006644)) ;
#37822=CARTESIAN_POINT('Ctrl Pts',(2.93807602782849,18.3433672413775,-318.51508049397)) ;
#37823=CARTESIAN_POINT('Ctrl Pts',(3.84160384304844,18.1662386140285,-318.526419542586)) ;
#37824=CARTESIAN_POINT('Ctrl Pts',(4.11029517597141,18.107336046666,-318.529825362182)) ;
#37825=CARTESIAN_POINT('Ctrl Pts',(4.58807701960243,17.9914136966011,-318.535972908446)) ;
#37826=CARTESIAN_POINT('Ctrl Pts',(4.79766558568324,17.936661401507,-318.538701387193)) ;
#37827=CARTESIAN_POINT('Ctrl Pts',(5.13506523197348,17.8421831495394,-318.543153613366)) ;
#37828=CARTESIAN_POINT('Ctrl Pts',(5.26348894196061,17.8047206822806,-318.544862382922)) ;
#37829=CARTESIAN_POINT('Ctrl Pts',(5.5136780625553,17.7287945678808,-318.548220312384)) ;
#37830=CARTESIAN_POINT('Ctrl Pts',(5.63547381165989,17.6904561125664,-318.549868553271)) ;
#37831=CARTESIAN_POINT('Ctrl Pts',(5.93598431759697,17.5924440175862,-318.553969487297)) ;
#37832=CARTESIAN_POINT('Ctrl Pts',(6.1142044638569,17.5313005773715,-318.55643181362)) ;
#37833=CARTESIAN_POINT('Ctrl Pts',(6.64595668316723,17.3397730033988,-318.563867606771)) ;
#37834=CARTESIAN_POINT('Ctrl Pts',(6.99648067898841,17.2013291650822,-318.568890111049)) ;
#37835=CARTESIAN_POINT('Ctrl Pts',(7.79254290494892,16.8585531381439,-318.580518963213)) ;
#37836=CARTESIAN_POINT('Ctrl Pts',(8.23469113401574,16.6470538043224,-318.587145676751)) ;
#37837=CARTESIAN_POINT('Ctrl Pts',(8.81609980789244,16.3401024373588,-318.595926855089)) ;
#37838=CARTESIAN_POINT('Ctrl Pts',(8.96317956412928,16.2598885515971,-318.598153619319)) ;
#37839=CARTESIAN_POINT('Ctrl Pts',(9.21884671867051,16.1159303803091,-318.602022216398)) ;
#37840=CARTESIAN_POINT('Ctrl Pts',(9.32790887175798,16.0530515168696,-318.60367175563)) ;
#37841=CARTESIAN_POINT('Ctrl Pts',(9.49805628517949,15.952635035051,-318.606239122047)) ;
#37842=CARTESIAN_POINT('Ctrl Pts',(9.55957791798111,15.9158445520717,-318.607166159245)) ;
#37843=CARTESIAN_POINT('Ctrl Pts',(9.67432929580857,15.8463168262155,-318.608891749969)) ;
#37844=CARTESIAN_POINT('Ctrl Pts',(9.7276097919673,15.8136653568912,-318.609691485485)) ;
#37845=CARTESIAN_POINT('Ctrl Pts',(9.87932726954172,15.7196326104818,-318.61196590319)) ;
#37846=CARTESIAN_POINT('Ctrl Pts',(9.97735528193598,15.6575968254532,-318.613432024187)) ;
#37847=CARTESIAN_POINT('Ctrl Pts',(10.4124171795256,15.3765285940358,-318.61993684575)) ;
#37848=CARTESIAN_POINT('Ctrl Pts',(10.7428673430728,15.1475036200241,-318.624874309655)) ;
#37849=CARTESIAN_POINT('Ctrl Pts',(11.4392363981211,14.630613894219,-318.635501819375)) ;
#37850=CARTESIAN_POINT('Ctrl Pts',(11.8022924624233,14.3393474287269,-318.641185621807)) ;
#37851=CARTESIAN_POINT('Ctrl Pts',(12.2614842130961,13.941689740524,-318.648714630063)) ;
#37852=CARTESIAN_POINT('Ctrl Pts',(12.3678737358538,13.8473971246321,-318.650483707777)) ;
#37853=CARTESIAN_POINT('Ctrl Pts',(12.6298718970273,13.609760912265,-318.654907636104)) ;
#37854=CARTESIAN_POINT('Ctrl Pts',(12.7841329818794,13.4649619346898,-318.657573073036)) ;
#37855=CARTESIAN_POINT('Ctrl Pts',(13.0302631450031,13.2258857100484,-318.661933668541)) ;
#37856=CARTESIAN_POINT('Ctrl Pts',(13.1236635202806,13.1332123332325,-318.663614482381)) ;
#37857=CARTESIAN_POINT('Ctrl Pts',(13.3045094654124,12.9499182721772,-318.666921759855)) ;
#37858=CARTESIAN_POINT('Ctrl Pts',(13.392033802588,12.8593851310248,-318.668547368957)) ;
#37859=CARTESIAN_POINT('Ctrl Pts',(13.5855118747432,12.6551381231626,-318.672197759126)) ;
#37860=CARTESIAN_POINT('Ctrl Pts',(13.6909723504897,12.5409700507982,-318.674226722456)) ;
#37861=CARTESIAN_POINT('Ctrl Pts',(14.2732844650016,11.8944774778714,-318.685650738065)) ;
#37862=CARTESIAN_POINT('Ctrl Pts',(14.7205210233672,11.3362911184259,-318.69529739059)) ;
#37863=CARTESIAN_POINT('Ctrl Pts',(15.2993019893397,10.5217322075699,-318.708755512442)) ;
#37864=CARTESIAN_POINT('Ctrl Pts',(15.4587849136962,10.285983634175,-318.712579501153)) ;
#37865=CARTESIAN_POINT('Ctrl Pts',(15.7097043879317,9.89604796700484,-318.718742919378)) ;
#37866=CARTESIAN_POINT('Ctrl Pts',(15.8044387785662,9.74403881422784,-318.721106763069)) ;
#37867=CARTESIAN_POINT('Ctrl Pts',(15.9384277147384,9.52194652831368,-318.724491941304)) ;
#37868=CARTESIAN_POINT('Ctrl Pts',(15.9794502044216,9.45294212901537,-318.725534286593)) ;
#37869=CARTESIAN_POINT('Ctrl Pts',(16.053453600627,9.32660182750237,-318.727424000042)) ;
#37870=CARTESIAN_POINT('Ctrl Pts',(16.0865780189105,9.26935174596814,-318.728273207419)) ;
#37871=CARTESIAN_POINT('Ctrl Pts',(16.1675446721413,9.12767306130208,-318.730358195759)) ;
#37872=CARTESIAN_POINT('Ctrl Pts',(16.2150322632963,9.04304401068473,-318.731589353394)) ;
#37873=CARTESIAN_POINT('Ctrl Pts',(16.4150211196561,8.67999726425118,-318.73681774899)) ;
#37874=CARTESIAN_POINT('Ctrl Pts',(16.5610319771791,8.39806475392093,-318.740746362187)) ;
#37875=CARTESIAN_POINT('Ctrl Pts',(16.8915132772734,7.71776470182411,-318.750048222256)) ;
#37876=CARTESIAN_POINT('Ctrl Pts',(17.0692260987333,7.31632650772171,-318.755398222172)) ;
#37877=CARTESIAN_POINT('Ctrl Pts',(17.336815034305,6.64889858287995,-318.764247519535)) ;
#37878=CARTESIAN_POINT('Ctrl Pts',(17.435182949256,6.38650163104886,-318.767714539907)) ;
#37879=CARTESIAN_POINT('Ctrl Pts',(17.5998078872297,5.91517109759757,-318.77395375779)) ;
#37880=CARTESIAN_POINT('Ctrl Pts',(17.6683753383254,5.70710079120582,-318.776711868424)) ;
#37881=CARTESIAN_POINT('Ctrl Pts',(17.772801633614,5.37027610886836,-318.781191453457)) ;
#37882=CARTESIAN_POINT('Ctrl Pts',(17.8109803999193,5.24226292022075,-318.782897288386)) ;
#37883=CARTESIAN_POINT('Ctrl Pts',(17.8825714032875,4.9924041401712,-318.786234527583)) ;
#37884=CARTESIAN_POINT('Ctrl Pts',(17.9161280021315,4.87060740051896,-318.787864856509)) ;
#37885=CARTESIAN_POINT('Ctrl Pts',(17.9878719651966,4.59942741508577,-318.791503119001)) ;
#37886=CARTESIAN_POINT('Ctrl Pts',(18.025446825523,4.44989179961282,-318.793514950972)) ;
#37887=CARTESIAN_POINT('Ctrl Pts',(18.25433226632,3.48849039844217,-318.806483433725)) ;
#37888=CARTESIAN_POINT('Ctrl Pts',(18.392609251568,2.6649807815381,-318.817796297087)) ;
#37889=CARTESIAN_POINT('Ctrl Pts',(18.4902689215981,1.68171798566272,-318.831046357692)) ;
#37890=CARTESIAN_POINT('Ctrl Pts',(18.5035834900991,1.52827297112301,-318.833105091512)) ;
#37891=CARTESIAN_POINT('Ctrl Pts',(18.5284746013748,1.19302505287816,-318.837572730536)) ;
#37892=CARTESIAN_POINT('Ctrl Pts',(18.5392878163098,1.01118113964923,-318.839976677257)) ;
#37893=CARTESIAN_POINT('Ctrl Pts',(18.5510529277244,0.748023208970792,-318.843414310031)) ;
#37894=CARTESIAN_POINT('Ctrl Pts',(18.5541493988392,0.666815985553406,-318.844469427861)) ;
#37895=CARTESIAN_POINT('Ctrl Pts',(18.5588082255007,0.519183065203262,-318.846375644876)) ;
#37896=CARTESIAN_POINT('Ctrl Pts',(18.5605473543417,0.452764519066003,-318.847228669419)) ;
#37897=CARTESIAN_POINT('Ctrl Pts',(18.5639567475703,0.288957371814897,-318.849321956189)) ;
#37898=CARTESIAN_POINT('Ctrl Pts',(18.5652172202946,0.191562238656035,-318.850557587054)) ;
#37899=CARTESIAN_POINT('Ctrl Pts',(18.5673482578771,-0.228611399058598,
-318.855857258373)) ;
#37900=CARTESIAN_POINT('Ctrl Pts',(18.5605676962895,-0.551373037934079,
-318.859850299482)) ;
#37901=CARTESIAN_POINT('Ctrl Pts',(18.5451378280777,-0.87885608722279,-318.863881370167)) ;
#37902=CARTESIAN_POINT('Ctrl Pts',(18.5448972467379,-0.883918091233771,
-318.863943674443)) ;
#37903=CARTESIAN_POINT('Ctrl Pts',(18.5446545937441,-0.888979977966575,
-318.864005972278)) ;
#37904=CARTESIAN_POINT('Origin',(0.,0.,-315.477129595899)) ;
#37905=CARTESIAN_POINT('',(18.5446554538441,-0.88896203566046,-320.660059650531)) ;
#37906=CARTESIAN_POINT('Ctrl Pts',(18.5446550920983,-0.888969581938671,
-320.660059750084)) ;
#37907=CARTESIAN_POINT('Ctrl Pts',(18.589273190788,0.0418015803997639,-320.647780645843)) ;
#37908=CARTESIAN_POINT('Ctrl Pts',(18.5637543137461,0.974592717322047,-320.635048004708)) ;
#37909=CARTESIAN_POINT('Ctrl Pts',(18.4549963209679,2.03089251855565,-320.620930538161)) ;
#37910=CARTESIAN_POINT('Ctrl Pts',(18.4403171247722,2.16011991256673,-320.61921007732)) ;
#37911=CARTESIAN_POINT('Ctrl Pts',(18.4144686995445,2.36815865994873,-320.616456413024)) ;
#37912=CARTESIAN_POINT('Ctrl Pts',(18.4041483514296,2.44707098477785,-320.615415644062)) ;
#37913=CARTESIAN_POINT('Ctrl Pts',(18.3849139688139,2.58713279723982,-320.613576463609)) ;
#37914=CARTESIAN_POINT('Ctrl Pts',(18.3762014213575,2.64830872146057,-320.612775896959)) ;
#37915=CARTESIAN_POINT('Ctrl Pts',(18.3574013160327,2.77575386891301,-320.611114668359)) ;
#37916=CARTESIAN_POINT('Ctrl Pts',(18.3472599694369,2.84201411374271,-320.610254836975)) ;
#37917=CARTESIAN_POINT('Ctrl Pts',(18.3233706743031,2.99263977822422,-320.608308017056)) ;
#37918=CARTESIAN_POINT('Ctrl Pts',(18.3093984815837,3.07696814729683,-320.60722356865)) ;
#37919=CARTESIAN_POINT('Ctrl Pts',(18.24532625923,3.44777430354018,-320.602473901092)) ;
#37920=CARTESIAN_POINT('Ctrl Pts',(18.1890812345201,3.73314914096403,-320.598867527116)) ;
#37921=CARTESIAN_POINT('Ctrl Pts',(18.0018010468585,4.57820712232696,-320.58820688783)) ;
#37922=CARTESIAN_POINT('Ctrl Pts',(17.851457819502,5.13325201940272,-320.58122097992)) ;
#37923=CARTESIAN_POINT('Ctrl Pts',(17.6052489297788,5.89937261776771,-320.571270868736)) ;
#37924=CARTESIAN_POINT('Ctrl Pts',(17.5308245118115,6.11699099811218,-320.56841032899)) ;
#37925=CARTESIAN_POINT('Ctrl Pts',(17.3901414750641,6.50467256229697,-320.563236576897)) ;
#37926=CARTESIAN_POINT('Ctrl Pts',(17.325381681515,6.67524794360466,-320.560932778364)) ;
#37927=CARTESIAN_POINT('Ctrl Pts',(17.2148320344999,6.95398033901283,-320.557118248154)) ;
#37928=CARTESIAN_POINT('Ctrl Pts',(17.1705113447932,7.06270660917089,-320.555617666966)) ;
#37929=CARTESIAN_POINT('Ctrl Pts',(17.0769180642834,7.28621783382526,-320.552505817593)) ;
#37930=CARTESIAN_POINT('Ctrl Pts',(17.0275123717725,7.40094070191585,-320.550893675624)) ;
#37931=CARTESIAN_POINT('Ctrl Pts',(16.9024095239062,7.68355161479172,-320.546884729432)) ;
#37932=CARTESIAN_POINT('Ctrl Pts',(16.825364968578,7.85082840492873,-320.544478631442)) ;
#37933=CARTESIAN_POINT('Ctrl Pts',(16.5007865651158,8.52881097617581,-320.534592602845)) ;
#37934=CARTESIAN_POINT('Ctrl Pts',(16.2323875959267,9.02918396261254,-320.526972447014)) ;
#37935=CARTESIAN_POINT('Ctrl Pts',(15.7564942678808,9.8263752974343,-320.514466441475)) ;
#37936=CARTESIAN_POINT('Ctrl Pts',(15.562497289475,10.1308164298362,-320.509600472102)) ;
#37937=CARTESIAN_POINT('Ctrl Pts',(15.2785972371669,10.5489258171139,-320.502866547339)) ;
#37938=CARTESIAN_POINT('Ctrl Pts',(15.1960520378454,10.667491363163,-320.500951231677)) ;
#37939=CARTESIAN_POINT('Ctrl Pts',(15.0515141518069,10.8700188566082,-320.497677234812)) ;
#37940=CARTESIAN_POINT('Ctrl Pts',(14.9901818155747,10.9544437278829,-320.496311739768)) ;
#37941=CARTESIAN_POINT('Ctrl Pts',(14.9271528348508,11.0396834379257,-320.494934189799)) ;
#37942=CARTESIAN_POINT('Ctrl Pts',(14.9261645412174,11.0410196201761,-320.494912596184)) ;
#37943=CARTESIAN_POINT('Ctrl Pts',(14.9241562792725,11.0437340467001,-320.494868729797)) ;
#37944=CARTESIAN_POINT('Ctrl Pts',(14.9231362994197,11.0451122824231,-320.494846457182)) ;
#37945=CARTESIAN_POINT('Ctrl Pts',(14.9210653351239,11.047909837906,-320.494801248676)) ;
#37946=CARTESIAN_POINT('Ctrl Pts',(14.9200143390571,11.0493291490419,-320.494778312942)) ;
#37947=CARTESIAN_POINT('Ctrl Pts',(14.9185678653785,11.0512819477927,-320.494746756654)) ;
#37948=CARTESIAN_POINT('Ctrl Pts',(14.9181725617037,11.0518155640936,-320.494738133721)) ;
#37949=CARTESIAN_POINT('Ctrl Pts',(14.9173082735625,11.0529821267643,-320.494719282846)) ;
#37950=CARTESIAN_POINT('Ctrl Pts',(14.9168392774149,11.0536150645315,-320.494709055064)) ;
#37951=CARTESIAN_POINT('Ctrl Pts',(14.8909803290288,11.0885085868346,-320.494145206794)) ;
#37952=CARTESIAN_POINT('Ctrl Pts',(14.8654724419213,11.1226816425733,-320.493593208123)) ;
#37953=CARTESIAN_POINT('Ctrl Pts',(14.799905728718,11.2098932904887,-320.492185341768)) ;
#37954=CARTESIAN_POINT('Ctrl Pts',(14.7596795019669,11.2628050749281,-320.491332168469)) ;
#37955=CARTESIAN_POINT('Ctrl Pts',(14.65914671431,11.3935778395313,-320.489225123336)) ;
#37956=CARTESIAN_POINT('Ctrl Pts',(14.5985031018322,11.4711771673058,-320.487976077157)) ;
#37957=CARTESIAN_POINT('Ctrl Pts',(14.3220776007096,11.8191477389605,-320.482372436743)) ;
#37958=CARTESIAN_POINT('Ctrl Pts',(14.0993818595498,12.0839394396551,-320.478099739798)) ;
#37959=CARTESIAN_POINT('Ctrl Pts',(13.4114930507716,12.8569375986979,-320.465389141573)) ;
#37960=CARTESIAN_POINT('Ctrl Pts',(12.9252851988334,13.34563575612,-320.457012916148)) ;
#37961=CARTESIAN_POINT('Ctrl Pts',(12.2511605211432,13.9517367518548,-320.445682427678)) ;
#37962=CARTESIAN_POINT('Ctrl Pts',(12.0867254424444,14.0944301178278,-320.442941156745)) ;
#37963=CARTESIAN_POINT('Ctrl Pts',(11.8177536497681,14.3196690143079,-320.438484336524)) ;
#37964=CARTESIAN_POINT('Ctrl Pts',(11.7147717603235,14.4040391747493,-320.436784210811)) ;
#37965=CARTESIAN_POINT('Ctrl Pts',(11.5125001822917,14.5661504206842,-320.433455716434)) ;
#37966=CARTESIAN_POINT('Ctrl Pts',(11.4133081972689,14.6440019962394,-320.43182839283)) ;
#37967=CARTESIAN_POINT('Ctrl Pts',(11.1911749538968,14.8147169423849,-320.428194514757)) ;
#37968=CARTESIAN_POINT('Ctrl Pts',(11.0678552826335,14.9070726260846,-320.426184037137)) ;
#37969=CARTESIAN_POINT('Ctrl Pts',(10.3566271446436,15.426029508022,-320.414629628021)) ;
#37970=CARTESIAN_POINT('Ctrl Pts',(9.74523493849762,15.8193710177711,-320.404825468476)) ;
#37971=CARTESIAN_POINT('Ctrl Pts',(8.87248368166176,16.3110191454446,-320.391344698482)) ;
#37972=CARTESIAN_POINT('Ctrl Pts',(8.62961130768387,16.4408065868858,-320.387648695088)) ;
#37973=CARTESIAN_POINT('Ctrl Pts',(8.22732415650954,16.6444119517029,-320.38166000695)) ;
#37974=CARTESIAN_POINT('Ctrl Pts',(8.06958941796149,16.7214544464697,-320.379344713582)) ;
#37975=CARTESIAN_POINT('Ctrl Pts',(7.83835967058113,16.8303602521073,-320.376010160024)) ;
#37976=CARTESIAN_POINT('Ctrl Pts',(7.76571364613351,16.8640030873791,-320.374970995909)) ;
#37977=CARTESIAN_POINT('Ctrl Pts',(7.63232953628261,16.9247294659801,-320.373080012037)) ;
#37978=CARTESIAN_POINT('Ctrl Pts',(7.57165935167884,16.9519584798445,-320.372226446842)) ;
#37979=CARTESIAN_POINT('Ctrl Pts',(7.42052451758098,17.0188151541721,-320.370115506499)) ;
#37980=CARTESIAN_POINT('Ctrl Pts',(7.32988745247924,17.0580480519605,-320.368863002112)) ;
#37981=CARTESIAN_POINT('Ctrl Pts',(6.98951781796482,17.2021657276769,-320.364202622321)) ;
#37982=CARTESIAN_POINT('Ctrl Pts',(6.73781223802198,17.3023048136194,-320.360842253274)) ;
#37983=CARTESIAN_POINT('Ctrl Pts',(5.93778281974094,17.6004840858427,-320.350320760546)) ;
#37984=CARTESIAN_POINT('Ctrl Pts',(5.38227495244984,17.7782288933439,-320.343237744653)) ;
#37985=CARTESIAN_POINT('Ctrl Pts',(4.66513129355442,17.9709917254191,-320.334056974556)) ;
#37986=CARTESIAN_POINT('Ctrl Pts',(4.51040734500845,18.0104474983281,-320.332074898616)) ;
#37987=CARTESIAN_POINT('Ctrl Pts',(4.13253098029535,18.1016339849885,-320.327223142056)) ;
#37988=CARTESIAN_POINT('Ctrl Pts',(3.9088931648892,18.1512401554142,-320.324342303235)) ;
#37989=CARTESIAN_POINT('Ctrl Pts',(3.55196154187433,18.223510262761,-320.319719289467)) ;
#37990=CARTESIAN_POINT('Ctrl Pts',(3.41923926590918,18.2488783181322,-320.317994848141)) ;
#37991=CARTESIAN_POINT('Ctrl Pts',(3.16173591308726,18.2951887432147,-320.314637295797)) ;
#37992=CARTESIAN_POINT('Ctrl Pts',(3.03699427155919,18.31630887691,-320.313005456138)) ;
#37993=CARTESIAN_POINT('Ctrl Pts',(2.7637991500359,18.3596962199525,-320.309419383519)) ;
#37994=CARTESIAN_POINT('Ctrl Pts',(2.61527175868124,18.3814413083073,-320.307461892687)) ;
#37995=CARTESIAN_POINT('Ctrl Pts',(2.00412125681012,18.4633591186382,-320.29937603076)) ;
#37996=CARTESIAN_POINT('Ctrl Pts',(1.53957503955576,18.5078858438168,-320.293151697139)) ;
#37997=CARTESIAN_POINT('Ctrl Pts',(0.609758023463925,18.5617562867355,-320.280633701536)) ;
#37998=CARTESIAN_POINT('Ctrl Pts',(0.144822765875304,18.5712042559841,-320.274345079612)) ;
#37999=CARTESIAN_POINT('Ctrl Pts',(-0.483448678337892,18.5603746770248,
-320.265951934022)) ;
#38000=CARTESIAN_POINT('Ctrl Pts',(-0.64687756191638,18.5553976059387,-320.263778772134)) ;
#38001=CARTESIAN_POINT('Ctrl Pts',(-0.933632067622933,18.5428716840832,
-320.259994451255)) ;
#38002=CARTESIAN_POINT('Ctrl Pts',(-1.0569879404011,18.5362492349128,-320.258375881455)) ;
#38003=CARTESIAN_POINT('Ctrl Pts',(-1.25085233263537,18.5238999705078,-320.255851612869)) ;
#38004=CARTESIAN_POINT('Ctrl Pts',(-1.32140983208596,18.5190004523242,-320.254936960759)) ;
#38005=CARTESIAN_POINT('Ctrl Pts',(-1.46329132091133,18.5083332051818,-320.253107099174)) ;
#38006=CARTESIAN_POINT('Ctrl Pts',(-1.53461341402841,18.5025560723666,-320.252192002265)) ;
#38007=CARTESIAN_POINT('Ctrl Pts',(-1.7331711968201,18.4853167938127,-320.249655611776)) ;
#38008=CARTESIAN_POINT('Ctrl Pts',(-1.86032474652054,18.4729535073326,-320.248044153148)) ;
#38009=CARTESIAN_POINT('Ctrl Pts',(-2.18891480000634,18.4375772401306,-320.243902744987)) ;
#38010=CARTESIAN_POINT('Ctrl Pts',(-2.39012021708224,18.4125752693644,-320.241389082151)) ;
#38011=CARTESIAN_POINT('Ctrl Pts',(-3.17771190458831,18.3015808766074,-320.231580719873)) ;
#38012=CARTESIAN_POINT('Ctrl Pts',(-3.76025159372194,18.1908280487864,-320.22438269932)) ;
#38013=CARTESIAN_POINT('Ctrl Pts',(-4.49291909800089,18.0148288294783,-320.215068573923)) ;
#38014=CARTESIAN_POINT('Ctrl Pts',(-4.64884789006029,17.9752216397224,-320.21307187091)) ;
#38015=CARTESIAN_POINT('Ctrl Pts',(-5.02660179785301,17.8740248956172,-320.208191434611)) ;
#38016=CARTESIAN_POINT('Ctrl Pts',(-5.24783404764432,17.8103264746178,-320.205296515049)) ;
#38017=CARTESIAN_POINT('Ctrl Pts',(-5.59714391020538,17.7026775184402,-320.200656734144)) ;
#38018=CARTESIAN_POINT('Ctrl Pts',(-5.726023917642,17.6614116452616,-320.198929846528)) ;
#38019=CARTESIAN_POINT('Ctrl Pts',(-5.97441671540665,17.5788744734997,-320.19557104091)) ;
#38020=CARTESIAN_POINT('Ctrl Pts',(-6.09398184177534,17.5377840134527,-320.19394043432)) ;
#38021=CARTESIAN_POINT('Ctrl Pts',(-6.38062886402289,17.4359878823611,-320.18999722914)) ;
#38022=CARTESIAN_POINT('Ctrl Pts',(-6.54727667816326,17.3740975618289,-320.187676705245)) ;
#38023=CARTESIAN_POINT('Ctrl Pts',(-7.47566094617769,17.0140561907429,-320.174593799675)) ;
#38024=CARTESIAN_POINT('Ctrl Pts',(-8.21793022773138,16.668209995275,-320.163497308287)) ;
#38025=CARTESIAN_POINT('Ctrl Pts',(-9.11946161975605,16.1732563144482,-320.149700286211)) ;
#38026=CARTESIAN_POINT('Ctrl Pts',(-9.30222620421671,16.0688328105123,-320.146888760632)) ;
#38027=CARTESIAN_POINT('Ctrl Pts',(-9.60980196023276,15.8860913964448,-320.142153922907)) ;
#38028=CARTESIAN_POINT('Ctrl Pts',(-9.73552850381538,15.809354143702,-320.14021756961)) ;
#38029=CARTESIAN_POINT('Ctrl Pts',(-9.92408759345924,15.691164621376,-320.137319661557)) ;
#38030=CARTESIAN_POINT('Ctrl Pts',(-9.98760295331322,15.6508130461312,-320.136344591362)) ;
#38031=CARTESIAN_POINT('Ctrl Pts',(-10.1074959309155,15.5736174671756,-320.134507434476)) ;
#38032=CARTESIAN_POINT('Ctrl Pts',(-10.1639217189721,15.5368507197949,-320.133644376945)) ;
#38033=CARTESIAN_POINT('Ctrl Pts',(-10.3110873954476,15.4398135395337,-320.131396121166)) ;
#38034=CARTESIAN_POINT('Ctrl Pts',(-10.4014991978202,15.3790500325348,-320.130017546942)) ;
#38035=CARTESIAN_POINT('Ctrl Pts',(-11.0314674816962,14.947567513022,-320.120413206063)) ;
#38036=CARTESIAN_POINT('Ctrl Pts',(-11.5516223402338,14.5493325418654,-320.112472518047)) ;
#38037=CARTESIAN_POINT('Ctrl Pts',(-12.4098739769892,13.8171531071765,-320.098624350499)) ;
#38038=CARTESIAN_POINT('Ctrl Pts',(-12.7582035519693,13.4961821565171,-320.092771396495)) ;
#38039=CARTESIAN_POINT('Ctrl Pts',(-13.210279238432,13.0464546345825,-320.084735021276)) ;
#38040=CARTESIAN_POINT('Ctrl Pts',(-13.3251361475084,12.9291222683097,-320.082653044646)) ;
#38041=CARTESIAN_POINT('Ctrl Pts',(-13.524467222832,12.7200171912822,-320.078965034228)) ;
#38042=CARTESIAN_POINT('Ctrl Pts',(-13.609601197605,12.6288877656985,-320.077365046512)) ;
#38043=CARTESIAN_POINT('Ctrl Pts',(-13.7891506476407,12.432769534724,-320.073936245527)) ;
#38044=CARTESIAN_POINT('Ctrl Pts',(-13.8832996604095,12.3275473777791,-320.072105242701)) ;
#38045=CARTESIAN_POINT('Ctrl Pts',(-14.1453171039769,12.0279041359731,-320.066914913687)) ;
#38046=CARTESIAN_POINT('Ctrl Pts',(-14.3103639000479,11.8310590611469,-320.063532611767)) ;
#38047=CARTESIAN_POINT('Ctrl Pts',(-14.5884607006544,11.4850470709389,-320.057640630475)) ;
#38048=CARTESIAN_POINT('Ctrl Pts',(-14.7034378217574,11.3374780237061,-320.055144017861)) ;
#38049=CARTESIAN_POINT('Ctrl Pts',(-15.1423860606155,10.7561931504176,-320.045385567056)) ;
#38050=CARTESIAN_POINT('Ctrl Pts',(-15.4495560737919,10.3101291325037,-320.038050697572)) ;
#38051=CARTESIAN_POINT('Ctrl Pts',(-15.8036135586821,9.7445449137338,-320.029126962571)) ;
#38052=CARTESIAN_POINT('Ctrl Pts',(-15.869344240706,9.6371297856845,-320.027448693463)) ;
#38053=CARTESIAN_POINT('Ctrl Pts',(-16.0159828418118,9.39192852465593,-320.023661159842)) ;
#38054=CARTESIAN_POINT('Ctrl Pts',(-16.09621519664,9.25374974218617,-320.021557437177)) ;
#38055=CARTESIAN_POINT('Ctrl Pts',(-16.2126786293103,9.0470741267786,-320.018465439613)) ;
#38056=CARTESIAN_POINT('Ctrl Pts',(-16.2502806143696,8.97935847200445,-320.017460954369)) ;
#38057=CARTESIAN_POINT('Ctrl Pts',(-16.3193593926118,8.85310260965741,-320.015605429166)) ;
#38058=CARTESIAN_POINT('Ctrl Pts',(-16.3509476261824,8.79462497883068,-320.014753007017)) ;
#38059=CARTESIAN_POINT('Ctrl Pts',(-16.4308440345105,8.6447985383438,-320.012585677615)) ;
#38060=CARTESIAN_POINT('Ctrl Pts',(-16.4787048552872,8.55321365298748,-320.011276468719)) ;
#38061=CARTESIAN_POINT('Ctrl Pts',(-16.6441670106533,8.23004633564286,-320.006703927432)) ;
#38062=CARTESIAN_POINT('Ctrl Pts',(-16.7576713070831,7.99639987874069,-320.003482091307)) ;
#38063=CARTESIAN_POINT('Ctrl Pts',(-17.1103923121456,7.22981073568241,-319.993082327014)) ;
#38064=CARTESIAN_POINT('Ctrl Pts',(-17.3293701326168,6.68794591498471,-319.985985262188)) ;
#38065=CARTESIAN_POINT('Ctrl Pts',(-17.575264584893,5.98582625184031,-319.976788184808)) ;
#38066=CARTESIAN_POINT('Ctrl Pts',(-17.6261398215666,5.83431538943539,-319.974804301298)) ;
#38067=CARTESIAN_POINT('Ctrl Pts',(-17.7451986765086,5.46396872089428,-319.969948997443)) ;
#38068=CARTESIAN_POINT('Ctrl Pts',(-17.8112982585629,5.24449085423753,-319.967066415359)) ;
#38069=CARTESIAN_POINT('Ctrl Pts',(-17.909887055619,4.89374186637616,-319.962441325652)) ;
#38070=CARTESIAN_POINT('Ctrl Pts',(-17.9450350776897,4.76324257159204,-319.960716581303)) ;
#38071=CARTESIAN_POINT('Ctrl Pts',(-18.0103186816377,4.50986954630541,-319.95735887546)) ;
#38072=CARTESIAN_POINT('Ctrl Pts',(-18.0406293564702,4.38704851890468,-319.9557271903)) ;
#38073=CARTESIAN_POINT('Ctrl Pts',(-18.1041437654839,4.11788699634963,-319.952141989477)) ;
#38074=CARTESIAN_POINT('Ctrl Pts',(-18.1368333566289,3.97143431291526,-319.950185222726)) ;
#38075=CARTESIAN_POINT('Ctrl Pts',(-18.2637127848125,3.36872762743181,-319.942108617553)) ;
#38076=CARTESIAN_POINT('Ctrl Pts',(-18.3424887783077,2.90940435395312,-319.935893105163)) ;
#38077=CARTESIAN_POINT('Ctrl Pts',(-18.4652698419783,1.98619602934424,-319.923375897237)) ;
#38078=CARTESIAN_POINT('Ctrl Pts',(-18.5092606437092,1.52264088932407,-319.917078982594)) ;
#38079=CARTESIAN_POINT('Ctrl Pts',(-18.5451061496133,0.894595137415581,
-319.908676350537)) ;
#38080=CARTESIAN_POINT('Ctrl Pts',(-18.5522689205552,0.73115017494928,-319.906501870915)) ;
#38081=CARTESIAN_POINT('Ctrl Pts',(-18.5610490294874,0.44410695793475,-319.902715543493)) ;
#38082=CARTESIAN_POINT('Ctrl Pts',(-18.5635939829878,0.320547305205466,
-319.901096274562)) ;
#38083=CARTESIAN_POINT('Ctrl Pts',(-18.5656555770196,0.126238340883433,
-319.898571178995)) ;
#38084=CARTESIAN_POINT('Ctrl Pts',(-18.5660017969246,0.0555015476074166,
-319.897656389765)) ;
#38085=CARTESIAN_POINT('Ctrl Pts',(-18.565892430471,-0.0777715679331076,
-319.895942380189)) ;
#38086=CARTESIAN_POINT('Ctrl Pts',(-18.5655251508092,-0.140306960566763,
-319.8951420525)) ;
#38087=CARTESIAN_POINT('Ctrl Pts',(-18.5635716173354,-0.319103830453604,
-319.892863653786)) ;
#38088=CARTESIAN_POINT('Ctrl Pts',(-18.5612091587844,-0.435353963888956,
-319.891394174298)) ;
#38089=CARTESIAN_POINT('Ctrl Pts',(-18.5441401948836,-1.00964037652752,
-319.884178693673)) ;
#38090=CARTESIAN_POINT('Ctrl Pts',(-18.5135703148142,-1.46704658749342,
-319.878565864524)) ;
#38091=CARTESIAN_POINT('Ctrl Pts',(-18.4216939222867,-2.34938104204668,
-319.867700069148)) ;
#38092=CARTESIAN_POINT('Ctrl Pts',(-18.3625155757877,-2.77424216081369,
-319.862450586824)) ;
#38093=CARTESIAN_POINT('Ctrl Pts',(-18.2396021542069,-3.47744987903692,
-319.853591866354)) ;
#38094=CARTESIAN_POINT('Ctrl Pts',(-18.1840656208683,-3.75706020909621,
-319.850024908786)) ;
#38095=CARTESIAN_POINT('Ctrl Pts',(-18.0907345996278,-4.17620217944348,
-319.844589062615)) ;
#38096=CARTESIAN_POINT('Ctrl Pts',(-18.0577126689862,-4.31675295616627,
-319.842751183851)) ;
#38097=CARTESIAN_POINT('Ctrl Pts',(-17.9932269219158,-4.57752368870319,
-319.839311280314)) ;
#38098=CARTESIAN_POINT('Ctrl Pts',(-17.9621889324688,-4.69784066218678,
-319.837712177261)) ;
#38099=CARTESIAN_POINT('Ctrl Pts',(-17.8886843298084,-4.97139361828649,
-319.834048425729)) ;
#38100=CARTESIAN_POINT('Ctrl Pts',(-17.8454522205785,-5.12441377104221,
-319.831978780777)) ;
#38101=CARTESIAN_POINT('Ctrl Pts',(-17.6940060998695,-5.63528208216325,
-319.825001598787)) ;
#38102=CARTESIAN_POINT('Ctrl Pts',(-17.5769511157485,-5.99041269765255,
-319.820037838604)) ;
#38103=CARTESIAN_POINT('Ctrl Pts',(-17.2603757059369,-6.861464245383,-319.807628695331)) ;
#38104=CARTESIAN_POINT('Ctrl Pts',(-17.0483734140392,-7.37246388527609,
-319.800134949259)) ;
#38105=CARTESIAN_POINT('Ctrl Pts',(-16.7599433945097,-7.98842756413033,
-319.791037471443)) ;
#38106=CARTESIAN_POINT('Ctrl Pts',(-16.704822356033,-8.10306038711319,-319.789342052749)) ;
#38107=CARTESIAN_POINT('Ctrl Pts',(-16.5773406620451,-8.36134833742875,
-319.785523086718)) ;
#38108=CARTESIAN_POINT('Ctrl Pts',(-16.5042822578401,-8.50464794964898,
-319.783405070073)) ;
#38109=CARTESIAN_POINT('Ctrl Pts',(-16.3932121144931,-8.71568261505193,
-319.780296587227)) ;
#38110=CARTESIAN_POINT('Ctrl Pts',(-16.3566226176274,-8.78415752611084,
-319.779289671204)) ;
#38111=CARTESIAN_POINT('Ctrl Pts',(-16.2879425561549,-8.91077079807433,
-319.777432454845)) ;
#38112=CARTESIAN_POINT('Ctrl Pts',(-16.2559675707652,-8.96897024506396,
-319.776580739249)) ;
#38113=CARTESIAN_POINT('Ctrl Pts',(-16.1820483866412,-9.10182076837794,
-319.774640078183)) ;
#38114=CARTESIAN_POINT('Ctrl Pts',(-16.139898573098,-9.17635577798928,-319.773553776277)) ;
#38115=CARTESIAN_POINT('Ctrl Pts',(-15.9512794075741,-9.50457752352469,
-319.768775824324)) ;
#38116=CARTESIAN_POINT('Ctrl Pts',(-15.7993333548143,-9.75506919028073,
-319.765143881003)) ;
#38117=CARTESIAN_POINT('Ctrl Pts',(-15.3328906526168,-10.484520915646,-319.754481175163)) ;
#38118=CARTESIAN_POINT('Ctrl Pts',(-15.002082097532,-10.9526365997029,-319.747517034356)) ;
#38119=CARTESIAN_POINT('Ctrl Pts',(-14.5528637001184,-11.5296897142065,
-319.738474438905)) ;
#38120=CARTESIAN_POINT('Ctrl Pts',(-14.4539724684033,-11.6534229559753,
-319.736507892625)) ;
#38121=CARTESIAN_POINT('Ctrl Pts',(-14.2090024684019,-11.9520147148731,
-319.731686649185)) ;
#38122=CARTESIAN_POINT('Ctrl Pts',(-14.0612649826143,-12.1254787001854,
-319.728820825041)) ;
#38123=CARTESIAN_POINT('Ctrl Pts',(-13.8210240906026,-12.3972574560836,
-319.72421569102)) ;
#38124=CARTESIAN_POINT('Ctrl Pts',(-13.7305764707638,-12.4973584833696,
-319.722493860154)) ;
#38125=CARTESIAN_POINT('Ctrl Pts',(-13.5531442360367,-12.6894763878504,
-319.719137606224)) ;
#38126=CARTESIAN_POINT('Ctrl Pts',(-13.4662933705959,-12.7816068036632,
-319.717504411412)) ;
#38127=CARTESIAN_POINT('Ctrl Pts',(-13.2741031281485,-12.9813465810857,
-319.713910725803)) ;
#38128=CARTESIAN_POINT('Ctrl Pts',(-13.1683831970627,-13.0885773406175,
-319.711946917912)) ;
#38129=CARTESIAN_POINT('Ctrl Pts',(-12.7379436134082,-13.5146735673453,
-319.704003837386)) ;
#38130=CARTESIAN_POINT('Ctrl Pts',(-12.4028549722467,-13.8228360181523,
-319.697934104992)) ;
#38131=CARTESIAN_POINT('Ctrl Pts',(-11.6974120629538,-14.4252689156461,
-319.685469289314)) ;
#38132=CARTESIAN_POINT('Ctrl Pts',(-11.3264540185173,-14.7183311354844,
-319.679075101517)) ;
#38133=CARTESIAN_POINT('Ctrl Pts',(-10.8116620103455,-15.0940252359024,
-319.670561337337)) ;
#38134=CARTESIAN_POINT('Ctrl Pts',(-10.6773175397551,-15.1893555993554,
-319.668371545987)) ;
#38135=CARTESIAN_POINT('Ctrl Pts',(-10.4394931789651,-15.3534004271312,
-319.6645619171)) ;
#38136=CARTESIAN_POINT('Ctrl Pts',(-10.3365590904613,-15.4228878215087,
-319.662934538102)) ;
#38137=CARTESIAN_POINT('Ctrl Pts',(-10.173813684113,-15.5303906930307,-319.660399847607)) ;
#38138=CARTESIAN_POINT('Ctrl Pts',(-10.1144687461817,-15.5691053680162,
-319.659483465818)) ;
#38139=CARTESIAN_POINT('Ctrl Pts',(-10.002405234924,-15.6413007412492,-319.657768944831)) ;
#38140=CARTESIAN_POINT('Ctrl Pts',(-9.94973653430783,-15.6748570096053,
-319.656969675867)) ;
#38141=CARTESIAN_POINT('Ctrl Pts',(-9.79895508253931,-15.7698566859488,
-319.654698711009)) ;
#38142=CARTESIAN_POINT('Ctrl Pts',(-9.70043552433415,-15.8306491119577,
-319.653235518469)) ;
#38143=CARTESIAN_POINT('Ctrl Pts',(-9.40632503290428,-16.0083562950231,
-319.64891953732)) ;
#38144=CARTESIAN_POINT('Ctrl Pts',(-9.20914307031659,-16.1225961346538,
-319.646093371657)) ;
#38145=CARTESIAN_POINT('Ctrl Pts',(-8.64613809009402,-16.4350810524499,
-319.638154393099)) ;
#38146=CARTESIAN_POINT('Ctrl Pts',(-8.27568391531246,-16.6246999785226,
-319.633080757162)) ;
#38147=CARTESIAN_POINT('Ctrl Pts',(-7.5688576005142,-16.9570079515821,-319.623492563115)) ;
#38148=CARTESIAN_POINT('Ctrl Pts',(-7.23403506658379,-17.1025278850562,
-319.618988307289)) ;
#38149=CARTESIAN_POINT('Ctrl Pts',(-6.6972691184655,-17.3172314106357,-319.611758369888)) ;
#38150=CARTESIAN_POINT('Ctrl Pts',(-6.49804868953566,-17.3929664053021,
-319.609073489313)) ;
#38151=CARTESIAN_POINT('Ctrl Pts',(-6.17309444926559,-17.5101374257881,
-319.604683771035)) ;
#38152=CARTESIAN_POINT('Ctrl Pts',(-6.04814383133484,-17.5536880422411,
-319.602993458984)) ;
#38153=CARTESIAN_POINT('Ctrl Pts',(-5.80277073989572,-17.6362800502884,
-319.599668181251)) ;
#38154=CARTESIAN_POINT('Ctrl Pts',(-5.68239329096042,-17.6754329142077,
-319.59803408364)) ;
#38155=CARTESIAN_POINT('Ctrl Pts',(-5.41250614154726,-17.7601718807105,
-319.594363822718)) ;
#38156=CARTESIAN_POINT('Ctrl Pts',(-5.26280218775656,-17.8051071605327,
-319.592323450258)) ;
#38157=CARTESIAN_POINT('Ctrl Pts',(-4.43492343116874,-18.0422505832194,
-319.581016970826)) ;
#38158=CARTESIAN_POINT('Ctrl Pts',(-3.74679571311203,-18.1976060495182,
-319.571509207816)) ;
#38159=CARTESIAN_POINT('Ctrl Pts',(-2.77012693716534,-18.3603450587266,
-319.558180557617)) ;
#38160=CARTESIAN_POINT('Ctrl Pts',(-2.48770068963297,-18.4007396459706,
-319.554349056747)) ;
#38161=CARTESIAN_POINT('Ctrl Pts',(-2.02628186463724,-18.4559172401889,
-319.54817395547)) ;
#38162=CARTESIAN_POINT('Ctrl Pts',(-1.84780794830388,-18.4746395189185,
-319.545806134378)) ;
#38163=CARTESIAN_POINT('Ctrl Pts',(-1.58874576667963,-18.4980240611802,
-319.542411836864)) ;
#38164=CARTESIAN_POINT('Ctrl Pts',(-1.50835451975316,-18.5047527393947,
-319.541364490148)) ;
#38165=CARTESIAN_POINT('Ctrl Pts',(-1.36174630030572,-18.5160619918388,
-319.539466910562)) ;
#38166=CARTESIAN_POINT('Ctrl Pts',(-1.29554393291029,-18.520811823039,-319.538614824716)) ;
#38167=CARTESIAN_POINT('Ctrl Pts',(-1.13185198966875,-18.531674285358,-319.536518965107)) ;
#38168=CARTESIAN_POINT('Ctrl Pts',(-1.03433692062121,-18.5373727350905,
-319.535279887093)) ;
#38169=CARTESIAN_POINT('Ctrl Pts',(-0.609092997731742,-18.5588566148113,
-319.52990989548)) ;
#38170=CARTESIAN_POINT('Ctrl Pts',(-0.281022531967197,-18.5667223936328,
-319.525852426534)) ;
#38171=CARTESIAN_POINT('Ctrl Pts',(0.184118473903266,-18.5655427690672,
-319.520134623313)) ;
#38172=CARTESIAN_POINT('Ctrl Pts',(0.32114476542577,-18.5636780833577,-319.518454656876)) ;
#38173=CARTESIAN_POINT('Ctrl Pts',(0.906303355729485,-18.5492341708577,
-319.511283498925)) ;
#38174=CARTESIAN_POINT('Ctrl Pts',(1.35392106694975,-18.5219429732882,-319.505801602371)) ;
#38175=CARTESIAN_POINT('Ctrl Pts',(1.93881339966618,-18.4649647457342,-319.498513547611)) ;
#38176=CARTESIAN_POINT('Ctrl Pts',(2.07735962557479,-18.4498915279457,-319.496778316142)) ;
#38177=CARTESIAN_POINT('Ctrl Pts',(2.4232214954552,-18.4083180858861,-319.492419424493)) ;
#38178=CARTESIAN_POINT('Ctrl Pts',(2.63028384640021,-18.3798744239215,-319.489785269557)) ;
#38179=CARTESIAN_POINT('Ctrl Pts',(2.96687142071308,-18.3278337687785,-319.485455853957)) ;
#38180=CARTESIAN_POINT('Ctrl Pts',(3.09670373300719,-18.3063443268507,-319.483774328255)) ;
#38181=CARTESIAN_POINT('Ctrl Pts',(3.35144072665906,-18.261393517356,-319.480451165037)) ;
#38182=CARTESIAN_POINT('Ctrl Pts',(3.47635483074433,-18.2380263508963,-319.478810229669)) ;
#38183=CARTESIAN_POINT('Ctrl Pts',(3.78749123606108,-18.1765106842142,-319.474694034491)) ;
#38184=CARTESIAN_POINT('Ctrl Pts',(3.97338594814523,-18.1367812592745,-319.472208647292)) ;
#38185=CARTESIAN_POINT('Ctrl Pts',(4.51494083217563,-18.0123143075917,-319.464893868234)) ;
#38186=CARTESIAN_POINT('Ctrl Pts',(4.86874678467191,-17.9199180008609,-319.460019296871)) ;
#38187=CARTESIAN_POINT('Ctrl Pts',(5.61655142170223,-17.7008459997476,-319.449560612637)) ;
#38188=CARTESIAN_POINT('Ctrl Pts',(6.00951244052909,-17.5713220583901,-319.443969806547)) ;
#38189=CARTESIAN_POINT('Ctrl Pts',(6.69232682536536,-17.3206721569203,-319.434207699202)) ;
#38190=CARTESIAN_POINT('Ctrl Pts',(6.9840484788382,-17.2051152236083,-319.430022090306)) ;
#38191=CARTESIAN_POINT('Ctrl Pts',(7.36171656553722,-17.0443242295472,-319.42464046336)) ;
#38192=CARTESIAN_POINT('Ctrl Pts',(7.45043366801918,-17.0057313112646,-319.423379084769)) ;
#38193=CARTESIAN_POINT('Ctrl Pts',(7.59940488049363,-16.939537669084,-319.42126824932)) ;
#38194=CARTESIAN_POINT('Ctrl Pts',(7.65982011193505,-16.9123045994988,-319.420414305255)) ;
#38195=CARTESIAN_POINT('Ctrl Pts',(7.79396136092571,-16.8509721901524,-319.418523451429)) ;
#38196=CARTESIAN_POINT('Ctrl Pts',(7.86761186664843,-16.8167113607032,-319.417488532541)) ;
#38197=CARTESIAN_POINT('Ctrl Pts',(8.10650110863314,-16.7036717068692,-319.414138908742)) ;
#38198=CARTESIAN_POINT('Ctrl Pts',(8.27080026357403,-16.6229321097865,-319.411846339661)) ;
#38199=CARTESIAN_POINT('Ctrl Pts',(8.69638681670377,-16.4059191721764,-319.405907796482)) ;
#38200=CARTESIAN_POINT('Ctrl Pts',(8.95567135540168,-16.2658316285078,-319.402289274278)) ;
#38201=CARTESIAN_POINT('Ctrl Pts',(9.80633387742465,-15.7797232771298,-319.39028165961)) ;
#38202=CARTESIAN_POINT('Ctrl Pts',(10.381886077836,-15.4071506637186,-319.381914294169)) ;
#38203=CARTESIAN_POINT('Ctrl Pts',(11.0774515813883,-14.900181513698,-319.371089710774)) ;
#38204=CARTESIAN_POINT('Ctrl Pts',(11.2179016110272,-14.7947296694031,-319.368866679468)) ;
#38205=CARTESIAN_POINT('Ctrl Pts',(11.4566050793388,-14.6101541862775,-319.365019752049)) ;
#38206=CARTESIAN_POINT('Ctrl Pts',(11.5555871827429,-14.5319926403659,-319.363403729201)) ;
#38207=CARTESIAN_POINT('Ctrl Pts',(11.7596883324532,-14.3674195379613,-319.360026884995)) ;
#38208=CARTESIAN_POINT('Ctrl Pts',(11.864669301118,-14.2808485799772,-319.358264795079)) ;
#38209=CARTESIAN_POINT('Ctrl Pts',(12.1479463653666,-14.0419685916833,-319.353440471498)) ;
#38210=CARTESIAN_POINT('Ctrl Pts',(12.3243235517851,-13.8874235009306,-319.350359918428)) ;
#38211=CARTESIAN_POINT('Ctrl Pts',(12.7275846140105,-13.5203440707657,-319.343141018793)) ;
#38212=CARTESIAN_POINT('Ctrl Pts',(12.9521523391632,-13.3053697101697,-319.338985534863)) ;
#38213=CARTESIAN_POINT('Ctrl Pts',(13.6407228177951,-12.6122548185456,-319.325860348181)) ;
#38214=CARTESIAN_POINT('Ctrl Pts',(14.0844514653631,-12.1147231422276,-319.316812260794)) ;
#38215=CARTESIAN_POINT('Ctrl Pts',(14.5705253646179,-11.5068184638548,-319.306572258987)) ;
#38216=CARTESIAN_POINT('Ctrl Pts',(14.6397775653115,-11.4185810614698,-319.305105374053)) ;
#38217=CARTESIAN_POINT('Ctrl Pts',(14.745969058318,-11.2807234377254,-319.302847068333)) ;
#38218=CARTESIAN_POINT('Ctrl Pts',(14.7834671033498,-11.231537079516,-319.302047844628)) ;
#38219=CARTESIAN_POINT('Ctrl Pts',(14.8639491190266,-11.124867092156,-319.300329470611)) ;
#38220=CARTESIAN_POINT('Ctrl Pts',(14.9068469414477,-11.0673197077355,-319.299411641926)) ;
#38221=CARTESIAN_POINT('Ctrl Pts',(15.0258371940304,-10.9057474257479,-319.296858298652)) ;
#38222=CARTESIAN_POINT('Ctrl Pts',(15.1011817947939,-10.8011767312512,-319.295232829479)) ;
#38223=CARTESIAN_POINT('Ctrl Pts',(15.275425437824,-10.5539567868967,-319.291443501416)) ;
#38224=CARTESIAN_POINT('Ctrl Pts',(15.3734250283514,-10.4106882194146,-319.289288527965)) ;
#38225=CARTESIAN_POINT('Ctrl Pts',(15.7641603301079,-9.8219095264266,-319.280560743145)) ;
#38226=CARTESIAN_POINT('Ctrl Pts',(16.0396538267447,-9.36526370183947,-319.274078941908)) ;
#38227=CARTESIAN_POINT('Ctrl Pts',(16.4035580828228,-8.69879218013309,-319.26472978127)) ;
#38228=CARTESIAN_POINT('Ctrl Pts',(16.5083598094517,-8.49822095449446,-319.261931090967)) ;
#38229=CARTESIAN_POINT('Ctrl Pts',(16.7178267743022,-8.07883505314419,-319.256089054779)) ;
#38230=CARTESIAN_POINT('Ctrl Pts',(16.8219233848406,-7.85978378745533,-319.253043061591)) ;
#38231=CARTESIAN_POINT('Ctrl Pts',(16.9782519439022,-7.51347810882402,-319.248223499294)) ;
#38232=CARTESIAN_POINT('Ctrl Pts',(17.0334118875921,-7.38757549961326,-319.246470563163)) ;
#38233=CARTESIAN_POINT('Ctrl Pts',(17.1363014433096,-7.14544993472415,-319.243096539011)) ;
#38234=CARTESIAN_POINT('Ctrl Pts',(17.1842594079578,-7.02933214983275,-319.241477171997)) ;
#38235=CARTESIAN_POINT('Ctrl Pts',(17.2950886627656,-6.7530735753301,-319.237620909285)) ;
#38236=CARTESIAN_POINT('Ctrl Pts',(17.3569198759194,-6.59252810801264,-319.235376999484)) ;
#38237=CARTESIAN_POINT('Ctrl Pts',(17.6149749324984,-5.89367627372671,-319.225598438985)) ;
#38238=CARTESIAN_POINT('Ctrl Pts',(17.788452638621,-5.34730871639522,-319.217915196714)) ;
#38239=CARTESIAN_POINT('Ctrl Pts',(18.0737427564873,-4.27987248603568,-319.203034167735)) ;
#38240=CARTESIAN_POINT('Ctrl Pts',(18.1889466423228,-3.76028014806394,-319.195849853529)) ;
#38241=CARTESIAN_POINT('Ctrl Pts',(18.3010007757784,-3.12732376796146,-319.187395377202)) ;
#38242=CARTESIAN_POINT('Ctrl Pts',(18.31934380851,-3.01801686980458,-319.185946268824)) ;
#38243=CARTESIAN_POINT('Ctrl Pts',(18.3463625236249,-2.847679797751,-319.183708439823)) ;
#38244=CARTESIAN_POINT('Ctrl Pts',(18.3557148824173,-2.78675963328895,-319.182912139066)) ;
#38245=CARTESIAN_POINT('Ctrl Pts',(18.3753571557655,-2.65442178406473,-319.181191952716)) ;
#38246=CARTESIAN_POINT('Ctrl Pts',(18.3855344372085,-2.58298840221,-319.180269455555)) ;
#38247=CARTESIAN_POINT('Ctrl Pts',(18.4129916835092,-2.38187963893132,-319.177687144177)) ;
#38248=CARTESIAN_POINT('Ctrl Pts',(18.4293178689586,-2.25207822311147,-319.17603773838)) ;
#38249=CARTESIAN_POINT('Ctrl Pts',(18.4645347151988,-1.94599252276742,-319.172178934301)) ;
#38250=CARTESIAN_POINT('Ctrl Pts',(18.4822748975798,-1.76958862527774,-319.169978865435)) ;
#38251=CARTESIAN_POINT('Ctrl Pts',(18.5176691574958,-1.35858909876342,-319.164885897476)) ;
#38252=CARTESIAN_POINT('Ctrl Pts',(18.5333937718384,-1.1238874679167,-319.162002294695)) ;
#38253=CARTESIAN_POINT('Ctrl Pts',(18.5446545942648,-0.888979967104711,
-319.159121327827)) ;
#38254=CARTESIAN_POINT('',(18.5446545933324,-0.888979986554686,-320.363441000746)) ;
#38255=CARTESIAN_POINT('Ctrl Pts',(18.5446545937441,-0.888979977966572,
-318.864005972278)) ;
#38256=CARTESIAN_POINT('Ctrl Pts',(18.5239048097641,-1.3218328951763,-318.869333195369)) ;
#38257=CARTESIAN_POINT('Ctrl Pts',(18.4880064180289,-1.75382819271705,-318.874616863806)) ;
#38258=CARTESIAN_POINT('Ctrl Pts',(18.4044894733845,-2.45881100342708,-318.88335565816)) ;
#38259=CARTESIAN_POINT('Ctrl Pts',(18.3658215259591,-2.73268799347742,-318.886778748155)) ;
#38260=CARTESIAN_POINT('Ctrl Pts',(18.2859291398535,-3.21968332545473,-318.892947460273)) ;
#38261=CARTESIAN_POINT('Ctrl Pts',(18.247058481313,-3.43313585008995,-318.895679448152)) ;
#38262=CARTESIAN_POINT('Ctrl Pts',(18.1783537986686,-3.77619129929169,-318.900124312305)) ;
#38263=CARTESIAN_POINT('Ctrl Pts',(18.1508526438783,-3.90624062201917,-318.901821897016)) ;
#38264=CARTESIAN_POINT('Ctrl Pts',(18.0945574417779,-4.15901155331034,-318.905147258973)) ;
#38265=CARTESIAN_POINT('Ctrl Pts',(18.0659054235743,-4.28175749982331,-318.90677401269)) ;
#38266=CARTESIAN_POINT('Ctrl Pts',(17.9923492921944,-4.58298319144293,-318.910796174569)) ;
#38267=CARTESIAN_POINT('Ctrl Pts',(17.9460370604387,-4.76110508698323,-318.913200715102)) ;
#38268=CARTESIAN_POINT('Ctrl Pts',(17.7265757794533,-5.5564296008708,-318.924052056488)) ;
#38269=CARTESIAN_POINT('Ctrl Pts',(17.5241802006144,-6.16510352217633,-318.932685717344)) ;
#38270=CARTESIAN_POINT('Ctrl Pts',(17.1769661461046,-7.05293303398665,-318.945526639362)) ;
#38271=CARTESIAN_POINT('Ctrl Pts',(17.0558999419879,-7.34086560802061,-318.949728053781)) ;
#38272=CARTESIAN_POINT('Ctrl Pts',(16.8497562788778,-7.79847157723484,-318.956405112556)) ;
#38273=CARTESIAN_POINT('Ctrl Pts',(16.7692403530135,-7.97013323646255,-318.958909612272)) ;
#38274=CARTESIAN_POINT('Ctrl Pts',(16.6500923380935,-8.21435767579969,-318.96245758868)) ;
#38275=CARTESIAN_POINT('Ctrl Pts',(16.6135858120306,-8.28794385748215,-318.963524590733)) ;
#38276=CARTESIAN_POINT('Ctrl Pts',(16.546846235046,-8.42025781307905,-318.965437823793)) ;
#38277=CARTESIAN_POINT('Ctrl Pts',(16.5167859451356,-8.47907093999281,-318.966286174342)) ;
#38278=CARTESIAN_POINT('Ctrl Pts',(16.4427167561653,-8.6220991529967,-318.968344868961)) ;
#38279=CARTESIAN_POINT('Ctrl Pts',(16.3983739621138,-8.70613918814556,-318.969550937377)) ;
#38280=CARTESIAN_POINT('Ctrl Pts',(16.2205951974769,-9.03689454864697,-318.974290075635)) ;
#38281=CARTESIAN_POINT('Ctrl Pts',(16.0822205171451,-9.28091350691477,-318.977770166413)) ;
#38282=CARTESIAN_POINT('Ctrl Pts',(15.6399177203402,-10.0212837031289,-318.988397161506)) ;
#38283=CARTESIAN_POINT('Ctrl Pts',(15.3181414640535,-10.5065549443357,-318.995468369947)) ;
#38284=CARTESIAN_POINT('Ctrl Pts',(14.8797779206677,-11.1046011832239,-319.004635630996)) ;
#38285=CARTESIAN_POINT('Ctrl Pts',(14.783794185736,-11.2320696137224,-319.006616357578)) ;
#38286=CARTESIAN_POINT('Ctrl Pts',(14.5461054389716,-11.5393994283668,-319.011465613476)) ;
#38287=CARTESIAN_POINT('Ctrl Pts',(14.4026933545458,-11.7179070856838,-319.014345302267)) ;
#38288=CARTESIAN_POINT('Ctrl Pts',(14.1694589055316,-11.997465981152,-319.018967081999)) ;
#38289=CARTESIAN_POINT('Ctrl Pts',(14.0817712212364,-12.1002675529442,-319.020691460425)) ;
#38290=CARTESIAN_POINT('Ctrl Pts',(13.9098038311551,-12.297474089388,-319.024049279851)) ;
#38291=CARTESIAN_POINT('Ctrl Pts',(13.8256655979386,-12.3919926694717,-319.02568145373)) ;
#38292=CARTESIAN_POINT('Ctrl Pts',(13.639572904166,-12.5967894220402,-319.029268804922)) ;
#38293=CARTESIAN_POINT('Ctrl Pts',(13.5372333057059,-12.7067055954676,-319.031227247094)) ;
#38294=CARTESIAN_POINT('Ctrl Pts',(13.0724397191812,-13.1939204721091,-319.040057222058)) ;
#38295=CARTESIAN_POINT('Ctrl Pts',(12.6954692369816,-13.5570378521579,-319.047053511322)) ;
#38296=CARTESIAN_POINT('Ctrl Pts',(11.9251716007837,-14.2386876796208,-319.060895070699)) ;
#38297=CARTESIAN_POINT('Ctrl Pts',(11.5331545114255,-14.5580318682217,-319.067730678607)) ;
#38298=CARTESIAN_POINT('Ctrl Pts',(10.9973180109475,-14.9592912561138,-319.076609754852)) ;
#38299=CARTESIAN_POINT('Ctrl Pts',(10.8647411462511,-15.055855947113,-319.07877023523)) ;
#38300=CARTESIAN_POINT('Ctrl Pts',(10.6670956887502,-15.1958442549146,-319.081927826572)) ;
#38301=CARTESIAN_POINT('Ctrl Pts',(10.603004345948,-15.2406335798324,-319.082942097779)) ;
#38302=CARTESIAN_POINT('Ctrl Pts',(10.4834563925153,-15.3230588660487,-319.08481465851)) ;
#38303=CARTESIAN_POINT('Ctrl Pts',(10.4280753705299,-15.3608018997376,-319.085674355254)) ;
#38304=CARTESIAN_POINT('Ctrl Pts',(10.3016989706831,-15.4459309617981,-319.087619519784)) ;
#38305=CARTESIAN_POINT('Ctrl Pts',(10.2305786917239,-15.4931289486109,-319.088702465644)) ;
#38306=CARTESIAN_POINT('Ctrl Pts',(9.91942702799352,-15.6965437156434,-319.093394791924)) ;
#38307=CARTESIAN_POINT('Ctrl Pts',(9.67612421714811,-15.8476855722377,-319.096947218304)) ;
#38308=CARTESIAN_POINT('Ctrl Pts',(8.93132554843639,-16.2868127060859,-319.107598774921)) ;
#38309=CARTESIAN_POINT('Ctrl Pts',(8.41978122199558,-16.5570567921206,-319.114626111497)) ;
#38310=CARTESIAN_POINT('Ctrl Pts',(7.75249401370287,-16.8706443234602,-319.123742170205)) ;
#38311=CARTESIAN_POINT('Ctrl Pts',(7.60766347017833,-16.9364476727888,-319.125717009088)) ;
#38312=CARTESIAN_POINT('Ctrl Pts',(7.25278532580786,-17.0922149173546,-319.13055458758)) ;
#38313=CARTESIAN_POINT('Ctrl Pts',(7.04188822126367,-17.1801779900213,-319.133428469975)) ;
#38314=CARTESIAN_POINT('Ctrl Pts',(6.70385988599226,-17.3138960061632,-319.138043293821)) ;
#38315=CARTESIAN_POINT('Ctrl Pts',(6.57776006256005,-17.3621946993573,-319.139766622674)) ;
#38316=CARTESIAN_POINT('Ctrl Pts',(6.33246014012001,-17.4530933715797,-319.143123834731)) ;
#38317=CARTESIAN_POINT('Ctrl Pts',(6.21332904144026,-17.4958584194064,-319.144756467252)) ;
#38318=CARTESIAN_POINT('Ctrl Pts',(5.92497661617308,-17.5960530429265,-319.148714024358)) ;
#38319=CARTESIAN_POINT('Ctrl Pts',(5.7553454206456,-17.6522641474869,-319.151047022867)) ;
#38320=CARTESIAN_POINT('Ctrl Pts',(5.19428110401107,-17.8292381395432,-319.158777857256)) ;
#38321=CARTESIAN_POINT('Ctrl Pts',(4.79966281914314,-17.9394962072996,-319.164240477413)) ;
#38322=CARTESIAN_POINT('Ctrl Pts',(4.34704079716518,-18.0499557855242,-319.170497486158)) ;
#38323=CARTESIAN_POINT('Ctrl Pts',(4.2922988829226,-18.0630517313536,-319.171254036483)) ;
#38324=CARTESIAN_POINT('Ctrl Pts',(4.00531255431341,-18.1303293866809,-319.175218521963)) ;
#38325=CARTESIAN_POINT('Ctrl Pts',(3.77209965359929,-18.1802815296054,-319.178434477915)) ;
#38326=CARTESIAN_POINT('Ctrl Pts',(3.26537600469475,-18.2786470384953,-319.185381663846)) ;
#38327=CARTESIAN_POINT('Ctrl Pts',(2.99160923062968,-18.3254438562568,-319.189109913104)) ;
#38328=CARTESIAN_POINT('Ctrl Pts',(2.54231816375434,-18.3919075158911,-319.195143130723)) ;
#38329=CARTESIAN_POINT('Ctrl Pts',(2.36738082938012,-18.4152423800399,-319.197471087954)) ;
#38330=CARTESIAN_POINT('Ctrl Pts',(2.1124902818856,-18.4455500741961,-319.200820085025)) ;
#38331=CARTESIAN_POINT('Ctrl Pts',(2.03278269999845,-18.4545042536832,-319.201861259473)) ;
#38332=CARTESIAN_POINT('Ctrl Pts',(1.88692394427232,-18.4699332684472,-319.203753809782)) ;
#38333=CARTESIAN_POINT('Ctrl Pts',(1.82079142166774,-18.4765699063621,-319.204606957925)) ;
#38334=CARTESIAN_POINT('Ctrl Pts',(1.65658055377771,-18.4921588663495,-319.206713994954)) ;
#38335=CARTESIAN_POINT('Ctrl Pts',(1.55846388479071,-18.5006861772765,-319.207963057453)) ;
#38336=CARTESIAN_POINT('Ctrl Pts',(1.11695386597697,-18.5355205690204,-319.213547498424)) ;
#38337=CARTESIAN_POINT('Ctrl Pts',(0.772935634072581,-18.5530504317124,
-319.217801750189)) ;
#38338=CARTESIAN_POINT('Ctrl Pts',(0.0158926184002063,-18.5705328095592,
-319.227103965614)) ;
#38339=CARTESIAN_POINT('Ctrl Pts',(-0.397046604407999,-18.5662946116803,
-319.232140091817)) ;
#38340=CARTESIAN_POINT('Ctrl Pts',(-1.08685987030517,-18.5361891927507,
-319.240638798175)) ;
#38341=CARTESIAN_POINT('Ctrl Pts',(-1.36391251313407,-18.5178647928887,
-319.244074712797)) ;
#38342=CARTESIAN_POINT('Ctrl Pts',(-1.85715757030585,-18.4741115369794,
-319.250263933246)) ;
#38343=CARTESIAN_POINT('Ctrl Pts',(-2.07351069451286,-18.4510808485935,
-319.253003468106)) ;
#38344=CARTESIAN_POINT('Ctrl Pts',(-2.4214855428232,-18.4078412859056,-319.257458108734)) ;
#38345=CARTESIAN_POINT('Ctrl Pts',(-2.5533819388906,-18.3900096153762,-319.25915781626)) ;
#38346=CARTESIAN_POINT('Ctrl Pts',(-2.80983972785376,-18.3525256808239,
-319.262485879989)) ;
#38347=CARTESIAN_POINT('Ctrl Pts',(-2.93441526355954,-18.3330195322253,
-319.264113195574)) ;
#38348=CARTESIAN_POINT('Ctrl Pts',(-3.21077512143554,-18.2868578189954,
-319.267747536089)) ;
#38349=CARTESIAN_POINT('Ctrl Pts',(-3.36244578582736,-18.2595784183176,
-319.269758490247)) ;
#38350=CARTESIAN_POINT('Ctrl Pts',(-4.2263845233712,-18.0930614878937,-319.281305235459)) ;
#38351=CARTESIAN_POINT('Ctrl Pts',(-4.93034124645549,-17.9140427199375,
-319.291100745919)) ;
#38352=CARTESIAN_POINT('Ctrl Pts',(-5.88477134465508,-17.6107916630486,
-319.304578295527)) ;
#38353=CARTESIAN_POINT('Ctrl Pts',(-6.14564708095058,-17.5214593867005,
-319.308279388589)) ;
#38354=CARTESIAN_POINT('Ctrl Pts',(-6.56933416195158,-17.3657482399414,
-319.314275072093)) ;
#38355=CARTESIAN_POINT('Ctrl Pts',(-6.73336358095217,-17.3028083945092,
-319.316592334836)) ;
#38356=CARTESIAN_POINT('Ctrl Pts',(-6.97082076714864,-17.2078054742524,
-319.319929060994)) ;
#38357=CARTESIAN_POINT('Ctrl Pts',(-7.04497323235441,-17.1775802599382,
-319.320968467206)) ;
#38358=CARTESIAN_POINT('Ctrl Pts',(-7.18033805084221,-17.1213803802278,
-319.322859600248)) ;
#38359=CARTESIAN_POINT('Ctrl Pts',(-7.24161067181002,-17.0955548468008,
-319.323713076339)) ;
#38360=CARTESIAN_POINT('Ctrl Pts',(-7.39349896150327,-17.0305729993541,
-319.325823305844)) ;
#38361=CARTESIAN_POINT('Ctrl Pts',(-7.48394361229586,-16.9910220890064,
-319.32707519626)) ;
#38362=CARTESIAN_POINT('Ctrl Pts',(-7.87917907735069,-16.8144198603484,
-319.332533426962)) ;
#38363=CARTESIAN_POINT('Ctrl Pts',(-8.18055378770408,-16.6698745922381,
-319.336663882051)) ;
#38364=CARTESIAN_POINT('Ctrl Pts',(-9.10152525283095,-16.1971652312636,
-319.349385160626)) ;
#38365=CARTESIAN_POINT('Ctrl Pts',(-9.70655597666266,-15.8419915340611,
-319.357904709276)) ;
#38366=CARTESIAN_POINT('Ctrl Pts',(-10.4708478389784,-15.3330696735458,
-319.369382105004)) ;
#38367=CARTESIAN_POINT('Ctrl Pts',(-10.6495176719626,-15.2095185063944,
-319.372117373067)) ;
#38368=CARTESIAN_POINT('Ctrl Pts',(-10.934063956693,-15.0052806052894,-319.376567121194)) ;
#38369=CARTESIAN_POINT('Ctrl Pts',(-11.0413125707712,-14.9265407012279,
-319.378266275821)) ;
#38370=CARTESIAN_POINT('Ctrl Pts',(-11.2485849340564,-14.7709089261429,
-319.381594595799)) ;
#38371=CARTESIAN_POINT('Ctrl Pts',(-11.3486896676676,-14.6941367999769,
-319.383222735165)) ;
#38372=CARTESIAN_POINT('Ctrl Pts',(-11.5694883267313,-14.5212000633758,
-319.386860714791)) ;
#38373=CARTESIAN_POINT('Ctrl Pts',(-11.6897814259169,-14.424538867556,-319.388874508813)) ;
#38374=CARTESIAN_POINT('Ctrl Pts',(-12.3655126594377,-13.867551884254,-319.400367303846)) ;
#38375=CARTESIAN_POINT('Ctrl Pts',(-12.8949527241165,-13.3766619248727,
-319.410102302259)) ;
#38376=CARTESIAN_POINT('Ctrl Pts',(-13.5870107167304,-12.6556288969575,
-319.423553243901)) ;
#38377=CARTESIAN_POINT('Ctrl Pts',(-13.7750096200314,-12.4507394667984,
-319.427286016803)) ;
#38378=CARTESIAN_POINT('Ctrl Pts',(-14.0747847599679,-12.108927434066,-319.433325447807)) ;
#38379=CARTESIAN_POINT('Ctrl Pts',(-14.1893330199395,-11.9744944895627,
-319.435655145479)) ;
#38380=CARTESIAN_POINT('Ctrl Pts',(-14.3531046481112,-11.7766431281461,
-319.439006155434)) ;
#38381=CARTESIAN_POINT('Ctrl Pts',(-14.4038622375929,-11.7145076324911,
-319.440047632248)) ;
#38382=CARTESIAN_POINT('Ctrl Pts',(-14.495929680981,-11.6002991253359,-319.441940505001)) ;
#38383=CARTESIAN_POINT('Ctrl Pts',(-14.5373655918537,-11.5483296954832,
-319.442793676275)) ;
#38384=CARTESIAN_POINT('Ctrl Pts',(-14.6394921063487,-11.4188206820169,
-319.444900496962)) ;
#38385=CARTESIAN_POINT('Ctrl Pts',(-14.6998466333324,-11.3410186446011,
-319.446149323912)) ;
#38386=CARTESIAN_POINT('Ctrl Pts',(-14.9690212521228,-10.988271077602,-319.451744345257)) ;
#38387=CARTESIAN_POINT('Ctrl Pts',(-15.1707668441045,-10.7080125608712,
-319.456008972419)) ;
#38388=CARTESIAN_POINT('Ctrl Pts',(-15.5963413522244,-10.0806290561425,
-319.465321525315)) ;
#38389=CARTESIAN_POINT('Ctrl Pts',(-15.8166412597065,-9.73133111185656,
-319.470357778874)) ;
#38390=CARTESIAN_POINT('Ctrl Pts',(-16.1650907288684,-9.13570935190439,
-319.478851738198)) ;
#38391=CARTESIAN_POINT('Ctrl Pts',(-16.2996918586295,-8.89333394255288,
-319.482282655383)) ;
#38392=CARTESIAN_POINT('Ctrl Pts',(-16.5300533034447,-8.45571254644613,
-319.488464155222)) ;
#38393=CARTESIAN_POINT('Ctrl Pts',(-16.6279062283607,-8.26162642003638,
-319.491201025431)) ;
#38394=CARTESIAN_POINT('Ctrl Pts',(-16.7801361857393,-7.94602001413403,
-319.495652571288)) ;
#38395=CARTESIAN_POINT('Ctrl Pts',(-16.8366533689915,-7.82555478849491,
-319.497351893413)) ;
#38396=CARTESIAN_POINT('Ctrl Pts',(-16.944209056286,-7.58974214479628,-319.500680006021)) ;
#38397=CARTESIAN_POINT('Ctrl Pts',(-16.995376769289,-7.47446150461247,-319.502307764712)) ;
#38398=CARTESIAN_POINT('Ctrl Pts',(-17.1064915475144,-7.21707906813494,
-319.505944161889)) ;
#38399=CARTESIAN_POINT('Ctrl Pts',(-17.1658506236061,-7.07473360724396,
-319.507956744087)) ;
#38400=CARTESIAN_POINT('Ctrl Pts',(-17.4935257941067,-6.26054395960238,
-319.519475047018)) ;
#38401=CARTESIAN_POINT('Ctrl Pts',(-17.724164668576,-5.5742114699139,-319.529238513901)) ;
#38402=CARTESIAN_POINT('Ctrl Pts',(-17.9869089557257,-4.60893865526558,
-319.542702316971)) ;
#38403=CARTESIAN_POINT('Ctrl Pts',(-18.0536624005308,-4.34010178958931,
-319.546420511394)) ;
#38404=CARTESIAN_POINT('Ctrl Pts',(-18.1529976434216,-3.89797587374466,
-319.552439817454)) ;
#38405=CARTESIAN_POINT('Ctrl Pts',(-18.1891699891861,-3.72553816866229,
-319.554763801168)) ;
#38406=CARTESIAN_POINT('Ctrl Pts',(-18.238220777323,-3.47393544510405,-319.558108222011)) ;
#38407=CARTESIAN_POINT('Ctrl Pts',(-18.253049290147,-3.3951607081905,-319.559148722954)) ;
#38408=CARTESIAN_POINT('Ctrl Pts',(-18.2792412556928,-3.25088565586482,
-319.56104074298)) ;
#38409=CARTESIAN_POINT('Ctrl Pts',(-18.290763916458,-3.1854157934459,-319.561894025508)) ;
#38410=CARTESIAN_POINT('Ctrl Pts',(-18.3184991170657,-3.02271499854085,
-319.564002295232)) ;
#38411=CARTESIAN_POINT('Ctrl Pts',(-18.3342894069702,-2.92541413251193,
-319.565252442192)) ;
#38412=CARTESIAN_POINT('Ctrl Pts',(-18.402242510466,-2.48450335993266,-319.570877554075)) ;
#38413=CARTESIAN_POINT('Ctrl Pts',(-18.4455257640374,-2.13959500572097,
-319.575169840832)) ;
#38414=CARTESIAN_POINT('Ctrl Pts',(-18.4865416086821,-1.71703460431869,
-319.580384504812)) ;
#38415=CARTESIAN_POINT('Ctrl Pts',(-18.4935038467758,-1.64034872967172,
-319.581329032511)) ;
#38416=CARTESIAN_POINT('Ctrl Pts',(-18.5399093606199,-1.09130195206812,
-319.58808329453)) ;
#38417=CARTESIAN_POINT('Ctrl Pts',(-18.5617271927112,-0.617626492395772,
-319.593871694817)) ;
#38418=CARTESIAN_POINT('Ctrl Pts',(-18.5677214768945,0.157147599598682,
-319.603473466903)) ;
#38419=CARTESIAN_POINT('Ctrl Pts',(-18.5627385678948,0.457943790936195,
-319.607232968799)) ;
#38420=CARTESIAN_POINT('Ctrl Pts',(-18.5444560085571,0.905084518578797,
-319.61289457403)) ;
#38421=CARTESIAN_POINT('Ctrl Pts',(-18.5367243238609,1.05160729322288,-319.614761341118)) ;
#38422=CARTESIAN_POINT('Ctrl Pts',(-18.519251253741,1.32182588836328,-319.61822732856)) ;
#38423=CARTESIAN_POINT('Ctrl Pts',(-18.5100051050406,1.44554544680253,-319.619823245149)) ;
#38424=CARTESIAN_POINT('Ctrl Pts',(-18.4863505684078,1.72441869773139,-319.623441612675)) ;
#38425=CARTESIAN_POINT('Ctrl Pts',(-18.4712275705704,1.87950235957931,-319.625468570995)) ;
#38426=CARTESIAN_POINT('Ctrl Pts',(-18.4151109568633,2.38854497977584,-319.632170063606)) ;
#38427=CARTESIAN_POINT('Ctrl Pts',(-18.3658801911698,2.74151462355908,-319.636895183147)) ;
#38428=CARTESIAN_POINT('Ctrl Pts',(-18.2108539057103,3.65911306735283,-319.649341253961)) ;
#38429=CARTESIAN_POINT('Ctrl Pts',(-18.0889624278294,4.22063324367381,-319.6571266098)) ;
#38430=CARTESIAN_POINT('Ctrl Pts',(-17.8952280267619,4.94846580360892,-319.667203581026)) ;
#38431=CARTESIAN_POINT('Ctrl Pts',(-17.8467180259244,5.12065970226074,-319.669585584653)) ;
#38432=CARTESIAN_POINT('Ctrl Pts',(-17.7582010069487,5.41831413967188,-319.673685541971)) ;
#38433=CARTESIAN_POINT('Ctrl Pts',(-17.7193336957532,5.54409997983431,-319.675412611917)) ;
#38434=CARTESIAN_POINT('Ctrl Pts',(-17.6570491662795,5.73832236347726,-319.678065147737)) ;
#38435=CARTESIAN_POINT('Ctrl Pts',(-17.6345643852379,5.80705327758613,-319.679001042792)) ;
#38436=CARTESIAN_POINT('Ctrl Pts',(-17.5922010763289,5.9340330736187,-319.680723768735)) ;
#38437=CARTESIAN_POINT('Ctrl Pts',(-17.5724333650502,5.9923178205215,-319.681511989539)) ;
#38438=CARTESIAN_POINT('Ctrl Pts',(-17.5164358181222,6.15476546772547,-319.683703098889)) ;
#38439=CARTESIAN_POINT('Ctrl Pts',(-17.4795671159689,6.25870555518904,-319.685098420167)) ;
#38440=CARTESIAN_POINT('Ctrl Pts',(-17.2196924098855,6.97113158525681,-319.694634221157)) ;
#38441=CARTESIAN_POINT('Ctrl Pts',(-16.9658847798747,7.56790871993275,-319.702497239951)) ;
#38442=CARTESIAN_POINT('Ctrl Pts',(-16.5397577983865,8.44008347033473,-319.714411703903)) ;
#38443=CARTESIAN_POINT('Ctrl Pts',(-16.3905902247648,8.72623336110013,-319.718389290374)) ;
#38444=CARTESIAN_POINT('Ctrl Pts',(-16.1789612946889,9.10761207210454,-319.723826136733)) ;
#38445=CARTESIAN_POINT('Ctrl Pts',(-16.122971185852,9.20636661987439,-319.725246423577)) ;
#38446=CARTESIAN_POINT('Ctrl Pts',(-15.9751615553829,9.4615867085999,-319.728951959854)) ;
#38447=CARTESIAN_POINT('Ctrl Pts',(-15.8819482667882,9.61723083167077,-319.731246377199)) ;
#38448=CARTESIAN_POINT('Ctrl Pts',(-15.71964220456,9.87944685914268,-319.73517565264)) ;
#38449=CARTESIAN_POINT('Ctrl Pts',(-15.6517096131371,9.98672155484111,-319.736801683126)) ;
#38450=CARTESIAN_POINT('Ctrl Pts',(-15.5097453416722,10.2058952744082,-319.740163190908)) ;
#38451=CARTESIAN_POINT('Ctrl Pts',(-15.4355903156368,10.317705678064,-319.741899556146)) ;
#38452=CARTESIAN_POINT('Ctrl Pts',(-15.2346380366665,10.6136843249216,-319.746554134101)) ;
#38453=CARTESIAN_POINT('Ctrl Pts',(-15.105714948132,10.7963821107631,-319.74948845167)) ;
#38454=CARTESIAN_POINT('Ctrl Pts',(-14.8138365795276,11.1945386718311,-319.756015757554)) ;
#38455=CARTESIAN_POINT('Ctrl Pts',(-14.6494151507777,11.4088599620917,-319.759618197178)) ;
#38456=CARTESIAN_POINT('Ctrl Pts',(-14.4114476179268,11.7054178519844,-319.764716238847)) ;
#38457=CARTESIAN_POINT('Ctrl Pts',(-14.3417553689894,11.7907032214126,-319.766195892485)) ;
#38458=CARTESIAN_POINT('Ctrl Pts',(-14.1220604864761,12.054723220087,-319.770815905728)) ;
#38459=CARTESIAN_POINT('Ctrl Pts',(-13.9694445735006,12.2312535160645,-319.773962342769)) ;
#38460=CARTESIAN_POINT('Ctrl Pts',(-13.6278621793669,12.6116256205328,-319.780842973065)) ;
#38461=CARTESIAN_POINT('Ctrl Pts',(-13.4375631121709,12.8141962793856,-319.784573933402)) ;
#38462=CARTESIAN_POINT('Ctrl Pts',(-13.119046828619,13.1383515247736,-319.790610848116)) ;
#38463=CARTESIAN_POINT('Ctrl Pts',(-12.9935146797489,13.2625128439319,-319.792939823999)) ;
#38464=CARTESIAN_POINT('Ctrl Pts',(-12.8083985314719,13.4404561453371,-319.796289954076)) ;
#38465=CARTESIAN_POINT('Ctrl Pts',(-12.7502067083679,13.4956720193375,-319.797331262211)) ;
#38466=CARTESIAN_POINT('Ctrl Pts',(-12.6431490888848,13.5959441769179,-319.79922395058)) ;
#38467=CARTESIAN_POINT('Ctrl Pts',(-12.5943958297316,13.6411183787552,-319.800077104591)) ;
#38468=CARTESIAN_POINT('Ctrl Pts',(-12.4728119687584,13.7525691284561,-319.802183981378)) ;
#38469=CARTESIAN_POINT('Ctrl Pts',(-12.3996946459614,13.8185299062045,-319.803432880374)) ;
#38470=CARTESIAN_POINT('Ctrl Pts',(-12.0681935569585,14.1128347651821,-319.809022528047)) ;
#38471=CARTESIAN_POINT('Ctrl Pts',(-11.8040027467239,14.3345359572437,-319.813281932622)) ;
#38472=CARTESIAN_POINT('Ctrl Pts',(-11.2102648370461,14.8052326426246,-319.822589408397)) ;
#38473=CARTESIAN_POINT('Ctrl Pts',(-10.8782734615348,15.0508510729773,-319.827625722343)) ;
#38474=CARTESIAN_POINT('Ctrl Pts',(-10.3099708235192,15.4426670033821,-319.836122265988)) ;
#38475=CARTESIAN_POINT('Ctrl Pts',(-10.0780707317283,15.5949976771392,-319.839555768992)) ;
#38476=CARTESIAN_POINT('Ctrl Pts',(-9.65846284602696,15.8573605127594,-319.845741302014)) ;
#38477=CARTESIAN_POINT('Ctrl Pts',(-9.47206997903367,15.9693981430799,-319.848479590589)) ;
#38478=CARTESIAN_POINT('Ctrl Pts',(-9.16850189045506,16.144682830759,-319.852932860013)) ;
#38479=CARTESIAN_POINT('Ctrl Pts',(-9.05253932730333,16.2099889662829,-319.85463246526)) ;
#38480=CARTESIAN_POINT('Ctrl Pts',(-8.82533735082764,16.3347428905617,-319.857960766976)) ;
#38481=CARTESIAN_POINT('Ctrl Pts',(-8.7141744196257,16.3943151362728,-319.859588427558)) ;
#38482=CARTESIAN_POINT('Ctrl Pts',(-8.46578558572374,16.5241866402308,-319.863224138451)) ;
#38483=CARTESIAN_POINT('Ctrl Pts',(-8.3282735280697,16.5939184537859,-319.865236126318)) ;
#38484=CARTESIAN_POINT('Ctrl Pts',(-7.53988370801585,16.9814390582658,-319.876765187352)) ;
#38485=CARTESIAN_POINT('Ctrl Pts',(-6.87171979668173,17.2626352898733,-319.886540733513)) ;
#38486=CARTESIAN_POINT('Ctrl Pts',(-5.92820194030155,17.5962310982935,-319.900009171244)) ;
#38487=CARTESIAN_POINT('Ctrl Pts',(-5.66553199569972,17.6825528310066,-319.903720390948)) ;
#38488=CARTESIAN_POINT('Ctrl Pts',(-5.23266435444511,17.8141710959272,-319.909730082764)) ;
#38489=CARTESIAN_POINT('Ctrl Pts',(-5.06357656710662,17.8629689754263,-319.912051342808)) ;
#38490=CARTESIAN_POINT('Ctrl Pts',(-4.81652668189091,17.930476584419,-319.915392692316)) ;
#38491=CARTESIAN_POINT('Ctrl Pts',(-4.73909691644011,17.9510969097205,-319.916432794473)) ;
#38492=CARTESIAN_POINT('Ctrl Pts',(-4.59718118539811,17.9879082928282,-319.918324525295)) ;
#38493=CARTESIAN_POINT('Ctrl Pts',(-4.53273727125493,18.0042553977027,-319.919177911769)) ;
#38494=CARTESIAN_POINT('Ctrl Pts',(-4.3724706414082,18.0439942590534,-319.921287079592)) ;
#38495=CARTESIAN_POINT('Ctrl Pts',(-4.27654666169823,18.066969226243,-319.922538010712)) ;
#38496=CARTESIAN_POINT('Ctrl Pts',(-3.84094213516165,18.1676382720442,-319.928175252157)) ;
#38497=CARTESIAN_POINT('Ctrl Pts',(-3.49929775127554,18.2365247036286,-319.932478455298)) ;
#38498=CARTESIAN_POINT('Ctrl Pts',(-2.7490992488878,18.3659298118304,-319.941828824024)) ;
#38499=CARTESIAN_POINT('Ctrl Pts',(-2.34005409434378,18.422515342876,-319.946864964147)) ;
#38500=CARTESIAN_POINT('Ctrl Pts',(-1.65551987148274,18.4940427655919,-319.955337967357)) ;
#38501=CARTESIAN_POINT('Ctrl Pts',(-1.38097356447629,18.5165675961726,-319.958747518266)) ;
#38502=CARTESIAN_POINT('Ctrl Pts',(-0.890008694264454,18.5458678578923,
-319.964895875783)) ;
#38503=CARTESIAN_POINT('Ctrl Pts',(-0.673780509989867,18.5549818018221,
-319.967621213158)) ;
#38504=CARTESIAN_POINT('Ctrl Pts',(-0.324584938680104,18.5635881755225,
-319.972059069452)) ;
#38505=CARTESIAN_POINT('Ctrl Pts',(-0.191695890545446,18.5654360023381,
-319.973756420582)) ;
#38506=CARTESIAN_POINT('Ctrl Pts',(0.0674249714563399,18.5662566454235,
-319.97708392605)) ;
#38507=CARTESIAN_POINT('Ctrl Pts',(0.193649211159391,18.5653691554949,-319.978713084605)) ;
#38508=CARTESIAN_POINT('Ctrl Pts',(0.504550860100535,18.5600121422162,-319.982746700352)) ;
#38509=CARTESIAN_POINT('Ctrl Pts',(0.6891892195366,18.5540734165393,-319.985160385014)) ;
#38510=CARTESIAN_POINT('Ctrl Pts',(1.51233830771507,18.5152933067266,-319.995999431483)) ;
#38511=CARTESIAN_POINT('Ctrl Pts',(2.14898649596295,18.4522384785831,-320.004609907316)) ;
#38512=CARTESIAN_POINT('Ctrl Pts',(3.0887807274062,18.3098544208974,-320.017411465897)) ;
#38513=CARTESIAN_POINT('Ctrl Pts',(3.39523397472678,18.2555120960985,-320.021597204388)) ;
#38514=CARTESIAN_POINT('Ctrl Pts',(3.88557008711895,18.1557879752052,-320.02825325447)) ;
#38515=CARTESIAN_POINT('Ctrl Pts',(4.0703769357173,18.1152511361994,-320.030752150826)) ;
#38516=CARTESIAN_POINT('Ctrl Pts',(4.33449654003708,18.0530714243576,-320.034294725367)) ;
#38517=CARTESIAN_POINT('Ctrl Pts',(4.41433521615896,18.0337154445048,-320.035361770274)) ;
#38518=CARTESIAN_POINT('Ctrl Pts',(4.55819934105968,17.9978246019581,-320.037275961302)) ;
#38519=CARTESIAN_POINT('Ctrl Pts',(4.62226971507521,17.9814764219975,-320.038125215467)) ;
#38520=CARTESIAN_POINT('Ctrl Pts',(4.77845717552494,17.9407337317494,-320.040188223477)) ;
#38521=CARTESIAN_POINT('Ctrl Pts',(4.87047639526634,17.9159716323842,-320.041397667061)) ;
#38522=CARTESIAN_POINT('Ctrl Pts',(5.24497135151118,17.8120977070797,-320.046302164943)) ;
#38523=CARTESIAN_POINT('Ctrl Pts',(5.52574451263457,17.7270047529477,-320.04993879566)) ;
#38524=CARTESIAN_POINT('Ctrl Pts',(6.34754608396632,17.4565215134081,-320.06059257353)) ;
#38525=CARTESIAN_POINT('Ctrl Pts',(6.88215907115174,17.2527497020884,-320.067543972492)) ;
#38526=CARTESIAN_POINT('Ctrl Pts',(7.55162703804269,16.9614996919909,-320.07657173726)) ;
#38527=CARTESIAN_POINT('Ctrl Pts',(7.69592687685017,16.896515976897,-320.078536593918)) ;
#38528=CARTESIAN_POINT('Ctrl Pts',(8.04578298633694,16.7335507974973,-320.08335451286)) ;
#38529=CARTESIAN_POINT('Ctrl Pts',(8.25040130628812,16.6336172905842,-320.086218698649)) ;
#38530=CARTESIAN_POINT('Ctrl Pts',(8.57322127727884,16.4685327198421,-320.090821880119)) ;
#38531=CARTESIAN_POINT('Ctrl Pts',(8.69264023068258,16.4058129566795,-320.092543424442)) ;
#38532=CARTESIAN_POINT('Ctrl Pts',(8.92281739151623,16.2817032939308,-320.095899534717)) ;
#38533=CARTESIAN_POINT('Ctrl Pts',(9.03365198864775,16.2204705248554,-320.097532877132)) ;
#38534=CARTESIAN_POINT('Ctrl Pts',(9.27494514780877,16.0839230599919,-320.101127396337)) ;
#38535=CARTESIAN_POINT('Ctrl Pts',(9.40513105028525,16.0081447498608,-320.103091896737)) ;
#38536=CARTESIAN_POINT('Ctrl Pts',(9.93666896574076,15.6900259134925,-320.111215926243)) ;
#38537=CARTESIAN_POINT('Ctrl Pts',(10.3296923532581,15.4341101756063,-320.117472350451)) ;
#38538=CARTESIAN_POINT('Ctrl Pts',(11.0899376495795,14.8970206119009,-320.129984184648)) ;
#38539=CARTESIAN_POINT('Ctrl Pts',(11.4571878805374,14.6164559976904,-320.136233512233)) ;
#38540=CARTESIAN_POINT('Ctrl Pts',(11.9393609646369,14.2187460603731,-320.144581680247)) ;
#38541=CARTESIAN_POINT('Ctrl Pts',(12.0637605490455,14.1133540062695,-320.14674857129)) ;
#38542=CARTESIAN_POINT('Ctrl Pts',(12.2797603217164,13.9254150399708,-320.150523340422)) ;
#38543=CARTESIAN_POINT('Ctrl Pts',(12.3719565054994,13.8435685390282,-320.152138580305)) ;
#38544=CARTESIAN_POINT('Ctrl Pts',(12.5157162349746,13.7133636247249,-320.154658909564)) ;
#38545=CARTESIAN_POINT('Ctrl Pts',(12.5678304142424,13.6656186643628,-320.155572908172)) ;
#38546=CARTESIAN_POINT('Ctrl Pts',(12.6655711162328,13.5750404759047,-320.157286674107)) ;
#38547=CARTESIAN_POINT('Ctrl Pts',(12.7112561675805,13.5322718815756,-320.158087537528)) ;
#38548=CARTESIAN_POINT('Ctrl Pts',(12.8413884142572,13.4092066014094,-320.160369687735)) ;
#38549=CARTESIAN_POINT('Ctrl Pts',(12.9252971235976,13.3283446990111,-320.161842338388)) ;
#38550=CARTESIAN_POINT('Ctrl Pts',(13.3366125049587,12.9244273584927,-320.169081810957)) ;
#38551=CARTESIAN_POINT('Ctrl Pts',(13.6526976119873,12.5900717163233,-320.174714636213)) ;
#38552=CARTESIAN_POINT('Ctrl Pts',(14.2379479098119,11.9230053296396,-320.185584059432)) ;
#38553=CARTESIAN_POINT('Ctrl Pts',(14.5086749540123,11.5920475947371,-320.19081706137)) ;
#38554=CARTESIAN_POINT('Ctrl Pts',(14.9401752058827,11.025725300284,-320.199652727215)) ;
#38555=CARTESIAN_POINT('Ctrl Pts',(15.1073879545976,10.7954750838082,-320.203213441597)) ;
#38556=CARTESIAN_POINT('Ctrl Pts',(15.3513268032109,10.4428006697178,-320.208641948314)) ;
#38557=CARTESIAN_POINT('Ctrl Pts',(15.4320244489777,10.3231749852063,-320.210478866598)) ;
#38558=CARTESIAN_POINT('Ctrl Pts',(15.5796050754802,10.0988041840275,-320.213917929155)) ;
#38559=CARTESIAN_POINT('Ctrl Pts',(15.6468467997275,9.99430464964471,-320.21551716458)) ;
#38560=CARTESIAN_POINT('Ctrl Pts',(15.7977885547452,9.75447050384159,-320.219182564621)) ;
#38561=CARTESIAN_POINT('Ctrl Pts',(15.8808079355028,9.61871910602072,-320.221253743268)) ;
#38562=CARTESIAN_POINT('Ctrl Pts',(16.1524546149686,9.16142301085318,-320.228218656002)) ;
#38563=CARTESIAN_POINT('Ctrl Pts',(16.3331410593165,8.83526816939149,-320.233168185275)) ;
#38564=CARTESIAN_POINT('Ctrl Pts',(16.6949491006004,8.13309138027728,-320.243744190874)) ;
#38565=CARTESIAN_POINT('Ctrl Pts',(16.8734613046573,7.7559528023655,-320.249378676435)) ;
#38566=CARTESIAN_POINT('Ctrl Pts',(17.1751764750888,7.05869596066065,-320.259595551739)) ;
#38567=CARTESIAN_POINT('Ctrl Pts',(17.3025054370407,6.74056243641117,-320.264183310802)) ;
#38568=CARTESIAN_POINT('Ctrl Pts',(17.4602303554772,6.31250797324157,-320.27018670905)) ;
#38569=CARTESIAN_POINT('Ctrl Pts',(17.4985230086725,6.20556955915865,-320.27167252722)) ;
#38570=CARTESIAN_POINT('Ctrl Pts',(17.5562243478787,6.03964737653708,-320.273952692707)) ;
#38571=CARTESIAN_POINT('Ctrl Pts',(17.5763224982979,5.98090638916209,-320.274755081634)) ;
#38572=CARTESIAN_POINT('Ctrl Pts',(17.6188997919324,5.85439725314229,-320.276471882379)) ;
#38573=CARTESIAN_POINT('Ctrl Pts',(17.6412834232062,5.78659798806358,-320.277385040377)) ;
#38574=CARTESIAN_POINT('Ctrl Pts',(17.7023779429912,5.59789517860218,-320.279909439235)) ;
#38575=CARTESIAN_POINT('Ctrl Pts',(17.7402407436729,5.47672107230045,-320.281510992794)) ;
#38576=CARTESIAN_POINT('Ctrl Pts',(17.8258630370353,5.19249183469465,-320.285231355031)) ;
#38577=CARTESIAN_POINT('Ctrl Pts',(17.8726330161994,5.02915039226601,-320.287341708953)) ;
#38578=CARTESIAN_POINT('Ctrl Pts',(18.0499734966762,4.37605424666018,-320.295703943975)) ;
#38579=CARTESIAN_POINT('Ctrl Pts',(18.1627068807465,3.88168443521965,-320.301871192323)) ;
#38580=CARTESIAN_POINT('Ctrl Pts',(18.3226297249567,3.01880393951633,-320.312662409177)) ;
#38581=CARTESIAN_POINT('Ctrl Pts',(18.3792547700535,2.65234435559654,-320.317252058086)) ;
#38582=CARTESIAN_POINT('Ctrl Pts',(18.4475384453953,2.10160987598044,-320.324221304029)) ;
#38583=CARTESIAN_POINT('Ctrl Pts',(18.4674839589907,1.91845636824946,-320.326550414766)) ;
#38584=CARTESIAN_POINT('Ctrl Pts',(18.4964891004421,1.60944193958221,-320.330503948382)) ;
#38585=CARTESIAN_POINT('Ctrl Pts',(18.506997491946,1.48373049431182,-320.332118908144)) ;
#38586=CARTESIAN_POINT('Ctrl Pts',(18.5259538031235,1.22524779539483,-320.335454077873)) ;
#38587=CARTESIAN_POINT('Ctrl Pts',(18.5342574400419,1.09247313882107,-320.337175128993)) ;
#38588=CARTESIAN_POINT('Ctrl Pts',(18.5523575088749,0.742756068931193,-320.341729375101)) ;
#38589=CARTESIAN_POINT('Ctrl Pts',(18.5597759406601,0.525711411823962,-320.344577418692)) ;
#38590=CARTESIAN_POINT('Ctrl Pts',(18.5679868762546,0.031773627231106,-320.351103987191)) ;
#38591=CARTESIAN_POINT('Ctrl Pts',(18.5663962055185,-0.245107563597892,
-320.354795004192)) ;
#38592=CARTESIAN_POINT('Ctrl Pts',(18.5551718341297,-0.644282005015534,
-320.360148157064)) ;
#38593=CARTESIAN_POINT('Ctrl Pts',(18.5505180401484,-0.766664977760487,
-320.361793608738)) ;
#38594=CARTESIAN_POINT('Ctrl Pts',(18.5446545929199,-0.888979995160607,
-320.363441000746)) ;
#38595=CARTESIAN_POINT('',(18.544654593745,-0.888979977948782,-315.477129595899)) ;
#38596=CARTESIAN_POINT('Origin',(0.,0.,-315.477129595899)) ;
#38597=CARTESIAN_POINT('',(18.544654593745,-0.888979977947869,-322.15838043089)) ;
#38598=CARTESIAN_POINT('',(18.5446545934554,-0.888979983988388,-321.863010318849)) ;
#38599=CARTESIAN_POINT('',(18.544654593745,-0.888979977948782,-315.477129595899)) ;
#38600=CARTESIAN_POINT('Ctrl Pts',(18.5446545937451,-0.888979977946956,
-322.15838043089)) ;
#38601=CARTESIAN_POINT('Ctrl Pts',(18.5487996595587,-0.802511423324546,
-322.157272162262)) ;
#38602=CARTESIAN_POINT('Ctrl Pts',(18.5523399110549,-0.716014844920947,
-322.156171030603)) ;
#38603=CARTESIAN_POINT('Ctrl Pts',(18.5628298984463,-0.406808063188213,
-322.152256951415)) ;
#38604=CARTESIAN_POINT('Ctrl Pts',(18.5663752672,-0.184001171814233,-322.149477575187)) ;
#38605=CARTESIAN_POINT('Ctrl Pts',(18.5650377213936,0.455758810308087,-322.141557399885)) ;
#38606=CARTESIAN_POINT('Ctrl Pts',(18.5501210484485,0.872554674511302,-322.136469030416)) ;
#38607=CARTESIAN_POINT('Ctrl Pts',(18.486526737587,1.78667737075809,-322.125236540751)) ;
#38608=CARTESIAN_POINT('Ctrl Pts',(18.4317827840163,2.28325839234699,-322.119084876013)) ;
#38609=CARTESIAN_POINT('Ctrl Pts',(18.3302147114612,2.95465787815983,-322.110550934314)) ;
#38610=CARTESIAN_POINT('Ctrl Pts',(18.300766083257,3.13189003138177,-322.108278207396)) ;
#38611=CARTESIAN_POINT('Ctrl Pts',(18.2461695268471,3.43334404513227,-322.10437405166)) ;
#38612=CARTESIAN_POINT('Ctrl Pts',(18.222313407616,3.55778691822792,-322.102751157992)) ;
#38613=CARTESIAN_POINT('Ctrl Pts',(18.170471084917,3.81400380454635,-322.099385583639)) ;
#38614=CARTESIAN_POINT('Ctrl Pts',(18.142320773578,3.94573711141024,-322.097641903981)) ;
#38615=CARTESIAN_POINT('Ctrl Pts',(18.0629616468464,4.29828984594866,-322.092939271591)) ;
#38616=CARTESIAN_POINT('Ctrl Pts',(18.0091383609485,4.51849690259196,-322.089963598779)) ;
#38617=CARTESIAN_POINT('Ctrl Pts',(17.9111874601896,4.88963890781372,-322.084886636578)) ;
#38618=CARTESIAN_POINT('Ctrl Pts',(17.8691499990125,5.04109939555204,-322.082797235378)) ;
#38619=CARTESIAN_POINT('Ctrl Pts',(17.6675659559886,5.7331774868269,-322.073177068932)) ;
#38620=CARTESIAN_POINT('Ctrl Pts',(17.4853745621891,6.26688800631222,-322.06554326626)) ;
#38621=CARTESIAN_POINT('Ctrl Pts',(17.1680672917803,7.07419541659538,-322.053907116497)) ;
#38622=CARTESIAN_POINT('Ctrl Pts',(17.0500254521064,7.35414223921198,-322.049857225287)) ;
#38623=CARTESIAN_POINT('Ctrl Pts',(16.8858803849559,7.71820442275282,-322.044622873257)) ;
#38624=CARTESIAN_POINT('Ctrl Pts',(16.8459202056976,7.80503737003947,-322.043376959761)) ;
#38625=CARTESIAN_POINT('Ctrl Pts',(16.7771734814474,7.95143542370017,-322.041283108319)) ;
#38626=CARTESIAN_POINT('Ctrl Pts',(16.74873594041,8.01116219744681,-322.040430869139)) ;
#38627=CARTESIAN_POINT('Ctrl Pts',(16.6843517497622,8.14454561722796,-322.038532532803)) ;
#38628=CARTESIAN_POINT('Ctrl Pts',(16.6482354216506,8.21811864062088,-322.037488552967)) ;
#38629=CARTESIAN_POINT('Ctrl Pts',(16.5277194054222,8.45956830293604,-322.034069196931)) ;
#38630=CARTESIAN_POINT('Ctrl Pts',(16.4412582536297,8.62640318326902,-322.031717231844)) ;
#38631=CARTESIAN_POINT('Ctrl Pts',(16.2065944922168,9.06286045647185,-322.025560620256)) ;
#38632=CARTESIAN_POINT('Ctrl Pts',(16.0541968237118,9.33016128040263,-322.021785838148)) ;
#38633=CARTESIAN_POINT('Ctrl Pts',(15.5540396636236,10.1588545606611,-322.009926437806)) ;
#38634=CARTESIAN_POINT('Ctrl Pts',(15.1829375846837,10.7055537539624,-322.001853855825)) ;
#38635=CARTESIAN_POINT('Ctrl Pts',(14.6759626629927,11.3728721957208,-321.991318106432)) ;
#38636=CARTESIAN_POINT('Ctrl Pts',(14.5663939243873,11.5128740967222,-321.98906857793)) ;
#38637=CARTESIAN_POINT('Ctrl Pts',(14.3754907319645,11.7497127398196,-321.985191198123)) ;
#38638=CARTESIAN_POINT('Ctrl Pts',(14.2951465345319,11.8473317146042,-321.983571571629)) ;
#38639=CARTESIAN_POINT('Ctrl Pts',(14.1267570630213,12.0477194999068,-321.980201097481)) ;
#38640=CARTESIAN_POINT('Ctrl Pts',(14.0385726028535,12.1503617013837,-321.978449127807)) ;
#38641=CARTESIAN_POINT('Ctrl Pts',(13.7973744066635,12.4249724861135,-321.973691839733)) ;
#38642=CARTESIAN_POINT('Ctrl Pts',(13.6422720040161,12.5950742777077,-321.970669090305)) ;
#38643=CARTESIAN_POINT('Ctrl Pts',(13.3734778831224,12.8790706909869,-321.965495095661)) ;
#38644=CARTESIAN_POINT('Ctrl Pts',(13.2613951364485,12.994451566119,-321.963355867377)) ;
#38645=CARTESIAN_POINT('Ctrl Pts',(12.7295298781362,13.5279181403464,-321.95329754996)) ;
#38646=CARTESIAN_POINT('Ctrl Pts',(12.291390773185,13.9272111606732,-321.945265532659)) ;
#38647=CARTESIAN_POINT('Ctrl Pts',(11.6774504042566,14.435145217785,-321.934595144184)) ;
#38648=CARTESIAN_POINT('Ctrl Pts',(11.5178470092958,14.5628110569883,-321.931872181912)) ;
#38649=CARTESIAN_POINT('Ctrl Pts',(11.255735027087,14.7654679945165,-321.927501288321)) ;
#38650=CARTESIAN_POINT('Ctrl Pts',(11.1545077010781,14.8420879300768,-321.925837013899)) ;
#38651=CARTESIAN_POINT('Ctrl Pts',(10.99513389696,14.96016803904,-321.923258658101)) ;
#38652=CARTESIAN_POINT('Ctrl Pts',(10.937520623894,15.0023411435658,-321.922335011599)) ;
#38653=CARTESIAN_POINT('Ctrl Pts',(10.8222354750771,15.085713170374,-321.92050471892)) ;
#38654=CARTESIAN_POINT('Ctrl Pts',(10.7645680905551,15.1269162876888,-321.919598026613)) ;
#38655=CARTESIAN_POINT('Ctrl Pts',(10.6051312803491,15.2394598356136,-321.917113536746)) ;
#38656=CARTESIAN_POINT('Ctrl Pts',(10.5028791639552,15.3101102183431,-321.9155449411)) ;
#38657=CARTESIAN_POINT('Ctrl Pts',(10.2633278797534,15.4720971762055,-321.91191888245)) ;
#38658=CARTESIAN_POINT('Ctrl Pts',(10.1255057892276,15.5626418975683,-321.909869302491)) ;
#38659=CARTESIAN_POINT('Ctrl Pts',(9.5871780159321,15.9061274048885,-321.901973837252)) ;
#38660=CARTESIAN_POINT('Ctrl Pts',(9.17825545263083,16.145541158633,-321.896204557637)) ;
#38661=CARTESIAN_POINT('Ctrl Pts',(8.36041795762826,16.5832431621111,-321.884813995728)) ;
#38662=CARTESIAN_POINT('Ctrl Pts',(7.95249087693705,16.7826824359189,-321.879200507621)) ;
#38663=CARTESIAN_POINT('Ctrl Pts',(7.40014379729122,17.0280655458937,-321.87158754533)) ;
#38664=CARTESIAN_POINT('Ctrl Pts',(7.26188372340456,17.0874863323628,-321.869681380037)) ;
#38665=CARTESIAN_POINT('Ctrl Pts',(7.00601269810024,17.1937869827731,-321.866150142373)) ;
#38666=CARTESIAN_POINT('Ctrl Pts',(6.88861512619969,17.2411573371497,-321.864528593878)) ;
#38667=CARTESIAN_POINT('Ctrl Pts',(6.64508671565606,17.3365375243023,-321.861161092913)) ;
#38668=CARTESIAN_POINT('Ctrl Pts',(6.51889832372935,17.3843802124067,-321.85941409182)) ;
#38669=CARTESIAN_POINT('Ctrl Pts',(6.17806942596655,17.5093682230922,-321.854689585883)) ;
#38670=CARTESIAN_POINT('Ctrl Pts',(5.9625107369892,17.5839410490731,-321.851695077855)) ;
#38671=CARTESIAN_POINT('Ctrl Pts',(5.59477809289496,17.7036189846872,-321.846579369567)) ;
#38672=CARTESIAN_POINT('Ctrl Pts',(5.44329996735557,17.7507789250897,-321.844470110137)) ;
#38673=CARTESIAN_POINT('Ctrl Pts',(4.74021165383412,17.9598263561176,-321.834678947671)) ;
#38674=CARTESIAN_POINT('Ctrl Pts',(4.18187522988316,18.0979801827844,-321.826890213764)) ;
#38675=CARTESIAN_POINT('Ctrl Pts',(3.33293282120812,18.2666512822746,-321.815286893583)) ;
#38676=CARTESIAN_POINT('Ctrl Pts',(3.04654090590706,18.3165930067094,-321.811414947406)) ;
#38677=CARTESIAN_POINT('Ctrl Pts',(2.67457516022838,18.3724917187028,-321.806486035236)) ;
#38678=CARTESIAN_POINT('Ctrl Pts',(2.58996908361435,18.3846094441639,-321.805371628944)) ;
#38679=CARTESIAN_POINT('Ctrl Pts',(2.43886581087167,18.4051874730474,-321.803395114084)) ;
#38680=CARTESIAN_POINT('Ctrl Pts',(2.37240076842532,18.4138726778305,-321.80253050881)) ;
#38681=CARTESIAN_POINT('Ctrl Pts',(2.22842778455192,18.431893646759,-321.800668773673)) ;
#38682=CARTESIAN_POINT('Ctrl Pts',(2.15090518075313,18.4411008543941,-321.799673070621)) ;
#38683=CARTESIAN_POINT('Ctrl Pts',(1.91097405005321,18.4680634840008,-321.79660933925)) ;
#38684=CARTESIAN_POINT('Ctrl Pts',(1.74838733653556,18.4841643724296,-321.794558591313)) ;
#38685=CARTESIAN_POINT('Ctrl Pts',(1.08290493219999,18.5412077444992,-321.786235060189)) ;
#38686=CARTESIAN_POINT('Ctrl Pts',(0.578652091199881,18.5637881830208,-321.780086470651)) ;
#38687=CARTESIAN_POINT('Ctrl Pts',(-0.407649254588204,18.5677250509697,
-321.767995191749)) ;
#38688=CARTESIAN_POINT('Ctrl Pts',(-0.889296348461817,18.5508959957287,
-321.762060415628)) ;
#38689=CARTESIAN_POINT('Ctrl Pts',(-1.55467839403078,18.5016719062076,-321.75368313893)) ;
#38690=CARTESIAN_POINT('Ctrl Pts',(-1.73939966838831,18.4852204983317,-321.751339040825)) ;
#38691=CARTESIAN_POINT('Ctrl Pts',(-2.04949957614768,18.452913368602,-321.747368062005)) ;
#38692=CARTESIAN_POINT('Ctrl Pts',(-2.17501891170769,18.4385398820578,-321.745750850888)) ;
#38693=CARTESIAN_POINT('Ctrl Pts',(-2.43206945327457,18.4064431554954,-321.742417694058)) ;
#38694=CARTESIAN_POINT('Ctrl Pts',(-2.56357703946243,18.388588422237,-321.740700976515)) ;
#38695=CARTESIAN_POINT('Ctrl Pts',(-2.90793927422231,18.3380685751711,-321.736175075831)) ;
#38696=CARTESIAN_POINT('Ctrl Pts',(-3.12043652426833,18.3031075376664,-321.733351392112)) ;
#38697=CARTESIAN_POINT('Ctrl Pts',(-3.60126935198572,18.2153815158039,-321.726895439337)) ;
#38698=CARTESIAN_POINT('Ctrl Pts',(-3.86914412389228,18.1603686099956,-321.723251107187)) ;
#38699=CARTESIAN_POINT('Ctrl Pts',(-4.47741226710087,18.0213800440598,-321.714889101795)) ;
#38700=CARTESIAN_POINT('Ctrl Pts',(-4.81683915442632,17.9336393276997,-321.71015954964)) ;
#38701=CARTESIAN_POINT('Ctrl Pts',(-5.24416761433995,17.8101683607781,-321.704172438769)) ;
#38702=CARTESIAN_POINT('Ctrl Pts',(-5.33455658544967,17.7833038845697,-321.702904262159)) ;
#38703=CARTESIAN_POINT('Ctrl Pts',(-5.73291839956111,17.6615963912092,-321.697311579922)) ;
#38704=CARTESIAN_POINT('Ctrl Pts',(-6.03859688022656,17.55943304675,-321.69300967336)) ;
#38705=CARTESIAN_POINT('Ctrl Pts',(-6.4333764213085,17.4159619712753,-321.687501142742)) ;
#38706=CARTESIAN_POINT('Ctrl Pts',(-6.52502605383703,17.3818324293006,-321.686225775439)) ;
#38707=CARTESIAN_POINT('Ctrl Pts',(-6.67842860185837,17.3233223670344,-321.684099459676)) ;
#38708=CARTESIAN_POINT('Ctrl Pts',(-6.74032805700307,17.2993318986975,-321.683243855703)) ;
#38709=CARTESIAN_POINT('Ctrl Pts',(-6.87709669785578,17.2454787507199,-321.681359202854)) ;
#38710=CARTESIAN_POINT('Ctrl Pts',(-6.95190262372793,17.2154595136883,-321.680332035678)) ;
#38711=CARTESIAN_POINT('Ctrl Pts',(-7.1922032880742,17.1172064025887,-321.677040892551)) ;
#38712=CARTESIAN_POINT('Ctrl Pts',(-7.35690764339327,17.0470658264597,-321.674798010701)) ;
#38713=CARTESIAN_POINT('Ctrl Pts',(-7.78035955291097,16.859455563299,-321.669037818533)) ;
#38714=CARTESIAN_POINT('Ctrl Pts',(-8.03747085924693,16.7384079070025,-321.665546055258)) ;
#38715=CARTESIAN_POINT('Ctrl Pts',(-8.92505589653861,16.2953661495479,-321.653384775717)) ;
#38716=CARTESIAN_POINT('Ctrl Pts',(-9.53981093312355,15.943261511577,-321.644746594839)) ;
#38717=CARTESIAN_POINT('Ctrl Pts',(-10.263522168483,15.4718742367918,-321.633879358036)) ;
#38718=CARTESIAN_POINT('Ctrl Pts',(-10.3930132002504,15.3851895090078,-321.631907415922)) ;
#38719=CARTESIAN_POINT('Ctrl Pts',(-10.6256039078403,15.2252105798601,-321.628312224208)) ;
#38720=CARTESIAN_POINT('Ctrl Pts',(-10.7290750709102,15.1524731868025,-321.626693353294)) ;
#38721=CARTESIAN_POINT('Ctrl Pts',(-10.9393947051829,15.0013897709901,-321.623361547521)) ;
#38722=CARTESIAN_POINT('Ctrl Pts',(-11.0461640351006,14.9229458092083,-321.621647890495)) ;
#38723=CARTESIAN_POINT('Ctrl Pts',(-11.3232203741165,14.7147884591784,-321.617142003634)) ;
#38724=CARTESIAN_POINT('Ctrl Pts',(-11.4921195280334,14.5832612108531,-321.614335517162)) ;
#38725=CARTESIAN_POINT('Ctrl Pts',(-11.7710476516844,14.3581953660808,-321.609602225746)) ;
#38726=CARTESIAN_POINT('Ctrl Pts',(-11.8823278815949,14.2662406063667,-321.607686773499)) ;
#38727=CARTESIAN_POINT('Ctrl Pts',(-12.3569680743402,13.864622385992,-321.599404245368)) ;
#38728=CARTESIAN_POINT('Ctrl Pts',(-12.70938147799,13.542305376322,-321.592960822087)) ;
#38729=CARTESIAN_POINT('Ctrl Pts',(-13.1888076029562,13.0686071696249,-321.583888466479)) ;
#38730=CARTESIAN_POINT('Ctrl Pts',(-13.326433789351,12.9282366117419,-321.581246674254)) ;
#38731=CARTESIAN_POINT('Ctrl Pts',(-13.6277804579957,12.6109549736229,-321.575398008909)) ;
#38732=CARTESIAN_POINT('Ctrl Pts',(-13.7903377390698,12.4329872113515,-321.572198863869)) ;
#38733=CARTESIAN_POINT('Ctrl Pts',(-14.0033019680442,12.1905171745171,-321.567974764716)) ;
#38734=CARTESIAN_POINT('Ctrl Pts',(-14.0568138828617,12.1287739890283,-321.566910509794)) ;
#38735=CARTESIAN_POINT('Ctrl Pts',(-14.1530416783587,12.0162520514127,-321.564993115923)) ;
#38736=CARTESIAN_POINT('Ctrl Pts',(-14.1958961934523,11.9655937341931,-321.564137973355)) ;
#38737=CARTESIAN_POINT('Ctrl Pts',(-14.290312509757,11.8527630346874,-321.562251688621)) ;
#38738=CARTESIAN_POINT('Ctrl Pts',(-14.3417419203426,11.7904818348291,-321.561222457326)) ;
#38739=CARTESIAN_POINT('Ctrl Pts',(-14.5065158545704,11.5882666969086,-321.55791584383)) ;
#38740=CARTESIAN_POINT('Ctrl Pts',(-14.6182315254804,11.4470185877134,-321.555659828862)) ;
#38741=CARTESIAN_POINT('Ctrl Pts',(-14.9025557995998,11.0765806667062,-321.549852844566)) ;
#38742=CARTESIAN_POINT('Ctrl Pts',(-15.0719382923908,10.8449751108958,-321.546327916026)) ;
#38743=CARTESIAN_POINT('Ctrl Pts',(-15.6361128171834,10.0347891237646,-321.534225822185)) ;
#38744=CARTESIAN_POINT('Ctrl Pts',(-16.0034974686149,9.43785383690433,-321.525677257406)) ;
#38745=CARTESIAN_POINT('Ctrl Pts',(-16.4190670036199,8.66828111787151,-321.5146752888)) ;
#38746=CARTESIAN_POINT('Ctrl Pts',(-16.499694292565,8.51380919030238,-321.512469312529)) ;
#38747=CARTESIAN_POINT('Ctrl Pts',(-16.6348258776578,8.24578223896283,-321.508641902744)) ;
#38748=CARTESIAN_POINT('Ctrl Pts',(-16.6903710473401,8.13276527151816,-321.507028117773)) ;
#38749=CARTESIAN_POINT('Ctrl Pts',(-16.8037554534973,7.89600888900553,-321.503646694235)) ;
#38750=CARTESIAN_POINT('Ctrl Pts',(-16.8613876501391,7.77217859805641,-321.501877689096)) ;
#38751=CARTESIAN_POINT('Ctrl Pts',(-17.0154569842627,7.43135943921193,-321.497007335688)) ;
#38752=CARTESIAN_POINT('Ctrl Pts',(-17.1091058977917,7.21313902140694,-321.49388704746)) ;
#38753=CARTESIAN_POINT('Ctrl Pts',(-17.4434474832382,6.39088278290552,-321.482132718024)) ;
#38754=CARTESIAN_POINT('Ctrl Pts',(-17.6565429536326,5.77613442327295,-321.473334193799)) ;
#38755=CARTESIAN_POINT('Ctrl Pts',(-17.9337361569647,4.81635581475174,-321.459908429103)) ;
#38756=CARTESIAN_POINT('Ctrl Pts',(-18.0210597868333,4.47856906930221,-321.45524464081)) ;
#38757=CARTESIAN_POINT('Ctrl Pts',(-18.1208090108261,4.04234028817951,-321.449374925292)) ;
#38758=CARTESIAN_POINT('Ctrl Pts',(-18.1420353476001,3.94598374300328,-321.448087988367)) ;
#38759=CARTESIAN_POINT('Ctrl Pts',(-18.1762782288956,3.78441934811357,-321.445948790714)) ;
#38760=CARTESIAN_POINT('Ctrl Pts',(-18.1897143551459,3.71930259201257,-321.44509173517)) ;
#38761=CARTESIAN_POINT('Ctrl Pts',(-18.2185677140576,3.57557094725609,-321.44321182946)) ;
#38762=CARTESIAN_POINT('Ctrl Pts',(-18.2338264609811,3.49692575915674,-321.442190774184)) ;
#38763=CARTESIAN_POINT('Ctrl Pts',(-18.2809559628799,3.24531665021227,-321.438945017754)) ;
#38764=CARTESIAN_POINT('Ctrl Pts',(-18.3108782737827,3.07199741370157,-321.43674061953)) ;
#38765=CARTESIAN_POINT('Ctrl Pts',(-18.3814490209434,2.62547384533979,-321.431116143139)) ;
#38766=CARTESIAN_POINT('Ctrl Pts',(-18.4184716994345,2.3517401358521,-321.427720204435)) ;
#38767=CARTESIAN_POINT('Ctrl Pts',(-18.5302756169096,1.35875415618312,-321.415466975611)) ;
#38768=CARTESIAN_POINT('Ctrl Pts',(-18.5691326711767,0.636112376331237,
-321.406649262026)) ;
#38769=CARTESIAN_POINT('Ctrl Pts',(-18.5650214629265,-0.241742058535704,
-321.395601475048)) ;
#38770=CARTESIAN_POINT('Ctrl Pts',(-18.5623606325034,-0.39652086832534,
-321.393642168482)) ;
#38771=CARTESIAN_POINT('Ctrl Pts',(-18.554015991005,-0.67744317070272,-321.390062424453)) ;
#38772=CARTESIAN_POINT('Ctrl Pts',(-18.5489803257875,-0.803596580637598,
-321.388446231327)) ;
#38773=CARTESIAN_POINT('Ctrl Pts',(-18.5360057298744,-1.06237513830523,
-321.385112190483)) ;
#38774=CARTESIAN_POINT('Ctrl Pts',(-18.5279291130494,-1.19498622238906,
-321.383393539874)) ;
#38775=CARTESIAN_POINT('Ctrl Pts',(-18.5029748879721,-1.5430942410394,-321.378854997202)) ;
#38776=CARTESIAN_POINT('Ctrl Pts',(-18.4837560873108,-1.75840273852584,
-321.376020449715)) ;
#38777=CARTESIAN_POINT('Ctrl Pts',(-18.4315581388728,-2.24672290020516,
-321.369533046572)) ;
#38778=CARTESIAN_POINT('Ctrl Pts',(-18.3962642893974,-2.51943624577202,
-321.365867937757)) ;
#38779=CARTESIAN_POINT('Ctrl Pts',(-18.2928622568172,-3.19939213119415,
-321.356649462532)) ;
#38780=CARTESIAN_POINT('Ctrl Pts',(-18.2172026127313,-3.60533605136708,
-321.351071687942)) ;
#38781=CARTESIAN_POINT('Ctrl Pts',(-18.0526673496658,-4.34944676330505,
-321.340829769545)) ;
#38782=CARTESIAN_POINT('Ctrl Pts',(-17.9676520818475,-4.68827954790101,
-321.336159915841)) ;
#38783=CARTESIAN_POINT('Ctrl Pts',(-17.8464172843778,-5.11953437651732,
-321.330283798345)) ;
#38784=CARTESIAN_POINT('Ctrl Pts',(-17.8189472675903,-5.21434180282661,
-321.328996327711)) ;
#38785=CARTESIAN_POINT('Ctrl Pts',(-17.7717088874472,-5.37264217338237,
-321.326856534197)) ;
#38786=CARTESIAN_POINT('Ctrl Pts',(-17.7523531157764,-5.43625602711678,
-321.325999410075)) ;
#38787=CARTESIAN_POINT('Ctrl Pts',(-17.7089314123988,-5.57625876556316,
-321.324119715452)) ;
#38788=CARTESIAN_POINT('Ctrl Pts',(-17.6847121379826,-5.65259853606334,
-321.323098935911)) ;
#38789=CARTESIAN_POINT('Ctrl Pts',(-17.6057745591643,-5.89593791946631,
-321.319855212502)) ;
#38790=CARTESIAN_POINT('Ctrl Pts',(-17.5491787803681,-6.06231854184286,
-321.31765253648)) ;
#38791=CARTESIAN_POINT('Ctrl Pts',(-17.3977002568815,-6.48772783950895,
-321.312034085747)) ;
#38792=CARTESIAN_POINT('Ctrl Pts',(-17.2993913045127,-6.7454909107858,-321.308642388856)) ;
#38793=CARTESIAN_POINT('Ctrl Pts',(-16.9218236738815,-7.67285086517161,
-321.296364294087)) ;
#38794=CARTESIAN_POINT('Ctrl Pts',(-16.6091271095143,-8.32812423915863,
-321.28751796952)) ;
#38795=CARTESIAN_POINT('Ctrl Pts',(-16.1844895669003,-9.09838166631953,
-321.276447431909)) ;
#38796=CARTESIAN_POINT('Ctrl Pts',(-16.10840611673,-9.23241592298982,-321.274496487235)) ;
#38797=CARTESIAN_POINT('Ctrl Pts',(-15.967050667723,-9.47437039733924,-321.270926941445)) ;
#38798=CARTESIAN_POINT('Ctrl Pts',(-15.9023309449355,-9.58260256487726,
-321.269312496044)) ;
#38799=CARTESIAN_POINT('Ctrl Pts',(-15.7670413936007,-9.80370451854424,
-321.265976833247)) ;
#38800=CARTESIAN_POINT('Ctrl Pts',(-15.6963502084062,-9.91649165111407,
-321.264254758497)) ;
#38801=CARTESIAN_POINT('Ctrl Pts',(-15.5069229827646,-10.2116199437786,
-321.259693817793)) ;
#38802=CARTESIAN_POINT('Ctrl Pts',(-15.3861839077494,-10.3926506131017,
-321.256840020618)) ;
#38803=CARTESIAN_POINT('Ctrl Pts',(-15.1041888982384,-10.7997719307196,
-321.250296723522)) ;
#38804=CARTESIAN_POINT('Ctrl Pts',(-14.94098638489,-11.0244510725298,-321.2465946287)) ;
#38805=CARTESIAN_POINT('Ctrl Pts',(-14.5227354164783,-11.5738978646879,
-321.237337398802)) ;
#38806=CARTESIAN_POINT('Ctrl Pts',(-14.2617757511996,-11.8939777922701,
-321.231758688496)) ;
#38807=CARTESIAN_POINT('Ctrl Pts',(-13.7640319265021,-12.4645279967601,
-321.22158476529)) ;
#38808=CARTESIAN_POINT('Ctrl Pts',(-13.5305274002108,-12.7176201458588,
-321.21698279818)) ;
#38809=CARTESIAN_POINT('Ctrl Pts',(-13.2213439333629,-13.0345796016436,
-321.211175022859)) ;
#38810=CARTESIAN_POINT('Ctrl Pts',(-13.1520071673275,-13.1045376991168,
-321.209890343524)) ;
#38811=CARTESIAN_POINT('Ctrl Pts',(-13.0349531942135,-13.2207757927619,
-321.207753664809)) ;
#38812=CARTESIAN_POINT('Ctrl Pts',(-12.9875382713322,-13.2673571981927,
-321.206896897808)) ;
#38813=CARTESIAN_POINT('Ctrl Pts',(-12.8823586180403,-13.3695837159411,
-321.205016091625)) ;
#38814=CARTESIAN_POINT('Ctrl Pts',(-12.8244814940322,-13.4251110510982,
-321.203993864037)) ;
#38815=CARTESIAN_POINT('Ctrl Pts',(-12.6381150642949,-13.601606123072,-321.200739450131)) ;
#38816=CARTESIAN_POINT('Ctrl Pts',(-12.5082600044262,-13.7211177882528,
-321.198527716494)) ;
#38817=CARTESIAN_POINT('Ctrl Pts',(-12.1697321553273,-14.023880797109,-321.192877529467)) ;
#38818=CARTESIAN_POINT('Ctrl Pts',(-11.9586159832558,-14.2043344617312,
-321.18946347939)) ;
#38819=CARTESIAN_POINT('Ctrl Pts',(-11.5584460208683,-14.5311365177886,
-321.183128385953)) ;
#38820=CARTESIAN_POINT('Ctrl Pts',(-11.3704594376938,-14.6787007294498,
-321.180205678497)) ;
#38821=CARTESIAN_POINT('Ctrl Pts',(-11.1364970237608,-14.8551626918416,
-321.176610858299)) ;
#38822=CARTESIAN_POINT('Ctrl Pts',(-11.0931750088994,-14.8875415291433,
-321.175946991067)) ;
#38823=CARTESIAN_POINT('Ctrl Pts',(-10.7170795188159,-15.1660818736563,
-321.170197464649)) ;
#38824=CARTESIAN_POINT('Ctrl Pts',(-10.3763020132811,-15.4012398305283,
-321.165077653316)) ;
#38825=CARTESIAN_POINT('Ctrl Pts',(-9.87855046465923,-15.720695100656,-321.157641884768)) ;
#38826=CARTESIAN_POINT('Ctrl Pts',(-9.72778275923691,-15.8144318956399,
-321.155395421945)) ;
#38827=CARTESIAN_POINT('Ctrl Pts',(-9.46741128734566,-15.9711802195836,
-321.151521572812)) ;
#38828=CARTESIAN_POINT('Ctrl Pts',(-9.35846566829252,-16.0352609698795,
-321.149902370479)) ;
#38829=CARTESIAN_POINT('Ctrl Pts',(-9.1314697835787,-16.1656763734935,-321.146531202773)) ;
#38830=CARTESIAN_POINT('Ctrl Pts',(-9.01333098238725,-16.2318420875986,
-321.144778098761)) ;
#38831=CARTESIAN_POINT('Ctrl Pts',(-8.69201142966656,-16.4072130754982,
-321.140013315394)) ;
#38832=CARTESIAN_POINT('Ctrl Pts',(-8.48750237065317,-16.5139337166767,
-321.136984106584)) ;
#38833=CARTESIAN_POINT('Ctrl Pts',(-8.13663973559233,-16.6887875492076,
-321.131796748152)) ;
#38834=CARTESIAN_POINT('Ctrl Pts',(-7.99128912571933,-16.7588732936713,
-321.129650632382)) ;
#38835=CARTESIAN_POINT('Ctrl Pts',(-7.30430432112103,-17.0791566467067,
-321.11952925617)) ;
#38836=CARTESIAN_POINT('Ctrl Pts',(-6.75172893726466,-17.3050457214866,
-321.111439588634)) ;
#38837=CARTESIAN_POINT('Ctrl Pts',(-6.02972049173782,-17.5603416286927,
-321.101187198994)) ;
#38838=CARTESIAN_POINT('Ctrl Pts',(-5.86943732355182,-17.6145630926653,
-321.098931735677)) ;
#38839=CARTESIAN_POINT('Ctrl Pts',(-5.57070866755272,-17.7110884316116,
-321.094778502953)) ;
#38840=CARTESIAN_POINT('Ctrl Pts',(-5.43246610636719,-17.7539787261206,
-321.092876318307)) ;
#38841=CARTESIAN_POINT('Ctrl Pts',(-5.22205801705098,-17.8165709907623,
-321.090018272863)) ;
#38842=CARTESIAN_POINT('Ctrl Pts',(-5.15025175736081,-17.8374605439789,
-321.089049422022)) ;
#38843=CARTESIAN_POINT('Ctrl Pts',(-5.01251899244279,-17.8766281170937,
-321.087204857893)) ;
#38844=CARTESIAN_POINT('Ctrl Pts',(-4.94661392167707,-17.8949766747085,
-321.086328379568)) ;
#38845=CARTESIAN_POINT('Ctrl Pts',(-4.77332140743007,-17.9421923760844,
-321.084038318427)) ;
#38846=CARTESIAN_POINT('Ctrl Pts',(-4.66577327704844,-17.9704597688143,
-321.082631655385)) ;
#38847=CARTESIAN_POINT('Ctrl Pts',(-4.42100569489804,-18.0324477717365,
-321.07945728508)) ;
#38848=CARTESIAN_POINT('Ctrl Pts',(-4.2836421025616,-18.0655715220009,-321.077694995562)) ;
#38849=CARTESIAN_POINT('Ctrl Pts',(-3.80869134639994,-18.1743791335283,
-321.071650161654)) ;
#38850=CARTESIAN_POINT('Ctrl Pts',(-3.4693750718466,-18.2421935053115,-321.067414504976)) ;
#38851=CARTESIAN_POINT('Ctrl Pts',(-2.55090668467733,-18.3992003563335,
-321.056001949037)) ;
#38852=CARTESIAN_POINT('Ctrl Pts',(-1.96910279591997,-18.4705260229598,
-321.048819995786)) ;
#38853=CARTESIAN_POINT('Ctrl Pts',(-1.19977361247041,-18.528073501455,-321.039133731395)) ;
#38854=CARTESIAN_POINT('Ctrl Pts',(-1.01444628055894,-18.5391440736732,
-321.036787103497)) ;
#38855=CARTESIAN_POINT('Ctrl Pts',(-0.70274171273618,-18.5530758239662,
-321.032813177132)) ;
#38856=CARTESIAN_POINT('Ctrl Pts',(-0.576444870820422,-18.5574292320431,
-321.03119558323)) ;
#38857=CARTESIAN_POINT('Ctrl Pts',(-0.317494920592336,-18.5637090696417,
-321.02786274773)) ;
#38858=CARTESIAN_POINT('Ctrl Pts',(-0.184845762462451,-18.5655037483158,
-321.026146745863)) ;
#38859=CARTESIAN_POINT('Ctrl Pts',(0.162848336460811,-18.5664811205678,
-321.021625525326)) ;
#38860=CARTESIAN_POINT('Ctrl Pts',(0.377879500041982,-18.5633495795523,
-321.018805863255)) ;
#38861=CARTESIAN_POINT('Ctrl Pts',(0.865538594469597,-18.5477707712694,
-321.012361536018)) ;
#38862=CARTESIAN_POINT('Ctrl Pts',(1.13804417427402,-18.5330465032616,-321.00872487761)) ;
#38863=CARTESIAN_POINT('Ctrl Pts',(1.76035905674306,-18.4856433641254,-321.000360923647)) ;
#38864=CARTESIAN_POINT('Ctrl Pts',(2.10976473556348,-18.4490316012564,-320.995621477894)) ;
#38865=CARTESIAN_POINT('Ctrl Pts',(2.67472303940375,-18.3735733562417,-320.987949575845)) ;
#38866=CARTESIAN_POINT('Ctrl Pts',(2.89099700256591,-18.3407872698519,-320.985010980969)) ;
#38867=CARTESIAN_POINT('Ctrl Pts',(3.32395468581166,-18.2673044038235,-320.979150678499)) ;
#38868=CARTESIAN_POINT('Ctrl Pts',(3.54059455844515,-18.2265541293349,-320.976229747398)) ;
#38869=CARTESIAN_POINT('Ctrl Pts',(3.84180506439198,-18.1643229535366,-320.972206660472)) ;
#38870=CARTESIAN_POINT('Ctrl Pts',(3.9270273744167,-18.1460891252998,-320.971072710082)) ;
#38871=CARTESIAN_POINT('Ctrl Pts',(4.07631377204857,-18.1130474626584,-320.969095827574)) ;
#38872=CARTESIAN_POINT('Ctrl Pts',(4.14043325883232,-18.0984981365315,-320.968249958418)) ;
#38873=CARTESIAN_POINT('Ctrl Pts',(4.28957087228558,-18.063823349431,-320.96628997208)) ;
#38874=CARTESIAN_POINT('Ctrl Pts',(4.37452674907062,-18.0434378104393,-320.965178879921)) ;
#38875=CARTESIAN_POINT('Ctrl Pts',(4.68093816193899,-17.9676217544116,-320.961186340006)) ;
#38876=CARTESIAN_POINT('Ctrl Pts',(4.90151098323219,-17.9087074923046,-320.958340182304)) ;
#38877=CARTESIAN_POINT('Ctrl Pts',(5.54119533449275,-17.7251462613375,-320.950105384838)) ;
#38878=CARTESIAN_POINT('Ctrl Pts',(5.95705865844338,-17.5897444218911,-320.944773699598)) ;
#38879=CARTESIAN_POINT('Ctrl Pts',(6.52898730769165,-17.3809173002409,-320.937306280708)) ;
#38880=CARTESIAN_POINT('Ctrl Pts',(6.68939668491061,-17.3198133189774,-320.935197241083)) ;
#38881=CARTESIAN_POINT('Ctrl Pts',(7.18265247710496,-17.1240448640527,-320.928650009788)) ;
#38882=CARTESIAN_POINT('Ctrl Pts',(7.51245640728795,-16.9819435579419,-320.924182775271)) ;
#38883=CARTESIAN_POINT('Ctrl Pts',(7.97955432853323,-16.7644152610639,-320.917678466205)) ;
#38884=CARTESIAN_POINT('Ctrl Pts',(8.12033879191652,-16.6966764397983,-320.91569461067)) ;
#38885=CARTESIAN_POINT('Ctrl Pts',(8.37137484181892,-16.571963634615,-320.912112281403)) ;
#38886=CARTESIAN_POINT('Ctrl Pts',(8.48194197793596,-16.5156457845681,-320.910518610243)) ;
#38887=CARTESIAN_POINT('Ctrl Pts',(8.72171101956119,-16.3904755162238,-320.907027147084)) ;
#38888=CARTESIAN_POINT('Ctrl Pts',(8.85067990100838,-16.3211946855445,-320.905126311799)) ;
#38889=CARTESIAN_POINT('Ctrl Pts',(9.2401331729044,-16.1060104399365,-320.89931640354)) ;
#38890=CARTESIAN_POINT('Ctrl Pts',(9.49792926356835,-15.9553430677548,-320.895373679594)) ;
#38891=CARTESIAN_POINT('Ctrl Pts',(10.1495847319862,-15.5530947181484,-320.885174929886)) ;
#38892=CARTESIAN_POINT('Ctrl Pts',(10.5377826787426,-15.2927420819336,-320.878871342854)) ;
#38893=CARTESIAN_POINT('Ctrl Pts',(11.0519558102177,-14.9190189967723,-320.87031301975)) ;
#38894=CARTESIAN_POINT('Ctrl Pts',(11.1868146477109,-14.8181656470127,-320.868048380536)) ;
#38895=CARTESIAN_POINT('Ctrl Pts',(11.5250936291658,-14.5579355553234,-320.862330984766)) ;
#38896=CARTESIAN_POINT('Ctrl Pts',(11.7265931647289,-14.3961204488615,-320.858890585307)) ;
#38897=CARTESIAN_POINT('Ctrl Pts',(12.0030453667017,-14.1644577368843,-320.854155430891)) ;
#38898=CARTESIAN_POINT('Ctrl Pts',(12.080896989979,-14.0981165060473,-320.852820306291)) ;
#38899=CARTESIAN_POINT('Ctrl Pts',(12.2088074101956,-13.9872801416566,-320.850626801878)) ;
#38900=CARTESIAN_POINT('Ctrl Pts',(12.2591807240461,-13.9431514427424,-320.84976304513)) ;
#38901=CARTESIAN_POINT('Ctrl Pts',(12.347012908264,-13.8653635923331,-320.848257719402)) ;
#38902=CARTESIAN_POINT('Ctrl Pts',(12.3845755026972,-13.8318229069246,-320.847614098582)) ;
#38903=CARTESIAN_POINT('Ctrl Pts',(12.422830908549,-13.797382826699,-320.846958501836)) ;
#38904=CARTESIAN_POINT('Ctrl Pts',(12.4236605585145,-13.7966357847014,-320.846944283774)) ;
#38905=CARTESIAN_POINT('Ctrl Pts',(12.4253334184184,-13.7951292176448,-320.846915615159)) ;
#38906=CARTESIAN_POINT('Ctrl Pts',(12.4261766261117,-13.7943696900967,-320.846901164644)) ;
#38907=CARTESIAN_POINT('Ctrl Pts',(12.4278775871989,-13.792837250299,-320.846872014218)) ;
#38908=CARTESIAN_POINT('Ctrl Pts',(12.4287353381248,-13.7920643353518,-320.846857314349)) ;
#38909=CARTESIAN_POINT('Ctrl Pts',(12.4304664070157,-13.7905041854523,-320.8468276477)) ;
#38910=CARTESIAN_POINT('Ctrl Pts',(12.4313397223338,-13.7897169475247,-320.846812680963)) ;
#38911=CARTESIAN_POINT('Ctrl Pts',(12.4331029805614,-13.7881271793275,-320.846782462391)) ;
#38912=CARTESIAN_POINT('Ctrl Pts',(12.4339929205518,-13.7873246458557,-320.846767210603)) ;
#38913=CARTESIAN_POINT('Ctrl Pts',(12.4357905311635,-13.7857032741128,-320.846736403009)) ;
#38914=CARTESIAN_POINT('Ctrl Pts',(12.4366981986449,-13.7848844323297,-320.846720847254)) ;
#38915=CARTESIAN_POINT('Ctrl Pts',(12.4385324136172,-13.7832293877603,-320.846689412012)) ;
#38916=CARTESIAN_POINT('Ctrl Pts',(12.4394589576725,-13.7823931811789,-320.84667353258)) ;
#38917=CARTESIAN_POINT('Ctrl Pts',(12.4413321252574,-13.7807023035147,-320.846641429409)) ;
#38918=CARTESIAN_POINT('Ctrl Pts',(12.442278745047,-13.7798476283161,-320.846625205729)) ;
#38919=CARTESIAN_POINT('Ctrl Pts',(12.4441933176402,-13.7781186588381,-320.846592392559)) ;
#38920=CARTESIAN_POINT('Ctrl Pts',(12.4451612663977,-13.7772443600736,-320.846575803134)) ;
#38921=CARTESIAN_POINT('Ctrl Pts',(12.4471198088701,-13.7754749336878,-320.846542235964)) ;
#38922=CARTESIAN_POINT('Ctrl Pts',(12.4481103981702,-13.7745798012134,-320.84652525829)) ;
#38923=CARTESIAN_POINT('Ctrl Pts',(12.4501155964154,-13.7727674382869,-320.846490891038)) ;
#38924=CARTESIAN_POINT('Ctrl Pts',(12.4511302005791,-13.7718502025498,-320.846473501536)) ;
#38925=CARTESIAN_POINT('Ctrl Pts',(12.4531848707809,-13.769992300043,-320.846438285883)) ;
#38926=CARTESIAN_POINT('Ctrl Pts',(12.454224931607,-13.7690516275461,-320.846420459814)) ;
#38927=CARTESIAN_POINT('Ctrl Pts',(12.4563320297982,-13.767145449827,-320.846384345035)) ;
#38928=CARTESIAN_POINT('Ctrl Pts',(12.4573990615042,-13.7661799383745,-320.846366056414)) ;
#38929=CARTESIAN_POINT('Ctrl Pts',(12.45956169374,-13.7642226074135,-320.846328989207)) ;
#38930=CARTESIAN_POINT('Ctrl Pts',(12.4606572881552,-13.7632307810954,-320.846310210716)) ;
#38931=CARTESIAN_POINT('Ctrl Pts',(12.4628787214654,-13.7612192658872,-320.84627213501)) ;
#38932=CARTESIAN_POINT('Ctrl Pts',(12.4640045536628,-13.7601995696302,-320.8462528379)) ;
#38933=CARTESIAN_POINT('Ctrl Pts',(12.4662882272162,-13.7581306753456,-320.846213694666)) ;
#38934=CARTESIAN_POINT('Ctrl Pts',(12.467446061298,-13.7570814692848,-320.846193848656)) ;
#38935=CARTESIAN_POINT('Ctrl Pts',(12.4697955986901,-13.7549518253206,-320.846153575691)) ;
#38936=CARTESIAN_POINT('Ctrl Pts',(12.4709872940606,-13.753871378684,-320.84613314886)) ;
#38937=CARTESIAN_POINT('Ctrl Pts',(12.4734065159742,-13.7516774262804,-320.846091680573)) ;
#38938=CARTESIAN_POINT('Ctrl Pts',(12.4746340338825,-13.7505639109789,-320.84607063925)) ;
#38939=CARTESIAN_POINT('Ctrl Pts',(12.4771269717987,-13.7483018897778,-320.84602790642)) ;
#38940=CARTESIAN_POINT('Ctrl Pts',(12.4783923823665,-13.7471533735007,-320.84600621506)) ;
#38941=CARTESIAN_POINT('Ctrl Pts',(12.4809632928688,-13.7448193074489,-320.845962144594)) ;
#38942=CARTESIAN_POINT('Ctrl Pts',(12.4822687824885,-13.7436337463595,-320.845939765649)) ;
#38943=CARTESIAN_POINT('Ctrl Pts',(12.4849221626022,-13.7412234285417,-320.845894280315)) ;
#38944=CARTESIAN_POINT('Ctrl Pts',(12.4862700418181,-13.7399986594663,-320.845871174101)) ;
#38945=CARTESIAN_POINT('Ctrl Pts',(12.489010645151,-13.7375076360629,-320.845824192248)) ;
#38946=CARTESIAN_POINT('Ctrl Pts',(12.4904033569655,-13.7362413682159,-320.845800316799)) ;
#38947=CARTESIAN_POINT('Ctrl Pts',(12.4932362110586,-13.733664921199,-320.845751752057)) ;
#38948=CARTESIAN_POINT('Ctrl Pts',(12.4946763398566,-13.7323547272602,-320.845727062971)) ;
#38949=CARTESIAN_POINT('Ctrl Pts',(12.4976067642843,-13.7296878562249,-320.845676823939)) ;
#38950=CARTESIAN_POINT('Ctrl Pts',(12.4990970451752,-13.7283311629399,-320.845651274217)) ;
#38951=CARTESIAN_POINT('Ctrl Pts',(12.5021306711494,-13.7255685653632,-320.84559926412)) ;
#38952=CARTESIAN_POINT('Ctrl Pts',(12.5036740000402,-13.724162643371,-320.845572803991)) ;
#38953=CARTESIAN_POINT('Ctrl Pts',(12.5068167907788,-13.7212986939471,-320.845518920331)) ;
#38954=CARTESIAN_POINT('Ctrl Pts',(12.5084162349025,-13.719840647072,-320.845491497067)) ;
#38955=CARTESIAN_POINT('Ctrl Pts',(12.5116745077088,-13.7168693752333,-320.845435631234)) ;
#38956=CARTESIAN_POINT('Ctrl Pts',(12.5133333169261,-13.715356128937,-320.845407188957)) ;
#38957=CARTESIAN_POINT('Ctrl Pts',(12.5167137664157,-13.7122711950416,-320.845349225831)) ;
#38958=CARTESIAN_POINT('Ctrl Pts',(12.5184353852484,-13.7106994840565,-320.845319705302)) ;
#38959=CARTESIAN_POINT('Ctrl Pts',(12.5207010381076,-13.7086303276533,-320.845280855335)) ;
#38960=CARTESIAN_POINT('Ctrl Pts',(12.5212453385744,-13.7081331740378,-320.845271521949)) ;
#38961=CARTESIAN_POINT('Ctrl Pts',(12.52238946442,-13.707088026418,-320.845251902919)) ;
#38962=CARTESIAN_POINT('Ctrl Pts',(12.5229892833514,-13.7065400255372,-320.845241617369)) ;
#38963=CARTESIAN_POINT('Ctrl Pts',(12.5242505324788,-13.7053875831748,-320.845219989595)) ;
#38964=CARTESIAN_POINT('Ctrl Pts',(12.5249119549761,-13.7047831331048,-320.845208647484)) ;
#38965=CARTESIAN_POINT('Ctrl Pts',(12.5263032406586,-13.7035115026549,-320.845184789413)) ;
#38966=CARTESIAN_POINT('Ctrl Pts',(12.5270330943375,-13.70284431181,-320.845172273595)) ;
#38967=CARTESIAN_POINT('Ctrl Pts',(12.5285689174822,-13.7014401241312,-320.845145936418)) ;
#38968=CARTESIAN_POINT('Ctrl Pts',(12.5293748751748,-13.7007031145336,-320.845132115234)) ;
#38969=CARTESIAN_POINT('Ctrl Pts',(12.5310715453699,-13.6991513162155,-320.845103019084)) ;
#38970=CARTESIAN_POINT('Ctrl Pts',(12.5319622434424,-13.6983365117332,-320.845087744329)) ;
#38971=CARTESIAN_POINT('Ctrl Pts',(12.533838134394,-13.6966201234746,-320.845055573887)) ;
#38972=CARTESIAN_POINT('Ctrl Pts',(12.5348233094746,-13.6957185202607,-320.845038678459)) ;
#38973=CARTESIAN_POINT('Ctrl Pts',(12.5368991531778,-13.693818357647,-320.845003077894)) ;
#38974=CARTESIAN_POINT('Ctrl Pts',(12.537989799808,-13.6928197742134,-320.844984373078)) ;
#38975=CARTESIAN_POINT('Ctrl Pts',(12.5402890262243,-13.6907141240886,-320.844944940207)) ;
#38976=CARTESIAN_POINT('Ctrl Pts',(12.5414975787445,-13.6896070276363,-320.844924212547)) ;
#38977=CARTESIAN_POINT('Ctrl Pts',(12.5440467071742,-13.6872712736131,-320.844880492086)) ;
#38978=CARTESIAN_POINT('Ctrl Pts',(12.5453872492322,-13.6860425790674,-320.844857499776)) ;
#38979=CARTESIAN_POINT('Ctrl Pts',(12.5482163392036,-13.6834487679956,-320.844808975583)) ;
#38980=CARTESIAN_POINT('Ctrl Pts',(12.5497048449031,-13.6820836054905,-320.844783444308)) ;
#38981=CARTESIAN_POINT('Ctrl Pts',(12.5528480138123,-13.6791999469402,-320.84472953045)) ;
#38982=CARTESIAN_POINT('Ctrl Pts',(12.5545026243144,-13.6776813935083,-320.844701148622)) ;
#38983=CARTESIAN_POINT('Ctrl Pts',(12.5579986406389,-13.6744716824819,-320.844641179143)) ;
#38984=CARTESIAN_POINT('Ctrl Pts',(12.5598399805121,-13.6727804530469,-320.844609592432)) ;
#38985=CARTESIAN_POINT('Ctrl Pts',(12.5637329407349,-13.6692034062649,-320.844542809657)) ;
#38986=CARTESIAN_POINT('Ctrl Pts',(12.5657844782362,-13.6673174988537,-320.844507614768)) ;
#38987=CARTESIAN_POINT('Ctrl Pts',(12.570124574674,-13.6633259951856,-320.844433156025)) ;
#38988=CARTESIAN_POINT('Ctrl Pts',(12.5724130293264,-13.6612202856685,-320.84439389364)) ;
#38989=CARTESIAN_POINT('Ctrl Pts',(12.5772574159256,-13.656760500591,-320.844310776258)) ;
#38990=CARTESIAN_POINT('Ctrl Pts',(12.5798132163043,-13.6544062822173,-320.844266923099)) ;
#38991=CARTESIAN_POINT('Ctrl Pts',(12.5852269761786,-13.649416708182,-320.844174027606)) ;
#38992=CARTESIAN_POINT('Ctrl Pts',(12.5880847692085,-13.6467811720843,-320.844124987578)) ;
#38993=CARTESIAN_POINT('Ctrl Pts',(12.5941419839316,-13.6411915188584,-320.844021039087)) ;
#38994=CARTESIAN_POINT('Ctrl Pts',(12.597341194515,-13.638237173278,-320.84396613352)) ;
#38995=CARTESIAN_POINT('Ctrl Pts',(12.6041261097789,-13.6319671457317,-320.843849681353)) ;
#38996=CARTESIAN_POINT('Ctrl Pts',(12.6077115462354,-13.6286511739221,-320.843788138393)) ;
#38997=CARTESIAN_POINT('Ctrl Pts',(12.6153198202074,-13.6216091304664,-320.843657534154)) ;
#38998=CARTESIAN_POINT('Ctrl Pts',(12.6193423163008,-13.6178826905415,-320.843588477452)) ;
#38999=CARTESIAN_POINT('Ctrl Pts',(12.6278823246765,-13.6099641945841,-320.843441851935)) ;
#39000=CARTESIAN_POINT('Ctrl Pts',(12.6323994017711,-13.6057716700626,-320.843364288875)) ;
#39001=CARTESIAN_POINT('Ctrl Pts',(12.6419935569205,-13.5968579596751,-320.843199528471)) ;
#39002=CARTESIAN_POINT('Ctrl Pts',(12.6470700797698,-13.5921361774447,-320.843112338354)) ;
#39003=CARTESIAN_POINT('Ctrl Pts',(12.7559151491712,-13.490783283132,-320.84124265685)) ;
#39004=CARTESIAN_POINT('Ctrl Pts',(12.8585760876792,-13.3929692737651,-320.839474299984)) ;
#39005=CARTESIAN_POINT('Ctrl Pts',(13.2094835596114,-13.0508749413233,-320.83339507716)) ;
#39006=CARTESIAN_POINT('Ctrl Pts',(13.4519708152967,-12.8007919462534,-320.829131610642)) ;
#39007=CARTESIAN_POINT('Ctrl Pts',(14.0834582008665,-12.1117517965977,-320.817684179353)) ;
#39008=CARTESIAN_POINT('Ctrl Pts',(14.458934082965,-11.6609412289553,-320.810494308593)) ;
#39009=CARTESIAN_POINT('Ctrl Pts',(14.9232976235467,-11.0464245610801,-320.800820895901)) ;
#39010=CARTESIAN_POINT('Ctrl Pts',(15.0319644135627,-10.8980894317352,-320.798496179525)) ;
#39011=CARTESIAN_POINT('Ctrl Pts',(15.1951310177363,-10.668275045164,-320.794905878076)) ;
#39012=CARTESIAN_POINT('Ctrl Pts',(15.2512189090527,-10.5879375162876,-320.793652903881)) ;
#39013=CARTESIAN_POINT('Ctrl Pts',(15.3618082707327,-10.4268326418247,-320.79114394585)) ;
#39014=CARTESIAN_POINT('Ctrl Pts',(15.4163151233284,-10.3460726984133,-320.789888056903)) ;
#39015=CARTESIAN_POINT('Ctrl Pts',(15.5581665798855,-10.1322887586249,-320.786567982216)) ;
#39016=CARTESIAN_POINT('Ctrl Pts',(15.644440906834,-9.99856446808686,-320.784495683405)) ;
#39017=CARTESIAN_POINT('Ctrl Pts',(15.8252165767743,-9.7102949448736,-320.780038208964)) ;
#39018=CARTESIAN_POINT('Ctrl Pts',(15.9191969056721,-9.55544228986516,-320.777649594224)) ;
#39019=CARTESIAN_POINT('Ctrl Pts',(16.1863093086688,-9.10043643957008,-320.770652604501)) ;
#39020=CARTESIAN_POINT('Ctrl Pts',(16.3533231653468,-8.79678197746626,-320.766008732895)) ;
#39021=CARTESIAN_POINT('Ctrl Pts',(16.7839538411502,-7.95913678783804,-320.753336220576)) ;
#39022=CARTESIAN_POINT('Ctrl Pts',(17.0305388138956,-7.41685331340842,-320.74527165753)) ;
#39023=CARTESIAN_POINT('Ctrl Pts',(17.2933933793987,-6.75621327027029,-320.735911031052)) ;
#39024=CARTESIAN_POINT('Ctrl Pts',(17.3351401608174,-6.64836731805396,-320.734397777836)) ;
#39025=CARTESIAN_POINT('Ctrl Pts',(17.3978682413441,-6.48171099600536,-320.732085870426)) ;
#39026=CARTESIAN_POINT('Ctrl Pts',(17.4195649763844,-6.42317311181392,-320.731278825554)) ;
#39027=CARTESIAN_POINT('Ctrl Pts',(17.4616779413934,-6.30776927918751,-320.729698439182)) ;
#39028=CARTESIAN_POINT('Ctrl Pts',(17.482112654417,-6.25091089004718,-320.728924868416)) ;
#39029=CARTESIAN_POINT('Ctrl Pts',(17.526419773313,-6.1257121612018,-320.727231666812)) ;
#39030=CARTESIAN_POINT('Ctrl Pts',(17.5501707797211,-6.05732987140556,-320.726313476044)) ;
#39031=CARTESIAN_POINT('Ctrl Pts',(17.6617734445469,-5.72984383007534,-320.721944267278)) ;
#39032=CARTESIAN_POINT('Ctrl Pts',(17.7442907779709,-5.46895757131407,-320.718546811316)) ;
#39033=CARTESIAN_POINT('Ctrl Pts',(17.8244844903586,-5.19445909918696,-320.715020738442)) ;
#39034=CARTESIAN_POINT('Ctrl Pts',(17.827944405358,-5.1825718479975,-320.714868136358)) ;
#39035=CARTESIAN_POINT('Ctrl Pts',(17.9629053570108,-4.71715121498048,-320.708896945127)) ;
#39036=CARTESIAN_POINT('Ctrl Pts',(18.0770676090544,-4.25876881699607,-320.703145854989)) ;
#39037=CARTESIAN_POINT('Ctrl Pts',(18.2577648608132,-3.39378896399032,-320.692274171537)) ;
#39038=CARTESIAN_POINT('Ctrl Pts',(18.3284883741086,-2.98835975916959,-320.687171453859)) ;
#39039=CARTESIAN_POINT('Ctrl Pts',(18.4078610802873,-2.4229322985058,-320.679971512952)) ;
#39040=CARTESIAN_POINT('Ctrl Pts',(18.428001193603,-2.2646682716537,-320.677947632587)) ;
#39041=CARTESIAN_POINT('Ctrl Pts',(18.4596253998129,-1.98769881711682,-320.674387965691)) ;
#39042=CARTESIAN_POINT('Ctrl Pts',(18.4720101908752,-1.8691056556958,-320.6728581244)) ;
#39043=CARTESIAN_POINT('Ctrl Pts',(18.4942285503858,-1.63449232577273,-320.669819773694)) ;
#39044=CARTESIAN_POINT('Ctrl Pts',(18.5041148287334,-1.51848253198411,-320.668311678593)) ;
#39045=CARTESIAN_POINT('Ctrl Pts',(18.5258613915667,-1.23140628741382,-320.664565458404)) ;
#39046=CARTESIAN_POINT('Ctrl Pts',(18.5364441843054,-1.06025403462769,-320.662319402394)) ;
#39047=CARTESIAN_POINT('Ctrl Pts',(18.544654593745,-0.888979977948724,-320.660059887232)) ;
#39048=CARTESIAN_POINT('Ctrl Pts',(18.5446545929199,-0.888979995160609,
-320.363441000746)) ;
#39049=CARTESIAN_POINT('Ctrl Pts',(18.5193716592953,-1.41639711783526,-320.370544484615)) ;
#39050=CARTESIAN_POINT('Ctrl Pts',(18.4715976939239,-1.94255064943188,-320.377691476469)) ;
#39051=CARTESIAN_POINT('Ctrl Pts',(18.3801584619138,-2.62487471795141,-320.386818421463)) ;
#39052=CARTESIAN_POINT('Ctrl Pts',(18.356811497647,-2.78346262004066,-320.388929041152)) ;
#39053=CARTESIAN_POINT('Ctrl Pts',(18.3191274118357,-3.01829142334129,-320.392028994592)) ;
#39054=CARTESIAN_POINT('Ctrl Pts',(18.3063614400486,-3.09477674403978,-320.393034654064)) ;
#39055=CARTESIAN_POINT('Ctrl Pts',(18.2816380081548,-3.23739515041758,-320.394900897312)) ;
#39056=CARTESIAN_POINT('Ctrl Pts',(18.2697999343643,-3.30354748251078,-320.395762773958)) ;
#39057=CARTESIAN_POINT('Ctrl Pts',(18.2387500911096,-3.47178406006102,-320.397946263074)) ;
#39058=CARTESIAN_POINT('Ctrl Pts',(18.2190402623446,-3.57377411313504,-320.399262172644)) ;
#39059=CARTESIAN_POINT('Ctrl Pts',(18.1043956400099,-4.14139873480308,-320.40655445357)) ;
#39060=CARTESIAN_POINT('Ctrl Pts',(17.9924661075652,-4.60342166354413,-320.412376491316)) ;
#39061=CARTESIAN_POINT('Ctrl Pts',(17.693740389311,-5.65785678600442,-320.425800636004)) ;
#39062=CARTESIAN_POINT('Ctrl Pts',(17.4947030179841,-6.24621145109414,-320.43340081197)) ;
#39063=CARTESIAN_POINT('Ctrl Pts',(17.1997330863639,-6.99262145291462,-320.44348371235)) ;
#39064=CARTESIAN_POINT('Ctrl Pts',(17.1304126483206,-7.16076360291563,-320.445783670312)) ;
#39065=CARTESIAN_POINT('Ctrl Pts',(17.008987049837,-7.44343204386877,-320.449703363068)) ;
#39066=CARTESIAN_POINT('Ctrl Pts',(16.9581676935921,-7.55849650900434,-320.45131403318)) ;
#39067=CARTESIAN_POINT('Ctrl Pts',(16.850931186642,-7.79477327342072,-320.454653692936)) ;
#39068=CARTESIAN_POINT('Ctrl Pts',(16.7943660971786,-7.9159105332999,-320.456383662993)) ;
#39069=CARTESIAN_POINT('Ctrl Pts',(16.6408801684696,-8.2355572061199,-320.460996291646)) ;
#39070=CARTESIAN_POINT('Ctrl Pts',(16.5417165587628,-8.4329655693732,-320.463894525112)) ;
#39071=CARTESIAN_POINT('Ctrl Pts',(16.3687656032414,-8.76247027133729,-320.468813228458)) ;
#39072=CARTESIAN_POINT('Ctrl Pts',(16.2968434236332,-8.89551948922025,-320.470822041759)) ;
#39073=CARTESIAN_POINT('Ctrl Pts',(15.9698111304275,-9.48321723483742,-320.479790516225)) ;
#39074=CARTESIAN_POINT('Ctrl Pts',(15.6972440931399,-9.92788007665474,-320.48683958191)) ;
#39075=CARTESIAN_POINT('Ctrl Pts',(15.2098622808899,-10.6526306193253,-320.498579551596)) ;
#39076=CARTESIAN_POINT('Ctrl Pts',(15.0051259613828,-10.9391336708383,-320.503288649293)) ;
#39077=CARTESIAN_POINT('Ctrl Pts',(14.7316748338556,-11.2996611733321,-320.509226608935)) ;
#39078=CARTESIAN_POINT('Ctrl Pts',(14.6703339610787,-11.3791865946703,-320.510537086004)) ;
#39079=CARTESIAN_POINT('Ctrl Pts',(14.5671782146053,-11.5107023611944,-320.512702690796)) ;
#39080=CARTESIAN_POINT('Ctrl Pts',(14.525722984345,-11.5629720143339,-320.513562897238)) ;
#39081=CARTESIAN_POINT('Ctrl Pts',(14.4344574769705,-11.6767805753733,-320.515434113947)) ;
#39082=CARTESIAN_POINT('Ctrl Pts',(14.3845335694874,-11.7382264959883,-320.516443497067)) ;
#39083=CARTESIAN_POINT('Ctrl Pts',(14.2261619267553,-11.9306212829844,-320.519604250803)) ;
#39084=CARTESIAN_POINT('Ctrl Pts',(14.1163074260117,-12.0604009963385,-320.521736759783)) ;
#39085=CARTESIAN_POINT('Ctrl Pts',(13.8328279435697,-12.3861171246223,-320.527113064288)) ;
#39086=CARTESIAN_POINT('Ctrl Pts',(13.6568128341549,-12.5799240816472,-320.530335198743)) ;
#39087=CARTESIAN_POINT('Ctrl Pts',(12.9529339046992,-13.3227625818285,-320.542890836321)) ;
#39088=CARTESIAN_POINT('Ctrl Pts',(12.3955920297996,-13.8428247923646,-320.552166281128)) ;
#39089=CARTESIAN_POINT('Ctrl Pts',(11.6815548918013,-14.431305411428,-320.563824446303)) ;
#39090=CARTESIAN_POINT('Ctrl Pts',(11.5538493224394,-14.5337492166543,-320.565899823802)) ;
#39091=CARTESIAN_POINT('Ctrl Pts',(11.326300204395,-14.7113915108615,-320.569584002307)) ;
#39092=CARTESIAN_POINT('Ctrl Pts',(11.2270208256463,-14.7872958932533,-320.571186877826)) ;
#39093=CARTESIAN_POINT('Ctrl Pts',(11.0149913247747,-14.9460375236911,-320.574601467596)) ;
#39094=CARTESIAN_POINT('Ctrl Pts',(10.9020558649811,-15.0286143535752,-320.576415149722)) ;
#39095=CARTESIAN_POINT('Ctrl Pts',(10.5790265694362,-15.2592513823096,-320.581588839354)) ;
#39096=CARTESIAN_POINT('Ctrl Pts',(10.3667769346681,-15.4042361535363,-320.584972100217)) ;
#39097=CARTESIAN_POINT('Ctrl Pts',(9.43889840845377,-16.0101917524411,-320.599677034769)) ;
#39098=CARTESIAN_POINT('Ctrl Pts',(8.69505118729786,-16.4260499290374,-320.611300674135)) ;
#39099=CARTESIAN_POINT('Ctrl Pts',(7.7759922587815,-16.8598845264129,-320.624782828388)) ;
#39100=CARTESIAN_POINT('Ctrl Pts',(7.62574443468624,-16.928372155302,-320.626958165112)) ;
#39101=CARTESIAN_POINT('Ctrl Pts',(7.40287525068303,-17.0263935551351,-320.630132612123)) ;
#39102=CARTESIAN_POINT('Ctrl Pts',(7.33094851569702,-17.0574861381796,-320.631149147234)) ;
#39103=CARTESIAN_POINT('Ctrl Pts',(7.19721557953243,-17.1142942664819,-320.633022981492)) ;
#39104=CARTESIAN_POINT('Ctrl Pts',(7.13546313077644,-17.1401326201928,-320.633881722819)) ;
#39105=CARTESIAN_POINT('Ctrl Pts',(6.97918969310046,-17.2045293849733,-320.636039550578)) ;
#39106=CARTESIAN_POINT('Ctrl Pts',(6.88448785613743,-17.2426432757354,-320.637333227203)) ;
#39107=CARTESIAN_POINT('Ctrl Pts',(6.67247750495302,-17.3259442842373,-320.640202929229)) ;
#39108=CARTESIAN_POINT('Ctrl Pts',(6.55501459945844,-17.3707249433977,-320.64177494667)) ;
#39109=CARTESIAN_POINT('Ctrl Pts',(6.1748866788987,-17.5112371877173,-320.646816330522)) ;
#39110=CARTESIAN_POINT('Ctrl Pts',(5.91051128012946,-17.6022302605808,-320.65025287239)) ;
#39111=CARTESIAN_POINT('Ctrl Pts',(4.95955635045958,-17.9056902199376,-320.662491724235)) ;
#39112=CARTESIAN_POINT('Ctrl Pts',(4.26282267319932,-18.0842274927248,-320.671257947083)) ;
#39113=CARTESIAN_POINT('Ctrl Pts',(3.40589453628108,-18.2515271164235,-320.68224657714)) ;
#39114=CARTESIAN_POINT('Ctrl Pts',(3.25392575824277,-18.2792321157788,-320.684201841342)) ;
#39115=CARTESIAN_POINT('Ctrl Pts',(2.97722309426901,-18.3261169715746,-320.687776652543)) ;
#39116=CARTESIAN_POINT('Ctrl Pts',(2.85260552008239,-18.3459276762617,-320.689391998074)) ;
#39117=CARTESIAN_POINT('Ctrl Pts',(2.59626449120315,-18.3840037065592,-320.692726807802)) ;
#39118=CARTESIAN_POINT('Ctrl Pts',(2.4645272111221,-18.4021272453484,-320.694447101111)) ;
#39119=CARTESIAN_POINT('Ctrl Pts',(2.11748773488935,-18.4460771838712,-320.698996389186)) ;
#39120=CARTESIAN_POINT('Ctrl Pts',(1.90190831532076,-18.4695495961033,-320.701840171462)) ;
#39121=CARTESIAN_POINT('Ctrl Pts',(1.41085733004987,-18.5143267764086,-320.708354362466)) ;
#39122=CARTESIAN_POINT('Ctrl Pts',(1.1352218550829,-18.5332696874902,-320.712037187506)) ;
#39123=CARTESIAN_POINT('Ctrl Pts',(0.446871419186728,-18.5651620111208,
-320.721274192816)) ;
#39124=CARTESIAN_POINT('Ctrl Pts',(0.0339533922777227,-18.5705083738189,
-320.72685238069)) ;
#39125=CARTESIAN_POINT('Ctrl Pts',(-0.725741605102334,-18.5550052139741,
-320.737063511099)) ;
#39126=CARTESIAN_POINT('Ctrl Pts',(-1.07241920081694,-18.5381994078459,
-320.741702639691)) ;
#39127=CARTESIAN_POINT('Ctrl Pts',(-1.51667508841897,-18.5041591654962,
-320.747546865568)) ;
#39128=CARTESIAN_POINT('Ctrl Pts',(-1.61486677574162,-18.4958485905259,
-320.748832149939)) ;
#39129=CARTESIAN_POINT('Ctrl Pts',(-1.77917719082368,-18.4806235443016,
-320.750969503372)) ;
#39130=CARTESIAN_POINT('Ctrl Pts',(-1.84533326089137,-18.4741349798789,
-320.751826347344)) ;
#39131=CARTESIAN_POINT('Ctrl Pts',(-1.9912071493842,-18.4590363321358,-320.75370691056)) ;
#39132=CARTESIAN_POINT('Ctrl Pts',(-2.07090676697799,-18.4502648601334,
-320.754728822699)) ;
#39133=CARTESIAN_POINT('Ctrl Pts',(-2.32567074987145,-18.4205548322995,
-320.757980905396)) ;
#39134=CARTESIAN_POINT('Ctrl Pts',(-2.50049487729528,-18.3976387160583,
-320.760190663647)) ;
#39135=CARTESIAN_POINT('Ctrl Pts',(-2.94936177529857,-18.3322844608753,
-320.765833919831)) ;
#39136=CARTESIAN_POINT('Ctrl Pts',(-3.22282822417419,-18.2861906110619,
-320.769243085707)) ;
#39137=CARTESIAN_POINT('Ctrl Pts',(-4.20503639547139,-18.097917250415,-320.781506029079)) ;
#39138=CARTESIAN_POINT('Ctrl Pts',(-4.90636203821725,-17.9205064443765,
-320.790321308779)) ;
#39139=CARTESIAN_POINT('Ctrl Pts',(-5.7426287535191,-17.6561747490109,-320.801360029236)) ;
#39140=CARTESIAN_POINT('Ctrl Pts',(-5.88911900450835,-17.6078553216548,
-320.803312583352)) ;
#39141=CARTESIAN_POINT('Ctrl Pts',(-6.15427188587219,-17.5167161913796,
-320.806884090276)) ;
#39142=CARTESIAN_POINT('Ctrl Pts',(-6.27313278925437,-17.4745018106372,
-320.808498870328)) ;
#39143=CARTESIAN_POINT('Ctrl Pts',(-6.51647758245965,-17.3852731758689,
-320.811834211267)) ;
#39144=CARTESIAN_POINT('Ctrl Pts',(-6.64090482468461,-17.3381252310895,
-320.813555618956)) ;
#39145=CARTESIAN_POINT('Ctrl Pts',(-6.9671803853991,-17.2104653661899,-320.818112196618)) ;
#39146=CARTESIAN_POINT('Ctrl Pts',(-7.16814035790034,-17.1277401951755,
-320.820962243944)) ;
#39147=CARTESIAN_POINT('Ctrl Pts',(-7.87722464414272,-16.8211798319423,
-320.831168527099)) ;
#39148=CARTESIAN_POINT('Ctrl Pts',(-8.37670686978186,-16.5781041689362,
-320.838643890504)) ;
#39149=CARTESIAN_POINT('Ctrl Pts',(-9.25674234508558,-16.0998901560729,
-320.852134786645)) ;
#39150=CARTESIAN_POINT('Ctrl Pts',(-9.64112979901616,-15.8726922455904,
-320.858142212965)) ;
#39151=CARTESIAN_POINT('Ctrl Pts',(-10.1142193174863,-15.5695347426882,
-320.865539419656)) ;
#39152=CARTESIAN_POINT('Ctrl Pts',(-10.21090013687,-15.5063007504566,-320.867051066866)) ;
#39153=CARTESIAN_POINT('Ctrl Pts',(-10.3588927164377,-15.4075220565231,
-320.869361114072)) ;
#39154=CARTESIAN_POINT('Ctrl Pts',(-10.4106258646635,-15.3726140701835,
-320.870167884188)) ;
#39155=CARTESIAN_POINT('Ctrl Pts',(-10.5207642992943,-15.2974849800264,
-320.871883001329)) ;
#39156=CARTESIAN_POINT('Ctrl Pts',(-10.5791171598126,-15.2571887413449,
-320.872790182385)) ;
#39157=CARTESIAN_POINT('Ctrl Pts',(-10.7392647230928,-15.1452365128485,
-320.875277696229)) ;
#39158=CARTESIAN_POINT('Ctrl Pts',(-10.8405719181734,-15.0728894504592,
-320.876848790576)) ;
#39159=CARTESIAN_POINT('Ctrl Pts',(-11.0746688883295,-14.9021315115285,
-320.880481969504)) ;
#39160=CARTESIAN_POINT('Ctrl Pts',(-11.2068875054635,-14.8029553514131,
-320.882536128561)) ;
#39161=CARTESIAN_POINT('Ctrl Pts',(-11.7147673121994,-14.4112936035401,
-320.890465622905)) ;
#39162=CARTESIAN_POINT('Ctrl Pts',(-12.0804481929238,-14.1061663503894,
-320.896263772568)) ;
#39163=CARTESIAN_POINT('Ctrl Pts',(-12.7691943815611,-13.4850255795518,
-320.907653703306)) ;
#39164=CARTESIAN_POINT('Ctrl Pts',(-13.0932561961628,-13.1706067028363,
-320.913236594749)) ;
#39165=CARTESIAN_POINT('Ctrl Pts',(-13.5094977649877,-12.7361905631823,
-320.920815162566)) ;
#39166=CARTESIAN_POINT('Ctrl Pts',(-13.6121382787943,-12.6264314562078,
-320.922718684115)) ;
#39167=CARTESIAN_POINT('Ctrl Pts',(-13.7987412060125,-12.4219666194397,
-320.926246732688)) ;
#39168=CARTESIAN_POINT('Ctrl Pts',(-13.8830895089743,-12.3276250428531,
-320.927867763352)) ;
#39169=CARTESIAN_POINT('Ctrl Pts',(-14.0554439670209,-12.1308380541493,
-320.931236037986)) ;
#39170=CARTESIAN_POINT('Ctrl Pts',(-14.1433101269116,-12.0282798269091,
-320.932984350049)) ;
#39171=CARTESIAN_POINT('Ctrl Pts',(-14.3768963867407,-11.7495370575697,
-320.937717499267)) ;
#39172=CARTESIAN_POINT('Ctrl Pts',(-14.52049366311,-11.5716046537157,-320.940719451999)) ;
#39173=CARTESIAN_POINT('Ctrl Pts',(-14.7584589546418,-11.2653335884569,
-320.945850502904)) ;
#39174=CARTESIAN_POINT('Ctrl Pts',(-14.8545284322047,-11.1383498126716,
-320.947967639855)) ;
#39175=CARTESIAN_POINT('Ctrl Pts',(-15.2925576635272,-10.5436185440467,
-320.957827933863)) ;
#39176=CARTESIAN_POINT('Ctrl Pts',(-15.6141344513214,-10.0612630948273,
-320.965679462726)) ;
#39177=CARTESIAN_POINT('Ctrl Pts',(-16.0593527340625,-9.32055815677543,
-320.977261871365)) ;
#39178=CARTESIAN_POINT('Ctrl Pts',(-16.2004414701441,-9.07310924334838,
-320.981054400805)) ;
#39179=CARTESIAN_POINT('Ctrl Pts',(-16.3763494467086,-8.74739767941218,
-320.985905016079)) ;
#39180=CARTESIAN_POINT('Ctrl Pts',(-16.4163984030275,-8.67200385508084,
-320.98701810583)) ;
#39181=CARTESIAN_POINT('Ctrl Pts',(-16.4869525235056,-8.53694243767363,
-320.988993042143)) ;
#39182=CARTESIAN_POINT('Ctrl Pts',(-16.5176573349996,-8.47738083961355,
-320.989857372597)) ;
#39183=CARTESIAN_POINT('Ctrl Pts',(-16.5834625710932,-8.34801610146167,
-320.991719628829)) ;
#39184=CARTESIAN_POINT('Ctrl Pts',(-16.6184461286385,-8.27815510659376,
-320.992716116189)) ;
#39185=CARTESIAN_POINT('Ctrl Pts',(-16.725382220958,-8.06119737157336,-320.995785338825)) ;
#39186=CARTESIAN_POINT('Ctrl Pts',(-16.7958305233936,-7.91336784735064,
-320.997840706024)) ;
#39187=CARTESIAN_POINT('Ctrl Pts',(-17.0755732533782,-7.30578294797287,
-321.006175883769)) ;
#39188=CARTESIAN_POINT('Ctrl Pts',(-17.2680186484266,-6.83850865352852,
-321.012331461682)) ;
#39189=CARTESIAN_POINT('Ctrl Pts',(-17.6209186493473,-5.87134667026382,
-321.024952902675)) ;
#39190=CARTESIAN_POINT('Ctrl Pts',(-17.7797156257219,-5.37133097263386,
-321.031417134798)) ;
#39191=CARTESIAN_POINT('Ctrl Pts',(-17.9564959858786,-4.72030862886497,
-321.039914773461)) ;
#39192=CARTESIAN_POINT('Ctrl Pts',(-17.9940976357184,-4.57487834093764,
-321.041817545377)) ;
#39193=CARTESIAN_POINT('Ctrl Pts',(-18.060115854795,-4.30612653321886,-321.045344690236)) ;
#39194=CARTESIAN_POINT('Ctrl Pts',(-18.089044322004,-4.18293985991804,-321.046965574619)) ;
#39195=CARTESIAN_POINT('Ctrl Pts',(-18.1462453946832,-3.92766120838814,
-321.050334071567)) ;
#39196=CARTESIAN_POINT('Ctrl Pts',(-18.1743402529945,-3.79553695735537,
-321.052082757768)) ;
#39197=CARTESIAN_POINT('Ctrl Pts',(-18.2461312995022,-3.43882768235407,
-321.056818374293)) ;
#39198=CARTESIAN_POINT('Ctrl Pts',(-18.2871219915042,-3.21372248255536,
-321.059822452332)) ;
#39199=CARTESIAN_POINT('Ctrl Pts',(-18.3495933365787,-2.83060573415165,
-321.064957886123)) ;
#39200=CARTESIAN_POINT('Ctrl Pts',(-18.3732178716206,-2.67297014561105,
-321.067077274874)) ;
#39201=CARTESIAN_POINT('Ctrl Pts',(-18.4734767312523,-1.93968747265878,
-321.076957468502)) ;
#39202=CARTESIAN_POINT('Ctrl Pts',(-18.5251055740794,-1.36095235873069,
-321.08482709712)) ;
#39203=CARTESIAN_POINT('Ctrl Pts',(-18.5614233639371,-0.498095116336742,
-321.096400656331)) ;
#39204=CARTESIAN_POINT('Ctrl Pts',(-18.5668582310402,-0.215202318513333,
-321.100167539376)) ;
#39205=CARTESIAN_POINT('Ctrl Pts',(-18.5655150223184,0.153131570288138,
-321.104994104965)) ;
#39206=CARTESIAN_POINT('Ctrl Pts',(-18.5646138793491,0.238555778466489,
-321.10610797171)) ;
#39207=CARTESIAN_POINT('Ctrl Pts',(-18.561953678839,0.390981958181049,-321.108083839441)) ;
#39208=CARTESIAN_POINT('Ctrl Pts',(-18.5604213256749,0.457986375672511,
-321.108948331881)) ;
#39209=CARTESIAN_POINT('Ctrl Pts',(-18.5563179967306,0.603042485896432,
-321.110810279628)) ;
#39210=CARTESIAN_POINT('Ctrl Pts',(-18.5536173160079,0.68108909025185,-321.111806303374)) ;
#39211=CARTESIAN_POINT('Ctrl Pts',(-18.5437380350147,0.922507739674279,
-321.114872279359)) ;
#39212=CARTESIAN_POINT('Ctrl Pts',(-18.5348933346528,1.08580388235186,-321.116924915394)) ;
#39213=CARTESIAN_POINT('Ctrl Pts',(-18.4899344429207,1.75260852954898,-321.125253207177)) ;
#39214=CARTESIAN_POINT('Ctrl Pts',(-18.4354499703916,2.25466161129387,-321.131404653285)) ;
#39215=CARTESIAN_POINT('Ctrl Pts',(-18.289190299241,3.22980268418589,-321.143492840528)) ;
#39216=CARTESIAN_POINT('Ctrl Pts',(-18.1993277829494,3.70277925181585,-321.149421544324)) ;
#39217=CARTESIAN_POINT('Ctrl Pts',(-18.0495192505376,4.35244163217773,-321.157792661133)) ;
#39218=CARTESIAN_POINT('Ctrl Pts',(-18.005142355098,4.53252048579793,-321.16013692883)) ;
#39219=CARTESIAN_POINT('Ctrl Pts',(-17.9260112406139,4.83410610606355,-321.164108105024)) ;
#39220=CARTESIAN_POINT('Ctrl Pts',(-17.8927009317089,4.9559776188439,-321.165725341579)) ;
#39221=CARTESIAN_POINT('Ctrl Pts',(-17.8218560745214,5.20514712284266,-321.169058476106)) ;
#39222=CARTESIAN_POINT('Ctrl Pts',(-17.784195275679,5.33240178958517,-321.170775145127)) ;
#39223=CARTESIAN_POINT('Ctrl Pts',(-17.6818601151187,5.66504051473134,-321.17530072952)) ;
#39224=CARTESIAN_POINT('Ctrl Pts',(-17.6149715707018,5.86972209518751,-321.178124141604)) ;
#39225=CARTESIAN_POINT('Ctrl Pts',(-17.4551068272755,6.33154717228465,-321.184579309028)) ;
#39226=CARTESIAN_POINT('Ctrl Pts',(-17.3599799383985,6.58789344749354,-321.188223122735)) ;
#39227=CARTESIAN_POINT('Ctrl Pts',(-17.1300351161867,7.16793492925832,-321.19658526272)) ;
#39228=CARTESIAN_POINT('Ctrl Pts',(-16.991638893254,7.49010024141506,-321.201315486226)) ;
#39229=CARTESIAN_POINT('Ctrl Pts',(-16.8044953428927,7.8938172541963,-321.207304951171)) ;
#39230=CARTESIAN_POINT('Ctrl Pts',(-16.7641327838068,7.97917706199322,-321.208574806681)) ;
#39231=CARTESIAN_POINT('Ctrl Pts',(-16.5832880139387,8.35420241637968,-321.214164954287)) ;
#39232=CARTESIAN_POINT('Ctrl Pts',(-16.4359362982263,8.64049408939169,-321.218462686487)) ;
#39233=CARTESIAN_POINT('Ctrl Pts',(-16.2341665074723,9.00865809886574,-321.223968555225)) ;
#39234=CARTESIAN_POINT('Ctrl Pts',(-16.1864395314654,9.09413317855522,-321.225245240994)) ;
#39235=CARTESIAN_POINT('Ctrl Pts',(-16.1052113535417,9.23694079198204,-321.227373021199)) ;
#39236=CARTESIAN_POINT('Ctrl Pts',(-16.0720746156947,9.2944782273945,-321.228228787018)) ;
#39237=CARTESIAN_POINT('Ctrl Pts',(-15.9980579159046,9.42141868450193,-321.230112881591)) ;
#39238=CARTESIAN_POINT('Ctrl Pts',(-15.9570335957347,9.49073579644474,-321.231139338693)) ;
#39239=CARTESIAN_POINT('Ctrl Pts',(-15.8235754521061,9.71292293630367,-321.23442517731)) ;
#39240=CARTESIAN_POINT('Ctrl Pts',(-15.7293858203537,9.86472675585621,-321.236663557968)) ;
#39241=CARTESIAN_POINT('Ctrl Pts',(-15.4802493805616,10.2536131745221,-321.242407769472)) ;
#39242=CARTESIAN_POINT('Ctrl Pts',(-15.322042226032,10.4885521617144,-321.245888220912)) ;
#39243=CARTESIAN_POINT('Ctrl Pts',(-14.7484061869017,11.2997138451177,-321.258068049271)) ;
#39244=CARTESIAN_POINT('Ctrl Pts',(-14.3053465158289,11.8556348917969,-321.26673513444)) ;
#39245=CARTESIAN_POINT('Ctrl Pts',(-13.7278278157521,12.5006163989102,-321.277629083777)) ;
#39246=CARTESIAN_POINT('Ctrl Pts',(-13.6226752597952,12.6151252694939,-321.279596560882)) ;
#39247=CARTESIAN_POINT('Ctrl Pts',(-13.4294434693726,12.8203168242976,-321.283186288704)) ;
#39248=CARTESIAN_POINT('Ctrl Pts',(-13.34185249404,12.9114463692653,-321.284804208268)) ;
#39249=CARTESIAN_POINT('Ctrl Pts',(-13.1604694361469,13.0963403218624,-321.288136774294)) ;
#39250=CARTESIAN_POINT('Ctrl Pts',(-13.0665894825651,13.1900085230339,-321.289852171234)) ;
#39251=CARTESIAN_POINT('Ctrl Pts',(-12.818050527327,13.432729153268,-321.294369436931)) ;
#39252=CARTESIAN_POINT('Ctrl Pts',(-12.6617945910645,13.5801174261797,-321.297185700842)) ;
#39253=CARTESIAN_POINT('Ctrl Pts',(-12.3016498752988,13.9082029503217,-321.303620212185)) ;
#39254=CARTESIAN_POINT('Ctrl Pts',(-12.0962704588932,14.0871906191903,-321.30725039405)) ;
#39255=CARTESIAN_POINT('Ctrl Pts',(-11.6167417330582,14.486877439103,-321.315615916459)) ;
#39256=CARTESIAN_POINT('Ctrl Pts',(-11.3401061268932,14.7044312751157,-321.320363636395)) ;
#39257=CARTESIAN_POINT('Ctrl Pts',(-10.9892289722789,14.9645768324444,-321.326242966776)) ;
#39258=CARTESIAN_POINT('Ctrl Pts',(-10.9206553617482,15.0146927925513,-321.327385356424)) ;
#39259=CARTESIAN_POINT('Ctrl Pts',(-10.5822525014676,15.2584645616812,-321.332987034861)) ;
#39260=CARTESIAN_POINT('Ctrl Pts',(-10.3076035153886,15.4453267801448,-321.337423271941)) ;
#39261=CARTESIAN_POINT('Ctrl Pts',(-9.94570660781616,15.6775955487692,-321.343062809468)) ;
#39262=CARTESIAN_POINT('Ctrl Pts',(-9.86290627571715,15.7298176072214,-321.34433943979)) ;
#39263=CARTESIAN_POINT('Ctrl Pts',(-9.72325870829841,15.8163569751191,-321.346467158386)) ;
#39264=CARTESIAN_POINT('Ctrl Pts',(-9.66663345701099,15.8510285317965,-321.347322917376)) ;
#39265=CARTESIAN_POINT('Ctrl Pts',(-9.54090415520071,15.9270881016373,-321.349207035323)) ;
#39266=CARTESIAN_POINT('Ctrl Pts',(-9.47171442221973,15.9683315792215,-321.350233522206)) ;
#39267=CARTESIAN_POINT('Ctrl Pts',(-9.24820577598284,16.0995996058698,-321.353519583147)) ;
#39268=CARTESIAN_POINT('Ctrl Pts',(-9.09285493241683,16.1878475073278,-321.355758152445)) ;
#39269=CARTESIAN_POINT('Ctrl Pts',(-8.6879795962993,16.4101717484031,-321.361503033109)) ;
#39270=CARTESIAN_POINT('Ctrl Pts',(-8.43661703185502,16.540804688525,-321.364983958062)) ;
#39271=CARTESIAN_POINT('Ctrl Pts',(-7.54486101314455,16.9786321230456,-321.37716303195)) ;
#39272=CARTESIAN_POINT('Ctrl Pts',(-6.88992291155278,17.2547917500965,-321.385828929384)) ;
#39273=CARTESIAN_POINT('Ctrl Pts',(-6.07429430837448,17.5448459679738,-321.396721775595)) ;
#39274=CARTESIAN_POINT('Ctrl Pts',(-5.92715956189682,17.5950973518105,-321.398689430733)) ;
#39275=CARTESIAN_POINT('Ctrl Pts',(-5.65929210221363,17.6828416573478,-321.402279376305)) ;
#39276=CARTESIAN_POINT('Ctrl Pts',(-5.5387744512947,17.720960857171,-321.403897333695)) ;
#39277=CARTESIAN_POINT('Ctrl Pts',(-5.29104113258263,17.7965437085786,-321.407229868785)) ;
#39278=CARTESIAN_POINT('Ctrl Pts',(-5.16379438083837,17.8338810068994,-321.408945195831)) ;
#39279=CARTESIAN_POINT('Ctrl Pts',(-4.82945525785488,17.9281058998016,-321.413462004474)) ;
#39280=CARTESIAN_POINT('Ctrl Pts',(-4.62175697511332,17.9827690152042,-321.41627787565)) ;
#39281=CARTESIAN_POINT('Ctrl Pts',(-4.14862213822516,18.0985525240186,-321.422711252947)) ;
#39282=CARTESIAN_POINT('Ctrl Pts',(-3.88269480506963,18.1574598927173,-321.426340686715)) ;
#39283=CARTESIAN_POINT('Ctrl Pts',(-3.27037357511702,18.2790320529916,-321.434706385579)) ;
#39284=CARTESIAN_POINT('Ctrl Pts',(-2.92329988653985,18.3377390523937,-321.43945505655)) ;
#39285=CARTESIAN_POINT('Ctrl Pts',(-2.47944983952775,18.3998937950808,-321.445487636589)) ;
#39286=CARTESIAN_POINT('Ctrl Pts',(-2.38402901419855,18.4125003420151,-321.446782085803)) ;
#39287=CARTESIAN_POINT('Ctrl Pts',(-1.9694817469615,18.4639918020053,-321.452390556825)) ;
#39288=CARTESIAN_POINT('Ctrl Pts',(-1.64947290386272,18.495326206806,-321.456682025195)) ;
#39289=CARTESIAN_POINT('Ctrl Pts',(-1.23146410867236,18.5253210748946,-321.462177725154)) ;
#39290=CARTESIAN_POINT('Ctrl Pts',(-1.13406269647112,18.5315387008074,-321.463450448728)) ;
#39291=CARTESIAN_POINT('Ctrl Pts',(-0.97035751361738,18.5406933448562,-321.465573830478)) ;
#39292=CARTESIAN_POINT('Ctrl Pts',(-0.904078920903511,18.5440433765597,
-321.466429112353)) ;
#39293=CARTESIAN_POINT('Ctrl Pts',(-0.757146689066578,18.5506804151138,
-321.468314896735)) ;
#39294=CARTESIAN_POINT('Ctrl Pts',(-0.67648685661603,18.5537969302624,-321.469343497276)) ;
#39295=CARTESIAN_POINT('Ctrl Pts',(-0.416151820788321,18.5621557776636,
-321.472645376182)) ;
#39296=CARTESIAN_POINT('Ctrl Pts',(-0.236419828834445,18.5653148456518,
-321.474897371089)) ;
#39297=CARTESIAN_POINT('Ctrl Pts',(0.229379589953863,18.566736644263,-321.480690006208)) ;
#39298=CARTESIAN_POINT('Ctrl Pts',(0.51541169693746,18.5609987827475,-321.484204757496)) ;
#39299=CARTESIAN_POINT('Ctrl Pts',(1.50325343420382,18.5183296042975,-321.496325492573)) ;
#39300=CARTESIAN_POINT('Ctrl Pts',(2.20302263230478,18.4481704515664,-321.504902048803)) ;
#39301=CARTESIAN_POINT('Ctrl Pts',(3.06880127824176,18.3113944419386,-321.515928851407)) ;
#39302=CARTESIAN_POINT('Ctrl Pts',(3.24008794888846,18.2818636262046,-321.518129473395)) ;
#39303=CARTESIAN_POINT('Ctrl Pts',(3.53465837936602,18.2268080548199,-321.521950769586)) ;
#39304=CARTESIAN_POINT('Ctrl Pts',(3.65814378877568,18.2024263683139,-321.523563865548)) ;
#39305=CARTESIAN_POINT('Ctrl Pts',(3.91525216625968,18.1489393517034,-321.526946807155)) ;
#39306=CARTESIAN_POINT('Ctrl Pts',(4.0488207947935,18.1196095217521,-321.528718050772)) ;
#39307=CARTESIAN_POINT('Ctrl Pts',(4.41433246276992,18.0351048217017,-321.533603350425)) ;
#39308=CARTESIAN_POINT('Ctrl Pts',(4.64555551121885,17.9769338507959,-321.536736549811)) ;
#39309=CARTESIAN_POINT('Ctrl Pts',(5.18329146056139,17.8305827141844,-321.544117224469)) ;
#39310=CARTESIAN_POINT('Ctrl Pts',(5.48878005674475,17.7389256492352,-321.548383041199)) ;
#39311=CARTESIAN_POINT('Ctrl Pts',(6.18700467137919,17.5096697969373,-321.558259792365)) ;
#39312=CARTESIAN_POINT('Ctrl Pts',(6.57778003876474,17.3666454107648,-321.563883117522)) ;
#39313=CARTESIAN_POINT('Ctrl Pts',(7.1783313263465,17.1236621798088,-321.572560240795)) ;
#39314=CARTESIAN_POINT('Ctrl Pts',(7.39159534272431,17.0326910873819,-321.57564802626)) ;
#39315=CARTESIAN_POINT('Ctrl Pts',(7.70704648244808,16.8910898400069,-321.580198713579)) ;
#39316=CARTESIAN_POINT('Ctrl Pts',(7.81056150998061,16.8434738229718,-321.581689251149)) ;
#39317=CARTESIAN_POINT('Ctrl Pts',(7.96984644043119,16.7684199857695,-321.583974871216)) ;
#39318=CARTESIAN_POINT('Ctrl Pts',(8.02592783070173,16.7416499656676,-321.584778055086)) ;
#39319=CARTESIAN_POINT('Ctrl Pts',(8.1460699349838,16.6835586328574,-321.586494506742)) ;
#39320=CARTESIAN_POINT('Ctrl Pts',(8.21008676528212,16.6521487912436,-321.587406537155)) ;
#39321=CARTESIAN_POINT('Ctrl Pts',(8.38714961336141,16.5640037044952,-321.589923971845)) ;
#39322=CARTESIAN_POINT('Ctrl Pts',(8.49979930678429,16.5064808237003,-321.591519774152)) ;
#39323=CARTESIAN_POINT('Ctrl Pts',(8.76158902219487,16.3694112537705,-321.595223619239)) ;
#39324=CARTESIAN_POINT('Ctrl Pts',(8.91024814132779,16.2889700465853,-321.597323308824)) ;
#39325=CARTESIAN_POINT('Ctrl Pts',(9.49496724126799,15.9621716341102,-321.605601170565)) ;
#39326=CARTESIAN_POINT('Ctrl Pts',(9.9220808266281,15.7002432949059,-321.611696171592)) ;
#39327=CARTESIAN_POINT('Ctrl Pts',(10.6425686314715,15.2172471239336,-321.622359435912)) ;
#39328=CARTESIAN_POINT('Ctrl Pts',(10.940943343888,15.0041539286127,-321.626895188228)) ;
#39329=CARTESIAN_POINT('Ctrl Pts',(11.3838681358433,14.6675846174657,-321.633875264549)) ;
#39330=CARTESIAN_POINT('Ctrl Pts',(11.5331545986901,14.5504926748882,-321.63627205675)) ;
#39331=CARTESIAN_POINT('Ctrl Pts',(11.7793503444038,14.3512208042749,-321.640304590439)) ;
#39332=CARTESIAN_POINT('Ctrl Pts',(11.8772578456402,14.2702970930319,-321.641929927098)) ;
#39333=CARTESIAN_POINT('Ctrl Pts',(12.0749565108811,14.1034486366182,-321.645257421477)) ;
#39334=CARTESIAN_POINT('Ctrl Pts',(12.1746794456967,14.0174540669482,-321.64696011822)) ;
#39335=CARTESIAN_POINT('Ctrl Pts',(12.4306400744634,13.7919382128315,-321.65139430076)) ;
#39336=CARTESIAN_POINT('Ctrl Pts',(12.5854463507763,13.6508209366875,-321.65413918112)) ;
#39337=CARTESIAN_POINT('Ctrl Pts',(12.8395504368079,13.4111890772959,-321.658749183073)) ;
#39338=CARTESIAN_POINT('Ctrl Pts',(12.940182484306,13.3141175111215,-321.660603172423)) ;
#39339=CARTESIAN_POINT('Ctrl Pts',(13.360660962612,12.8992453488769,-321.668466314579)) ;
#39340=CARTESIAN_POINT('Ctrl Pts',(13.6699708490437,12.5709859454001,-321.674544424176)) ;
#39341=CARTESIAN_POINT('Ctrl Pts',(14.247254545063,11.9118075164964,-321.686345206954)) ;
#39342=CARTESIAN_POINT('Ctrl Pts',(14.516407656839,11.5822851858498,-321.69206437684)) ;
#39343=CARTESIAN_POINT('Ctrl Pts',(14.8440660071315,11.1517526354932,-321.699187274537)) ;
#39344=CARTESIAN_POINT('Ctrl Pts',(14.9132647878151,11.0590422686061,-321.700701112628)) ;
#39345=CARTESIAN_POINT('Ctrl Pts',(15.0184697109015,10.9153087564481,-321.703013697433)) ;
#39346=CARTESIAN_POINT('Ctrl Pts',(15.0550924459194,10.8647406394531,-321.703820842318)) ;
#39347=CARTESIAN_POINT('Ctrl Pts',(15.1327412416412,10.7563778806971,-321.705535843599)) ;
#39348=CARTESIAN_POINT('Ctrl Pts',(15.1736928621663,10.6985310925191,-321.706442541296)) ;
#39349=CARTESIAN_POINT('Ctrl Pts',(15.2855419383057,10.538603027454,-321.708927064982)) ;
#39350=CARTESIAN_POINT('Ctrl Pts',(15.3557472153486,10.4360420491688,-321.710495688647)) ;
#39351=CARTESIAN_POINT('Ctrl Pts',(15.5166920065175,10.195781518194,-321.714121827195)) ;
#39352=CARTESIAN_POINT('Ctrl Pts',(15.606637338683,10.0575624627969,-321.716171458557)) ;
#39353=CARTESIAN_POINT('Ctrl Pts',(15.947789220838,9.51771589421415,-321.724067305245)) ;
#39354=CARTESIAN_POINT('Ctrl Pts',(16.1854305052835,9.10772953941646,-321.729836908404)) ;
#39355=CARTESIAN_POINT('Ctrl Pts',(16.619558332862,8.28799113082099,-321.741227460931)) ;
#39356=CARTESIAN_POINT('Ctrl Pts',(16.8172038827703,7.87922384643061,-321.74684060395)) ;
#39357=CARTESIAN_POINT('Ctrl Pts',(17.0601641895699,7.32584067329485,-321.754453178995)) ;
#39358=CARTESIAN_POINT('Ctrl Pts',(17.1189807615024,7.18732504816598,-321.756359315207)) ;
#39359=CARTESIAN_POINT('Ctrl Pts',(17.2241639269202,6.93099571682241,-321.759890517585)) ;
#39360=CARTESIAN_POINT('Ctrl Pts',(17.2710218928518,6.81339323178998,-321.761512060175)) ;
#39361=CARTESIAN_POINT('Ctrl Pts',(17.3653397988709,6.56945087033152,-321.764879568934)) ;
#39362=CARTESIAN_POINT('Ctrl Pts',(17.4126323144763,6.4430541580304,-321.766626583935)) ;
#39363=CARTESIAN_POINT('Ctrl Pts',(17.536135750312,6.10167707020369,-321.771351182546)) ;
#39364=CARTESIAN_POINT('Ctrl Pts',(17.6097700097935,5.88578966891215,-321.774345770545)) ;
#39365=CARTESIAN_POINT('Ctrl Pts',(17.7278471320026,5.51752708258251,-321.779461643665)) ;
#39366=CARTESIAN_POINT('Ctrl Pts',(17.7743478961441,5.36583878138583,-321.781570987735)) ;
#39367=CARTESIAN_POINT('Ctrl Pts',(17.980342379388,4.66179289272225,-321.791362889235)) ;
#39368=CARTESIAN_POINT('Ctrl Pts',(18.1160691307113,4.10281149643404,-321.799152294138)) ;
#39369=CARTESIAN_POINT('Ctrl Pts',(18.2810278126606,3.25314908045536,-321.810755460361)) ;
#39370=CARTESIAN_POINT('Ctrl Pts',(18.329709487072,2.96659865032559,-321.814626626024)) ;
#39371=CARTESIAN_POINT('Ctrl Pts',(18.3839772162613,2.59445281438515,-321.819554738078)) ;
#39372=CARTESIAN_POINT('Ctrl Pts',(18.3957255439917,2.50979788652768,-321.820669101697)) ;
#39373=CARTESIAN_POINT('Ctrl Pts',(18.4156441742154,2.35861016756145,-321.822645565276)) ;
#39374=CARTESIAN_POINT('Ctrl Pts',(18.4240394792799,2.29210854448195,-321.823510161527)) ;
#39375=CARTESIAN_POINT('Ctrl Pts',(18.4414328394865,2.14805701475749,-321.825371913067)) ;
#39376=CARTESIAN_POINT('Ctrl Pts',(18.4503022430775,2.07049300244084,-321.826367641172)) ;
#39377=CARTESIAN_POINT('Ctrl Pts',(18.4762201475247,1.83043264255559,-321.82943154835)) ;
#39378=CARTESIAN_POINT('Ctrl Pts',(18.4916130632767,1.66776529323097,-321.831482444235)) ;
#39379=CARTESIAN_POINT('Ctrl Pts',(18.5457559521328,1.00200950645863,-321.839806348449)) ;
#39380=CARTESIAN_POINT('Ctrl Pts',(18.5661369063153,0.497643941982251,-321.845955161873)) ;
#39381=CARTESIAN_POINT('Ctrl Pts',(18.5658389860298,-0.30109714749415,-321.855747028671)) ;
#39382=CARTESIAN_POINT('Ctrl Pts',(18.558737673329,-0.595198509947113,-321.859362734055)) ;
#39383=CARTESIAN_POINT('Ctrl Pts',(18.5446545931659,-0.888979990027978,
-321.863010318849)) ;
#39384=CARTESIAN_POINT('Origin',(0.,0.,-315.477129595899)) ;
#39385=CARTESIAN_POINT('',(18.5446550725491,-0.888969989752756,-323.660107772569)) ;
#39386=CARTESIAN_POINT('',(18.5446545937424,-0.888979978001647,-323.364389984898)) ;
#39387=CARTESIAN_POINT('',(18.544654593745,-0.888979977948782,-315.477129595899)) ;
#39388=CARTESIAN_POINT('Ctrl Pts',(18.5446545937669,-0.88897997749115,-323.660107898464)) ;
#39389=CARTESIAN_POINT('Ctrl Pts',(18.5503237782399,-0.770717395047024,
-323.658617203796)) ;
#39390=CARTESIAN_POINT('Ctrl Pts',(18.5548612046501,-0.652413378015465,
-323.65712004335)) ;
#39391=CARTESIAN_POINT('Ctrl Pts',(18.561366413947,-0.426362988663961,-323.654246572906)) ;
#39392=CARTESIAN_POINT('Ctrl Pts',(18.5635281938753,-0.318636961806443,
-323.652871671419)) ;
#39393=CARTESIAN_POINT('Ctrl Pts',(18.5661081922414,-0.091527361846506,
-323.649960657052)) ;
#39394=CARTESIAN_POINT('Ctrl Pts',(18.566312902283,0.0278537801060046,-323.648423229591)) ;
#39395=CARTESIAN_POINT('Ctrl Pts',(18.5640988187805,0.307047520700836,-323.644810180929)) ;
#39396=CARTESIAN_POINT('Ctrl Pts',(18.5607677730369,0.466843337428206,-323.642728813943)) ;
#39397=CARTESIAN_POINT('Ctrl Pts',(18.5412689196309,1.04428087719617,-323.635159590194)) ;
#39398=CARTESIAN_POINT('Ctrl Pts',(18.5130633804492,1.46138917679022,-323.629598320572)) ;
#39399=CARTESIAN_POINT('Ctrl Pts',(18.422992305004,2.34765365123846,-323.617647715205)) ;
#39400=CARTESIAN_POINT('Ctrl Pts',(18.357221770728,2.81611993049503,-323.611249064971)) ;
#39401=CARTESIAN_POINT('Ctrl Pts',(18.2715782248556,3.29303270247428,-323.604758360695)) ;
#39402=CARTESIAN_POINT('Ctrl Pts',(18.2695076501888,3.30450078322009,-323.60460229901)) ;
#39403=CARTESIAN_POINT('Ctrl Pts',(18.2197144195942,3.57880815554623,-323.600869883175)) ;
#39404=CARTESIAN_POINT('Ctrl Pts',(18.1663351722883,3.84058957172962,-323.597317434124)) ;
#39405=CARTESIAN_POINT('Ctrl Pts',(18.0913798123934,4.17153293123352,-323.592873557643)) ;
#39406=CARTESIAN_POINT('Ctrl Pts',(18.0750233309047,4.24184418810534,-323.591932178512)) ;
#39407=CARTESIAN_POINT('Ctrl Pts',(18.0441972742068,4.37093911678392,-323.590209957139)) ;
#39408=CARTESIAN_POINT('Ctrl Pts',(18.0298494527621,4.42975086872242,-323.589427739595)) ;
#39409=CARTESIAN_POINT('Ctrl Pts',(18.0000796385871,4.54923635417858,-323.587844139034)) ;
#39410=CARTESIAN_POINT('Ctrl Pts',(17.9846378925075,4.60990436874624,-323.58704300336)) ;
#39411=CARTESIAN_POINT('Ctrl Pts',(17.9395429453599,4.78339913642182,-323.584758949733)) ;
#39412=CARTESIAN_POINT('Ctrl Pts',(17.909132764943,4.89602614968282,-323.583284690565)) ;
#39413=CARTESIAN_POINT('Ctrl Pts',(17.7172790410817,5.58086046772953,-323.57435363134)) ;
#39414=CARTESIAN_POINT('Ctrl Pts',(17.5294870144372,6.14532911905883,-323.567122913388)) ;
#39415=CARTESIAN_POINT('Ctrl Pts',(17.1901185608794,7.02238975020227,-323.555591254465)) ;
#39416=CARTESIAN_POINT('Ctrl Pts',(17.0563116952428,7.34141436204539,-323.551334665066)) ;
#39417=CARTESIAN_POINT('Ctrl Pts',(16.8390438163416,7.82137136039368,-323.544775161069)) ;
#39418=CARTESIAN_POINT('Ctrl Pts',(16.7620097359234,7.98512843289862,-323.542509092296)) ;
#39419=CARTESIAN_POINT('Ctrl Pts',(16.6127772081841,8.290684064121,-323.538220959871)) ;
#39420=CARTESIAN_POINT('Ctrl Pts',(16.541125858467,8.43273170762426,-323.536202706452)) ;
#39421=CARTESIAN_POINT('Ctrl Pts',(16.4221170690771,8.66131024987194,-323.532912066623)) ;
#39422=CARTESIAN_POINT('Ctrl Pts',(16.3758801693497,8.7484154524514,-323.531647856911)) ;
#39423=CARTESIAN_POINT('Ctrl Pts',(16.2798652188715,8.92586844555025,-323.529050918605)) ;
#39424=CARTESIAN_POINT('Ctrl Pts',(16.2300237703544,9.01617809475384,-323.527717756314)) ;
#39425=CARTESIAN_POINT('Ctrl Pts',(16.0895683212822,9.26573581046243,-323.524001354571)) ;
#39426=CARTESIAN_POINT('Ctrl Pts',(15.9973457769208,9.42406477107794,-323.521606448748)) ;
#39427=CARTESIAN_POINT('Ctrl Pts',(15.6224760716144,10.0462831714071,-323.512049008671)) ;
#39428=CARTESIAN_POINT('Ctrl Pts',(15.3218733435263,10.4990360548116,-323.504760435583)) ;
#39429=CARTESIAN_POINT('Ctrl Pts',(14.781351998349,11.2403833148442,-323.492403407264)) ;
#39430=CARTESIAN_POINT('Ctrl Pts',(14.5517543468974,11.5360751423254,-323.487354655104)) ;
#39431=CARTESIAN_POINT('Ctrl Pts',(14.2196282772862,11.9381044320937,-323.48040369684)) ;
#39432=CARTESIAN_POINT('Ctrl Pts',(14.1245336638935,12.0504653290566,-323.478451423275)) ;
#39433=CARTESIAN_POINT('Ctrl Pts',(14.0242961654838,12.1660860762444,-323.476437285097)) ;
#39434=CARTESIAN_POINT('Ctrl Pts',(14.0204773592986,12.1704867597478,-323.47636061636)) ;
#39435=CARTESIAN_POINT('Ctrl Pts',(14.0138723901079,12.1780909037963,-323.476228123801)) ;
#39436=CARTESIAN_POINT('Ctrl Pts',(14.0110871988395,12.181295207566,-323.476172288845)) ;
#39437=CARTESIAN_POINT('Ctrl Pts',(14.0062743418172,12.186828463538,-323.476075865169)) ;
#39438=CARTESIAN_POINT('Ctrl Pts',(14.0042471937814,12.1891578656366,-323.476035270451)) ;
#39439=CARTESIAN_POINT('Ctrl Pts',(14.0007462905928,12.1931787382118,-323.475965194816)) ;
#39440=CARTESIAN_POINT('Ctrl Pts',(13.9992728101978,12.1948704470848,-323.475935710701)) ;
#39441=CARTESIAN_POINT('Ctrl Pts',(13.9936473911845,12.2013266505203,-323.475823184108)) ;
#39442=CARTESIAN_POINT('Ctrl Pts',(13.9894933263703,12.2060892923554,-323.47574016663)) ;
#39443=CARTESIAN_POINT('Ctrl Pts',(13.9816334202048,12.2150914041549,-323.475583236027)) ;
#39444=CARTESIAN_POINT('Ctrl Pts',(13.9779280804049,12.2193313109958,-323.475509316927)) ;
#39445=CARTESIAN_POINT('Ctrl Pts',(13.9709152486981,12.2273485156703,-323.475369532489)) ;
#39446=CARTESIAN_POINT('Ctrl Pts',(13.9676081523547,12.2311261587905,-323.47530366237)) ;
#39447=CARTESIAN_POINT('Ctrl Pts',(13.9613468872955,12.2382724503911,-323.475179044985)) ;
#39448=CARTESIAN_POINT('Ctrl Pts',(13.9583930307397,12.2416413718422,-323.475120293897)) ;
#39449=CARTESIAN_POINT('Ctrl Pts',(13.9527983324012,12.2480175585899,-323.475009092014)) ;
#39450=CARTESIAN_POINT('Ctrl Pts',(13.9501577371959,12.2510250398708,-323.474956638165)) ;
#39451=CARTESIAN_POINT('Ctrl Pts',(13.9451541953384,12.2567200619548,-323.474857305444)) ;
#39452=CARTESIAN_POINT('Ctrl Pts',(13.9427914437388,12.2594077738402,-323.474810424133)) ;
#39453=CARTESIAN_POINT('Ctrl Pts',(13.9383123154742,12.2644999677681,-323.474721597863)) ;
#39454=CARTESIAN_POINT('Ctrl Pts',(13.9361960933454,12.2669045855467,-323.474679650954)) ;
#39455=CARTESIAN_POINT('Ctrl Pts',(13.932182408608,12.2714628701886,-323.474600131711)) ;
#39456=CARTESIAN_POINT('Ctrl Pts',(13.9302850686952,12.2736166449027,-323.474562557818)) ;
#39457=CARTESIAN_POINT('Ctrl Pts',(13.9266847846417,12.2777016147674,-323.474491290651)) ;
#39458=CARTESIAN_POINT('Ctrl Pts',(13.9249819380804,12.2796328958226,-323.474457596128)) ;
#39459=CARTESIAN_POINT('Ctrl Pts',(13.9217491544514,12.2832978157025,-323.474393653399)) ;
#39460=CARTESIAN_POINT('Ctrl Pts',(13.9202192951733,12.285031523077,-323.474363404191)) ;
#39461=CARTESIAN_POINT('Ctrl Pts',(13.9173135374517,12.2883232226044,-323.474305970111)) ;
#39462=CARTESIAN_POINT('Ctrl Pts',(13.9159377011823,12.2898812695546,-323.474278784434)) ;
#39463=CARTESIAN_POINT('Ctrl Pts',(13.9133232730959,12.2928409409497,-323.47422714125)) ;
#39464=CARTESIAN_POINT('Ctrl Pts',(13.9120847310595,12.2942426093266,-323.474202683095)) ;
#39465=CARTESIAN_POINT('Ctrl Pts',(13.909730135176,12.2969065137494,-323.47415619885)) ;
#39466=CARTESIAN_POINT('Ctrl Pts',(13.908614121282,12.2981687850912,-323.474134172236)) ;
#39467=CARTESIAN_POINT('Ctrl Pts',(13.9064915446121,12.3005688742403,-323.474092289978)) ;
#39468=CARTESIAN_POINT('Ctrl Pts',(13.9054850139649,12.3017067204797,-323.474072433909)) ;
#39469=CARTESIAN_POINT('Ctrl Pts',(13.9035698736828,12.3038711814465,-323.474034662232)) ;
#39470=CARTESIAN_POINT('Ctrl Pts',(13.9026612899867,12.3048978190765,-323.474016746282)) ;
#39471=CARTESIAN_POINT('Ctrl Pts',(13.9009318343427,12.3068515499615,-323.473982651062)) ;
#39472=CARTESIAN_POINT('Ctrl Pts',(13.9001109833619,12.3077786617267,-323.473966471517)) ;
#39473=CARTESIAN_POINT('Ctrl Pts',(13.8985479419105,12.3095436861754,-323.473935668705)) ;
#39474=CARTESIAN_POINT('Ctrl Pts',(13.8978057684013,12.3103816138752,-323.473921045214)) ;
#39475=CARTESIAN_POINT('Ctrl Pts',(13.8540989812646,12.3597183995863,-323.473060011453)) ;
#39476=CARTESIAN_POINT('Ctrl Pts',(13.8108808228006,12.4079921184024,-323.472216985576)) ;
#39477=CARTESIAN_POINT('Ctrl Pts',(13.7360751665116,12.4906733167759,-323.470772915351)) ;
#39478=CARTESIAN_POINT('Ctrl Pts',(13.704608901706,12.5251896490504,-323.470170018341)) ;
#39479=CARTESIAN_POINT('Ctrl Pts',(13.6307253300317,12.6056231077138,-323.46876537125)) ;
#39480=CARTESIAN_POINT('Ctrl Pts',(13.5882056947003,12.6514454892282,-323.467965357299)) ;
#39481=CARTESIAN_POINT('Ctrl Pts',(13.466041493772,12.7817725683267,-323.465689159943)) ;
#39482=CARTESIAN_POINT('Ctrl Pts',(13.3858343857396,12.8657460475946,-323.464221541928)) ;
#39483=CARTESIAN_POINT('Ctrl Pts',(13.0244927551137,13.2370186190326,-323.457714876407)) ;
#39484=CARTESIAN_POINT('Ctrl Pts',(12.7348591372855,13.5158957433074,-323.452776803151)) ;
#39485=CARTESIAN_POINT('Ctrl Pts',(12.0905261872447,14.0971866565799,-323.442141515355)) ;
#39486=CARTESIAN_POINT('Ctrl Pts',(11.7330294212639,14.3960937573776,-323.436450574123)) ;
#39487=CARTESIAN_POINT('Ctrl Pts',(11.1289644631762,14.8636973247729,-323.426981665765)) ;
#39488=CARTESIAN_POINT('Ctrl Pts',(10.8888987088302,15.0404532029573,-323.423255361437)) ;
#39489=CARTESIAN_POINT('Ctrl Pts',(10.52479627491,15.2952467673429,-323.417632604116)) ;
#39490=CARTESIAN_POINT('Ctrl Pts',(10.4039228921554,15.3777208544005,-323.415770722326)) ;
#39491=CARTESIAN_POINT('Ctrl Pts',(10.1787687630971,15.527477679217,-323.412309258019)) ;
#39492=CARTESIAN_POINT('Ctrl Pts',(10.074763943415,15.5951604045832,-323.410712915426)) ;
#39493=CARTESIAN_POINT('Ctrl Pts',(9.83822275615837,15.7457393468884,-323.407087450815)) ;
#39494=CARTESIAN_POINT('Ctrl Pts',(9.70530222750609,15.82801450442,-323.405053743867)) ;
#39495=CARTESIAN_POINT('Ctrl Pts',(9.27689476108783,16.0857644782117,-323.398510654345)) ;
#39496=CARTESIAN_POINT('Ctrl Pts',(8.9775694101289,16.2547175245648,-323.393955252391)) ;
#39497=CARTESIAN_POINT('Ctrl Pts',(8.07239186473413,16.7330079504755,-323.380269995338)) ;
#39498=CARTESIAN_POINT('Ctrl Pts',(7.45405168113789,17.0174667866865,-323.371022501614)) ;
#39499=CARTESIAN_POINT('Ctrl Pts',(6.64783929924503,17.3359625597361,-323.359494607043)) ;
#39500=CARTESIAN_POINT('Ctrl Pts',(6.47315036202161,17.4019450013065,-323.357028879074)) ;
#39501=CARTESIAN_POINT('Ctrl Pts',(6.22056076950735,17.4930217983991,-323.353523718497)) ;
#39502=CARTESIAN_POINT('Ctrl Pts',(6.14344330860009,17.5202537728642,-323.352461562311)) ;
#39503=CARTESIAN_POINT('Ctrl Pts',(6.00360291696061,17.5685978633952,-323.350551584627)) ;
#39504=CARTESIAN_POINT('Ctrl Pts',(5.94094243979778,17.5898857811635,-323.349701717918)) ;
#39505=CARTESIAN_POINT('Ctrl Pts',(5.78724335727805,17.6411876684146,-323.347630981698)) ;
#39506=CARTESIAN_POINT('Ctrl Pts',(5.69608356481473,17.6708324673515,-323.346414513763)) ;
#39507=CARTESIAN_POINT('Ctrl Pts',(5.31273200211769,17.7922221699779,-323.341340690626)) ;
#39508=CARTESIAN_POINT('Ctrl Pts',(5.0185222094316,17.877436245743,-323.337547327287)) ;
#39509=CARTESIAN_POINT('Ctrl Pts',(4.6345425293482,17.9784247466082,-323.332661395469)) ;
#39510=CARTESIAN_POINT('Ctrl Pts',(4.5465777818002,18.0008714041265,-323.331546523555)) ;
#39511=CARTESIAN_POINT('Ctrl Pts',(3.97621646159951,18.1419674929887,-323.32433902006)) ;
#39512=CARTESIAN_POINT('Ctrl Pts',(3.48938698789912,18.2418601110935,-323.318279418466)) ;
#39513=CARTESIAN_POINT('Ctrl Pts',(2.69512740539551,18.3718721803915,-323.30831136477)) ;
#39514=CARTESIAN_POINT('Ctrl Pts',(2.38992447485823,18.4140614628864,-323.304463191795)) ;
#39515=CARTESIAN_POINT('Ctrl Pts',(1.93698773644386,18.4652216581462,-323.298698053594)) ;
#39516=CARTESIAN_POINT('Ctrl Pts',(1.78996894540428,18.4800525829168,-323.296818509563)) ;
#39517=CARTESIAN_POINT('Ctrl Pts',(1.51926957527869,18.5040994590875,-323.293340600501)) ;
#39518=CARTESIAN_POINT('Ctrl Pts',(1.39564348538494,18.513834180013,-323.291745706158)) ;
#39519=CARTESIAN_POINT('Ctrl Pts',(1.11775912275271,18.5329165125479,-323.288145293981)) ;
#39520=CARTESIAN_POINT('Ctrl Pts',(0.963462987689927,18.5415781122223,-323.286135464969)) ;
#39521=CARTESIAN_POINT('Ctrl Pts',(0.481379714385811,18.5626065716895,-323.279822824562)) ;
#39522=CARTESIAN_POINT('Ctrl Pts',(0.153362038502939,18.5682139266589,-323.275478842516)) ;
#39523=CARTESIAN_POINT('Ctrl Pts',(-0.23657036804274,18.564546067458,-323.27027123668)) ;
#39524=CARTESIAN_POINT('Ctrl Pts',(-0.298506436942952,18.5636534694313,
-323.269442804479)) ;
#39525=CARTESIAN_POINT('Ctrl Pts',(-0.512279398028653,18.559502527546,-323.266579577389)) ;
#39526=CARTESIAN_POINT('Ctrl Pts',(-0.664079970053959,18.5546911050701,
-323.264539580786)) ;
#39527=CARTESIAN_POINT('Ctrl Pts',(-1.24790198818545,18.5290126458142,-323.256677432499)) ;
#39528=CARTESIAN_POINT('Ctrl Pts',(-1.67920354976889,18.4949140176799,-323.250831618158)) ;
#39529=CARTESIAN_POINT('Ctrl Pts',(-2.26598784024006,18.427826551131,-323.242947929109)) ;
#39530=CARTESIAN_POINT('Ctrl Pts',(-2.42282042162764,18.4078633633876,-323.240848056056)) ;
#39531=CARTESIAN_POINT('Ctrl Pts',(-2.69880563117029,18.3691450808065,-323.23717564102)) ;
#39532=CARTESIAN_POINT('Ctrl Pts',(-2.81806633368682,18.351227344344,-323.235596253059)) ;
#39533=CARTESIAN_POINT('Ctrl Pts',(-3.00641745702622,18.3210500642899,-323.233118293633)) ;
#39534=CARTESIAN_POINT('Ctrl Pts',(-3.07562743877243,18.3095586312135,-323.232211284222)) ;
#39535=CARTESIAN_POINT('Ctrl Pts',(-3.21593039487008,18.285445151023,-323.230380915386)) ;
#39536=CARTESIAN_POINT('Ctrl Pts',(-3.28701818942103,18.272800117011,-323.229457814163)) ;
#39537=CARTESIAN_POINT('Ctrl Pts',(-3.48694629915977,18.2360326352666,-323.226871670499)) ;
#39538=CARTESIAN_POINT('Ctrl Pts',(-3.61560762441776,18.2109599516676,-323.225219085501)) ;
#39539=CARTESIAN_POINT('Ctrl Pts',(-4.13173325787617,18.1046953976303,-323.218619682922)) ;
#39540=CARTESIAN_POINT('Ctrl Pts',(-4.51682215079011,18.0124827318817,-323.213761822793)) ;
#39541=CARTESIAN_POINT('Ctrl Pts',(-5.33492586574961,17.7886937945559,-323.203370040131)) ;
#39542=CARTESIAN_POINT('Ctrl Pts',(-5.76667659037494,17.653455800313,-323.197840623271)) ;
#39543=CARTESIAN_POINT('Ctrl Pts',(-6.46969411556895,17.404702445927,-323.188593351146)) ;
#39544=CARTESIAN_POINT('Ctrl Pts',(-6.7439717006612,17.3002732451864,-323.184923609616)) ;
#39545=CARTESIAN_POINT('Ctrl Pts',(-7.1505012689632,17.1343527003912,-323.179367104328)) ;
#39546=CARTESIAN_POINT('Ctrl Pts',(-7.28469189153641,17.077733304651,-323.177513626326)) ;
#39547=CARTESIAN_POINT('Ctrl Pts',(-7.53199853149051,16.9699412855552,-323.17405982061)) ;
#39548=CARTESIAN_POINT('Ctrl Pts',(-7.64529435365952,16.9192016155736,-323.172462622079)) ;
#39549=CARTESIAN_POINT('Ctrl Pts',(-7.90090977777712,16.8016321431667,-323.168824345505)) ;
#39550=CARTESIAN_POINT('Ctrl Pts',(-8.0429064189153,16.7341230491819,-323.166778544015)) ;
#39551=CARTESIAN_POINT('Ctrl Pts',(-8.50892601176434,16.5052626206335,-323.159982705293)) ;
#39552=CARTESIAN_POINT('Ctrl Pts',(-8.82908736682221,16.3362398129791,-323.155180387365)) ;
#39553=CARTESIAN_POINT('Ctrl Pts',(-9.63713570586959,15.8789498201472,-323.142757609997)) ;
#39554=CARTESIAN_POINT('Ctrl Pts',(-10.1171392499201,15.5775134037096,-323.135078592906)) ;
#39555=CARTESIAN_POINT('Ctrl Pts',(-10.7287977375206,15.1531863211195,-323.125119544532)) ;
#39556=CARTESIAN_POINT('Ctrl Pts',(-10.8735232091636,15.0496727451883,-323.122750605868)) ;
#39557=CARTESIAN_POINT('Ctrl Pts',(-11.1223052625073,14.8662714180601,-323.118670260359)) ;
#39558=CARTESIAN_POINT('Ctrl Pts',(-11.227044548546,14.7873314367539,-323.116949847738)) ;
#39559=CARTESIAN_POINT('Ctrl Pts',(-11.3881467606397,14.6632134305196,-323.114305175881)) ;
#39560=CARTESIAN_POINT('Ctrl Pts',(-11.4450972070057,14.6188051731731,-323.113370580112)) ;
#39561=CARTESIAN_POINT('Ctrl Pts',(-11.5501401343129,14.5359057672667,-323.111648507283)) ;
#39562=CARTESIAN_POINT('Ctrl Pts',(-11.5983029280691,14.497505398825,-323.110859657134)) ;
#39563=CARTESIAN_POINT('Ctrl Pts',(-11.7324132664571,14.3894827014484,-323.108663840561)) ;
#39564=CARTESIAN_POINT('Ctrl Pts',(-11.8179311487339,14.3193308813554,-323.107264496208)) ;
#39565=CARTESIAN_POINT('Ctrl Pts',(-12.3201680291789,13.8997731928975,-323.099036020632)) ;
#39566=CARTESIAN_POINT('Ctrl Pts',(-12.7220004765878,13.5329576500112,-323.092402328526)) ;
#39567=CARTESIAN_POINT('Ctrl Pts',(-13.4380222292776,12.8192165239113,-323.080016702163)) ;
#39568=CARTESIAN_POINT('Ctrl Pts',(-13.7563256812105,12.4770291562704,-323.074277882653)) ;
#39569=CARTESIAN_POINT('Ctrl Pts',(-14.2032359513814,11.9586697063806,-323.065723070661)) ;
#39570=CARTESIAN_POINT('Ctrl Pts',(-14.3421905196898,11.7916607606686,-323.062987450998)) ;
#39571=CARTESIAN_POINT('Ctrl Pts',(-14.5614682099217,11.5185000776005,-323.058537357585)) ;
#39572=CARTESIAN_POINT('Ctrl Pts',(-14.6436366290522,11.4138559076622,-323.056838216513)) ;
#39573=CARTESIAN_POINT('Ctrl Pts',(-14.8015025965645,11.2082974226561,-323.053510081082)) ;
#39574=CARTESIAN_POINT('Ctrl Pts',(-14.8773105066636,11.1074768631553,-323.051882114371)) ;
#39575=CARTESIAN_POINT('Ctrl Pts',(-15.0435410107717,10.8816439456824,-323.048244747554)) ;
#39576=CARTESIAN_POINT('Ctrl Pts',(-15.133444625169,10.7562611898794,-323.046231396909)) ;
#39577=CARTESIAN_POINT('Ctrl Pts',(-15.6941398917748,9.9533487032572,-323.033378836211)) ;
#39578=CARTESIAN_POINT('Ctrl Pts',(-16.1208901651071,9.24619186564224,-323.022191239364)) ;
#39579=CARTESIAN_POINT('Ctrl Pts',(-16.5979220084065,8.32164958215965,-323.008230013588)) ;
#39580=CARTESIAN_POINT('Ctrl Pts',(-16.6933207549158,8.12858592543286,-323.005352410259)) ;
#39581=CARTESIAN_POINT('Ctrl Pts',(-16.8492590606531,7.79867562975424,-323.000521509604)) ;
#39582=CARTESIAN_POINT('Ctrl Pts',(-16.9115419938052,7.66267707698794,-322.998554521327)) ;
#39583=CARTESIAN_POINT('Ctrl Pts',(-17.0028452961706,7.45677383075563,-322.995620941627)) ;
#39584=CARTESIAN_POINT('Ctrl Pts',(-17.0330927325559,7.38742012567348,-322.994640356556)) ;
#39585=CARTESIAN_POINT('Ctrl Pts',(-17.0893851923168,7.25616448453195,-322.992800079662)) ;
#39586=CARTESIAN_POINT('Ctrl Pts',(-17.1155198953955,7.19430246645539,-322.99193933814)) ;
#39587=CARTESIAN_POINT('Ctrl Pts',(-17.1827226844417,7.03279153716999,-322.989707871236)) ;
#39588=CARTESIAN_POINT('Ctrl Pts',(-17.2232597531966,6.93292428788047,-322.988343577622)) ;
#39589=CARTESIAN_POINT('Ctrl Pts',(-17.3533077633921,6.60435639011049,-322.983897688224)) ;
#39590=CARTESIAN_POINT('Ctrl Pts',(-17.4391508644068,6.37423181228684,-322.980850966978)) ;
#39591=CARTESIAN_POINT('Ctrl Pts',(-17.7149511566361,5.58755626624956,-322.970574351714)) ;
#39592=CARTESIAN_POINT('Ctrl Pts',(-17.8830256510212,5.02371123536483,-322.963430874508)) ;
#39593=CARTESIAN_POINT('Ctrl Pts',(-18.0625065034053,4.2972149511946,-322.954179956868)) ;
#39594=CARTESIAN_POINT('Ctrl Pts',(-18.0989369698454,4.14109623288026,-322.952190142788)) ;
#39595=CARTESIAN_POINT('Ctrl Pts',(-18.1826296642394,3.76021570295067,-322.947323206578)) ;
#39596=CARTESIAN_POINT('Ctrl Pts',(-18.2277519228483,3.53501106097198,-322.944434911236)) ;
#39597=CARTESIAN_POINT('Ctrl Pts',(-18.2927862148409,3.17596572402927,-322.939803018233)) ;
#39598=CARTESIAN_POINT('Ctrl Pts',(-18.3154333818866,3.04264453251384,-322.93807728118)) ;
#39599=CARTESIAN_POINT('Ctrl Pts',(-18.3564380114294,2.78418332336711,-322.934719069227)) ;
#39600=CARTESIAN_POINT('Ctrl Pts',(-18.3749772497311,2.65907958951756,-322.93308788694)) ;
#39601=CARTESIAN_POINT('Ctrl Pts',(-18.4126910806977,2.38532368279199,-322.929505527675)) ;
#39602=CARTESIAN_POINT('Ctrl Pts',(-18.4313467260544,2.23660896919226,-322.927551121723)) ;
#39603=CARTESIAN_POINT('Ctrl Pts',(-18.500287393079,1.62740246474633,-322.919511810699)) ;
#39604=CARTESIAN_POINT('Ctrl Pts',(-18.5351306587741,1.1653332872747,-322.913332425615)) ;
#39605=CARTESIAN_POINT('Ctrl Pts',(-18.5703583953788,0.234917139341171,
-322.900819677559)) ;
#39606=CARTESIAN_POINT('Ctrl Pts',(-18.5703811056925,-0.233114595382776,
-322.894490033861)) ;
#39607=CARTESIAN_POINT('Ctrl Pts',(-18.5465365329178,-0.864505845623008,
-322.88604998023)) ;
#39608=CARTESIAN_POINT('Ctrl Pts',(-18.5381777681597,-1.0282766550428,-322.883870318959)) ;
#39609=CARTESIAN_POINT('Ctrl Pts',(-18.5197035274377,-1.31544829007845,
-322.880076103168)) ;
#39610=CARTESIAN_POINT('Ctrl Pts',(-18.5105211479912,-1.43889883352907,
-322.878454086882)) ;
#39611=CARTESIAN_POINT('Ctrl Pts',(-18.4941492317929,-1.63277463555328,
-322.875925741264)) ;
#39612=CARTESIAN_POINT('Ctrl Pts',(-18.4877903702771,-1.70326629290526,
-322.875010412893)) ;
#39613=CARTESIAN_POINT('Ctrl Pts',(-18.4750569326367,-1.8359405784202,-322.873296233084)) ;
#39614=CARTESIAN_POINT('Ctrl Pts',(-18.4687711084613,-1.89813071910815,
-322.872496266676)) ;
#39615=CARTESIAN_POINT('Ctrl Pts',(-18.4499130892744,-2.07573726788903,
-322.870220402999)) ;
#39616=CARTESIAN_POINT('Ctrl Pts',(-18.4365721890096,-2.19106918870898,
-322.868753067158)) ;
#39617=CARTESIAN_POINT('Ctrl Pts',(-18.374737777818,-2.68499382332531,-322.862501371871)) ;
#39618=CARTESIAN_POINT('Ctrl Pts',(-18.3156574773483,-3.0621679804896,-322.857807316607)) ;
#39619=CARTESIAN_POINT('Ctrl Pts',(-18.1795910609839,-3.78441068004417,
-322.848796861754)) ;
#39620=CARTESIAN_POINT('Ctrl Pts',(-18.1042934974024,-4.12963100874972,
-322.844480332318)) ;
#39621=CARTESIAN_POINT('Ctrl Pts',(-17.9538384404681,-4.73579834774724,
-322.836788968964)) ;
#39622=CARTESIAN_POINT('Ctrl Pts',(-17.8827205571754,-4.99764003198292,
-322.833429320777)) ;
#39623=CARTESIAN_POINT('Ctrl Pts',(-17.7452308294695,-5.46325562450603,
-322.827358585756)) ;
#39624=CARTESIAN_POINT('Ctrl Pts',(-17.6810207713455,-5.66761708858894,
-322.824660409652)) ;
#39625=CARTESIAN_POINT('Ctrl Pts',(-17.5713877923288,-5.99653142922168,
-322.820254874485)) ;
#39626=CARTESIAN_POINT('Ctrl Pts',(-17.5281418345596,-6.12178910912928,
-322.81856225096)) ;
#39627=CARTESIAN_POINT('Ctrl Pts',(-17.4410106586243,-6.36566091493105,
-322.815236289201)) ;
#39628=CARTESIAN_POINT('Ctrl Pts',(-17.3972470106402,-6.48431091750484,
-322.813603861435)) ;
#39629=CARTESIAN_POINT('Ctrl Pts',(-17.2968857228202,-6.74807395571698,
-322.809942500152)) ;
#39630=CARTESIAN_POINT('Ctrl Pts',(-17.2396672871168,-6.89294055911324,
-322.807909427544)) ;
#39631=CARTESIAN_POINT('Ctrl Pts',(-16.9121528580071,-7.69254966820199,
-322.796565913654)) ;
#39632=CARTESIAN_POINT('Ctrl Pts',(-16.6063815128054,-8.33212576115319,
-322.787010772789)) ;
#39633=CARTESIAN_POINT('Ctrl Pts',(-16.1278884455994,-9.20143202801274,
-322.773653471666)) ;
#39634=CARTESIAN_POINT('Ctrl Pts',(-15.9852671611417,-9.44702975446794,
-322.769839652861)) ;
#39635=CARTESIAN_POINT('Ctrl Pts',(-15.7436834039316,-9.84189776200365,
-322.763688798819)) ;
#39636=CARTESIAN_POINT('Ctrl Pts',(-15.6480959823002,-9.99317822339049,
-322.761327755182)) ;
#39637=CARTESIAN_POINT('Ctrl Pts',(-15.5063066145703,-10.2105558021007,
-322.757941155485)) ;
#39638=CARTESIAN_POINT('Ctrl Pts',(-15.4618375611102,-10.2777708609849,
-322.756894854923)) ;
#39639=CARTESIAN_POINT('Ctrl Pts',(-15.3799419298375,-10.3998217753429,
-322.754998129675)) ;
#39640=CARTESIAN_POINT('Ctrl Pts',(-15.342656288674,-10.4547503425963,-322.754145865699)) ;
#39641=CARTESIAN_POINT('Ctrl Pts',(-15.2497074597909,-10.590112820872,-322.752048129485)) ;
#39642=CARTESIAN_POINT('Ctrl Pts',(-15.1937016983783,-10.6703090821572,
-322.750807374841)) ;
#39643=CARTESIAN_POINT('Ctrl Pts',(-14.950509631956,-11.0127457171388,-322.745510465112)) ;
#39644=CARTESIAN_POINT('Ctrl Pts',(-14.7571477027636,-11.2705323340075,
-322.741524831967)) ;
#39645=CARTESIAN_POINT('Ctrl Pts',(-14.4986398936552,-11.5971046097757,
-322.736403772201)) ;
#39646=CARTESIAN_POINT('Ctrl Pts',(-14.4395417058521,-11.6706053582831,
-322.735246400695)) ;
#39647=CARTESIAN_POINT('Ctrl Pts',(-14.1581689266422,-12.0151411368643,
-322.729792597873)) ;
#39648=CARTESIAN_POINT('Ctrl Pts',(-13.928807792406,-12.2802963054764,-322.725509615492)) ;
#39649=CARTESIAN_POINT('Ctrl Pts',(-13.5074152727782,-12.7404471859981,
-322.71782712948)) ;
#39650=CARTESIAN_POINT('Ctrl Pts',(-13.3183201648812,-12.9379909379211,
-322.714441781986)) ;
#39651=CARTESIAN_POINT('Ctrl Pts',(-12.9726296547381,-13.2835141636971,
-322.708331044084)) ;
#39652=CARTESIAN_POINT('Ctrl Pts',(-12.8176911047191,-13.4330809275679,
-322.705618850601)) ;
#39653=CARTESIAN_POINT('Ctrl Pts',(-12.5631165312608,-13.6704138326154,
-322.701196637184)) ;
#39654=CARTESIAN_POINT('Ctrl Pts',(-12.4650794708005,-13.7598657354793,
-322.699501575298)) ;
#39655=CARTESIAN_POINT('Ctrl Pts',(-12.2718578745426,-13.9324069953263,
-322.696174842626)) ;
#39656=CARTESIAN_POINT('Ctrl Pts',(-12.1767674930752,-14.0155910949952,
-322.694544126557)) ;
#39657=CARTESIAN_POINT('Ctrl Pts',(-11.9400211334082,-14.2184663120646,
-322.690499434486)) ;
#39658=CARTESIAN_POINT('Ctrl Pts',(-11.7974068554624,-14.3370178299206,
-322.688076111243)) ;
#39659=CARTESIAN_POINT('Ctrl Pts',(-11.277849402391,-14.7559101875759,-322.679296820116)) ;
#39660=CARTESIAN_POINT('Ctrl Pts',(-10.891022741352,-15.0436828575766,-322.67284642717)) ;
#39661=CARTESIAN_POINT('Ctrl Pts',(-10.0772907658551,-15.6011916367726,
-322.659571683811)) ;
#39662=CARTESIAN_POINT('Ctrl Pts',(-9.64969442359706,-15.8692270615061,
-322.652749277622)) ;
#39663=CARTESIAN_POINT('Ctrl Pts',(-9.06992225666922,-16.200545689302,-322.643892842789)) ;
#39664=CARTESIAN_POINT('Ctrl Pts',(-8.92706623668201,-16.2797008244498,
-322.641741675198)) ;
#39665=CARTESIAN_POINT('Ctrl Pts',(-8.71441540396617,-16.3938877734179,
-322.638595014131)) ;
#39666=CARTESIAN_POINT('Ctrl Pts',(-8.64541419574475,-16.430380566699,-322.637582509809)) ;
#39667=CARTESIAN_POINT('Ctrl Pts',(-8.51673218363405,-16.4974017876336,
-322.635711542434)) ;
#39668=CARTESIAN_POINT('Ctrl Pts',(-8.45711235293185,-16.528044151393,-322.634851692247)) ;
#39669=CARTESIAN_POINT('Ctrl Pts',(-8.32108678272701,-16.5970274989947,
-322.632904755465)) ;
#39670=CARTESIAN_POINT('Ctrl Pts',(-8.24457951267131,-16.6351650347717,
-322.631820210022)) ;
#39671=CARTESIAN_POINT('Ctrl Pts',(-7.90652348865025,-16.8007750333337,
-322.627068774591)) ;
#39672=CARTESIAN_POINT('Ctrl Pts',(-7.64226194797811,-16.9226176588425,
-322.623460784774)) ;
#39673=CARTESIAN_POINT('Ctrl Pts',(-6.84790706050794,-17.2664663539402,
-322.612799978036)) ;
#39674=CARTESIAN_POINT('Ctrl Pts',(-6.31025509066353,-17.4701280287219,
-322.605815410438)) ;
#39675=CARTESIAN_POINT('Ctrl Pts',(-5.61325079542622,-17.6977702760099,
-322.59674904727)) ;
#39676=CARTESIAN_POINT('Ctrl Pts',(-5.46185156870605,-17.7450791659003,
-322.594779802315)) ;
#39677=CARTESIAN_POINT('Ctrl Pts',(-5.09134551910705,-17.8556630983488,
-322.589953251791)) ;
#39678=CARTESIAN_POINT('Ctrl Pts',(-4.87164339100633,-17.9168522423779,
-322.587084813705)) ;
#39679=CARTESIAN_POINT('Ctrl Pts',(-4.52022852702689,-18.0077828577757,
-322.582476567261)) ;
#39680=CARTESIAN_POINT('Ctrl Pts',(-4.38922227563307,-18.0401617825421,
-322.580754282145)) ;
#39681=CARTESIAN_POINT('Ctrl Pts',(-4.13465534802278,-18.1001422781457,
-322.577397806033)) ;
#39682=CARTESIAN_POINT('Ctrl Pts',(-4.01114228166471,-18.1279139141295,
-322.575764850827)) ;
#39683=CARTESIAN_POINT('Ctrl Pts',(-3.74019654077387,-18.1859307642103,
-322.572172505606)) ;
#39684=CARTESIAN_POINT('Ctrl Pts',(-3.59266058338345,-18.2156509015746,
-322.570209808915)) ;
#39685=CARTESIAN_POINT('Ctrl Pts',(-2.99860315955674,-18.3278217403999,
-322.562281487074)) ;
#39686=CARTESIAN_POINT('Ctrl Pts',(-2.5494873876402,-18.3956729327063,-322.556225851467)) ;
#39687=CARTESIAN_POINT('Ctrl Pts',(-1.62782497544954,-18.5005116782299,
-322.54376235784)) ;
#39688=CARTESIAN_POINT('Ctrl Pts',(-1.15543668915085,-18.5360112306732,
-322.537354945567)) ;
#39689=CARTESIAN_POINT('Ctrl Pts',(-0.517445199277493,-18.5594701918291,
-322.528826093164)) ;
#39690=CARTESIAN_POINT('Ctrl Pts',(-0.352607441716422,-18.5633335219827,
-322.526634240782)) ;
#39691=CARTESIAN_POINT('Ctrl Pts',(-0.0634749710545198,-18.5662573963225,
-322.52282147745)) ;
#39692=CARTESIAN_POINT('Ctrl Pts',(0.0607997067637385,-18.5662663519132,
-322.521193008782)) ;
#39693=CARTESIAN_POINT('Ctrl Pts',(0.255933559320724,-18.5643211628228,
-322.518657028985)) ;
#39694=CARTESIAN_POINT('Ctrl Pts',(0.326797348675451,-18.5632089288624,
-322.517740433064)) ;
#39695=CARTESIAN_POINT('Ctrl Pts',(0.460077060916918,-18.5603536345706,
-322.516025840187)) ;
#39696=CARTESIAN_POINT('Ctrl Pts',(0.522493931622624,-18.5587014105402,
-322.51522671048)) ;
#39697=CARTESIAN_POINT('Ctrl Pts',(0.700540219090692,-18.5530894581941,
-322.512956728868)) ;
#39698=CARTESIAN_POINT('Ctrl Pts',(0.816142665487155,-18.5483637082764,
-322.511494368653)) ;
#39699=CARTESIAN_POINT('Ctrl Pts',(1.35586959976043,-18.5212444683981,-322.504706749635)) ;
#39700=CARTESIAN_POINT('Ctrl Pts',(1.77919062630473,-18.485382375016,-322.499495346281)) ;
#39701=CARTESIAN_POINT('Ctrl Pts',(2.64901054851744,-18.3815369150559,-322.488762686957)) ;
#39702=CARTESIAN_POINT('Ctrl Pts',(3.0950123364984,-18.311719049829,-322.48324521533)) ;
#39703=CARTESIAN_POINT('Ctrl Pts',(3.67534929554771,-18.1990624868313,-322.475914298686)) ;
#39704=CARTESIAN_POINT('Ctrl Pts',(3.81236726688987,-18.1708536842034,-322.474172645317)) ;
#39705=CARTESIAN_POINT('Ctrl Pts',(4.15378995607066,-18.096530934177,-322.469800717777)) ;
#39706=CARTESIAN_POINT('Ctrl Pts',(4.35775721340732,-18.048500067951,-322.467159927168)) ;
#39707=CARTESIAN_POINT('Ctrl Pts',(4.68852165900283,-17.9646766240867,-322.462822627848)) ;
#39708=CARTESIAN_POINT('Ctrl Pts',(4.81582792062362,-17.9309688230722,-322.461139956664)) ;
#39709=CARTESIAN_POINT('Ctrl Pts',(5.06519033783497,-17.8620961153777,-322.457816565212)) ;
#39710=CARTESIAN_POINT('Ctrl Pts',(5.18726569797387,-17.8270273830884,-322.456176569192)) ;
#39711=CARTESIAN_POINT('Ctrl Pts',(5.49071339324919,-17.7364747706402,-322.452066869102)) ;
#39712=CARTESIAN_POINT('Ctrl Pts',(5.67161332129041,-17.6794590701848,-322.449587109017)) ;
#39713=CARTESIAN_POINT('Ctrl Pts',(6.18912607636877,-17.5075898146768,-322.442409259899)) ;
#39714=CARTESIAN_POINT('Ctrl Pts',(6.52335327089297,-17.3858230712936,-322.437669281679)) ;
#39715=CARTESIAN_POINT('Ctrl Pts',(6.9370540463038,-17.2214921202381,-322.43169682807)) ;
#39716=CARTESIAN_POINT('Ctrl Pts',(7.01999232395873,-17.1878508677771,-322.43049418813)) ;
#39717=CARTESIAN_POINT('Ctrl Pts',(7.31943397746948,-17.0638630126255,-322.426134916864)) ;
#39718=CARTESIAN_POINT('Ctrl Pts',(7.53446333261199,-16.9700146411905,-322.422971442112)) ;
#39719=CARTESIAN_POINT('Ctrl Pts',(8.00025692286102,-16.7561227692663,-322.416073031352)) ;
#39720=CARTESIAN_POINT('Ctrl Pts',(8.25022111472117,-16.6344706244798,-322.412341268799)) ;
#39721=CARTESIAN_POINT('Ctrl Pts',(8.65435654787149,-16.4264357503732,-322.40630324816)) ;
#39722=CARTESIAN_POINT('Ctrl Pts',(8.81019271936543,-16.3433834671654,-322.403973959314)) ;
#39723=CARTESIAN_POINT('Ctrl Pts',(9.03507064487054,-16.2193844955481,-322.400623469226)) ;
#39724=CARTESIAN_POINT('Ctrl Pts',(9.10506896646183,-16.1801932655979,-322.399582108493)) ;
#39725=CARTESIAN_POINT('Ctrl Pts',(9.23259260294843,-16.107704700335,-322.39768937313)) ;
#39726=CARTESIAN_POINT('Ctrl Pts',(9.29019716498837,-16.0745498697289,-322.396836224092)) ;
#39727=CARTESIAN_POINT('Ctrl Pts',(9.43269765328075,-15.9915105579538,-322.394729422307)) ;
#39728=CARTESIAN_POINT('Ctrl Pts',(9.5173771388148,-15.9412586511136,-322.393480592396)) ;
#39729=CARTESIAN_POINT('Ctrl Pts',(9.89713389017053,-15.7117926001061,-322.387885796956)) ;
#39730=CARTESIAN_POINT('Ctrl Pts',(10.1875781451274,-15.5250423060953,-322.383621388743)) ;
#39731=CARTESIAN_POINT('Ctrl Pts',(11.0421017665899,-14.9412883994295,-322.370908913289)) ;
#39732=CARTESIAN_POINT('Ctrl Pts',(11.5894384998584,-14.5208480011863,-322.362523112885)) ;
#39733=CARTESIAN_POINT('Ctrl Pts',(12.2770699293531,-13.9289420137174,-322.351182996688)) ;
#39734=CARTESIAN_POINT('Ctrl Pts',(12.4395159273802,-13.7840601755729,-322.348442314322)) ;
#39735=CARTESIAN_POINT('Ctrl Pts',(12.6971494448055,-13.5460184459629,-322.343986194695)) ;
#39736=CARTESIAN_POINT('Ctrl Pts',(12.7939475983153,-13.454632085342,-322.342286171533)) ;
#39737=CARTESIAN_POINT('Ctrl Pts',(12.9805081825982,-13.2746678700117,-322.338957714887)) ;
#39738=CARTESIAN_POINT('Ctrl Pts',(13.0703675598689,-13.1862007998507,-322.337330324653)) ;
#39739=CARTESIAN_POINT('Ctrl Pts',(13.2680140228534,-12.9876112384417,-322.333696084767)) ;
#39740=CARTESIAN_POINT('Ctrl Pts',(13.3753454511505,-12.877048410202,-322.331685309123)) ;
#39741=CARTESIAN_POINT('Ctrl Pts',(13.9804509658335,-12.237996478676,-322.320135484392)) ;
#39742=CARTESIAN_POINT('Ctrl Pts',(14.4482616813532,-11.6820072176031,-322.310336528142)) ;
#39743=CARTESIAN_POINT('Ctrl Pts',(15.0470480272017,-10.8791896765663,-322.296858039948)) ;
#39744=CARTESIAN_POINT('Ctrl Pts',(15.2068491544979,-10.6546779138979,-322.293159307168)) ;
#39745=CARTESIAN_POINT('Ctrl Pts',(15.4602200753268,-10.2813878061923,-322.287166850157)) ;
#39746=CARTESIAN_POINT('Ctrl Pts',(15.5567794773916,-10.1346905466541,-322.284850485168)) ;
#39747=CARTESIAN_POINT('Ctrl Pts',(15.6943128293501,-9.91914589985208,-322.281514710889)) ;
#39748=CARTESIAN_POINT('Ctrl Pts',(15.7369453722879,-9.85136848064576,-322.280475378158)) ;
#39749=CARTESIAN_POINT('Ctrl Pts',(15.8141788118294,-9.72680162147317,-322.27858426035)) ;
#39750=CARTESIAN_POINT('Ctrl Pts',(15.8489155049886,-9.67009816832151,-322.27773072761)) ;
#39751=CARTESIAN_POINT('Ctrl Pts',(15.9344727764156,-9.52873686196501,-322.275620107367)) ;
#39752=CARTESIAN_POINT('Ctrl Pts',(15.9849240681972,-9.44385786752175,-322.27436788692)) ;
#39753=CARTESIAN_POINT('Ctrl Pts',(16.2026784757274,-9.07076434642673,-322.268921122029)) ;
#39754=CARTESIAN_POINT('Ctrl Pts',(16.3628817658125,-8.77847691501777,-322.264801991637)) ;
#39755=CARTESIAN_POINT('Ctrl Pts',(16.7605906175474,-8.00410929579952,-322.254104012751)) ;
#39756=CARTESIAN_POINT('Ctrl Pts',(16.985188154469,-7.51575327708908,-322.247562732555)) ;
#39757=CARTESIAN_POINT('Ctrl Pts',(17.272892710054,-6.81115001590324,-322.238145272996)) ;
#39758=CARTESIAN_POINT('Ctrl Pts',(17.3537417272353,-6.6024415909807,-322.235359421902)) ;
#39759=CARTESIAN_POINT('Ctrl Pts',(17.4953337785239,-6.21634369698405,-322.230197547204)) ;
#39760=CARTESIAN_POINT('Ctrl Pts',(17.557201095437,-6.03939752916188,-322.227828831957)) ;
#39761=CARTESIAN_POINT('Ctrl Pts',(17.6567655862335,-5.74016487002462,-322.223812955855)) ;
#39762=CARTESIAN_POINT('Ctrl Pts',(17.6958971599025,-5.61837052473176,-322.22217564164)) ;
#39763=CARTESIAN_POINT('Ctrl Pts',(17.7683176808687,-5.38470127482329,-322.219028114743)) ;
#39764=CARTESIAN_POINT('Ctrl Pts',(17.8018164992113,-5.27289771504453,-322.21751941301)) ;
#39765=CARTESIAN_POINT('Ctrl Pts',(17.8892105903719,-4.9708877310793,-322.213436400646)) ;
#39766=CARTESIAN_POINT('Ctrl Pts',(17.9411257008595,-4.78012434667114,-322.210849175349)) ;
#39767=CARTESIAN_POINT('Ctrl Pts',(18.0725872114106,-4.26471513382368,-322.203839597565)) ;
#39768=CARTESIAN_POINT('Ctrl Pts',(18.1464298710929,-3.93869088019811,-322.199384311686)) ;
#39769=CARTESIAN_POINT('Ctrl Pts',(18.311241752124,-3.10745762984853,-322.188016484232)) ;
#39770=CARTESIAN_POINT('Ctrl Pts',(18.3901367340055,-2.60014185461628,-322.181066576659)) ;
#39771=CARTESIAN_POINT('Ctrl Pts',(18.4756607474731,-1.8453188249167,-322.170911456651)) ;
#39772=CARTESIAN_POINT('Ctrl Pts',(18.4985288482755,-1.59989765106995,-322.167639679005)) ;
#39773=CARTESIAN_POINT('Ctrl Pts',(18.5230267638305,-1.26490183827105,-322.163244458239)) ;
#39774=CARTESIAN_POINT('Ctrl Pts',(18.528904765265,-1.17566380638093,-322.162080494127)) ;
#39775=CARTESIAN_POINT('Ctrl Pts',(18.5379858226082,-1.02073778824992,-322.160073677379)) ;
#39776=CARTESIAN_POINT('Ctrl Pts',(18.5414850279525,-0.955069081350536,
-322.159227513438)) ;
#39777=CARTESIAN_POINT('Ctrl Pts',(18.5446417153482,-0.889248593493978,
-322.158383873619)) ;
#39778=CARTESIAN_POINT('Ctrl Pts',(18.5446481553962,-0.889114285759121,
-322.158382152315)) ;
#39779=CARTESIAN_POINT('Ctrl Pts',(18.5446545937451,-0.888979977946956,
-322.15838043089)) ;
#39780=CARTESIAN_POINT('',(0.000274526296954267,-18.5659499979704,-322.226379248718)) ;
#39781=CARTESIAN_POINT('Ctrl Pts',(18.5446545931659,-0.888979990027976,
-321.863010318849)) ;
#39782=CARTESIAN_POINT('Ctrl Pts',(18.535675921736,-1.07628044925217,-321.865335837486)) ;
#39783=CARTESIAN_POINT('Ctrl Pts',(18.5238593692262,-1.26345088814058,-321.867674125245)) ;
#39784=CARTESIAN_POINT('Ctrl Pts',(18.4947201691002,-1.63530246681083,-321.87235735625)) ;
#39785=CARTESIAN_POINT('Ctrl Pts',(18.4774638015849,-1.8199504380384,-321.874701456261)) ;
#39786=CARTESIAN_POINT('Ctrl Pts',(18.4438053970694,-2.12990675361984,-321.878672437106)) ;
#39787=CARTESIAN_POINT('Ctrl Pts',(18.4288849724849,-2.25536225954101,-321.880289648314)) ;
#39788=CARTESIAN_POINT('Ctrl Pts',(18.39566820886,-2.51227040600905,-321.883622804306)) ;
#39789=CARTESIAN_POINT('Ctrl Pts',(18.3772404824554,-2.64369885407315,-321.885339520908)) ;
#39790=CARTESIAN_POINT('Ctrl Pts',(18.325220281141,-2.9878372447093,-321.889865416447)) ;
#39791=CARTESIAN_POINT('Ctrl Pts',(18.2893334714954,-3.20017978694584,-321.892689095903)) ;
#39792=CARTESIAN_POINT('Ctrl Pts',(18.1995127783954,-3.68062481398582,-321.89914503651)) ;
#39793=CARTESIAN_POINT('Ctrl Pts',(18.1433330176666,-3.94825670301182,-321.902789360683)) ;
#39794=CARTESIAN_POINT('Ctrl Pts',(18.0016947012494,-4.55591348932771,-321.911151368143)) ;
#39795=CARTESIAN_POINT('Ctrl Pts',(17.9124752699819,-4.89495548653125,-321.915880930624)) ;
#39796=CARTESIAN_POINT('Ctrl Pts',(17.7871422360078,-5.32174430435427,-321.921868077427)) ;
#39797=CARTESIAN_POINT('Ctrl Pts',(17.7598834962691,-5.41201714443049,-321.923136279583)) ;
#39798=CARTESIAN_POINT('Ctrl Pts',(17.6364420973623,-5.80984049331601,-321.928728902645)) ;
#39799=CARTESIAN_POINT('Ctrl Pts',(17.5329495202847,-6.11506486258897,-321.93303072531)) ;
#39800=CARTESIAN_POINT('Ctrl Pts',(17.38776086875,-6.50921162407933,-321.938539205523)) ;
#39801=CARTESIAN_POINT('Ctrl Pts',(17.3532314681898,-6.60071372259848,-321.939814602295)) ;
#39802=CARTESIAN_POINT('Ctrl Pts',(17.2940525325771,-6.75386211403319,-321.941940950671)) ;
#39803=CARTESIAN_POINT('Ctrl Pts',(17.2697924373257,-6.81565665666956,-321.942796558143)) ;
#39804=CARTESIAN_POINT('Ctrl Pts',(17.2153441378235,-6.95218831295049,-321.94468119804)) ;
#39805=CARTESIAN_POINT('Ctrl Pts',(17.1849996716115,-7.02686149238606,-321.945708348992)) ;
#39806=CARTESIAN_POINT('Ctrl Pts',(17.0857039699265,-7.26672278496012,-321.948999371421)) ;
#39807=CARTESIAN_POINT('Ctrl Pts',(17.0148497014702,-7.43111230012272,-321.951242150917)) ;
#39808=CARTESIAN_POINT('Ctrl Pts',(16.825408565896,-7.85371575208497,-321.957001979528)) ;
#39809=CARTESIAN_POINT('Ctrl Pts',(16.7032515628816,-8.11027818030459,-321.960493485417)) ;
#39810=CARTESIAN_POINT('Ctrl Pts',(16.2563345702195,-8.9959572317637,-321.972655198958)) ;
#39811=CARTESIAN_POINT('Ctrl Pts',(15.9015262046198,-9.60922078533316,-321.981294049578)) ;
#39812=CARTESIAN_POINT('Ctrl Pts',(15.4269603602362,-10.3309085297965,-321.992161902245)) ;
#39813=CARTESIAN_POINT('Ctrl Pts',(15.339716525285,-10.4600130897495,-321.994133737819)) ;
#39814=CARTESIAN_POINT('Ctrl Pts',(15.1787308685438,-10.6918952641756,-321.997728798913)) ;
#39815=CARTESIAN_POINT('Ctrl Pts',(15.1055440825231,-10.7950466899102,-321.999347646884)) ;
#39816=CARTESIAN_POINT('Ctrl Pts',(14.9535443735311,-11.0047064042251,-322.00267946985)) ;
#39817=CARTESIAN_POINT('Ctrl Pts',(14.8746337735717,-11.1111350641795,-322.004393167684)) ;
#39818=CARTESIAN_POINT('Ctrl Pts',(14.6652579711084,-11.3872970908768,-322.00889932241)) ;
#39819=CARTESIAN_POINT('Ctrl Pts',(14.5329845584379,-11.5556343820061,-322.011706039199)) ;
#39820=CARTESIAN_POINT('Ctrl Pts',(14.3066820445924,-11.8336043029948,-322.016439793426)) ;
#39821=CARTESIAN_POINT('Ctrl Pts',(14.2142314600262,-11.9444952116615,-322.018355477367)) ;
#39822=CARTESIAN_POINT('Ctrl Pts',(13.8104663827197,-12.4174687769428,-322.026639631045)) ;
#39823=CARTESIAN_POINT('Ctrl Pts',(13.4865405778721,-12.768544722777,-322.033084477673)) ;
#39824=CARTESIAN_POINT('Ctrl Pts',(13.0009110167178,-13.2557564631522,-322.042344332145)) ;
#39825=CARTESIAN_POINT('Ctrl Pts',(12.849856953625,-13.4022364946781,-322.045171633086)) ;
#39826=CARTESIAN_POINT('Ctrl Pts',(12.5290381005741,-13.7029298211261,-322.051043866911)) ;
#39827=CARTESIAN_POINT('Ctrl Pts',(12.3588391409912,-13.8566293465554,-322.054085050731)) ;
#39828=CARTESIAN_POINT('Ctrl Pts',(12.1248516071538,-14.0601922805303,-322.058143468442)) ;
#39829=CARTESIAN_POINT('Ctrl Pts',(12.0635206111987,-14.1128488955102,-322.059196123107)) ;
#39830=CARTESIAN_POINT('Ctrl Pts',(11.9513214212688,-14.2079133331656,-322.061100185692)) ;
#39831=CARTESIAN_POINT('Ctrl Pts',(11.9005665166872,-14.2504526809463,-322.061953481352)) ;
#39832=CARTESIAN_POINT('Ctrl Pts',(11.8347431674475,-14.3050244755886,-322.063049517435)) ;
#39833=CARTESIAN_POINT('Ctrl Pts',(11.8198822704366,-14.3173061083432,-322.063296290273)) ;
#39834=CARTESIAN_POINT('Ctrl Pts',(11.8035379939324,-14.3307708734579,-322.063566966799)) ;
#39835=CARTESIAN_POINT('Ctrl Pts',(11.8020735360014,-14.3319769485082,-322.063591213178)) ;
#39836=CARTESIAN_POINT('Ctrl Pts',(11.7981766645179,-14.3351852698509,-322.063655714919)) ;
#39837=CARTESIAN_POINT('Ctrl Pts',(11.7957439260656,-14.3371871215666,-322.063695964409)) ;
#39838=CARTESIAN_POINT('Ctrl Pts',(11.7911234627865,-14.3409872361603,-322.063772376267)) ;
#39839=CARTESIAN_POINT('Ctrl Pts',(11.7889358358678,-14.3427856178701,-322.063808540391)) ;
#39840=CARTESIAN_POINT('Ctrl Pts',(11.7847961856874,-14.3461871117266,-322.063876947042)) ;
#39841=CARTESIAN_POINT('Ctrl Pts',(11.7828442465864,-14.3477903261634,-322.063909191072)) ;
#39842=CARTESIAN_POINT('Ctrl Pts',(11.779164081544,-14.350811751976,-322.063969962458)) ;
#39843=CARTESIAN_POINT('Ctrl Pts',(11.7774359264955,-14.3522300496432,-322.063998491075)) ;
#39844=CARTESIAN_POINT('Ctrl Pts',(11.7741893089175,-14.3548935689742,-322.064052070205)) ;
#39845=CARTESIAN_POINT('Ctrl Pts',(11.7726709049408,-14.3561388619212,-322.064077121754)) ;
#39846=CARTESIAN_POINT('Ctrl Pts',(11.7698281175199,-14.3584695709068,-322.06412401115)) ;
#39847=CARTESIAN_POINT('Ctrl Pts',(11.7685037814176,-14.3595550446864,-322.064145849833)) ;
#39848=CARTESIAN_POINT('Ctrl Pts',(11.7660323636788,-14.3615801365324,-322.064186594668)) ;
#39849=CARTESIAN_POINT('Ctrl Pts',(11.7648853196421,-14.3625198003988,-322.064205501481)) ;
#39850=CARTESIAN_POINT('Ctrl Pts',(11.7627512060374,-14.364267649095,-322.064240671105)) ;
#39851=CARTESIAN_POINT('Ctrl Pts',(11.7617641657249,-14.3650758696165,-322.06425693443)) ;
#39852=CARTESIAN_POINT('Ctrl Pts',(11.7599328145455,-14.3665751238862,-322.064287104093)) ;
#39853=CARTESIAN_POINT('Ctrl Pts',(11.7590885260315,-14.3672661849721,-322.064301010824)) ;
#39854=CARTESIAN_POINT('Ctrl Pts',(11.757525944384,-14.3685449482881,-322.064326745118)) ;
#39855=CARTESIAN_POINT('Ctrl Pts',(11.7568076681107,-14.3691326710728,-322.064338572977)) ;
#39856=CARTESIAN_POINT('Ctrl Pts',(11.755481265493,-14.3702178214666,-322.064360412094)) ;
#39857=CARTESIAN_POINT('Ctrl Pts',(11.7548731515948,-14.3707152643725,-322.064370423571)) ;
#39858=CARTESIAN_POINT('Ctrl Pts',(11.7537523853557,-14.3716319429916,-322.064388872954)) ;
#39859=CARTESIAN_POINT('Ctrl Pts',(11.7532397421933,-14.3720511898476,-322.064397311019)) ;
#39860=CARTESIAN_POINT('Ctrl Pts',(11.7513601101291,-14.3735882118087,-322.064428246823)) ;
#39861=CARTESIAN_POINT('Ctrl Pts',(11.7499929842702,-14.374705819257,-322.064450742175)) ;
#39862=CARTESIAN_POINT('Ctrl Pts',(11.7472982812165,-14.376908062359,-322.064495071502)) ;
#39863=CARTESIAN_POINT('Ctrl Pts',(11.7459707131715,-14.3779927092315,-322.064516905637)) ;
#39864=CARTESIAN_POINT('Ctrl Pts',(11.7433560711052,-14.3801283148243,-322.06455989793)) ;
#39865=CARTESIAN_POINT('Ctrl Pts',(11.7420690061799,-14.3811792846652,-322.064581056246)) ;
#39866=CARTESIAN_POINT('Ctrl Pts',(11.6599381424263,-14.448225948841,-322.065930918547)) ;
#39867=CARTESIAN_POINT('Ctrl Pts',(11.5785393785103,-14.5135390742588,-322.067250013829)) ;
#39868=CARTESIAN_POINT('Ctrl Pts',(11.3831437054603,-14.6676315234339,-322.070377291639)) ;
#39869=CARTESIAN_POINT('Ctrl Pts',(11.2686525441204,-14.7557732788085,-322.07217844202)) ;
#39870=CARTESIAN_POINT('Ctrl Pts',(10.8645300687677,-15.0594428120212,-322.078446466134)) ;
#39871=CARTESIAN_POINT('Ctrl Pts',(10.5696513811148,-15.2678519043173,-322.082863099093)) ;
#39872=CARTESIAN_POINT('Ctrl Pts',(9.79620043689015,-15.7813455004837,-322.094234261653)) ;
#39873=CARTESIAN_POINT('Ctrl Pts',(9.30938045641168,-16.0733270658502,-322.101197275441)) ;
#39874=CARTESIAN_POINT('Ctrl Pts',(8.64785098806182,-16.4299448522855,-322.110635313847)) ;
#39875=CARTESIAN_POINT('Ctrl Pts',(8.48445369121153,-16.5149162871027,-322.112963614673)) ;
#39876=CARTESIAN_POINT('Ctrl Pts',(8.20815657212574,-16.653416067908,-322.116900538467)) ;
#39877=CARTESIAN_POINT('Ctrl Pts',(8.09593169778051,-16.708261158385,-322.118499552128)) ;
#39878=CARTESIAN_POINT('Ctrl Pts',(7.87716299809421,-16.8124533281273,-322.121617424277)) ;
#39879=CARTESIAN_POINT('Ctrl Pts',(7.77068756868404,-16.8619304492606,-322.123135258033)) ;
#39880=CARTESIAN_POINT('Ctrl Pts',(7.49739174486862,-16.985787460795,-322.127032396544)) ;
#39881=CARTESIAN_POINT('Ctrl Pts',(7.32993014003453,-17.0587215999645,-322.129421602249)) ;
#39882=CARTESIAN_POINT('Ctrl Pts',(6.94909899666808,-17.2179407141432,-322.134856139573)) ;
#39883=CARTESIAN_POINT('Ctrl Pts',(6.73514628559345,-17.3027530626543,-322.137910202091)) ;
#39884=CARTESIAN_POINT('Ctrl Pts',(5.98059693556983,-17.5857453287367,-322.148667466031)) ;
#39885=CARTESIAN_POINT('Ctrl Pts',(5.43240854829221,-17.7627394762174,-322.156468329422)) ;
#39886=CARTESIAN_POINT('Ctrl Pts',(4.5974384296159,-17.9900510861332,-322.168068662631)) ;
#39887=CARTESIAN_POINT('Ctrl Pts',(4.31624806872453,-18.0595786608134,-322.171926300698)) ;
#39888=CARTESIAN_POINT('Ctrl Pts',(3.950169654302,-18.1410571669753,-322.176840643701)) ;
#39889=CARTESIAN_POINT('Ctrl Pts',(3.86666588556886,-18.159038806875,-322.177954363148)) ;
#39890=CARTESIAN_POINT('Ctrl Pts',(3.71742782304458,-18.1900995420399,-322.179930054271)) ;
#39891=CARTESIAN_POINT('Ctrl Pts',(3.65174117689683,-18.2034001600166,-322.180794515968)) ;
#39892=CARTESIAN_POINT('Ctrl Pts',(3.52534452759131,-18.2282820082814,-322.182447422676)) ;
#39893=CARTESIAN_POINT('Ctrl Pts',(3.46464604548661,-18.2399163046955,-322.183236668903)) ;
#39894=CARTESIAN_POINT('Ctrl Pts',(3.32561902237845,-18.2658450954218,-322.18503515042)) ;
#39895=CARTESIAN_POINT('Ctrl Pts',(3.24725431919159,-18.2799392323626,-322.186042190625)) ;
#39896=CARTESIAN_POINT('Ctrl Pts',(3.04055253725548,-18.3157440727528,-322.188683367376)) ;
#39897=CARTESIAN_POINT('Ctrl Pts',(2.9120735392729,-18.3366100586124,-322.190309770728)) ;
#39898=CARTESIAN_POINT('Ctrl Pts',(1.8622602576627,-18.4957959163459,-322.203507515841)) ;
#39899=CARTESIAN_POINT('Ctrl Pts',(0.931937063063516,-18.5659362218982,
-322.214702258193)) ;
#39900=CARTESIAN_POINT('Ctrl Pts',(0.000274526296958344,-18.5659499979704,
-322.226379248718)) ;
#39901=CARTESIAN_POINT('Ctrl Pts',(0.000274526296966671,-18.5659499979704,
-322.226379248718)) ;
#39902=CARTESIAN_POINT('Ctrl Pts',(-0.17127499577746,-18.5659525345955,
-322.228529364307)) ;
#39903=CARTESIAN_POINT('Ctrl Pts',(-0.342816106782395,-18.5635773933165,
-322.230692607528)) ;
#39904=CARTESIAN_POINT('Ctrl Pts',(-0.6306775490769,-18.5556002192189,-322.234349106168)) ;
#39905=CARTESIAN_POINT('Ctrl Pts',(-0.747022644124064,-18.5512805702038,
-322.23583417216)) ;
#39906=CARTESIAN_POINT('Ctrl Pts',(-0.982475836102893,-18.5403201072191,
-322.238855149987)) ;
#39907=CARTESIAN_POINT('Ctrl Pts',(-1.101576030394,-18.5336250812034,-322.240391344776)) ;
#39908=CARTESIAN_POINT('Ctrl Pts',(-1.37989345246346,-18.5152876551864,
-322.244000657076)) ;
#39909=CARTESIAN_POINT('Ctrl Pts',(-1.53904140381831,-18.5027385633866,
-322.246079501278)) ;
#39910=CARTESIAN_POINT('Ctrl Pts',(-2.10919646486465,-18.450373768721,-322.253580164116)) ;
#39911=CARTESIAN_POINT('Ctrl Pts',(-2.51900994752054,-18.3989018484258,
-322.259073337982)) ;
#39912=CARTESIAN_POINT('Ctrl Pts',(-3.3943499302506,-18.2591647059414,-322.270962533878)) ;
#39913=CARTESIAN_POINT('Ctrl Pts',(-3.8589079977686,-18.1666600040671,-322.277369468432)) ;
#39914=CARTESIAN_POINT('Ctrl Pts',(-4.58924822288483,-17.991950246664,-322.287431142309)) ;
#39915=CARTESIAN_POINT('Ctrl Pts',(-4.85759603396007,-17.9213625107553,
-322.291124529114)) ;
#39916=CARTESIAN_POINT('Ctrl Pts',(-5.19523388521698,-17.8244073322759,
-322.295728358093)) ;
#39917=CARTESIAN_POINT('Ctrl Pts',(-5.26608432653722,-17.8036037855265,
-322.29669196258)) ;
#39918=CARTESIAN_POINT('Ctrl Pts',(-5.39474680641894,-17.7649898805929,
-322.298436151604)) ;
#39919=CARTESIAN_POINT('Ctrl Pts',(-5.45259950972636,-17.7473185907129,
-322.299218317454)) ;
#39920=CARTESIAN_POINT('Ctrl Pts',(-5.56912535076216,-17.7111018449986,
-322.300788735408)) ;
#39921=CARTESIAN_POINT('Ctrl Pts',(-5.6277946977462,-17.6925468087214,-322.301576808449)) ;
#39922=CARTESIAN_POINT('Ctrl Pts',(-5.79128287986047,-17.6399458033243,
-322.303766836397)) ;
#39923=CARTESIAN_POINT('Ctrl Pts',(-5.8958925296753,-17.6052576428838,-322.305161236504)) ;
#39924=CARTESIAN_POINT('Ctrl Pts',(-6.56866592757272,-17.3754995875418,
-322.314100896557)) ;
#39925=CARTESIAN_POINT('Ctrl Pts',(-7.12738926330805,-17.1538825171434,
-322.321407125439)) ;
#39926=CARTESIAN_POINT('Ctrl Pts',(-7.99246583352356,-16.7611758012988,
-322.333055275585)) ;
#39927=CARTESIAN_POINT('Ctrl Pts',(-8.30640736381268,-16.6078331092422,
-322.337353110021)) ;
#39928=CARTESIAN_POINT('Ctrl Pts',(-8.77697786698898,-16.3613035222652,
-322.343966244176)) ;
#39929=CARTESIAN_POINT('Ctrl Pts',(-8.9368708743613,-16.2745178813324,-322.346243932381)) ;
#39930=CARTESIAN_POINT('Ctrl Pts',(-9.2346352756907,-16.1071877256535,-322.350550565587)) ;
#39931=CARTESIAN_POINT('Ctrl Pts',(-9.37279342024897,-16.0271871675418,
-322.352575618555)) ;
#39932=CARTESIAN_POINT('Ctrl Pts',(-9.593731726245,-15.8954187715121,-322.355860161626)) ;
#39933=CARTESIAN_POINT('Ctrl Pts',(-9.67716537056744,-15.8447624381988,
-322.357111282986)) ;
#39934=CARTESIAN_POINT('Ctrl Pts',(-9.84344097751455,-15.7420057642807,
-322.359626733205)) ;
#39935=CARTESIAN_POINT('Ctrl Pts',(-9.9262782378198,-15.6899036351665,-322.360891048471)) ;
#39936=CARTESIAN_POINT('Ctrl Pts',(-10.1630327761385,-15.5383667371287,
-322.364536941529)) ;
#39937=CARTESIAN_POINT('Ctrl Pts',(-10.3158948190304,-15.437305140142,-322.366930764325)) ;
#39938=CARTESIAN_POINT('Ctrl Pts',(-10.9580991120082,-14.9989260647076,
-322.37715583758)) ;
#39939=CARTESIAN_POINT('Ctrl Pts',(-11.4325889155877,-14.6404790047745,
-322.38514380207)) ;
#39940=CARTESIAN_POINT('Ctrl Pts',(-12.153093705884,-14.0397642789368,-322.397780346735)) ;
#39941=CARTESIAN_POINT('Ctrl Pts',(-12.4109569763725,-13.8123428461418,
-322.402411493097)) ;
#39942=CARTESIAN_POINT('Ctrl Pts',(-12.7653435244286,-13.4818520334931,
-322.408864723883)) ;
#39943=CARTESIAN_POINT('Ctrl Pts',(-12.8672336228626,-13.3846415166313,
-322.410730718596)) ;
#39944=CARTESIAN_POINT('Ctrl Pts',(-12.9695356351892,-13.2847901514057,
-322.412610979222)) ;
#39945=CARTESIAN_POINT('Ctrl Pts',(-12.971063004959,-13.2832988553561,-322.412639053056)) ;
#39946=CARTESIAN_POINT('Ctrl Pts',(-12.9772950777296,-13.2772118730777,
-322.412753607913)) ;
#39947=CARTESIAN_POINT('Ctrl Pts',(-12.9819975960612,-13.2726139502712,
-322.412840061649)) ;
#39948=CARTESIAN_POINT('Ctrl Pts',(-12.9908773040995,-13.2639225147793,
-322.413003337542)) ;
#39949=CARTESIAN_POINT('Ctrl Pts',(-12.995055004569,-13.2598295251663,-322.41308016617)) ;
#39950=CARTESIAN_POINT('Ctrl Pts',(-13.0029477592488,-13.2520894984617,
-322.413225335567)) ;
#39951=CARTESIAN_POINT('Ctrl Pts',(-13.0066632148376,-13.2484428715525,
-322.413293681487)) ;
#39952=CARTESIAN_POINT('Ctrl Pts',(-13.0136866047863,-13.241543787482,-322.413422892637)) ;
#39953=CARTESIAN_POINT('Ctrl Pts',(-13.0169948548552,-13.2382916523272,
-322.413483761967)) ;
#39954=CARTESIAN_POINT('Ctrl Pts',(-13.0232522075587,-13.2321358241763,
-322.413598904748)) ;
#39955=CARTESIAN_POINT('Ctrl Pts',(-13.0262015588289,-13.229232384379,-322.413653181462)) ;
#39956=CARTESIAN_POINT('Ctrl Pts',(-13.0877306517851,-13.1686205667784,
-322.414785601769)) ;
#39957=CARTESIAN_POINT('Ctrl Pts',(-13.1459273849018,-13.1105245684571,
-322.415858673326)) ;
#39958=CARTESIAN_POINT('Ctrl Pts',(-13.2518163449607,-13.0034049538387,
-322.41781312738)) ;
#39959=CARTESIAN_POINT('Ctrl Pts',(-13.2996273712613,-12.9545007105393,
-322.418696343608)) ;
#39960=CARTESIAN_POINT('Ctrl Pts',(-13.3991735811314,-12.8515463831969,
-322.420535812825)) ;
#39961=CARTESIAN_POINT('Ctrl Pts',(-13.4508544070228,-12.7974455590814,
-322.421491259464)) ;
#39962=CARTESIAN_POINT('Ctrl Pts',(-13.6016823651333,-12.637631944614,-322.424283491572)) ;
#39963=CARTESIAN_POINT('Ctrl Pts',(-13.6999204367205,-12.5310687681045,
-322.426107067187)) ;
#39964=CARTESIAN_POINT('Ctrl Pts',(-14.0202785818352,-12.1752916390353,
-322.432089187644)) ;
#39965=CARTESIAN_POINT('Ctrl Pts',(-14.2369254060334,-11.9212370905213,
-322.436193177196)) ;
#39966=CARTESIAN_POINT('Ctrl Pts',(-14.7471156158916,-11.2891975411636,
-322.446151181402)) ;
#39967=CARTESIAN_POINT('Ctrl Pts',(-15.0331238700007,-10.9054383984895,
-322.451992394644)) ;
#39968=CARTESIAN_POINT('Ctrl Pts',(-15.3858101438176,-10.3919311255983,
-322.459711562054)) ;
#39969=CARTESIAN_POINT('Ctrl Pts',(-15.4662375685578,-10.2718489920668,
-322.461509604472)) ;
#39970=CARTESIAN_POINT('Ctrl Pts',(-15.6623821064718,-9.97146826035132,
-322.465995508089)) ;
#39971=CARTESIAN_POINT('Ctrl Pts',(-15.7763960030746,-9.79008281069018,
-322.46869406625)) ;
#39972=CARTESIAN_POINT('Ctrl Pts',(-15.9558136905284,-9.49336974146189,
-322.473100055769)) ;
#39973=CARTESIAN_POINT('Ctrl Pts',(-16.0231660738069,-9.3792434921586,-322.474792745539)) ;
#39974=CARTESIAN_POINT('Ctrl Pts',(-16.1523929056292,-9.1548180881739,-322.478118727095)) ;
#39975=CARTESIAN_POINT('Ctrl Pts',(-16.2143736361861,-9.0445883453869,-322.479751107198)) ;
#39976=CARTESIAN_POINT('Ctrl Pts',(-16.3501616114037,-8.79721366450402,
-322.483412214697)) ;
#39977=CARTESIAN_POINT('Ctrl Pts',(-16.4233790921494,-8.6597558900629,-322.485445079188)) ;
#39978=CARTESIAN_POINT('Ctrl Pts',(-16.8200155949451,-7.89198673975013,
-322.496789695689)) ;
#39979=CARTESIAN_POINT('Ctrl Pts',(-17.1088801753455,-7.2444868979147,-322.506346237202)) ;
#39980=CARTESIAN_POINT('Ctrl Pts',(-17.4606946912828,-6.31658576798109,
-322.519704372618)) ;
#39981=CARTESIAN_POINT('Ctrl Pts',(-17.5552509096346,-6.04882473553525,
-322.523517657129)) ;
#39982=CARTESIAN_POINT('Ctrl Pts',(-17.6993226692579,-5.60896516899133,
-322.529667778063)) ;
#39983=CARTESIAN_POINT('Ctrl Pts',(-17.752555321532,-5.43813322456599,-322.532028616482)) ;
#39984=CARTESIAN_POINT('Ctrl Pts',(-17.8261713374102,-5.18927833875265,
-322.535414982942)) ;
#39985=CARTESIAN_POINT('Ctrl Pts',(-17.8485288427502,-5.11185019356561,
-322.536461251682)) ;
#39986=CARTESIAN_POINT('Ctrl Pts',(-17.8883830932591,-4.97037796290353,
-322.538357950831)) ;
#39987=CARTESIAN_POINT('Ctrl Pts',(-17.90604175566,-4.90638109243522,-322.539210220114)) ;
#39988=CARTESIAN_POINT('Ctrl Pts',(-17.9488695463753,-4.747857408782,-322.541308012954)) ;
#39989=CARTESIAN_POINT('Ctrl Pts',(-17.9736355987195,-4.65322376116195,
-322.542548818255)) ;
#39990=CARTESIAN_POINT('Ctrl Pts',(-18.0788474256281,-4.23782220772093,
-322.547953073021)) ;
#39991=CARTESIAN_POINT('Ctrl Pts',(-18.1514627025081,-3.91513270021438,
-322.552041882715)) ;
#39992=CARTESIAN_POINT('Ctrl Pts',(-18.3199592136442,-3.06035354488316,
-322.562750321654)) ;
#39993=CARTESIAN_POINT('Ctrl Pts',(-18.4012883306582,-2.5257192497463,-322.569330244433)) ;
#39994=CARTESIAN_POINT('Ctrl Pts',(-18.4756697719667,-1.83516943608711,
-322.577923842941)) ;
#39995=CARTESIAN_POINT('Ctrl Pts',(-18.4902578423361,-1.68183983734956,
-322.579837267822)) ;
#39996=CARTESIAN_POINT('Ctrl Pts',(-18.5213440831971,-1.30549409996041,
-322.584553638139)) ;
#39997=CARTESIAN_POINT('Ctrl Pts',(-18.5357241108584,-1.08232754789527,
-322.587367592958)) ;
#39998=CARTESIAN_POINT('Ctrl Pts',(-18.5522767319188,-0.724933192378983,
-322.591910955447)) ;
#39999=CARTESIAN_POINT('Ctrl Pts',(-18.5570310056149,-0.590847073819983,
-322.593623752261)) ;
#40000=CARTESIAN_POINT('Ctrl Pts',(-18.5634198433313,-0.331216232653277,
-322.596957510338)) ;
#40001=CARTESIAN_POINT('Ctrl Pts',(-18.5652351146783,-0.205683145668503,
-322.598577208613)) ;
#40002=CARTESIAN_POINT('Ctrl Pts',(-18.5665551160946,0.100111914086229,
-322.602542310271)) ;
#40003=CARTESIAN_POINT('Ctrl Pts',(-18.5647080663818,0.280366782065616,
-322.604896206454)) ;
#40004=CARTESIAN_POINT('Ctrl Pts',(-18.5507578581033,0.84254292289514,-322.612287715341)) ;
#40005=CARTESIAN_POINT('Ctrl Pts',(-18.5294896603066,1.22413537569122,-322.617379052172)) ;
#40006=CARTESIAN_POINT('Ctrl Pts',(-18.4874892441675,1.70822057316831,-322.623899669589)) ;
#40007=CARTESIAN_POINT('Ctrl Pts',(-18.4776488158167,1.81156570632273,-322.625295162937)) ;
#40008=CARTESIAN_POINT('Ctrl Pts',(-18.4230214451507,2.33840321713817,-322.632422301014)) ;
#40009=CARTESIAN_POINT('Ctrl Pts',(-18.3645400967907,2.76034706622736,-322.63817689996)) ;
#40010=CARTESIAN_POINT('Ctrl Pts',(-18.2530211510424,3.40183153295329,-322.646866894112)) ;
#40011=CARTESIAN_POINT('Ctrl Pts',(-18.2104047343149,3.62303721675657,-322.649852002231)) ;
#40012=CARTESIAN_POINT('Ctrl Pts',(-18.1457633707265,3.92852901673376,-322.653935055867)) ;
#40013=CARTESIAN_POINT('Ctrl Pts',(-18.127154898035,4.01351764341147,-322.655066678312)) ;
#40014=CARTESIAN_POINT('Ctrl Pts',(-18.0948724830815,4.15615191125085,-322.656956795723)) ;
#40015=CARTESIAN_POINT('Ctrl Pts',(-18.0815187992598,4.21386839063102,-322.657719030513)) ;
#40016=CARTESIAN_POINT('Ctrl Pts',(-18.0483968686338,4.35396918431943,-322.659562958909)) ;
#40017=CARTESIAN_POINT('Ctrl Pts',(-18.0283405374,4.43628388188943,-322.660641228985)) ;
#40018=CARTESIAN_POINT('Ctrl Pts',(-17.9607132778176,4.70580342257276,-322.664158898713)) ;
#40019=CARTESIAN_POINT('Ctrl Pts',(-17.9107842774774,4.89240371451056,-322.666574014534)) ;
#40020=CARTESIAN_POINT('Ctrl Pts',(-17.7797327754401,5.35325905982929,-322.672520734322)) ;
#40021=CARTESIAN_POINT('Ctrl Pts',(-17.6951678514747,5.62648337880519,-322.676030711984)) ;
#40022=CARTESIAN_POINT('Ctrl Pts',(-17.4584889336851,6.33296410468003,-322.685160631419)) ;
#40023=CARTESIAN_POINT('Ctrl Pts',(-17.2965556492303,6.76272375520635,-322.6907713178)) ;
#40024=CARTESIAN_POINT('Ctrl Pts',(-17.0641872680774,7.31628079220495,-322.698214354166)) ;
#40025=CARTESIAN_POINT('Ctrl Pts',(-17.008030176082,7.44589559590484,-322.699972621004)) ;
#40026=CARTESIAN_POINT('Ctrl Pts',(-16.8643437953347,7.76742531099051,-322.704378220408)) ;
#40027=CARTESIAN_POINT('Ctrl Pts',(-16.7750128932203,7.95851304079422,-322.707036124417)) ;
#40028=CARTESIAN_POINT('Ctrl Pts',(-16.6245439396819,8.26658603701062,-322.711393764484)) ;
#40029=CARTESIAN_POINT('Ctrl Pts',(-16.5653802453157,8.38451448669527,-322.713079397315)) ;
#40030=CARTESIAN_POINT('Ctrl Pts',(-16.4468822967459,8.61456035355865,-322.716403451)) ;
#40031=CARTESIAN_POINT('Ctrl Pts',(-16.3876459925431,8.72672023939676,-322.718041091183)) ;
#40032=CARTESIAN_POINT('Ctrl Pts',(-16.2374820082116,9.00412393773313,-322.72213442688)) ;
#40033=CARTESIAN_POINT('Ctrl Pts',(-16.1451769541271,9.16860571733807,-322.724599998984)) ;
#40034=CARTESIAN_POINT('Ctrl Pts',(-15.8701686067569,9.64161830692855,-322.731800958927)) ;
#40035=CARTESIAN_POINT('Ctrl Pts',(-15.6810142629751,9.94629810015572,-322.736579492333)) ;
#40036=CARTESIAN_POINT('Ctrl Pts',(-15.4268495051036,10.330402960371,-322.742759221398)) ;
#40037=CARTESIAN_POINT('Ctrl Pts',(-15.3698414915035,10.4150316126359,-322.744130638706)) ;
#40038=CARTESIAN_POINT('Ctrl Pts',(-15.0226495234136,10.9213805428511,-322.752390816278)) ;
#40039=CARTESIAN_POINT('Ctrl Pts',(-14.7158227035902,11.3314215368165,-322.759316801468)) ;
#40040=CARTESIAN_POINT('Ctrl Pts',(-14.2862892125413,11.8585276964675,-322.768340212243)) ;
#40041=CARTESIAN_POINT('Ctrl Pts',(-14.1783697860248,11.9873503731716,-322.770554904133)) ;
#40042=CARTESIAN_POINT('Ctrl Pts',(-14.0172679661198,12.1744369378905,-322.773774508957)) ;
#40043=CARTESIAN_POINT('Ctrl Pts',(-13.9654395321194,12.2338552666865,-322.774797529725)) ;
#40044=CARTESIAN_POINT('Ctrl Pts',(-13.8690045020727,12.3430010826833,-322.776676102596)) ;
#40045=CARTESIAN_POINT('Ctrl Pts',(-13.8245051064762,12.3928213154934,-322.777533184753)) ;
#40046=CARTESIAN_POINT('Ctrl Pts',(-13.7232480059677,12.504961758982,-322.77946239842)) ;
#40047=CARTESIAN_POINT('Ctrl Pts',(-13.6663327872064,12.5671378046869,-322.780532145115)) ;
#40048=CARTESIAN_POINT('Ctrl Pts',(-13.4180895795675,12.834646010466,-322.785140130186)) ;
#40049=CARTESIAN_POINT('Ctrl Pts',(-13.2225424483544,13.0360131186499,-322.788623403675)) ;
#40050=CARTESIAN_POINT('Ctrl Pts',(-12.7262919564699,13.5243746565147,-322.797204400396)) ;
#40051=CARTESIAN_POINT('Ctrl Pts',(-12.4203739193012,13.8058512613495,-322.802272422524)) ;
#40052=CARTESIAN_POINT('Ctrl Pts',(-11.8660443144664,14.2825431945862,-322.811249257289)) ;
#40053=CARTESIAN_POINT('Ctrl Pts',(-11.6216155270353,14.4821303648834,-322.815141181741)) ;
#40054=CARTESIAN_POINT('Ctrl Pts',(-11.1850639078728,14.8204219248919,-322.822028206075)) ;
#40055=CARTESIAN_POINT('Ctrl Pts',(-10.9951508941971,14.9618587470929,-322.825003840728)) ;
#40056=CARTESIAN_POINT('Ctrl Pts',(-10.6915989894363,15.1790260887002,-322.829739708169)) ;
#40057=CARTESIAN_POINT('Ctrl Pts',(-10.5797409533026,15.2572016846858,-322.831480565525)) ;
#40058=CARTESIAN_POINT('Ctrl Pts',(-10.362990608877,15.4051547558922,-322.834847136696)) ;
#40059=CARTESIAN_POINT('Ctrl Pts',(-10.2582298959153,15.4751118497351,-322.836471315908)) ;
#40060=CARTESIAN_POINT('Ctrl Pts',(-10.0066288968964,15.6394483378442,-322.840365630701)) ;
#40061=CARTESIAN_POINT('Ctrl Pts',(-9.85915372314473,15.7328336264385,-322.84264317811)) ;
#40062=CARTESIAN_POINT('Ctrl Pts',(-9.11485571303427,16.1895678359832,-322.854110567979)) ;
#40063=CARTESIAN_POINT('Ctrl Pts',(-8.49917436234268,16.5210995062818,-322.863533905941)) ;
#40064=CARTESIAN_POINT('Ctrl Pts',(-7.60586537404308,16.9389481578567,-322.876810365956)) ;
#40065=CARTESIAN_POINT('Ctrl Pts',(-7.34265633256373,17.0546929343031,-322.880672368199)) ;
#40066=CARTESIAN_POINT('Ctrl Pts',(-6.91016937762621,17.2330081523047,-322.886889241106)) ;
#40067=CARTESIAN_POINT('Ctrl Pts',(-6.74248030187543,17.299305488436,-322.889268699919)) ;
#40068=CARTESIAN_POINT('Ctrl Pts',(-6.49828116716997,17.3917615801095,-322.892676208916)) ;
#40069=CARTESIAN_POINT('Ctrl Pts',(-6.42252428897695,17.4198797575881,-322.893725346132)) ;
#40070=CARTESIAN_POINT('Ctrl Pts',(-6.28423683014801,17.4701822738495,-322.895624393359)) ;
#40071=CARTESIAN_POINT('Ctrl Pts',(-6.22176647166556,17.4925276385599,-322.896476179755)) ;
#40072=CARTESIAN_POINT('Ctrl Pts',(-6.06724603148982,17.5468664311816,-322.898568855612)) ;
#40073=CARTESIAN_POINT('Ctrl Pts',(-5.97506126370977,17.5784708918308,-322.899805086393)) ;
#40074=CARTESIAN_POINT('Ctrl Pts',(-5.5592434858207,17.7173802309106,-322.905334570043)) ;
#40075=CARTESIAN_POINT('Ctrl Pts',(-5.23293966112374,17.8164837713082,-322.90954787855)) ;
#40076=CARTESIAN_POINT('Ctrl Pts',(-4.82064247999461,17.9294002018915,-322.914800254231)) ;
#40077=CARTESIAN_POINT('Ctrl Pts',(-4.73703437413505,17.9516709769095,-322.91586165429)) ;
#40078=CARTESIAN_POINT('Ctrl Pts',(-4.19474242517839,18.0920695068885,-322.922728225468)) ;
#40079=CARTESIAN_POINT('Ctrl Pts',(-3.73183619769794,18.1931921733634,-322.928512400127)) ;
#40080=CARTESIAN_POINT('Ctrl Pts',(-2.96958324878344,18.3293884416981,-322.938108410506)) ;
#40081=CARTESIAN_POINT('Ctrl Pts',(-2.67235459758366,18.3750762084813,-322.941866472777)) ;
#40082=CARTESIAN_POINT('Ctrl Pts',(-2.22864922231542,18.432285369773,-322.947526381345)) ;
#40083=CARTESIAN_POINT('Ctrl Pts',(-2.0829330922385,18.4493200677167,-322.949392924369)) ;
#40084=CARTESIAN_POINT('Ctrl Pts',(-1.82608446140126,18.47626475877,-322.952698605503)) ;
#40085=CARTESIAN_POINT('Ctrl Pts',(-1.71503582873146,18.4869033633402,-322.954132920835)) ;
#40086=CARTESIAN_POINT('Ctrl Pts',(-1.45498158596716,18.5094535542963,-322.957504291364)) ;
#40087=CARTESIAN_POINT('Ctrl Pts',(-1.30591466942753,18.5205677310935,-322.959446406053)) ;
#40088=CARTESIAN_POINT('Ctrl Pts',(-0.836857992938834,18.5498486492047,
-322.965587609346)) ;
#40089=CARTESIAN_POINT('Ctrl Pts',(-0.516523333184205,18.561530623166,-322.969826542955)) ;
#40090=CARTESIAN_POINT('Ctrl Pts',(-0.0116220883004283,18.5668624426045,
-322.976562153599)) ;
#40091=CARTESIAN_POINT('Ctrl Pts',(0.172822257716258,18.5660617366694,-322.979033883032)) ;
#40092=CARTESIAN_POINT('Ctrl Pts',(0.828910724535513,18.5534357281749,-322.987851412228)) ;
#40093=CARTESIAN_POINT('Ctrl Pts',(1.30007993527823,18.526382870547,-322.99423455782)) ;
#40094=CARTESIAN_POINT('Ctrl Pts',(1.93355269242442,18.4657240678223,-323.002735719634)) ;
#40095=CARTESIAN_POINT('Ctrl Pts',(2.09718390716215,18.4478565460352,-323.004923786074)) ;
#40096=CARTESIAN_POINT('Ctrl Pts',(2.38375399823455,18.4127027462809,-323.008730791201)) ;
#40097=CARTESIAN_POINT('Ctrl Pts',(2.50679751352192,18.3963548522265,-323.010357257756)) ;
#40098=CARTESIAN_POINT('Ctrl Pts',(2.69979621813662,18.368740251823,-323.012890868477)) ;
#40099=CARTESIAN_POINT('Ctrl Pts',(2.76986655090538,18.3583048609993,-323.013807070801)) ;
#40100=CARTESIAN_POINT('Ctrl Pts',(2.90159980068149,18.3379147986977,-323.015521533172)) ;
#40101=CARTESIAN_POINT('Ctrl Pts',(2.96327554104603,18.3280495047162,-323.016320920473)) ;
#40102=CARTESIAN_POINT('Ctrl Pts',(3.13917304822823,18.2990028774615,-323.018592715469)) ;
#40103=CARTESIAN_POINT('Ctrl Pts',(3.25326679488404,18.2790636784316,-323.020056609989)) ;
#40104=CARTESIAN_POINT('Ctrl Pts',(3.59113255560094,18.2167541878368,-323.024371717465)) ;
#40105=CARTESIAN_POINT('Ctrl Pts',(3.81431994302679,18.1713326385624,-323.027196361659)) ;
#40106=CARTESIAN_POINT('Ctrl Pts',(4.61240152963709,17.9935608149586,-323.037277322273)) ;
#40107=CARTESIAN_POINT('Ctrl Pts',(5.18174798887874,17.8379362034796,-323.044442918194)) ;
#40108=CARTESIAN_POINT('Ctrl Pts',(5.89538272484891,17.6058153504855,-323.053719476534)) ;
#40109=CARTESIAN_POINT('Ctrl Pts',(6.04739663767838,17.5541808541518,-323.055712094674)) ;
#40110=CARTESIAN_POINT('Ctrl Pts',(6.4154111264272,17.4238297923769,-323.060584527398)) ;
#40111=CARTESIAN_POINT('Ctrl Pts',(6.63065610970241,17.3430603940443,-323.063475520547)) ;
#40112=CARTESIAN_POINT('Ctrl Pts',(6.97008384732953,17.2084493002973,-323.06811062586)) ;
#40113=CARTESIAN_POINT('Ctrl Pts',(7.09527350963028,17.1572110180726,-323.06983683138)) ;
#40114=CARTESIAN_POINT('Ctrl Pts',(7.33638888977303,17.0554357037165,-323.073195283766)) ;
#40115=CARTESIAN_POINT('Ctrl Pts',(7.45238031752238,17.0050732587243,-323.074826230352)) ;
#40116=CARTESIAN_POINT('Ctrl Pts',(7.70463106536363,16.8924716143047,-323.078407255877)) ;
#40117=CARTESIAN_POINT('Ctrl Pts',(7.84066994099358,16.8297603037657,-323.080360553414)) ;
#40118=CARTESIAN_POINT('Ctrl Pts',(8.64707379969398,16.4461237104936,-323.092070081746)) ;
#40119=CARTESIAN_POINT('Ctrl Pts',(9.29843316531179,16.0868269538081,-323.102103331319)) ;
#40120=CARTESIAN_POINT('Ctrl Pts',(10.1564249615511,15.5439879566535,-323.11576563641)) ;
#40121=CARTESIAN_POINT('Ctrl Pts',(10.3831293834222,15.3934776481392,-323.119417174517)) ;
#40122=CARTESIAN_POINT('Ctrl Pts',(10.7494435716941,15.1385044954508,-323.125344381295)) ;
#40123=CARTESIAN_POINT('Ctrl Pts',(10.8910351422731,15.036961434136,-323.127642137074)) ;
#40124=CARTESIAN_POINT('Ctrl Pts',(11.0954029584469,14.8859970604822,-323.130956701801)) ;
#40125=CARTESIAN_POINT('Ctrl Pts',(11.1593226259447,14.8381398378867,-323.131993096389)) ;
#40126=CARTESIAN_POINT('Ctrl Pts',(11.2759435874274,14.7496448798731,-323.133881892296)) ;
#40127=CARTESIAN_POINT('Ctrl Pts',(11.3287387866487,14.7091333995547,-323.134736002419)) ;
#40128=CARTESIAN_POINT('Ctrl Pts',(11.4596436746655,14.6075629498738,-323.136852257152)) ;
#40129=CARTESIAN_POINT('Ctrl Pts',(11.5374842718662,14.5461604969419,-323.138109469561)) ;
#40130=CARTESIAN_POINT('Ctrl Pts',(11.880929743985,14.2707515833488,-323.143659593439)) ;
#40131=CARTESIAN_POINT('Ctrl Pts',(12.1410998304265,14.050072537942,-323.14787341054)) ;
#40132=CARTESIAN_POINT('Ctrl Pts',(12.7024345516268,13.5467017464953,-323.157136124032)) ;
#40133=CARTESIAN_POINT('Ctrl Pts',(13.0005452478334,13.2608746024258,-323.162172618686)) ;
#40134=CARTESIAN_POINT('Ctrl Pts',(13.4834154063907,12.7659551212048,-323.170682850408)) ;
#40135=CARTESIAN_POINT('Ctrl Pts',(13.6734401443441,12.562210611947,-323.174130195803)) ;
#40136=CARTESIAN_POINT('Ctrl Pts',(14.0039133877789,12.1914913359547,-323.180337189452)) ;
#40137=CARTESIAN_POINT('Ctrl Pts',(14.1461393644204,12.02617112833,-323.183082937777)) ;
#40138=CARTESIAN_POINT('Ctrl Pts',(14.3704908693923,11.755901975186,-323.187545087618)) ;
#40139=CARTESIAN_POINT('Ctrl Pts',(14.4544564537656,11.6525073542921,-323.189245993398)) ;
#40140=CARTESIAN_POINT('Ctrl Pts',(14.6157098962865,11.4495158665365,-323.19257477718)) ;
#40141=CARTESIAN_POINT('Ctrl Pts',(14.6931103241828,11.3500175461696,-323.194201596378)) ;
#40142=CARTESIAN_POINT('Ctrl Pts',(14.8807624113691,11.1036539695857,-323.198218492017)) ;
#40143=CARTESIAN_POINT('Ctrl Pts',(14.9898597613537,10.9559265055322,-323.200617615748)) ;
#40144=CARTESIAN_POINT('Ctrl Pts',(15.4695628481123,10.2857848395632,-323.211455851184)) ;
#40145=CARTESIAN_POINT('Ctrl Pts',(15.8151758419385,9.74602236574991,-323.220081414026)) ;
#40146=CARTESIAN_POINT('Ctrl Pts',(16.2866283163094,8.91838441015143,-323.232909755593)) ;
#40147=CARTESIAN_POINT('Ctrl Pts',(16.4341983302619,8.64343496419874,-323.237106618175)) ;
#40148=CARTESIAN_POINT('Ctrl Pts',(16.6601418906165,8.19573522806367,-323.243777626614)) ;
#40149=CARTESIAN_POINT('Ctrl Pts',(16.7429196169837,8.02527548860272,-323.246280497556)) ;
#40150=CARTESIAN_POINT('Ctrl Pts',(16.857842541274,7.77910021333865,-323.249827549817)) ;
#40151=CARTESIAN_POINT('Ctrl Pts',(16.8921165199983,7.70439191473494,-323.250895175483)) ;
#40152=CARTESIAN_POINT('Ctrl Pts',(16.9530631418285,7.56918231525463,-323.252809870452)) ;
#40153=CARTESIAN_POINT('Ctrl Pts',(16.9799107602422,7.50876164122818,-323.253659055251)) ;
#40154=CARTESIAN_POINT('Ctrl Pts',(17.0446369766174,7.36097259323369,-323.255721160738)) ;
#40155=CARTESIAN_POINT('Ctrl Pts',(17.0821672440496,7.27345375091314,-323.256929781855)) ;
#40156=CARTESIAN_POINT('Ctrl Pts',(17.2345268554031,6.91047369566122,-323.261897793557)) ;
#40157=CARTESIAN_POINT('Ctrl Pts',(17.3433797284869,6.63255177007683,-323.265596458817)) ;
#40158=CARTESIAN_POINT('Ctrl Pts',(17.6398799022102,5.81824343138718,-323.276265437195)) ;
#40159=CARTESIAN_POINT('Ctrl Pts',(17.8096636060615,5.27571823362761,-323.28317350547)) ;
#40160=CARTESIAN_POINT('Ctrl Pts',(18.0125813401712,4.50486688160747,-323.293030837852)) ;
#40161=CARTESIAN_POINT('Ctrl Pts',(18.0667611545328,4.28241209096131,-323.29587885209)) ;
#40162=CARTESIAN_POINT('Ctrl Pts',(18.1584523714035,3.8731616642823,-323.301140627959)) ;
#40163=CARTESIAN_POINT('Ctrl Pts',(18.1972293203258,3.68668125803792,-323.303546546329)) ;
#40164=CARTESIAN_POINT('Ctrl Pts',(18.2573364685599,3.37352269437296,-323.307606043079)) ;
#40165=CARTESIAN_POINT('Ctrl Pts',(18.2802336043302,3.24716023795198,-323.309249253836)) ;
#40166=CARTESIAN_POINT('Ctrl Pts',(18.3213505008205,3.00601396478791,-323.312395933714)) ;
#40167=CARTESIAN_POINT('Ctrl Pts',(18.3398070738416,2.89127663546369,-323.313897764518)) ;
#40168=CARTESIAN_POINT('Ctrl Pts',(18.3862593058974,2.58413778391364,-323.317930746195)) ;
#40169=CARTESIAN_POINT('Ctrl Pts',(18.4123119416186,2.39145732258099,-323.320474230439)) ;
#40170=CARTESIAN_POINT('Ctrl Pts',(18.4772532420006,1.84687371282489,-323.327698343762)) ;
#40171=CARTESIAN_POINT('Ctrl Pts',(18.5091097260421,1.49421755782957,-323.332419090114)) ;
#40172=CARTESIAN_POINT('Ctrl Pts',(18.5617689159865,0.638885677969979,-323.343919950841)) ;
#40173=CARTESIAN_POINT('Ctrl Pts',(18.5722638043924,0.135855972020733,-323.35072946396)) ;
#40174=CARTESIAN_POINT('Ctrl Pts',(18.5599214427197,-0.488440993619338,
-323.359075417064)) ;
#40175=CARTESIAN_POINT('Ctrl Pts',(18.5563279569996,-0.609878152566911,
-323.360693555459)) ;
#40176=CARTESIAN_POINT('Ctrl Pts',(18.5494702386873,-0.783850857382472,
-323.363000534812)) ;
#40177=CARTESIAN_POINT('Ctrl Pts',(18.5471741332696,-0.836420874962716,
-323.363696175323)) ;
#40178=CARTESIAN_POINT('Ctrl Pts',(18.5446545937399,-0.88897997805457,-323.364389984898)) ;
#40179=CARTESIAN_POINT('Origin',(0.,0.,-315.477129595899)) ;
#40180=CARTESIAN_POINT('',(18.544654593745,-0.888979977948519,-325.159020379883)) ;
#40181=CARTESIAN_POINT('',(18.544654593744,-0.888979977969434,-324.862668413757)) ;
#40182=CARTESIAN_POINT('',(18.544654593745,-0.888979977948782,-315.477129595899)) ;
#40183=CARTESIAN_POINT('Ctrl Pts',(18.544654593745,-0.888979977948194,-325.159020379883)) ;
#40184=CARTESIAN_POINT('Ctrl Pts',(18.5446586219495,-0.888895947190053,
-325.159019247604)) ;
#40185=CARTESIAN_POINT('Ctrl Pts',(18.5446626495217,-0.888811916393853,
-325.159018115291)) ;
#40186=CARTESIAN_POINT('Ctrl Pts',(18.5501207282953,-0.774920754442528,
-325.157483483499)) ;
#40187=CARTESIAN_POINT('Ctrl Pts',(18.5545270287366,-0.661065782942734,
-325.155951557284)) ;
#40188=CARTESIAN_POINT('Ctrl Pts',(18.5668366567267,-0.243576615309611,
-325.15034869941)) ;
#40189=CARTESIAN_POINT('Ctrl Pts',(18.568336752981,0.0601988172090561,-325.146299308515)) ;
#40190=CARTESIAN_POINT('Ctrl Pts',(18.5605105695105,0.459437238522425,-325.141065491681)) ;
#40191=CARTESIAN_POINT('Ctrl Pts',(18.5578993314717,0.554984340332674,-325.139819627603)) ;
#40192=CARTESIAN_POINT('Ctrl Pts',(18.5522326295111,0.716616868973615,-325.137725830194)) ;
#40193=CARTESIAN_POINT('Ctrl Pts',(18.5495615709723,0.782713761614237,-325.136873596225)) ;
#40194=CARTESIAN_POINT('Ctrl Pts',(18.5427902246401,0.930670564738783,-325.134975234847)) ;
#40195=CARTESIAN_POINT('Ctrl Pts',(18.5385010107146,1.01252027927148,-325.133931225173)) ;
#40196=CARTESIAN_POINT('Ctrl Pts',(18.5225937283258,1.28192521596375,-325.130511636973)) ;
#40197=CARTESIAN_POINT('Ctrl Pts',(18.5086701834537,1.46933282498183,-325.128159473866)) ;
#40198=CARTESIAN_POINT('Ctrl Pts',(18.4644513987463,1.96295856367827,-325.122002126026)) ;
#40199=CARTESIAN_POINT('Ctrl Pts',(18.4293845340087,2.26869080337882,-325.118226813985)) ;
#40200=CARTESIAN_POINT('Ctrl Pts',(18.29520119118,3.22741616193632,-325.106365715861)) ;
#40201=CARTESIAN_POINT('Ctrl Pts',(18.1688376500615,3.8760726501937,-325.09829193675)) ;
#40202=CARTESIAN_POINT('Ctrl Pts',(17.9649544354914,4.68897527553325,-325.087755749685)) ;
#40203=CARTESIAN_POINT('Ctrl Pts',(17.9192521112493,4.86070783313849,-325.08550709052)) ;
#40204=CARTESIAN_POINT('Ctrl Pts',(17.8368299731006,5.15344323358092,-325.081630712099)) ;
#40205=CARTESIAN_POINT('Ctrl Pts',(17.8013264295623,5.27477562989638,-325.080011206072)) ;
#40206=CARTESIAN_POINT('Ctrl Pts',(17.7252528722859,5.52523549828796,-325.076640536377)) ;
#40207=CARTESIAN_POINT('Ctrl Pts',(17.6845044116812,5.65430104833426,-325.074888245983)) ;
#40208=CARTESIAN_POINT('Ctrl Pts',(17.5706100509652,6.00176698015689,-325.070128839152)) ;
#40209=CARTESIAN_POINT('Ctrl Pts',(17.4948055253037,6.2192703569369,-325.067104263885)) ;
#40210=CARTESIAN_POINT('Ctrl Pts',(17.3591704454147,6.58632068260151,-325.061926493004)) ;
#40211=CARTESIAN_POINT('Ctrl Pts',(17.3014048055989,6.73660228565294,-325.059785319124)) ;
#40212=CARTESIAN_POINT('Ctrl Pts',(17.021516369721,7.43739675538367,-325.049709254346)) ;
#40213=CARTESIAN_POINT('Ctrl Pts',(16.7750281396525,7.97780161750594,-325.041661020433)) ;
#40214=CARTESIAN_POINT('Ctrl Pts',(16.414161209679,8.67798828922514,-325.031113422437)) ;
#40215=CARTESIAN_POINT('Ctrl Pts',(16.3225460237165,8.84910506472168,-325.028527074016)) ;
#40216=CARTESIAN_POINT('Ctrl Pts',(16.1641261509983,9.13416435549494,-325.024221078249)) ;
#40217=CARTESIAN_POINT('Ctrl Pts',(16.0987581958567,9.24888735681717,-325.0224888568)) ;
#40218=CARTESIAN_POINT('Ctrl Pts',(15.9956662993177,9.42541240915578,-325.019830258873)) ;
#40219=CARTESIAN_POINT('Ctrl Pts',(15.958795300298,9.48770741661333,-325.018893380711)) ;
#40220=CARTESIAN_POINT('Ctrl Pts',(15.885552200875,9.60981953095132,-325.017060776327)) ;
#40221=CARTESIAN_POINT('Ctrl Pts',(15.8492042401821,9.66964968866288,-325.016164782777)) ;
#40222=CARTESIAN_POINT('Ctrl Pts',(15.7497347874064,9.83131260141312,-325.013747138673)) ;
#40223=CARTESIAN_POINT('Ctrl Pts',(15.6859645031338,9.93274237134299,-325.012233891678)) ;
#40224=CARTESIAN_POINT('Ctrl Pts',(15.5365574878551,10.1653539475783,-325.008764344738)) ;
#40225=CARTESIAN_POINT('Ctrl Pts',(15.4502332000911,10.2960834118683,-325.006815022515)) ;
#40226=CARTESIAN_POINT('Ctrl Pts',(15.1239853337283,10.7768092890646,-324.999623897708)) ;
#40227=CARTESIAN_POINT('Ctrl Pts',(14.8737389543412,11.119642137153,-324.994446927006)) ;
#40228=CARTESIAN_POINT('Ctrl Pts',(14.5814632262791,11.4925138398334,-324.988638362559)) ;
#40229=CARTESIAN_POINT('Ctrl Pts',(14.5508047722516,11.5313062858068,-324.988031877881)) ;
#40230=CARTESIAN_POINT('Ctrl Pts',(14.2277943107438,11.9366752607788,-324.981669927358)) ;
#40231=CARTESIAN_POINT('Ctrl Pts',(13.9218109530843,12.292173348847,-324.975875796179)) ;
#40232=CARTESIAN_POINT('Ctrl Pts',(13.4999940366237,12.7462713621953,-324.968069734093)) ;
#40233=CARTESIAN_POINT('Ctrl Pts',(13.3959442022042,12.85558055762,-324.96615832901)) ;
#40234=CARTESIAN_POINT('Ctrl Pts',(13.2021201219743,13.0542932135564,-324.962620763335)) ;
#40235=CARTESIAN_POINT('Ctrl Pts',(13.1127410878124,13.1440696943821,-324.960998181207)) ;
#40236=CARTESIAN_POINT('Ctrl Pts',(12.9264000006235,13.3274469657149,-324.957632171361)) ;
#40237=CARTESIAN_POINT('Ctrl Pts',(12.8293234681424,13.4209209402564,-324.955887733289)) ;
#40238=CARTESIAN_POINT('Ctrl Pts',(12.5660212408701,13.6689844007998,-324.951180109024)) ;
#40239=CARTESIAN_POINT('Ctrl Pts',(12.3979640630761,13.8215958258115,-324.948200138307)) ;
#40240=CARTESIAN_POINT('Ctrl Pts',(12.1086208105135,14.0748219111802,-324.943114343732)) ;
#40241=CARTESIAN_POINT('Ctrl Pts',(11.9887752409198,14.1770440468635,-324.941020420206)) ;
#40242=CARTESIAN_POINT('Ctrl Pts',(11.4322344408434,14.639640583419,-324.931361711411)) ;
#40243=CARTESIAN_POINT('Ctrl Pts',(10.9804982276953,14.9814457691134,-324.923693041859)) ;
#40244=CARTESIAN_POINT('Ctrl Pts',(10.2658631159338,15.4724621671584,-324.912063395682)) ;
#40245=CARTESIAN_POINT('Ctrl Pts',(10.0137676923007,15.636799170095,-324.90805274844)) ;
#40246=CARTESIAN_POINT('Ctrl Pts',(9.67668035855467,15.8450448459758,-324.902859757055)) ;
#40247=CARTESIAN_POINT('Ctrl Pts',(9.59518605848538,15.8945271547578,-324.901617118573)) ;
#40248=CARTESIAN_POINT('Ctrl Pts',(9.45652785951009,15.9772636285781,-324.899526844709)) ;
#40249=CARTESIAN_POINT('Ctrl Pts',(9.39956094901987,16.0108440193366,-324.898674947478)) ;
#40250=CARTESIAN_POINT('Ctrl Pts',(9.27145091723238,16.0854418908666,-324.896774935489)) ;
#40251=CARTESIAN_POINT('Ctrl Pts',(9.20021275689051,16.1262930702718,-324.895728965662)) ;
#40252=CARTESIAN_POINT('Ctrl Pts',(8.96415073459125,16.2595883453578,-324.892294088395)) ;
#40253=CARTESIAN_POINT('Ctrl Pts',(8.79818623455953,16.349988708402,-324.889928880841)) ;
#40254=CARTESIAN_POINT('Ctrl Pts',(8.35587246372056,16.5822304693836,-324.88372289411)) ;
#40255=CARTESIAN_POINT('Ctrl Pts',(8.07729402747451,16.7196977740968,-324.879912538078)) ;
#40256=CARTESIAN_POINT('Ctrl Pts',(7.21584002410261,17.1182338247516,-324.868283524226)) ;
#40257=CARTESIAN_POINT('Ctrl Pts',(6.62283465587795,17.3562765795629,-324.860475030763)) ;
#40258=CARTESIAN_POINT('Ctrl Pts',(5.843287620965,17.6234188149593,-324.85012842599)) ;
#40259=CARTESIAN_POINT('Ctrl Pts',(5.6669368494997,17.6809142166644,-324.847783905352)) ;
#40260=CARTESIAN_POINT('Ctrl Pts',(5.36906210827938,17.7731154764182,-324.843812434282)) ;
#40261=CARTESIAN_POINT('Ctrl Pts',(5.2479916861208,17.809240434949,-324.842195159287)) ;
#40262=CARTESIAN_POINT('Ctrl Pts',(4.99901978426692,17.8807692874505,-324.838862056494)) ;
#40263=CARTESIAN_POINT('Ctrl Pts',(4.8710884173046,17.9160432764322,-324.837145458801)) ;
#40264=CARTESIAN_POINT('Ctrl Pts',(4.53464529951934,18.0049393296381,-324.832620341877)) ;
#40265=CARTESIAN_POINT('Ctrl Pts',(4.32556006620695,18.0563113098255,-324.829797331651)) ;
#40266=CARTESIAN_POINT('Ctrl Pts',(3.84909137267631,18.1646279571872,-324.823343326407)) ;
#40267=CARTESIAN_POINT('Ctrl Pts',(3.58124846766905,18.2193268871801,-324.819700280012)) ;
#40268=CARTESIAN_POINT('Ctrl Pts',(2.96728423410764,18.3306483838568,-324.811337941607)) ;
#40269=CARTESIAN_POINT('Ctrl Pts',(2.62056955508137,18.3834180929022,-324.806606725256)) ;
#40270=CARTESIAN_POINT('Ctrl Pts',(2.17865847696782,18.4379201665148,-324.800613540854)) ;
#40271=CARTESIAN_POINT('Ctrl Pts',(2.08466029269882,18.4487843582694,-324.799340964799)) ;
#40272=CARTESIAN_POINT('Ctrl Pts',(1.67065558293275,18.4934300026517,-324.793750136042)) ;
#40273=CARTESIAN_POINT('Ctrl Pts',(1.34988447362793,18.5196073389262,-324.789454433463)) ;
#40274=CARTESIAN_POINT('Ctrl Pts',(0.93085666052038,18.5428581263998,-324.783950618395)) ;
#40275=CARTESIAN_POINT('Ctrl Pts',(0.833076740527781,18.5475083179144,-324.782674022182)) ;
#40276=CARTESIAN_POINT('Ctrl Pts',(0.668920596993591,18.5540144731446,-324.780546341371)) ;
#40277=CARTESIAN_POINT('Ctrl Pts',(0.602563015113682,18.5562880362072,-324.77969058647)) ;
#40278=CARTESIAN_POINT('Ctrl Pts',(0.455677815184263,18.5605319284449,-324.77780645371)) ;
#40279=CARTESIAN_POINT('Ctrl Pts',(0.375146844164681,18.562334244577,-324.776779948186)) ;
#40280=CARTESIAN_POINT('Ctrl Pts',(0.115963066857499,18.5664475204769,-324.773493748674)) ;
#40281=CARTESIAN_POINT('Ctrl Pts',(-0.0627124239954405,18.5667037546687,
-324.77125506188)) ;
#40282=CARTESIAN_POINT('Ctrl Pts',(-0.524607960403906,18.5606984412463,
-324.765509764544)) ;
#40283=CARTESIAN_POINT('Ctrl Pts',(-0.807731001154924,18.5505339863079,
-324.762028544782)) ;
#40284=CARTESIAN_POINT('Ctrl Pts',(-1.79941751467278,18.492184425519,-324.749849941773)) ;
#40285=CARTESIAN_POINT('Ctrl Pts',(-2.50534814252148,18.4098348306686,-324.741184784979)) ;
#40286=CARTESIAN_POINT('Ctrl Pts',(-3.35796935287776,18.2604139060853,-324.730292626257)) ;
#40287=CARTESIAN_POINT('Ctrl Pts',(-3.51077446870182,18.2316520571646,-324.728324859711)) ;
#40288=CARTESIAN_POINT('Ctrl Pts',(-3.78711653819901,18.1760343587453,-324.724734777685)) ;
#40289=CARTESIAN_POINT('Ctrl Pts',(-3.91077492934762,18.1498296433566,-324.723116796434)) ;
#40290=CARTESIAN_POINT('Ctrl Pts',(-4.16359234592587,18.0935508446481,-324.719784280077)) ;
#40291=CARTESIAN_POINT('Ctrl Pts',(-4.29271619370536,18.0633515995515,-324.718068996332)) ;
#40292=CARTESIAN_POINT('Ctrl Pts',(-4.63006398011498,17.9806317729402,-324.713552471857)) ;
#40293=CARTESIAN_POINT('Ctrl Pts',(-4.83771938331841,17.9258774494145,-324.710736845017)) ;
#40294=CARTESIAN_POINT('Ctrl Pts',(-5.30644125997606,17.7935474734949,-324.70430417337)) ;
#40295=CARTESIAN_POINT('Ctrl Pts',(-5.56684477106812,17.7138050521781,-324.700675205138)) ;
#40296=CARTESIAN_POINT('Ctrl Pts',(-6.15960132947834,17.5179250619453,-324.692309396975)) ;
#40297=CARTESIAN_POINT('Ctrl Pts',(-6.49059479770754,17.3980046514237,-324.687560134686)) ;
#40298=CARTESIAN_POINT('Ctrl Pts',(-6.91427674802556,17.2307282300353,-324.681428923802)) ;
#40299=CARTESIAN_POINT('Ctrl Pts',(-7.01025532549145,17.1919032851968,-324.680036604406)) ;
#40300=CARTESIAN_POINT('Ctrl Pts',(-7.39746459177869,17.0314889076669,-324.674410982087)) ;
#40301=CARTESIAN_POINT('Ctrl Pts',(-7.68589844254006,16.9032855576917,-324.670199910596)) ;
#40302=CARTESIAN_POINT('Ctrl Pts',(-8.05850070316169,16.7261612036311,-324.66479060758)) ;
#40303=CARTESIAN_POINT('Ctrl Pts',(-8.14574970358435,16.6838444010591,-324.663526275409)) ;
#40304=CARTESIAN_POINT('Ctrl Pts',(-8.29208214970525,16.6114498993797,-324.66141218093)) ;
#40305=CARTESIAN_POINT('Ctrl Pts',(-8.35134317255403,16.5817357772064,-324.66055789588)) ;
#40306=CARTESIAN_POINT('Ctrl Pts',(-8.4827396236188,16.5149690901555,-324.658668396748)) ;
#40307=CARTESIAN_POINT('Ctrl Pts',(-8.55479385902869,16.4777600912521,-324.657635150079)) ;
#40308=CARTESIAN_POINT('Ctrl Pts',(-8.78791755769494,16.3554331101089,-324.654298230134)) ;
#40309=CARTESIAN_POINT('Ctrl Pts',(-8.94797872598171,16.2684161536449,-324.652016464265)) ;
#40310=CARTESIAN_POINT('Ctrl Pts',(-9.24104346340062,16.1034583096805,-324.647835494054)) ;
#40311=CARTESIAN_POINT('Ctrl Pts',(-9.37440697152772,16.0261894357702,-324.645931662362)) ;
#40312=CARTESIAN_POINT('Ctrl Pts',(-10.2269894113764,15.5179315783491,-324.633713602122)) ;
#40313=CARTESIAN_POINT('Ctrl Pts',(-10.9172736991398,15.0403009270707,-324.623554436759)) ;
#40314=CARTESIAN_POINT('Ctrl Pts',(-11.6932872480977,14.42169310885,-324.611063023564)) ;
#40315=CARTESIAN_POINT('Ctrl Pts',(-11.81246712061,14.3242388707555,-324.609114186389)) ;
#40316=CARTESIAN_POINT('Ctrl Pts',(-12.0270137055586,14.1443039231261,-324.605547207702)) ;
#40317=CARTESIAN_POINT('Ctrl Pts',(-12.1227786507147,14.0623123943508,-324.603933199599)) ;
#40318=CARTESIAN_POINT('Ctrl Pts',(-12.3179728500818,13.8917161912039,-324.600597109432)) ;
#40319=CARTESIAN_POINT('Ctrl Pts',(-12.4172987861137,13.8030041898748,-324.59887415615)) ;
#40320=CARTESIAN_POINT('Ctrl Pts',(-12.6766463545541,13.5663053169609,-324.594307467427)) ;
#40321=CARTESIAN_POINT('Ctrl Pts',(-12.8350311334094,13.416556126447,-324.591448729686)) ;
#40322=CARTESIAN_POINT('Ctrl Pts',(-13.1896112100128,13.0692823101806,-324.584891052363)) ;
#40323=CARTESIAN_POINT('Ctrl Pts',(-13.3840742423691,12.8700637225103,-324.581179429134)) ;
#40324=CARTESIAN_POINT('Ctrl Pts',(-13.855668897194,12.3646838807002,-324.571912172819)) ;
#40325=CARTESIAN_POINT('Ctrl Pts',(-14.1272057209714,12.0535067977024,-324.566333177034)) ;
#40326=CARTESIAN_POINT('Ctrl Pts',(-14.604387175395,11.4683674374813,-324.556188007992)) ;
#40327=CARTESIAN_POINT('Ctrl Pts',(-14.8132615854392,11.1972701353975,-324.55161468909)) ;
#40328=CARTESIAN_POINT('Ctrl Pts',(-15.0726602483096,10.8406264039178,-324.545829816827)) ;
#40329=CARTESIAN_POINT('Ctrl Pts',(-15.1301563148155,10.760234092299,-324.544540615264)) ;
#40330=CARTESIAN_POINT('Ctrl Pts',(-15.2252644732489,10.6249820955699,-324.542398888305)) ;
#40331=CARTESIAN_POINT('Ctrl Pts',(-15.2632285907929,10.5703725494005,-324.541541540812)) ;
#40332=CARTESIAN_POINT('Ctrl Pts',(-15.3462192787946,10.4496151097457,-324.539662526114)) ;
#40333=CARTESIAN_POINT('Ctrl Pts',(-15.3911132212989,10.3833778669287,-324.538642637158)) ;
#40334=CARTESIAN_POINT('Ctrl Pts',(-15.5329792775945,10.1711247076182,-324.535405471684)) ;
#40335=CARTESIAN_POINT('Ctrl Pts',(-15.6283125154668,10.0240246988668,-324.533208350041)) ;
#40336=CARTESIAN_POINT('Ctrl Pts',(-15.8676704537504,9.64297658818647,-324.527609305558)) ;
#40337=CARTESIAN_POINT('Ctrl Pts',(-16.0086116741577,9.4071417422158,-324.524231262496)) ;
#40338=CARTESIAN_POINT('Ctrl Pts',(-16.5035615075361,8.53559171872297,-324.511940314212)) ;
#40339=CARTESIAN_POINT('Ctrl Pts',(-16.825354108921,7.88234276124894,-324.503068740249)) ;
#40340=CARTESIAN_POINT('Ctrl Pts',(-17.1677953807705,7.07000797839121,-324.491972609439)) ;
#40341=CARTESIAN_POINT('Ctrl Pts',(-17.2258431692104,6.9273759873389,-324.490023281795)) ;
#40342=CARTESIAN_POINT('Ctrl Pts',(-17.3281779123183,6.66668167429108,-324.486455705793)) ;
#40343=CARTESIAN_POINT('Ctrl Pts',(-17.3730493571668,6.54885870116318,-324.484841596037)) ;
#40344=CARTESIAN_POINT('Ctrl Pts',(-17.4628376176707,6.30567460135265,-324.481505606007)) ;
#40345=CARTESIAN_POINT('Ctrl Pts',(-17.5076128291577,6.1802688291551,-324.479782857746)) ;
#40346=CARTESIAN_POINT('Ctrl Pts',(-17.622081813725,5.84843550227691,-324.475217510485)) ;
#40347=CARTESIAN_POINT('Ctrl Pts',(-17.689497652719,5.64124434915855,-324.472359925784)) ;
#40348=CARTESIAN_POINT('Ctrl Pts',(-17.8346597107566,5.16689522803652,-324.465805605824)) ;
#40349=CARTESIAN_POINT('Ctrl Pts',(-17.9100784961249,4.89907962085505,-324.462096207668)) ;
#40350=CARTESIAN_POINT('Ctrl Pts',(-18.0824065841646,4.22983890984074,-324.452831294259)) ;
#40351=CARTESIAN_POINT('Ctrl Pts',(-18.1719964825838,3.82668374190341,-324.447252366751)) ;
#40352=CARTESIAN_POINT('Ctrl Pts',(-18.311232802637,3.08395223328582,-324.437098674596)) ;
#40353=CARTESIAN_POINT('Ctrl Pts',(-18.3650514273055,2.74534060542625,-324.432516874476)) ;
#40354=CARTESIAN_POINT('Ctrl Pts',(-18.4222514714943,2.30757239692762,-324.426725803979)) ;
#40355=CARTESIAN_POINT('Ctrl Pts',(-18.4342577468173,2.20961105430747,-324.425438500317)) ;
#40356=CARTESIAN_POINT('Ctrl Pts',(-18.4530446205108,2.04549865174853,-324.423298893235)) ;
#40357=CARTESIAN_POINT('Ctrl Pts',(-18.4602519435972,1.97939857430754,-324.422441790582)) ;
#40358=CARTESIAN_POINT('Ctrl Pts',(-18.4753580671253,1.83359182870452,-324.420562029993)) ;
#40359=CARTESIAN_POINT('Ctrl Pts',(-18.4830964566858,1.75387003489079,-324.419541164246)) ;
#40360=CARTESIAN_POINT('Ctrl Pts',(-18.5061686803337,1.49903901159186,-324.416296805358)) ;
#40361=CARTESIAN_POINT('Ctrl Pts',(-18.5195317048159,1.32376085735172,-324.414093591029)) ;
#40362=CARTESIAN_POINT('Ctrl Pts',(-18.5474714206386,0.87289823368202,-324.408473257293)) ;
#40363=CARTESIAN_POINT('Ctrl Pts',(-18.5583965602283,0.597130576764395,
-324.405080234962)) ;
#40364=CARTESIAN_POINT('Ctrl Pts',(-18.5757186892474,-0.40390227118912,
-324.392803331715)) ;
#40365=CARTESIAN_POINT('Ctrl Pts',(-18.5457678542622,-1.12913966912419,
-324.383959403295)) ;
#40366=CARTESIAN_POINT('Ctrl Pts',(-18.4581081514156,-2.00412035107501,
-324.37289130985)) ;
#40367=CARTESIAN_POINT('Ctrl Pts',(-18.4408346634734,-2.15728341550672,
-324.370940228323)) ;
#40368=CARTESIAN_POINT('Ctrl Pts',(-18.405964400338,-2.43533910379303,-324.36737051579)) ;
#40369=CARTESIAN_POINT('Ctrl Pts',(-18.3889982929313,-2.56030150306097,
-324.365756041947)) ;
#40370=CARTESIAN_POINT('Ctrl Pts',(-18.3515107117888,-2.8167836395877,-324.362420406641)) ;
#40371=CARTESIAN_POINT('Ctrl Pts',(-18.3308452982443,-2.94827510013788,
-324.36069838872)) ;
#40372=CARTESIAN_POINT('Ctrl Pts',(-18.2726810437337,-3.29407944234658,
-324.356137819817)) ;
#40373=CARTESIAN_POINT('Ctrl Pts',(-18.2328260110372,-3.50797481310281,
-324.353284342207)) ;
#40374=CARTESIAN_POINT('Ctrl Pts',(-18.1595860851892,-3.86597918388449,
-324.34845636185)) ;
#40375=CARTESIAN_POINT('Ctrl Pts',(-18.1282216218701,-4.01047909801559,
-324.346493371257)) ;
#40376=CARTESIAN_POINT('Ctrl Pts',(-17.9834342466204,-4.64109434134236,
-324.337869688728)) ;
#40377=CARTESIAN_POINT('Ctrl Pts',(-17.8521592930299,-5.12289673776954,
-324.331126311901)) ;
#40378=CARTESIAN_POINT('Ctrl Pts',(-17.6824483477044,-5.65946690870653,
-324.323555516011)) ;
#40379=CARTESIAN_POINT('Ctrl Pts',(-17.6629552171256,-5.72001383393836,
-324.322700438641)) ;
#40380=CARTESIAN_POINT('Ctrl Pts',(-17.5411251877826,-6.09186414830413,
-324.31744598544)) ;
#40381=CARTESIAN_POINT('Ctrl Pts',(-17.4308721932401,-6.40051380852478,
-324.313070674569)) ;
#40382=CARTESIAN_POINT('Ctrl Pts',(-17.2775081934495,-6.79644019426209,
-324.307503707819)) ;
#40383=CARTESIAN_POINT('Ctrl Pts',(-17.2418013121382,-6.88652134542935,
-324.306240303337)) ;
#40384=CARTESIAN_POINT('Ctrl Pts',(-17.1804835685987,-7.03774661996558,
-324.304127233201)) ;
#40385=CARTESIAN_POINT('Ctrl Pts',(-17.1552475105334,-7.09904050021906,
-324.303273055965)) ;
#40386=CARTESIAN_POINT('Ctrl Pts',(-17.0983926158861,-7.23505717728028,
-324.30138313462)) ;
#40387=CARTESIAN_POINT('Ctrl Pts',(-17.0666111729221,-7.30971035693333,
-324.300349365266)) ;
#40388=CARTESIAN_POINT('Ctrl Pts',(-16.9617763463394,-7.55155153433974,
-324.29700847943)) ;
#40389=CARTESIAN_POINT('Ctrl Pts',(-16.8867475665012,-7.71787174250962,
-324.294723341542)) ;
#40390=CARTESIAN_POINT('Ctrl Pts',(-16.7436822581327,-8.02293411564987,
-324.290534516993)) ;
#40391=CARTESIAN_POINT('Ctrl Pts',(-16.676341621403,-8.16198490484776,-324.28862621689)) ;
#40392=CARTESIAN_POINT('Ctrl Pts',(-16.2326531562394,-9.04973148786076,
-324.276410256749)) ;
#40393=CARTESIAN_POINT('Ctrl Pts',(-15.8077181648226,-9.77306088105379,
-324.266256755699)) ;
#40394=CARTESIAN_POINT('Ctrl Pts',(-15.2486580630856,-10.5922894917194,
-324.253772645921)) ;
#40395=CARTESIAN_POINT('Ctrl Pts',(-15.1603597817781,-10.7182862715112,
-324.251824985247)) ;
#40396=CARTESIAN_POINT('Ctrl Pts',(-14.9968905508428,-10.9454858624436,
-324.248259439054)) ;
#40397=CARTESIAN_POINT('Ctrl Pts',(-14.9222353598274,-11.047048419009,-324.2466456745)) ;
#40398=CARTESIAN_POINT('Ctrl Pts',(-14.7665680993526,-11.2543640488365,
-324.243309342443)) ;
#40399=CARTESIAN_POINT('Ctrl Pts',(-14.6854403786343,-11.3600213203631,
-324.241585895958)) ;
#40400=CARTESIAN_POINT('Ctrl Pts',(-14.4684654485283,-11.6363912162853,
-324.237015980035)) ;
#40401=CARTESIAN_POINT('Ctrl Pts',(-14.3307343580113,-11.8055980564885,
-324.234154468334)) ;
#40402=CARTESIAN_POINT('Ctrl Pts',(-14.0102986229613,-12.1853902264077,
-324.227588710751)) ;
#40403=CARTESIAN_POINT('Ctrl Pts',(-13.8257685387155,-12.394366718756,-324.223871731209)) ;
#40404=CARTESIAN_POINT('Ctrl Pts',(-13.3564125061291,-12.9023726681295,
-324.214598831097)) ;
#40405=CARTESIAN_POINT('Ctrl Pts',(-13.0661829667452,-13.1962054292246,
-324.209019666932)) ;
#40406=CARTESIAN_POINT('Ctrl Pts',(-12.5197147569701,-13.7137403820609,
-324.198907011125)) ;
#40407=CARTESIAN_POINT('Ctrl Pts',(-12.266663020355,-13.9405492009657,-324.194365985552)) ;
#40408=CARTESIAN_POINT('Ctrl Pts',(-11.9315651479546,-14.2247029034452,
-324.188601636262)) ;
#40409=CARTESIAN_POINT('Ctrl Pts',(-11.8550827840547,-14.2885069827735,
-324.1873022458)) ;
#40410=CARTESIAN_POINT('Ctrl Pts',(-11.726604724349,-14.3939458516107,-324.185149109122)) ;
#40411=CARTESIAN_POINT('Ctrl Pts',(-11.6748917780134,-14.4359217769132,
-324.184290417989)) ;
#40412=CARTESIAN_POINT('Ctrl Pts',(-11.5608798022477,-14.5274531238544,
-324.182415264015)) ;
#40413=CARTESIAN_POINT('Ctrl Pts',(-11.4984857923705,-14.5768878905526,
-324.181400505901)) ;
#40414=CARTESIAN_POINT('Ctrl Pts',(-11.2997286626254,-14.7322929507531,
-324.178200874231)) ;
#40415=CARTESIAN_POINT('Ctrl Pts',(-11.1622037943643,-14.8367627894388,
-324.176035514997)) ;
#40416=CARTESIAN_POINT('Ctrl Pts',(-10.80735536776,-15.0985943436397,-324.170546648979)) ;
#40417=CARTESIAN_POINT('Ctrl Pts',(-10.5880415394942,-15.2531917289847,
-324.167245911931)) ;
#40418=CARTESIAN_POINT('Ctrl Pts',(-9.74330876575939,-15.8216556176582,
-324.154756876079)) ;
#40419=CARTESIAN_POINT('Ctrl Pts',(-9.0963673782391,-16.202251475044,-324.145618227089)) ;
#40420=CARTESIAN_POINT('Ctrl Pts',(-8.28189350385132,-16.6172108619708,
-324.13410222967)) ;
#40421=CARTESIAN_POINT('Ctrl Pts',(-8.13461693476493,-16.6898011987631,
-324.132020975683)) ;
#40422=CARTESIAN_POINT('Ctrl Pts',(-7.87353097874972,-16.8142094815833,
-324.128330219968)) ;
#40423=CARTESIAN_POINT('Ctrl Pts',(-7.76012460251026,-16.8668490437766,
-324.126726717366)) ;
#40424=CARTESIAN_POINT('Ctrl Pts',(-7.5189344068974,-16.975854267733,-324.123314766404)) ;
#40425=CARTESIAN_POINT('Ctrl Pts',(-7.39102875179493,-17.0319316770664,
-324.121504393135)) ;
#40426=CARTESIAN_POINT('Ctrl Pts',(-7.02733059118297,-17.1865186031997,
-324.116353584985)) ;
#40427=CARTESIAN_POINT('Ctrl Pts',(-6.79012029602376,-17.2816105409755,
-324.112990236013)) ;
#40428=CARTESIAN_POINT('Ctrl Pts',(-6.37425972290613,-17.4384345961324,
-324.107093703077)) ;
#40429=CARTESIAN_POINT('Ctrl Pts',(-6.19648916873253,-17.5023915518779,
-324.104573148269)) ;
#40430=CARTESIAN_POINT('Ctrl Pts',(-5.67930316437138,-17.6795934953287,
-324.097250463925)) ;
#40431=CARTESIAN_POINT('Ctrl Pts',(-5.33755120228227,-17.7857543381615,
-324.092423216182)) ;
#40432=CARTESIAN_POINT('Ctrl Pts',(-4.94556263289974,-17.8952041029779,
-324.086944612391)) ;
#40433=CARTESIAN_POINT('Ctrl Pts',(-4.89812668367064,-17.9082459954837,
-324.086282618446)) ;
#40434=CARTESIAN_POINT('Ctrl Pts',(-4.51983041772977,-18.0106380850315,
-324.08101224688)) ;
#40435=CARTESIAN_POINT('Ctrl Pts',(-4.18660496775709,-18.0910002714573,
-324.076422981647)) ;
#40436=CARTESIAN_POINT('Ctrl Pts',(-3.74022423692884,-18.1856571350349,
-324.070418017646)) ;
#40437=CARTESIAN_POINT('Ctrl Pts',(-3.62888810184296,-18.2082007342818,
-324.068932093925)) ;
#40438=CARTESIAN_POINT('Ctrl Pts',(-3.45639137039489,-18.2414832906194,
-324.066651806675)) ;
#40439=CARTESIAN_POINT('Ctrl Pts',(-3.39537207382562,-18.2529395561836,
-324.065849400192)) ;
#40440=CARTESIAN_POINT('Ctrl Pts',(-3.26406129542807,-18.2769116822503,
-324.064132607734)) ;
#40441=CARTESIAN_POINT('Ctrl Pts',(-3.19375273946748,-18.2893285890387,
-324.063219475209)) ;
#40442=CARTESIAN_POINT('Ctrl Pts',(-2.99824571202545,-18.3226945408502,
-324.060695234254)) ;
#40443=CARTESIAN_POINT('Ctrl Pts',(-2.87290127967153,-18.3427656285621,
-324.059093811185)) ;
#40444=CARTESIAN_POINT('Ctrl Pts',(-2.57935373390492,-18.3866879020212,
-324.055373824097)) ;
#40445=CARTESIAN_POINT('Ctrl Pts',(-2.41100939119533,-18.409519046888,-324.053263712518)) ;
#40446=CARTESIAN_POINT('Ctrl Pts',(-1.73937492663051,-18.4912365486306,
-324.044903407833)) ;
#40447=CARTESIAN_POINT('Ctrl Pts',(-1.2340795514919,-18.531818669057,-324.038737813985)) ;
#40448=CARTESIAN_POINT('Ctrl Pts',(-0.356523487429989,-18.5662440326999,
-324.027938598878)) ;
#40449=CARTESIAN_POINT('Ctrl Pts',(0.0150637715096853,-18.5696607071013,
-324.023339099343)) ;
#40450=CARTESIAN_POINT('Ctrl Pts',(0.570407863445169,-18.5580971612075,
-324.016363096674)) ;
#40451=CARTESIAN_POINT('Ctrl Pts',(0.75424625917996,-18.5515349177353,-324.014037447566)) ;
#40452=CARTESIAN_POINT('Ctrl Pts',(1.06389874598875,-18.5358711931867,-324.010087938392)) ;
#40453=CARTESIAN_POINT('Ctrl Pts',(1.18977267314184,-18.5282174632479,-324.008473493907)) ;
#40454=CARTESIAN_POINT('Ctrl Pts',(1.44833023345666,-18.5098502469707,-324.005137830225)) ;
#40455=CARTESIAN_POINT('Ctrl Pts',(1.5809963300354,-18.4989909771302,-324.003415753645)) ;
#40456=CARTESIAN_POINT('Ctrl Pts',(1.9301902670985,-18.4666241673015,-323.998854800968)) ;
#40457=CARTESIAN_POINT('Ctrl Pts',(2.14647637078742,-18.4427351966224,-323.996000993502)) ;
#40458=CARTESIAN_POINT('Ctrl Pts',(2.63769967944871,-18.3797208149829,-323.989457666467)) ;
#40459=CARTESIAN_POINT('Ctrl Pts',(2.91227948003948,-18.3382175971565,-323.985755551813)) ;
#40460=CARTESIAN_POINT('Ctrl Pts',(3.59256440275971,-18.2197265839976,-323.976498301065)) ;
#40461=CARTESIAN_POINT('Ctrl Pts',(3.99682786182519,-18.1353335334041,-323.970919590183)) ;
#40462=CARTESIAN_POINT('Ctrl Pts',(4.73242512880404,-17.9559790356222,-323.960745712935)) ;
#40463=CARTESIAN_POINT('Ctrl Pts',(5.06457753498572,-17.8651360466682,-323.95614379169)) ;
#40464=CARTESIAN_POINT('Ctrl Pts',(5.48825912435923,-17.7364938086253,-323.950336057502)) ;
#40465=CARTESIAN_POINT('Ctrl Pts',(5.58227728303499,-17.7071279776248,-323.949051375214)) ;
#40466=CARTESIAN_POINT('Ctrl Pts',(5.73934250951164,-17.6566946198847,-323.946914693206)) ;
#40467=CARTESIAN_POINT('Ctrl Pts',(5.80251807256303,-17.6360341742374,-323.946057925829)) ;
#40468=CARTESIAN_POINT('Ctrl Pts',(5.94167881458699,-17.5896954250417,-323.944177120832)) ;
#40469=CARTESIAN_POINT('Ctrl Pts',(6.01761114965898,-17.5638631387484,-323.943154894784)) ;
#40470=CARTESIAN_POINT('Ctrl Pts',(6.26006913357981,-17.4796217256306,-323.939900492261)) ;
#40471=CARTESIAN_POINT('Ctrl Pts',(6.42593054189615,-17.4193300126884,-323.937688768271)) ;
#40472=CARTESIAN_POINT('Ctrl Pts',(6.85051227254076,-17.258102266702,-323.932038615105)) ;
#40473=CARTESIAN_POINT('Ctrl Pts',(7.1078731598804,-17.153709563211,-323.928624588892)) ;
#40474=CARTESIAN_POINT('Ctrl Pts',(8.02566353876108,-16.7572258646357,-323.916365743075)) ;
#40475=CARTESIAN_POINT('Ctrl Pts',(8.67126197135678,-16.4324407654209,-323.907558988817)) ;
#40476=CARTESIAN_POINT('Ctrl Pts',(9.42984617922406,-15.9936332031631,-323.896529035393)) ;
#40477=CARTESIAN_POINT('Ctrl Pts',(9.56242512126461,-15.9147204722667,-323.894576072639)) ;
#40478=CARTESIAN_POINT('Ctrl Pts',(9.80158371768117,-15.7683026041225,-323.891004067443)) ;
#40479=CARTESIAN_POINT('Ctrl Pts',(9.90848837761735,-15.7013460699236,-323.889389202079)) ;
#40480=CARTESIAN_POINT('Ctrl Pts',(10.1267311247918,-15.5615396700233,-323.886053941443)) ;
#40481=CARTESIAN_POINT('Ctrl Pts',(10.2379851807161,-15.4885719016366,-323.884332702041)) ;
#40482=CARTESIAN_POINT('Ctrl Pts',(10.5288040314402,-15.2933310829978,-323.879777226237)) ;
#40483=CARTESIAN_POINT('Ctrl Pts',(10.7070235180935,-15.1690915044497,-323.876928126078)) ;
#40484=CARTESIAN_POINT('Ctrl Pts',(11.4262440415811,-14.6487204933647,-323.865199757429)) ;
#40485=CARTESIAN_POINT('Ctrl Pts',(11.9477755915366,-14.226549742773,-323.85613153917)) ;
#40486=CARTESIAN_POINT('Ctrl Pts',(12.6944750198875,-13.5520306840359,-323.842602310485)) ;
#40487=CARTESIAN_POINT('Ctrl Pts',(12.9374764823871,-13.3202452934011,-323.838107943541)) ;
#40488=CARTESIAN_POINT('Ctrl Pts',(13.2537666821861,-13.0017292901879,-323.832201286496)) ;
#40489=CARTESIAN_POINT('Ctrl Pts',(13.3327393016974,-12.9207336700945,-323.830721657337)) ;
#40490=CARTESIAN_POINT('Ctrl Pts',(13.4538467041377,-12.7942312428942,-323.828448641825)) ;
#40491=CARTESIAN_POINT('Ctrl Pts',(13.4965019630739,-12.7492266044238,-323.827647292065)) ;
#40492=CARTESIAN_POINT('Ctrl Pts',(13.5805326517058,-12.6596733233988,-323.826067901992)) ;
#40493=CARTESIAN_POINT('Ctrl Pts',(13.6219163044653,-12.6151334501198,-323.825289707207)) ;
#40494=CARTESIAN_POINT('Ctrl Pts',(13.7126126655071,-12.5165532491704,-323.823582398383)) ;
#40495=CARTESIAN_POINT('Ctrl Pts',(13.7618262672711,-12.4624230854013,-323.82265477762)) ;
#40496=CARTESIAN_POINT('Ctrl Pts',(13.8859207326933,-12.3242998359823,-323.820310740166)) ;
#40497=CARTESIAN_POINT('Ctrl Pts',(13.9603603470932,-12.2399142182297,-323.818899943423)) ;
#40498=CARTESIAN_POINT('Ctrl Pts',(14.1852361017983,-11.9802721105117,-323.814615545179)) ;
#40499=CARTESIAN_POINT('Ctrl Pts',(14.3331731828673,-11.8028805754952,-323.811765421478)) ;
#40500=CARTESIAN_POINT('Ctrl Pts',(14.9774860264629,-11.0003004641634,-323.799117384957)) ;
#40501=CARTESIAN_POINT('Ctrl Pts',(15.4365437439498,-10.3462465354409,-323.789423065738)) ;
#40502=CARTESIAN_POINT('Ctrl Pts',(15.9395618716525,-9.52119262451529,-323.777261028321)) ;
#40503=CARTESIAN_POINT('Ctrl Pts',(16.0250917601493,-9.37652257578823,-323.775132620822)) ;
#40504=CARTESIAN_POINT('Ctrl Pts',(16.1699677823714,-9.12369737218593,-323.771416730385)) ;
#40505=CARTESIAN_POINT('Ctrl Pts',(16.2302219367189,-9.0160749585012,-323.76983611921)) ;
#40506=CARTESIAN_POINT('Ctrl Pts',(16.3489940596022,-8.79888177545719,-323.766647762129)) ;
#40507=CARTESIAN_POINT('Ctrl Pts',(16.4074937707379,-8.68930810660271,-323.765039983652)) ;
#40508=CARTESIAN_POINT('Ctrl Pts',(16.5285631378471,-8.45695497029693,-323.761631974288)) ;
#40509=CARTESIAN_POINT('Ctrl Pts',(16.5908743118414,-8.33404921229807,-323.759830026894)) ;
#40510=CARTESIAN_POINT('Ctrl Pts',(16.8590241651065,-7.79020878450014,-323.751861293062)) ;
#40511=CARTESIAN_POINT('Ctrl Pts',(17.0502527713835,-7.36226371092268,-323.745598039847)) ;
#40512=CARTESIAN_POINT('Ctrl Pts',(17.4441548294995,-6.38284070631251,-323.731398551454)) ;
#40513=CARTESIAN_POINT('Ctrl Pts',(17.6372619262477,-5.82805157360503,-323.723444159015)) ;
#40514=CARTESIAN_POINT('Ctrl Pts',(17.8402192559855,-5.14175142939186,-323.714000003907)) ;
#40515=CARTESIAN_POINT('Ctrl Pts',(17.8753995488649,-5.01807950464265,-323.712314038899)) ;
#40516=CARTESIAN_POINT('Ctrl Pts',(17.9281970815263,-4.8248722302068,-323.709710038425)) ;
#40517=CARTESIAN_POINT('Ctrl Pts',(17.94670078078,-4.75558342738961,-323.708782142463)) ;
#40518=CARTESIAN_POINT('Ctrl Pts',(17.9800914025034,-4.62757836529475,-323.70708006426)) ;
#40519=CARTESIAN_POINT('Ctrl Pts',(17.9950933281718,-4.56889313574603,-323.706304434242)) ;
#40520=CARTESIAN_POINT('Ctrl Pts',(18.0273296059092,-4.44016769866279,-323.704612419135)) ;
#40521=CARTESIAN_POINT('Ctrl Pts',(18.0444435415294,-4.37009830608841,-323.703697425084)) ;
#40522=CARTESIAN_POINT('Ctrl Pts',(18.0865627569399,-4.19318350708098,-323.701400530486)) ;
#40523=CARTESIAN_POINT('Ctrl Pts',(18.1110299393917,-4.08621277771819,-323.700023934776)) ;
#40524=CARTESIAN_POINT('Ctrl Pts',(18.1819948471042,-3.76278821352656,-323.695891215054)) ;
#40525=CARTESIAN_POINT('Ctrl Pts',(18.2255707308513,-3.54571340282537,-323.693156842973)) ;
#40526=CARTESIAN_POINT('Ctrl Pts',(18.4120929858388,-2.5219852308164,-323.680360849551)) ;
#40527=CARTESIAN_POINT('Ctrl Pts',(18.5054305691396,-1.70722583022592,-323.670421853881)) ;
#40528=CARTESIAN_POINT('Ctrl Pts',(18.544655072549,-0.888969989752754,-323.660107772569)) ;
#40529=CARTESIAN_POINT('Ctrl Pts',(18.5446545937399,-0.888979978054576,
-323.364389984898)) ;
#40530=CARTESIAN_POINT('Ctrl Pts',(18.539705026844,-0.992230906915975,-323.365752954944)) ;
#40531=CARTESIAN_POINT('Ctrl Pts',(18.533893193385,-1.09543971499047,-323.36710886668)) ;
#40532=CARTESIAN_POINT('Ctrl Pts',(18.5222615862343,-1.27523458707085,-323.369456552669)) ;
#40533=CARTESIAN_POINT('Ctrl Pts',(18.5168280309002,-1.35184215659057,-323.370452303384)) ;
#40534=CARTESIAN_POINT('Ctrl Pts',(18.5057881537854,-1.49490872800445,-323.372301954481)) ;
#40535=CARTESIAN_POINT('Ctrl Pts',(18.5002987611782,-1.56137536642769,-323.37315711715)) ;
#40536=CARTESIAN_POINT('Ctrl Pts',(18.4852571964577,-1.73227081279554,-323.375346393268)) ;
#40537=CARTESIAN_POINT('Ctrl Pts',(18.4751781861318,-1.8366509812536,-323.376674557344)) ;
#40538=CARTESIAN_POINT('Ctrl Pts',(18.4378377825636,-2.19187121817369,-323.381171357321)) ;
#40539=CARTESIAN_POINT('Ctrl Pts',(18.406347576809,-2.44223890400711,-323.384301769558)) ;
#40540=CARTESIAN_POINT('Ctrl Pts',(18.2846053127072,-3.27302287709881,-323.394652282921)) ;
#40541=CARTESIAN_POINT('Ctrl Pts',(18.1719175349712,-3.84979022566562,-323.401787601913)) ;
#40542=CARTESIAN_POINT('Ctrl Pts',(17.9939349012851,-4.57585804941936,-323.411029059352)) ;
#40543=CARTESIAN_POINT('Ctrl Pts',(17.9537762322332,-4.73097125854654,-323.413017835529)) ;
#40544=CARTESIAN_POINT('Ctrl Pts',(17.8512020325932,-5.10703360840786,-323.417882736566)) ;
#40545=CARTESIAN_POINT('Ctrl Pts',(17.7866861796911,-5.32738216705103,-323.420770032646)) ;
#40546=CARTESIAN_POINT('Ctrl Pts',(17.6777065113091,-5.67551534516244,-323.425400735559)) ;
#40547=CARTESIAN_POINT('Ctrl Pts',(17.6359039847283,-5.80410824417468,-323.427126298822)) ;
#40548=CARTESIAN_POINT('Ctrl Pts',(17.5522896086686,-6.05207603347171,-323.430484421345)) ;
#40549=CARTESIAN_POINT('Ctrl Pts',(17.5106551997093,-6.17150299719148,-323.432115690835)) ;
#40550=CARTESIAN_POINT('Ctrl Pts',(17.4170129585743,-6.43153408654003,-323.435698544326)) ;
#40551=CARTESIAN_POINT('Ctrl Pts',(17.3645158383175,-6.57195258035621,-323.437653361151)) ;
#40552=CARTESIAN_POINT('Ctrl Pts',(17.1426893115152,-7.14406959323832,-323.445699558237)) ;
#40553=CARTESIAN_POINT('Ctrl Pts',(16.9589161370008,-7.56998602608412,-323.45188564002)) ;
#40554=CARTESIAN_POINT('Ctrl Pts',(16.5582670305711,-8.41051596655,-323.464399267013)) ;
#40555=CARTESIAN_POINT('Ctrl Pts',(16.3412801388939,-8.82471241091497,-323.470722894878)) ;
#40556=CARTESIAN_POINT('Ctrl Pts',(16.0274062481404,-9.37249239566411,-323.479156072337)) ;
#40557=CARTESIAN_POINT('Ctrl Pts',(15.9440384104932,-9.51362202494632,-323.481334783387)) ;
#40558=CARTESIAN_POINT('Ctrl Pts',(15.79446681661,-9.75933561227325,-323.485127552774)) ;
#40559=CARTESIAN_POINT('Ctrl Pts',(15.7290655845843,-9.86439605475504,-323.486749065418)) ;
#40560=CARTESIAN_POINT('Ctrl Pts',(15.6246196813183,-10.0284977731937,-323.48927681513)) ;
#40561=CARTESIAN_POINT('Ctrl Pts',(15.5862794515146,-10.0879829824248,-323.490192044554)) ;
#40562=CARTESIAN_POINT('Ctrl Pts',(15.5134340208546,-10.1995966598642,-323.49190619267)) ;
#40563=CARTESIAN_POINT('Ctrl Pts',(15.4790038351896,-10.2517728918177,-323.492706224934)) ;
#40564=CARTESIAN_POINT('Ctrl Pts',(15.379860742541,-10.4003783147004,-323.494982551317)) ;
#40565=CARTESIAN_POINT('Ctrl Pts',(15.314505667694,-10.4963756490633,-323.496450278512)) ;
#40566=CARTESIAN_POINT('Ctrl Pts',(15.0193972775206,-10.921223877402,-323.502946911536)) ;
#40567=CARTESIAN_POINT('Ctrl Pts',(14.7799215551909,-11.2431910913136,-323.50787528335)) ;
#40568=CARTESIAN_POINT('Ctrl Pts',(14.2399015016662,-11.9221303640034,-323.518507286255)) ;
#40569=CARTESIAN_POINT('Ctrl Pts',(13.9359500139086,-12.2760451352662,-323.524204521123)) ;
#40570=CARTESIAN_POINT('Ctrl Pts',(13.416292843738,-12.8369209774765,-323.533682028209)) ;
#40571=CARTESIAN_POINT('Ctrl Pts',(13.208346897629,-13.0507863954024,-323.537410496588)) ;
#40572=CARTESIAN_POINT('Ctrl Pts',(12.8908182229612,-13.3619880043206,-323.543035786374)) ;
#40573=CARTESIAN_POINT('Ctrl Pts',(12.7850891698389,-13.4631873166709,-323.544897986929)) ;
#40574=CARTESIAN_POINT('Ctrl Pts',(12.5875269499987,-13.6478592261056,-323.548359743646)) ;
#40575=CARTESIAN_POINT('Ctrl Pts',(12.4960320180572,-13.7316816131623,-323.549956055694)) ;
#40576=CARTESIAN_POINT('Ctrl Pts',(12.2874157764585,-13.9189919752601,-323.553581045082)) ;
#40577=CARTESIAN_POINT('Ctrl Pts',(12.1698141909309,-14.0219309129883,-323.555614302201)) ;
#40578=CARTESIAN_POINT('Ctrl Pts',(11.7905788862626,-14.345517716308,-323.562138469836)) ;
#40579=CARTESIAN_POINT('Ctrl Pts',(11.5241385872486,-14.5604209388132,-323.566674923889)) ;
#40580=CARTESIAN_POINT('Ctrl Pts',(10.7099331151377,-15.1807804668337,-323.580357077851)) ;
#40581=CARTESIAN_POINT('Ctrl Pts',(10.1456348005316,-15.563574595004,-323.589621784976)) ;
#40582=CARTESIAN_POINT('Ctrl Pts',(9.4013627128699,-16.010740540667,-323.601168913555)) ;
#40583=CARTESIAN_POINT('Ctrl Pts',(9.23970408350948,-16.1045739523244,-323.603637100746)) ;
#40584=CARTESIAN_POINT('Ctrl Pts',(9.00528869496427,-16.2359467825268,-323.607145037673)) ;
#40585=CARTESIAN_POINT('Ctrl Pts',(8.93365765930777,-16.2754709073548,-323.608207558408)) ;
#40586=CARTESIAN_POINT('Ctrl Pts',(8.80361898002909,-16.346105687975,-323.610117848131)) ;
#40587=CARTESIAN_POINT('Ctrl Pts',(8.74530197161909,-16.3773798798947,-323.610967667025)) ;
#40588=CARTESIAN_POINT('Ctrl Pts',(8.60213932837005,-16.4531723017898,-323.613037816977)) ;
#40589=CARTESIAN_POINT('Ctrl Pts',(8.51711389007415,-16.4973467817862,-323.614253753368)) ;
#40590=CARTESIAN_POINT('Ctrl Pts',(8.18379450336982,-16.6672572715916,-323.618974526123)) ;
#40591=CARTESIAN_POINT('Ctrl Pts',(7.93302743539708,-16.7880622397032,-323.622427635515)) ;
#40592=CARTESIAN_POINT('Ctrl Pts',(7.01926950190053,-17.2032107219358,-323.634795144119)) ;
#40593=CARTESIAN_POINT('Ctrl Pts',(6.34188560579116,-17.4642804977528,-323.643586853735)) ;
#40594=CARTESIAN_POINT('Ctrl Pts',(5.42390919650671,-17.7576047969066,-323.655602086964)) ;
#40595=CARTESIAN_POINT('Ctrl Pts',(5.19547442175171,-17.8257780846087,-323.658597318588)) ;
#40596=CARTESIAN_POINT('Ctrl Pts',(4.83403222518032,-17.926107491275,-323.663356505027)) ;
#40597=CARTESIAN_POINT('Ctrl Pts',(4.70187379795501,-17.9612243475874,-323.665100737526)) ;
#40598=CARTESIAN_POINT('Ctrl Pts',(4.44734264949641,-18.0258560313336,-323.668469328127)) ;
#40599=CARTESIAN_POINT('Ctrl Pts',(4.32503390907904,-18.0555925944412,-323.670092098988)) ;
#40600=CARTESIAN_POINT('Ctrl Pts',(4.03312163953547,-18.1234280252547,-323.673975420308)) ;
#40601=CARTESIAN_POINT('Ctrl Pts',(3.86326694324537,-18.1603932208046,-323.676243267535)) ;
#40602=CARTESIAN_POINT('Ctrl Pts',(3.00433517995802,-18.3347252119986,-323.687751046602)) ;
#40603=CARTESIAN_POINT('Ctrl Pts',(2.30837543410544,-18.4352806738096,-323.697227915984)) ;
#40604=CARTESIAN_POINT('Ctrl Pts',(1.32339132720001,-18.5209335274373,-323.710537542992)) ;
#40605=CARTESIAN_POINT('Ctrl Pts',(1.03784802112278,-18.5391266011936,-323.71438026684)) ;
#40606=CARTESIAN_POINT('Ctrl Pts',(0.572383341458803,-18.557995347468,-323.720570746154)) ;
#40607=CARTESIAN_POINT('Ctrl Pts',(0.392671647027375,-18.5626674586618,
-323.722942857314)) ;
#40608=CARTESIAN_POINT('Ctrl Pts',(0.13220455061334,-18.5656547755997,-323.726342026205)) ;
#40609=CARTESIAN_POINT('Ctrl Pts',(0.0514835533319589,-18.56605409768,-323.727390034011)) ;
#40610=CARTESIAN_POINT('Ctrl Pts',(-0.0955999450868811,-18.5658224712016,
-323.729288154021)) ;
#40611=CARTESIAN_POINT('Ctrl Pts',(-0.161961168924328,-18.5653621552626,
-323.730140127854)) ;
#40612=CARTESIAN_POINT('Ctrl Pts',(-0.310077309297243,-18.5635405287751,
-323.732032568184)) ;
#40613=CARTESIAN_POINT('Ctrl Pts',(-0.391828567636493,-18.561994916996,
-323.733070983871)) ;
#40614=CARTESIAN_POINT('Ctrl Pts',(-0.714902374646459,-18.5537514986789,
-323.737154821241)) ;
#40615=CARTESIAN_POINT('Ctrl Pts',(-0.956095187033817,-18.5428871135722,
-323.740160027758)) ;
#40616=CARTESIAN_POINT('Ctrl Pts',(-2.00659433908352,-18.4750167774234,
-323.753168131234)) ;
#40617=CARTESIAN_POINT('Ctrl Pts',(-2.81188197848714,-18.3697030875708,
-323.76297057117)) ;
#40618=CARTESIAN_POINT('Ctrl Pts',(-3.82119444668937,-18.1697645171,-323.775830886454)) ;
#40619=CARTESIAN_POINT('Ctrl Pts',(-4.03393224413369,-18.1237209208171,
-323.778571510467)) ;
#40620=CARTESIAN_POINT('Ctrl Pts',(-4.3754003375343,-18.0435055192205,-323.783027560451)) ;
#40621=CARTESIAN_POINT('Ctrl Pts',(-4.50465841605385,-18.0116704397114,
-323.78472757326)) ;
#40622=CARTESIAN_POINT('Ctrl Pts',(-4.75566958478692,-17.9469776467239,
-323.788056025662)) ;
#40623=CARTESIAN_POINT('Ctrl Pts',(-4.87745245116757,-17.9142640760013,
-323.789683422183)) ;
#40624=CARTESIAN_POINT('Ctrl Pts',(-5.14728986616577,-17.8388242182939,
-323.793317697014)) ;
#40625=CARTESIAN_POINT('Ctrl Pts',(-5.29516482784907,-17.7954902098312,
-323.795328501594)) ;
#40626=CARTESIAN_POINT('Ctrl Pts',(-6.13654753101533,-17.5375111442387,
-323.806877868866)) ;
#40627=CARTESIAN_POINT('Ctrl Pts',(-6.81753086240384,-17.284177067517,-323.816676306804)) ;
#40628=CARTESIAN_POINT('Ctrl Pts',(-7.73411826798254,-16.8805760561065,
-323.830154568869)) ;
#40629=CARTESIAN_POINT('Ctrl Pts',(-7.98380956548507,-16.7639261062606,
-323.833853574647)) ;
#40630=CARTESIAN_POINT('Ctrl Pts',(-8.38823308916128,-16.5639031764877,
-323.839846408533)) ;
#40631=CARTESIAN_POINT('Ctrl Pts',(-8.5445418843198,-16.4838146971828,-323.842162880615)) ;
#40632=CARTESIAN_POINT('Ctrl Pts',(-8.77042729694959,-16.3640006049362,
-323.845498776788)) ;
#40633=CARTESIAN_POINT('Ctrl Pts',(-8.8409201886417,-16.326023429215,-323.846538126273)) ;
#40634=CARTESIAN_POINT('Ctrl Pts',(-8.96950182988737,-16.2556746449036,
-323.848429257214)) ;
#40635=CARTESIAN_POINT('Ctrl Pts',(-9.02766639664809,-16.2234447840582,
-323.849282786557)) ;
#40636=CARTESIAN_POINT('Ctrl Pts',(-9.17176266897457,-16.1425839918251,
-323.851393374272)) ;
#40637=CARTESIAN_POINT('Ctrl Pts',(-9.25748198520534,-16.0935787108959,
-323.852645565963)) ;
#40638=CARTESIAN_POINT('Ctrl Pts',(-9.63085604940103,-15.8761525650157,
-323.858093305349)) ;
#40639=CARTESIAN_POINT('Ctrl Pts',(-9.91433687355013,-15.7006857774954,
-323.862213398769)) ;
#40640=CARTESIAN_POINT('Ctrl Pts',(-10.6419574345238,-15.2227411481744,
-323.872911666842)) ;
#40641=CARTESIAN_POINT('Ctrl Pts',(-11.0779611919801,-14.9084500343722,
-323.879452312755)) ;
#40642=CARTESIAN_POINT('Ctrl Pts',(-11.62026839743,-14.4805883423499,-323.887999798035)) ;
#40643=CARTESIAN_POINT('Ctrl Pts',(-11.7396307068311,-14.3839892647788,
-323.889907534588)) ;
#40644=CARTESIAN_POINT('Ctrl Pts',(-12.0294923303816,-14.1433946485244,
-323.894612629072)) ;
#40645=CARTESIAN_POINT('Ctrl Pts',(-12.1986198822566,-13.9977844897618,
-323.897420982805)) ;
#40646=CARTESIAN_POINT('Ctrl Pts',(-12.4651022248643,-13.7598584698423,
-323.901957675155)) ;
#40647=CARTESIAN_POINT('Ctrl Pts',(-12.5641527718401,-13.6694748856444,
-323.903669495621)) ;
#40648=CARTESIAN_POINT('Ctrl Pts',(-12.754058873601,-13.4923775733218,-323.907002808177)) ;
#40649=CARTESIAN_POINT('Ctrl Pts',(-12.8450308507631,-13.4057992198298,
-323.908623053695)) ;
#40650=CARTESIAN_POINT('Ctrl Pts',(-13.0439094789223,-13.2126426236198,
-323.912217959475)) ;
#40651=CARTESIAN_POINT('Ctrl Pts',(-13.1514027374575,-13.1056516640792,
-323.914196237261)) ;
#40652=CARTESIAN_POINT('Ctrl Pts',(-13.5580809037679,-12.6908314864055,
-323.921816323016)) ;
#40653=CARTESIAN_POINT('Ctrl Pts',(-13.8478670510679,-12.3739782608301,
-323.92753672665)) ;
#40654=CARTESIAN_POINT('Ctrl Pts',(-14.4444817281997,-11.674404414738,-323.939882560336)) ;
#40655=CARTESIAN_POINT('Ctrl Pts',(-14.7476587905868,-11.2889915689595,
-323.946517515641)) ;
#40656=CARTESIAN_POINT('Ctrl Pts',(-15.1334564391573,-10.7564413220802,
-323.955305237844)) ;
#40657=CARTESIAN_POINT('Ctrl Pts',(-15.2298461524232,-10.619525413575,-323.957531800775)) ;
#40658=CARTESIAN_POINT('Ctrl Pts',(-15.3953002994273,-10.3776208024618,
-323.961397282393)) ;
#40659=CARTESIAN_POINT('Ctrl Pts',(-15.4651754295498,-10.2731997858886,
-323.963044034665)) ;
#40660=CARTESIAN_POINT('Ctrl Pts',(-15.5729472825247,-10.1085544643828,
-323.965601654979)) ;
#40661=CARTESIAN_POINT('Ctrl Pts',(-15.6115668320745,-10.0488079635763,
-323.966521852004)) ;
#40662=CARTESIAN_POINT('Ctrl Pts',(-15.6881090970104,-9.92888670684282,
-323.968351860028)) ;
#40663=CARTESIAN_POINT('Ctrl Pts',(-15.726031330753,-9.86871303050863,-323.969261657649)) ;
#40664=CARTESIAN_POINT('Ctrl Pts',(-15.8299415797294,-9.70171197077004,
-323.971765322999)) ;
#40665=CARTESIAN_POINT('Ctrl Pts',(-15.8951931357065,-9.59443071984208,
-323.973349756565)) ;
#40666=CARTESIAN_POINT('Ctrl Pts',(-16.0652294870347,-9.30837462762842,
-323.977521500787)) ;
#40667=CARTESIAN_POINT('Ctrl Pts',(-16.1681182712859,-9.1284932204573,-323.980090796395)) ;
#40668=CARTESIAN_POINT('Ctrl Pts',(-16.5533231895385,-8.42808472390377,
-323.989947783485)) ;
#40669=CARTESIAN_POINT('Ctrl Pts',(-16.8136870526762,-7.89588817229777,
-323.997139857357)) ;
#40670=CARTESIAN_POINT('Ctrl Pts',(-17.1118556839643,-7.20449547407663,
-324.00644709476)) ;
#40671=CARTESIAN_POINT('Ctrl Pts',(-17.1736164390241,-7.05600866748605,
-324.00844305087)) ;
#40672=CARTESIAN_POINT('Ctrl Pts',(-17.3190556277311,-6.69311413874813,
-324.013322024012)) ;
#40673=CARTESIAN_POINT('Ctrl Pts',(-17.4006913297935,-6.47791676983834,
-324.016216225918)) ;
#40674=CARTESIAN_POINT('Ctrl Pts',(-17.5239380314501,-6.13387352151208,
-324.020855152102)) ;
#40675=CARTESIAN_POINT('Ctrl Pts',(-17.56817692178,-6.00599434635214,-324.022581914922)) ;
#40676=CARTESIAN_POINT('Ctrl Pts',(-17.6510393599688,-5.75771599431401,
-324.025940655414)) ;
#40677=CARTESIAN_POINT('Ctrl Pts',(-17.6898387211444,-5.63738325149682,
-324.027571323706)) ;
#40678=CARTESIAN_POINT('Ctrl Pts',(-17.7718858653347,-5.37373059732031,
-324.031150771236)) ;
#40679=CARTESIAN_POINT('Ctrl Pts',(-17.8146354597751,-5.23026491593894,
-324.033102756787)) ;
#40680=CARTESIAN_POINT('Ctrl Pts',(-17.9817830474478,-4.64348687351731,
-324.041102768237)) ;
#40681=CARTESIAN_POINT('Ctrl Pts',(-18.0914044770507,-4.1961379618827,-324.047244019601)) ;
#40682=CARTESIAN_POINT('Ctrl Pts',(-18.2791698126968,-3.284465131321,-324.059751957753)) ;
#40683=CARTESIAN_POINT('Ctrl Pts',(-18.3565138536121,-2.82031189593331,
-324.066116073327)) ;
#40684=CARTESIAN_POINT('Ctrl Pts',(-18.4461489062061,-2.11898391226726,
-324.075560962735)) ;
#40685=CARTESIAN_POINT('Ctrl Pts',(-18.4716596230034,-1.88369144161412,
-324.078700048023)) ;
#40686=CARTESIAN_POINT('Ctrl Pts',(-18.5005070762339,-1.55998133948917,
-324.082951338903)) ;
#40687=CARTESIAN_POINT('Ctrl Pts',(-18.5077205305798,-1.47193228449077,
-324.084100827533)) ;
#40688=CARTESIAN_POINT('Ctrl Pts',(-18.5192057283192,-1.31827201937813,
-324.08609293446)) ;
#40689=CARTESIAN_POINT('Ctrl Pts',(-18.5237578729388,-1.25268360122756,
-324.086938688335)) ;
#40690=CARTESIAN_POINT('Ctrl Pts',(-18.5334728918954,-1.1010504402287,-324.088883524569)) ;
#40691=CARTESIAN_POINT('Ctrl Pts',(-18.5383851002295,-1.01499133527106,
-324.089979775295)) ;
#40692=CARTESIAN_POINT('Ctrl Pts',(-18.5508523473216,-0.766120490061058,
-324.093131830707)) ;
#40693=CARTESIAN_POINT('Ctrl Pts',(-18.5568630394829,-0.603239336752139,
-324.095172399095)) ;
#40694=CARTESIAN_POINT('Ctrl Pts',(-18.567355789222,-0.160920308868857,
-324.100674562745)) ;
#40695=CARTESIAN_POINT('Ctrl Pts',(-18.567674517597,0.118573812836487,-324.104109250648)) ;
#40696=CARTESIAN_POINT('Ctrl Pts',(-18.5541197532939,0.750782601332609,
-324.111861938473)) ;
#40697=CARTESIAN_POINT('Ctrl Pts',(-18.5364975924869,1.10330925274586,-324.116173948557)) ;
#40698=CARTESIAN_POINT('Ctrl Pts',(-18.4875533154418,1.7258713362352,-324.1238641765)) ;
#40699=CARTESIAN_POINT('Ctrl Pts',(-18.4603290444846,1.99612392089792,-324.127227349924)) ;
#40700=CARTESIAN_POINT('Ctrl Pts',(-18.4010277568686,2.47843172522886,-324.133303575734)) ;
#40701=CARTESIAN_POINT('Ctrl Pts',(-18.3711869885596,2.69071268000922,-324.136003678311)) ;
#40702=CARTESIAN_POINT('Ctrl Pts',(-18.3169576172568,3.03333629516447,-324.140411505258)) ;
#40703=CARTESIAN_POINT('Ctrl Pts',(-18.2948368747106,3.16401787268748,-324.142104463582)) ;
#40704=CARTESIAN_POINT('Ctrl Pts',(-18.2488819474081,3.41888797420616,-324.145430527637)) ;
#40705=CARTESIAN_POINT('Ctrl Pts',(-18.225174498806,3.54309211631266,-324.147062716791)) ;
#40706=CARTESIAN_POINT('Ctrl Pts',(-18.1694524714901,3.81965055839441,-324.150722804066)) ;
#40707=CARTESIAN_POINT('Ctrl Pts',(-18.1367866631158,3.97186391264434,-324.15275483126)) ;
#40708=CARTESIAN_POINT('Ctrl Pts',(-17.9447695069173,4.81479103820004,-324.164103920793)) ;
#40709=CARTESIAN_POINT('Ctrl Pts',(-17.7478763809153,5.49634799684162,-324.173666136872)) ;
#40710=CARTESIAN_POINT('Ctrl Pts',(-17.4182716560495,6.43263842295779,-324.187027643438)) ;
#40711=CARTESIAN_POINT('Ctrl Pts',(-17.3179192901622,6.69811140088752,-324.190838755185)) ;
#40712=CARTESIAN_POINT('Ctrl Pts',(-17.1444584601289,7.12699341337816,-324.196985894895)) ;
#40713=CARTESIAN_POINT('Ctrl Pts',(-17.0750025990897,7.29182949890128,-324.199345898812)) ;
#40714=CARTESIAN_POINT('Ctrl Pts',(-16.9708164458865,7.52943436296937,-324.20273131719)) ;
#40715=CARTESIAN_POINT('Ctrl Pts',(-16.9379770088996,7.60302094804456,-324.203777456884)) ;
#40716=CARTESIAN_POINT('Ctrl Pts',(-16.877209481932,7.7368409021025,-324.205674050935)) ;
#40717=CARTESIAN_POINT('Ctrl Pts',(-16.8494354578039,7.79714253999942,-324.206526342475)) ;
#40718=CARTESIAN_POINT('Ctrl Pts',(-16.7799334737977,7.94593631101331,-324.208624368038)) ;
#40719=CARTESIAN_POINT('Ctrl Pts',(-16.7378283306994,8.03425006182183,-324.209865381101)) ;
#40720=CARTESIAN_POINT('Ctrl Pts',(-16.5502105180837,8.41989361480937,-324.215273928545)) ;
#40721=CARTESIAN_POINT('Ctrl Pts',(-16.3974585496524,8.71363476340976,-324.219366672211)) ;
#40722=CARTESIAN_POINT('Ctrl Pts',(-15.9749446249027,9.47562833895723,-324.230075764247)) ;
#40723=CARTESIAN_POINT('Ctrl Pts',(-15.6924550293611,9.93646032958495,-324.236652596206)) ;
#40724=CARTESIAN_POINT('Ctrl Pts',(-15.3041482968991,10.5119576665882,-324.245242567396)) ;
#40725=CARTESIAN_POINT('Ctrl Pts',(-15.2164399100211,10.6385227111206,-324.247155546407)) ;
#40726=CARTESIAN_POINT('Ctrl Pts',(-14.9975448100899,10.9461470482429,-324.25187103321)) ;
#40727=CARTESIAN_POINT('Ctrl Pts',(-14.8646425266992,11.125955591658,-324.254684549326)) ;
#40728=CARTESIAN_POINT('Ctrl Pts',(-14.6468460369367,11.4097501970167,-324.259227389375)) ;
#40729=CARTESIAN_POINT('Ctrl Pts',(-14.5640154354839,11.5152921248197,-324.260940109721)) ;
#40730=CARTESIAN_POINT('Ctrl Pts',(-14.4014723224883,11.7178434954987,-324.264273832678)) ;
#40731=CARTESIAN_POINT('Ctrl Pts',(-14.3219052730378,11.8149604543419,-324.265893573586)) ;
#40732=CARTESIAN_POINT('Ctrl Pts',(-14.1441730244388,12.0274609142514,-324.269485656118)) ;
#40733=CARTESIAN_POINT('Ctrl Pts',(-14.0455682798255,12.142465079025,-324.271461593137)) ;
#40734=CARTESIAN_POINT('Ctrl Pts',(-13.6571009401313,12.5844761052013,-324.279180322461)) ;
#40735=CARTESIAN_POINT('Ctrl Pts',(-13.3571374800356,12.9024153331622,-324.285005123218)) ;
#40736=CARTESIAN_POINT('Ctrl Pts',(-12.9679882991646,13.2867555969037,-324.292351013689)) ;
#40737=CARTESIAN_POINT('Ctrl Pts',(-12.889054177129,13.3633407958953,-324.293830511261)) ;
#40738=CARTESIAN_POINT('Ctrl Pts',(-12.3927598227565,13.8363782807931,-324.303061002039)) ;
#40739=CARTESIAN_POINT('Ctrl Pts',(-11.9578297118556,14.2139427810809,-324.310847955634)) ;
#40740=CARTESIAN_POINT('Ctrl Pts',(-11.4223337296037,14.6368088711685,-324.319814521377)) ;
#40741=CARTESIAN_POINT('Ctrl Pts',(-11.3380356491296,14.7022049173412,-324.32120836544)) ;
#40742=CARTESIAN_POINT('Ctrl Pts',(-11.1999055796125,14.8074677283556,-324.323460529833)) ;
#40743=CARTESIAN_POINT('Ctrl Pts',(-11.1464132751362,14.8477761519391,-324.324325028041)) ;
#40744=CARTESIAN_POINT('Ctrl Pts',(-11.0317032485867,14.9332451157236,-324.326161661636)) ;
#40745=CARTESIAN_POINT('Ctrl Pts',(-10.9704238054972,14.978320593432,-324.327132634947)) ;
#40746=CARTESIAN_POINT('Ctrl Pts',(-10.7859849524016,15.1122496921848,-324.330027332871)) ;
#40747=CARTESIAN_POINT('Ctrl Pts',(-10.6620104932061,15.1999702145794,-324.331936371896)) ;
#40748=CARTESIAN_POINT('Ctrl Pts',(-10.440854319518,15.3524164002585,-324.33528914206)) ;
#40749=CARTESIAN_POINT('Ctrl Pts',(-10.3441121145819,15.4177648460854,-324.336738292432)) ;
#40750=CARTESIAN_POINT('Ctrl Pts',(-9.8586678692911,15.7390519865276,-324.343937122767)) ;
#40751=CARTESIAN_POINT('Ctrl Pts',(-9.46105475063361,15.9812244114188,-324.349606968786)) ;
#40752=CARTESIAN_POINT('Ctrl Pts',(-8.64798352947633,16.4354492379765,-324.361040018164)) ;
#40753=CARTESIAN_POINT('Ctrl Pts',(-8.23279419330226,16.6473033605225,-324.366799601881)) ;
#40754=CARTESIAN_POINT('Ctrl Pts',(-7.67394169943359,16.9064376973664,-324.37455946645)) ;
#40755=CARTESIAN_POINT('Ctrl Pts',(-7.53704659592083,16.9679092804009,-324.37646039916)) ;
#40756=CARTESIAN_POINT('Ctrl Pts',(-7.2833985956329,17.0781324382906,-324.379985327671)) ;
#40757=CARTESIAN_POINT('Ctrl Pts',(-7.16686353865906,17.1273631843124,-324.381605854043)) ;
#40758=CARTESIAN_POINT('Ctrl Pts',(-6.92481376661192,17.2267152193293,-324.384974901486)) ;
#40759=CARTESIAN_POINT('Ctrl Pts',(-6.79923653214833,17.2766647667963,-324.386724509828)) ;
#40760=CARTESIAN_POINT('Ctrl Pts',(-6.45926239258203,17.4076118813034,-324.391466209516)) ;
#40761=CARTESIAN_POINT('Ctrl Pts',(-6.24389298369518,17.4860179049564,-324.394475527915)) ;
#40762=CARTESIAN_POINT('Ctrl Pts',(-5.87598331878911,17.6122927295453,-324.399621774137)) ;
#40763=CARTESIAN_POINT('Ctrl Pts',(-5.72417563663214,17.6622152730534,-324.401746720793)) ;
#40764=CARTESIAN_POINT('Ctrl Pts',(-5.01469412694131,17.8854230643169,-324.411676302628)) ;
#40765=CARTESIAN_POINT('Ctrl Pts',(-4.44968896443668,18.0342945881159,-324.419590888887)) ;
#40766=CARTESIAN_POINT('Ctrl Pts',(-3.6232410265317,18.2108432910851,-324.430913897107)) ;
#40767=CARTESIAN_POINT('Ctrl Pts',(-3.36674871518028,18.2600025312862,-324.434391390069)) ;
#40768=CARTESIAN_POINT('Ctrl Pts',(-3.00800824240249,18.3209427403234,-324.439168998776)) ;
#40769=CARTESIAN_POINT('Ctrl Pts',(-2.90657053032288,18.3373090795478,-324.440510325029)) ;
#40770=CARTESIAN_POINT('Ctrl Pts',(-2.73873621216545,18.3629604668013,-324.442710885177)) ;
#40771=CARTESIAN_POINT('Ctrl Pts',(-2.67241588457293,18.3727294250189,-324.443575571237)) ;
#40772=CARTESIAN_POINT('Ctrl Pts',(-2.52876852843879,18.3930943735101,-324.445437153986)) ;
#40773=CARTESIAN_POINT('Ctrl Pts',(-2.45142478384017,18.4035623577219,-324.446432627266)) ;
#40774=CARTESIAN_POINT('Ctrl Pts',(-2.21209270934666,18.4344189125433,-324.449494752219)) ;
#40775=CARTESIAN_POINT('Ctrl Pts',(-2.04989955283367,18.4531587208636,-324.451544149119)) ;
#40776=CARTESIAN_POINT('Ctrl Pts',(-1.38571922609436,18.5210333123235,-324.459864273711)) ;
#40777=CARTESIAN_POINT('Ctrl Pts',(-0.882076138796647,18.5518418666242,
-324.466010819242)) ;
#40778=CARTESIAN_POINT('Ctrl Pts',(0.104180440712025,18.5719156590424,-324.478103884316)) ;
#40779=CARTESIAN_POINT('Ctrl Pts',(0.586363543142085,18.5629491558235,-324.484042574201)) ;
#40780=CARTESIAN_POINT('Ctrl Pts',(1.25279041943156,18.5245622530413,-324.492424001211)) ;
#40781=CARTESIAN_POINT('Ctrl Pts',(1.43776148413839,18.5111245541986,-324.494768174686)) ;
#40782=CARTESIAN_POINT('Ctrl Pts',(1.74835396756131,18.4838772703247,-324.498739241115)) ;
#40783=CARTESIAN_POINT('Ctrl Pts',(1.87409191517363,18.4715521811394,-324.500356463428)) ;
#40784=CARTESIAN_POINT('Ctrl Pts',(2.13163095670585,18.4436509536328,-324.503689610014)) ;
#40785=CARTESIAN_POINT('Ctrl Pts',(2.26341058377905,18.4279430078867,-324.505406305769)) ;
#40786=CARTESIAN_POINT('Ctrl Pts',(2.60854019359328,18.3830461036312,-324.509932064979)) ;
#40787=CARTESIAN_POINT('Ctrl Pts',(2.82157029892458,18.3515559772245,-324.512755627286)) ;
#40788=CARTESIAN_POINT('Ctrl Pts',(3.30374402845528,18.2716865895805,-324.519211229117)) ;
#40789=CARTESIAN_POINT('Ctrl Pts',(3.57246364315119,18.2210526189448,-324.522855329624)) ;
#40790=CARTESIAN_POINT('Ctrl Pts',(4.18292286917412,18.0920018566472,-324.531217395195)) ;
#40791=CARTESIAN_POINT('Ctrl Pts',(4.52375710741976,18.0098027811781,-324.535947247355)) ;
#40792=CARTESIAN_POINT('Ctrl Pts',(4.95311624671509,17.8932959724943,-324.541935394451)) ;
#40793=CARTESIAN_POINT('Ctrl Pts',(5.04398375018243,17.8678938112029,-324.5432043056)) ;
#40794=CARTESIAN_POINT('Ctrl Pts',(5.44417387341787,17.7527239473073,-324.548795550816)) ;
#40795=CARTESIAN_POINT('Ctrl Pts',(5.75132435800101,17.6556083323244,-324.553095306633)) ;
#40796=CARTESIAN_POINT('Ctrl Pts',(6.14829269583703,17.5186349696355,-324.558602517575)) ;
#40797=CARTESIAN_POINT('Ctrl Pts',(6.24053867217814,17.4859872868109,-324.559878613981)) ;
#40798=CARTESIAN_POINT('Ctrl Pts',(6.39493271446416,17.4299668053486,-324.562005739409)) ;
#40799=CARTESIAN_POINT('Ctrl Pts',(6.45722120746729,17.4069871480101,-324.56286143272)) ;
#40800=CARTESIAN_POINT('Ctrl Pts',(6.59482637025094,17.3553811934651,-324.564745776105)) ;
#40801=CARTESIAN_POINT('Ctrl Pts',(6.67008251218251,17.3265977770865,-324.565772550043)) ;
#40802=CARTESIAN_POINT('Ctrl Pts',(6.91173575077784,17.2323643012918,-324.569060754749)) ;
#40803=CARTESIAN_POINT('Ctrl Pts',(7.0773756963453,17.1649999694861,-324.571301143092)) ;
#40804=CARTESIAN_POINT('Ctrl Pts',(7.50317245671976,16.984620817098,-324.577052479042)) ;
#40805=CARTESIAN_POINT('Ctrl Pts',(7.76175898468539,16.8680182324122,-324.580537972568)) ;
#40806=CARTESIAN_POINT('Ctrl Pts',(8.65725778979356,16.4392635963865,-324.592709666869)) ;
#40807=CARTESIAN_POINT('Ctrl Pts',(9.2788682826451,16.0965866879065,-324.601364003498)) ;
#40808=CARTESIAN_POINT('Ctrl Pts',(10.0111014883923,15.6363858600552,-324.612246137638)) ;
#40809=CARTESIAN_POINT('Ctrl Pts',(10.1418101823302,15.5519259870914,-324.614215550832)) ;
#40810=CARTESIAN_POINT('Ctrl Pts',(10.37676097268,15.3958863287364,-324.617807647135)) ;
#40811=CARTESIAN_POINT('Ctrl Pts',(10.4813631381111,15.3248657692395,-324.619425978489)) ;
#40812=CARTESIAN_POINT('Ctrl Pts',(10.6941333593913,15.1772060166064,-324.622758210772)) ;
#40813=CARTESIAN_POINT('Ctrl Pts',(10.8022224610996,15.1004655761914,-324.624472849874)) ;
#40814=CARTESIAN_POINT('Ctrl Pts',(11.0830155509729,14.8965520094093,-324.628985159841)) ;
#40815=CARTESIAN_POINT('Ctrl Pts',(11.2543537881431,14.7675324964426,-324.631797165475)) ;
#40816=CARTESIAN_POINT('Ctrl Pts',(11.5375342631315,14.5465033115619,-324.636541548852)) ;
#40817=CARTESIAN_POINT('Ctrl Pts',(11.6506047481779,14.4561012864183,-324.638462554768)) ;
#40818=CARTESIAN_POINT('Ctrl Pts',(12.1338923240003,14.060350198098,-324.646784138546)) ;
#40819=CARTESIAN_POINT('Ctrl Pts',(12.4932503784913,13.7420334794546,-324.653261774176)) ;
#40820=CARTESIAN_POINT('Ctrl Pts',(12.9042830285731,13.3484804927794,-324.660921460213)) ;
#40821=CARTESIAN_POINT('Ctrl Pts',(12.9682502829186,13.2863439874793,-324.66212088407)) ;
#40822=CARTESIAN_POINT('Ctrl Pts',(13.2657618104115,12.993151715513,-324.667730379253)) ;
#40823=CARTESIAN_POINT('Ctrl Pts',(13.493594870502,12.7563837414125,-324.672117526406)) ;
#40824=CARTESIAN_POINT('Ctrl Pts',(13.7808787327236,12.441520269464,-324.677707071031)) ;
#40825=CARTESIAN_POINT('Ctrl Pts',(13.8461611037519,12.3688264597231,-324.678981191469)) ;
#40826=CARTESIAN_POINT('Ctrl Pts',(13.9548244378176,12.2458882857338,-324.681106122939)) ;
#40827=CARTESIAN_POINT('Ctrl Pts',(13.9985151942239,12.1959205224098,-324.681961574479)) ;
#40828=CARTESIAN_POINT('Ctrl Pts',(14.0947030561704,12.0847155884654,-324.683846758524)) ;
#40829=CARTESIAN_POINT('Ctrl Pts',(14.1470708503968,12.0233685576739,-324.684874599791)) ;
#40830=CARTESIAN_POINT('Ctrl Pts',(14.3145931520765,11.8245122957983,-324.68817078775)) ;
#40831=CARTESIAN_POINT('Ctrl Pts',(14.428155485717,11.6856748895056,-324.690417951463)) ;
#40832=CARTESIAN_POINT('Ctrl Pts',(14.7169391794318,11.3219895532334,-324.69619337261)) ;
#40833=CARTESIAN_POINT('Ctrl Pts',(14.8890260111889,11.094712754573,-324.699695922776)) ;
#40834=CARTESIAN_POINT('Ctrl Pts',(15.4686136549433,10.2914623185011,-324.711838576095)) ;
#40835=CARTESIAN_POINT('Ctrl Pts',(15.8484714228753,9.69629610487714,-324.720448245434)) ;
#40836=CARTESIAN_POINT('Ctrl Pts',(16.2699357734574,8.94472398387492,-324.731289370676)) ;
#40837=CARTESIAN_POINT('Ctrl Pts',(16.3446127985239,8.80752687151463,-324.733265953058)) ;
#40838=CARTESIAN_POINT('Ctrl Pts',(16.4766468524527,8.55748942413728,-324.736866828345)) ;
#40839=CARTESIAN_POINT('Ctrl Pts',(16.5345981628697,8.44497366979848,-324.738486693089)) ;
#40840=CARTESIAN_POINT('Ctrl Pts',(16.6507908460302,8.21359732251355,-324.741817740228)) ;
#40841=CARTESIAN_POINT('Ctrl Pts',(16.708920711874,8.09468871279821,-324.743529615604)) ;
#40842=CARTESIAN_POINT('Ctrl Pts',(16.8574026586591,7.78254299763999,-324.748023852401)) ;
#40843=CARTESIAN_POINT('Ctrl Pts',(16.945704574732,7.58835266220957,-324.75082032914)) ;
#40844=CARTESIAN_POINT('Ctrl Pts',(17.1763878301818,7.05692409235652,-324.758470612091)) ;
#40845=CARTESIAN_POINT('Ctrl Pts',(17.3121736002563,6.71692793003951,-324.76336350778)) ;
#40846=CARTESIAN_POINT('Ctrl Pts',(17.6630807818063,5.7567960480472,-324.777102807033)) ;
#40847=CARTESIAN_POINT('Ctrl Pts',(17.8555056050564,5.12894167138362,-324.786010947495)) ;
#40848=CARTESIAN_POINT('Ctrl Pts',(18.0405672410463,4.38682484279444,-324.796066011163)) ;
#40849=CARTESIAN_POINT('Ctrl Pts',(18.0659244919529,4.28119970154073,-324.797485663999)) ;
#40850=CARTESIAN_POINT('Ctrl Pts',(18.1054876289773,4.10978658554265,-324.799767639971)) ;
#40851=CARTESIAN_POINT('Ctrl Pts',(18.1202652971264,4.04413323998005,-324.800636459264)) ;
#40852=CARTESIAN_POINT('Ctrl Pts',(18.1508335401383,3.90479446948766,-324.80246842664)) ;
#40853=CARTESIAN_POINT('Ctrl Pts',(18.1665330853654,3.8310904099575,-324.803430548767)) ;
#40854=CARTESIAN_POINT('Ctrl Pts',(18.2117120533573,3.61246645183499,-324.80626651823)) ;
#40855=CARTESIAN_POINT('Ctrl Pts',(18.2399091895371,3.46728750721235,-324.808126534658)) ;
#40856=CARTESIAN_POINT('Ctrl Pts',(18.3042526298113,3.11346560450989,-324.812618060399)) ;
#40857=CARTESIAN_POINT('Ctrl Pts',(18.3385699601185,2.90451105038135,-324.815235702515)) ;
#40858=CARTESIAN_POINT('Ctrl Pts',(18.4602769642495,2.07495238479324,-324.825553387073)) ;
#40859=CARTESIAN_POINT('Ctrl Pts',(18.5197942068525,1.45068150627204,-324.833167486342)) ;
#40860=CARTESIAN_POINT('Ctrl Pts',(18.5601405522589,0.543174177248273,-324.844443663741)) ;
#40861=CARTESIAN_POINT('Ctrl Pts',(18.5662454908204,0.261502216244568,-324.847969864823)) ;
#40862=CARTESIAN_POINT('Ctrl Pts',(18.56578249821,-0.164059476479644,-324.853357772871)) ;
#40863=CARTESIAN_POINT('Ctrl Pts',(18.5639539073582,-0.307913188073675,
-324.855189351218)) ;
#40864=CARTESIAN_POINT('Ctrl Pts',(18.5574578308975,-0.57482012306736,-324.858608602313)) ;
#40865=CARTESIAN_POINT('Ctrl Pts',(18.5532376662952,-0.69787632684319,-324.860193286471)) ;
#40866=CARTESIAN_POINT('Ctrl Pts',(18.5467890391715,-0.843582900306995,
-324.862079777443)) ;
#40867=CARTESIAN_POINT('Ctrl Pts',(18.5457426493003,-0.866282487621405,
-324.862373963682)) ;
#40868=CARTESIAN_POINT('Ctrl Pts',(18.544654593743,-0.888979977990137,-324.862668413757)) ;
#40869=CARTESIAN_POINT('Origin',(0.,0.,-315.477129595899)) ;
#40870=CARTESIAN_POINT('',(18.5446545943314,-0.888979965716109,-326.659259832385)) ;
#40871=CARTESIAN_POINT('',(18.5446545937382,-0.888979978089839,-326.364137692133)) ;
#40872=CARTESIAN_POINT('',(18.544654593745,-0.888979977948782,-315.477129595899)) ;
#40873=CARTESIAN_POINT('Ctrl Pts',(18.5446545943314,-0.888979965716149,
-326.659259832385)) ;
#40874=CARTESIAN_POINT('Ctrl Pts',(18.5702422063668,-0.355207051375194,
-326.652714073557)) ;
#40875=CARTESIAN_POINT('Ctrl Pts',(18.5727724921029,0.179411176510274,-326.646152532977)) ;
#40876=CARTESIAN_POINT('Ctrl Pts',(18.5466431199678,0.858914281140881,-326.637624094489)) ;
#40877=CARTESIAN_POINT('Ctrl Pts',(18.5393358311989,1.00435632427266,-326.635788225339)) ;
#40878=CARTESIAN_POINT('Ctrl Pts',(18.5230476142734,1.26688270475765,-326.632452823504)) ;
#40879=CARTESIAN_POINT('Ctrl Pts',(18.514665493499,1.38399650655875,-326.630957117559)) ;
#40880=CARTESIAN_POINT('Ctrl Pts',(18.4951421688321,1.62468738571748,-326.627866089292)) ;
#40881=CARTESIAN_POINT('Ctrl Pts',(18.483871920925,1.74824818218474,-326.62627000416)) ;
#40882=CARTESIAN_POINT('Ctrl Pts',(18.45563439337,2.02691964757025,-326.622648627966)) ;
#40883=CARTESIAN_POINT('Ctrl Pts',(18.4379485501066,2.18194804773963,-326.62061879637)) ;
#40884=CARTESIAN_POINT('Ctrl Pts',(18.3756626173753,2.672890198652,-326.614142720018)) ;
#40885=CARTESIAN_POINT('Ctrl Pts',(18.3238197963312,3.00781412503908,-326.609652028375)) ;
#40886=CARTESIAN_POINT('Ctrl Pts',(18.2545435802755,3.38648249859851,-326.604507495274)) ;
#40887=CARTESIAN_POINT('Ctrl Pts',(18.2460776868003,3.43180332816606,-326.603890697157)) ;
#40888=CARTESIAN_POINT('Ctrl Pts',(18.1953862252423,3.69768142571455,-326.60026623038)) ;
#40889=CARTESIAN_POINT('Ctrl Pts',(18.1493306951165,3.9174893763584,-326.597245379007)) ;
#40890=CARTESIAN_POINT('Ctrl Pts',(18.0146054177974,4.50699442595136,-326.589101444833)) ;
#40891=CARTESIAN_POINT('Ctrl Pts',(17.9185497858009,4.87489291921913,-326.583972460105)) ;
#40892=CARTESIAN_POINT('Ctrl Pts',(17.7523660031536,5.43981269911378,-326.576122075417)) ;
#40893=CARTESIAN_POINT('Ctrl Pts',(17.690091548706,5.63903557280363,-326.573359005911)) ;
#40894=CARTESIAN_POINT('Ctrl Pts',(17.6218590374155,5.84505367837416,-326.570521465574)) ;
#40895=CARTESIAN_POINT('Ctrl Pts',(17.619241461581,5.85293932619718,-326.570412885097)) ;
#40896=CARTESIAN_POINT('Ctrl Pts',(17.6145941848183,5.86690823452684,-326.570220597726)) ;
#40897=CARTESIAN_POINT('Ctrl Pts',(17.6125666240029,5.87299220527856,-326.570136868314)) ;
#40898=CARTESIAN_POINT('Ctrl Pts',(17.6089240296833,5.88390345181218,-326.569986738948)) ;
#40899=CARTESIAN_POINT('Ctrl Pts',(17.6073101624236,5.88873111609163,-326.569920326542)) ;
#40900=CARTESIAN_POINT('Ctrl Pts',(17.60437781623,5.89749084827315,-326.569799844474)) ;
#40901=CARTESIAN_POINT('Ctrl Pts',(17.6030600048481,5.90142313918915,-326.569745767603)) ;
#40902=CARTESIAN_POINT('Ctrl Pts',(17.6006398919603,5.90863662593557,-326.56964658294)) ;
#40903=CARTESIAN_POINT('Ctrl Pts',(17.5995379902297,5.91191795564468,-326.56960147079)) ;
#40904=CARTESIAN_POINT('Ctrl Pts',(17.5974939402152,5.91799925262315,-326.569517875161)) ;
#40905=CARTESIAN_POINT('Ctrl Pts',(17.5965520411652,5.92079930351666,-326.569479388944)) ;
#40906=CARTESIAN_POINT('Ctrl Pts',(17.5947881058356,5.92603894187128,-326.56940737907)) ;
#40907=CARTESIAN_POINT('Ctrl Pts',(17.5939662303993,5.92847858336349,-326.569373853634)) ;
#40908=CARTESIAN_POINT('Ctrl Pts',(17.5924130576212,5.93308582828845,-326.56931054732)) ;
#40909=CARTESIAN_POINT('Ctrl Pts',(17.5916818670251,5.93525346764398,-326.569280765255)) ;
#40910=CARTESIAN_POINT('Ctrl Pts',(17.5902879659944,5.93938321418496,-326.56922403001)) ;
#40911=CARTESIAN_POINT('Ctrl Pts',(17.5896253278628,5.94134534570729,-326.569197076022)) ;
#40912=CARTESIAN_POINT('Ctrl Pts',(17.5883513407013,5.94511565588149,-326.569145287071)) ;
#40913=CARTESIAN_POINT('Ctrl Pts',(17.5877400411056,5.9469238512234,-326.569120451551)) ;
#40914=CARTESIAN_POINT('Ctrl Pts',(17.586554877157,5.95042772915556,-326.569072329457)) ;
#40915=CARTESIAN_POINT('Ctrl Pts',(17.5859810463725,5.95212342309748,-326.569049042504)) ;
#40916=CARTESIAN_POINT('Ctrl Pts',(17.5848591748378,5.95543702188073,-326.569003540073)) ;
#40917=CARTESIAN_POINT('Ctrl Pts',(17.5843111560446,5.9570549340988,-326.568981324347)) ;
#40918=CARTESIAN_POINT('Ctrl Pts',(17.566008770633,6.01106441208532,-326.568239764466)) ;
#40919=CARTESIAN_POINT('Ctrl Pts',(17.5480205488011,6.06337647875357,-326.567523081235)) ;
#40920=CARTESIAN_POINT('Ctrl Pts',(17.5078787163113,6.17843917006968,-326.565950797208)) ;
#40921=CARTESIAN_POINT('Ctrl Pts',(17.4856210375909,6.24115250942391,-326.565096699864)) ;
#40922=CARTESIAN_POINT('Ctrl Pts',(17.4293678128239,6.39698869552229,-326.562980569414)) ;
#40923=CARTESIAN_POINT('Ctrl Pts',(17.3949626681717,6.48996152066947,-326.561723467072)) ;
#40924=CARTESIAN_POINT('Ctrl Pts',(17.2351266824184,6.91148191241109,-326.556040017663)) ;
#40925=CARTESIAN_POINT('Ctrl Pts',(17.101120758108,7.23670118052104,-326.551698157677)) ;
#40926=CARTESIAN_POINT('Ctrl Pts',(16.7448329160087,8.0361163555858,-326.540949882988)) ;
#40927=CARTESIAN_POINT('Ctrl Pts',(16.511574965163,8.50508600406551,-326.534571802745)) ;
#40928=CARTESIAN_POINT('Ctrl Pts',(16.1519310108722,9.15743586826784,-326.525351560858)) ;
#40929=CARTESIAN_POINT('Ctrl Pts',(16.0415924164435,9.34937535865893,-326.522595087342)) ;
#40930=CARTESIAN_POINT('Ctrl Pts',(15.8384209931595,9.68861252247362,-326.517630632447)) ;
#40931=CARTESIAN_POINT('Ctrl Pts',(15.7468988641999,9.83666448547054,-326.515431683849)) ;
#40932=CARTESIAN_POINT('Ctrl Pts',(15.5936916158589,10.076883103105,-326.511806487052)) ;
#40933=CARTESIAN_POINT('Ctrl Pts',(15.5332384647051,10.1698227146273,-326.510389597768)) ;
#40934=CARTESIAN_POINT('Ctrl Pts',(15.4024648629208,10.3669851638398,-326.507352293127)) ;
#40935=CARTESIAN_POINT('Ctrl Pts',(15.3319108663188,10.471046479457,-326.505730113518)) ;
#40936=CARTESIAN_POINT('Ctrl Pts',(15.1735482171346,10.6995858073751,-326.502124446477)) ;
#40937=CARTESIAN_POINT('Ctrl Pts',(15.085253538371,10.8237159764185,-326.500137257167)) ;
#40938=CARTESIAN_POINT('Ctrl Pts',(14.5570270395417,11.5473090846212,-326.488384048818)) ;
#40939=CARTESIAN_POINT('Ctrl Pts',(14.0829310810694,12.1209911281496,-326.478342376394)) ;
#40940=CARTESIAN_POINT('Ctrl Pts',(13.3932588240344,12.8602745641086,-326.464739468862)) ;
#40941=CARTESIAN_POINT('Ctrl Pts',(13.2065943173152,13.0518929900552,-326.46115082963)) ;
#40942=CARTESIAN_POINT('Ctrl Pts',(12.8929419144747,13.360249157689,-326.455310856005)) ;
#40943=CARTESIAN_POINT('Ctrl Pts',(12.7683518055667,13.4793694627025,-326.453038165669)) ;
#40944=CARTESIAN_POINT('Ctrl Pts',(12.5838629515905,13.6509054922516,-326.449752206078)) ;
#40945=CARTESIAN_POINT('Ctrl Pts',(12.5252573541044,13.7046983104199,-326.448719802299)) ;
#40946=CARTESIAN_POINT('Ctrl Pts',(12.4169416075096,13.8028438519424,-326.446834117313)) ;
#40947=CARTESIAN_POINT('Ctrl Pts',(12.3673351190881,13.8473087396007,-326.445979180319)) ;
#40948=CARTESIAN_POINT('Ctrl Pts',(12.2428914497442,13.9576519756633,-326.443855069296)) ;
#40949=CARTESIAN_POINT('Ctrl Pts',(12.1677608674609,14.0231963274567,-326.442590918102)) ;
#40950=CARTESIAN_POINT('Ctrl Pts',(11.8247366995782,14.3176203473069,-326.436892584026)) ;
#40951=CARTESIAN_POINT('Ctrl Pts',(11.5508880035671,14.5394510876483,-326.432542916145)) ;
#40952=CARTESIAN_POINT('Ctrl Pts',(10.7303469441769,15.1663071700223,-326.41986282476)) ;
#40953=CARTESIAN_POINT('Ctrl Pts',(10.1675134962265,15.5492407772484,-326.411587461683)) ;
#40954=CARTESIAN_POINT('Ctrl Pts',(9.39869396794216,16.0126932005314,-326.400367003105)) ;
#40955=CARTESIAN_POINT('Ctrl Pts',(9.21048987678015,16.1216831573904,-326.39762857707)) ;
#40956=CARTESIAN_POINT('Ctrl Pts',(8.90409312310711,16.2920022347175,-326.393175143229)) ;
#40957=CARTESIAN_POINT('Ctrl Pts',(8.78707956293618,16.355410231906,-326.391475513213)) ;
#40958=CARTESIAN_POINT('Ctrl Pts',(8.55787312328783,16.4764441553734,-326.388147200498)) ;
#40959=CARTESIAN_POINT('Ctrl Pts',(8.44575471700162,16.5341958258056,-326.386519554103)) ;
#40960=CARTESIAN_POINT('Ctrl Pts',(8.19528711927791,16.6599981149077,-326.382883923964)) ;
#40961=CARTESIAN_POINT('Ctrl Pts',(8.0566611076429,16.7274767929147,-326.380872003315)) ;
#40962=CARTESIAN_POINT('Ctrl Pts',(7.26196858210809,17.1021368020462,-326.369341641724)) ;
#40963=CARTESIAN_POINT('Ctrl Pts',(6.5892096713528,17.372437309749,-326.359564639076)) ;
#40964=CARTESIAN_POINT('Ctrl Pts',(5.64032792335114,17.6906075851473,-326.346095571732)) ;
#40965=CARTESIAN_POINT('Ctrl Pts',(5.37633879341372,17.772615938546,-326.342385124817)) ;
#40966=CARTESIAN_POINT('Ctrl Pts',(4.94145820108379,17.8971352738967,-326.336376498875)) ;
#40967=CARTESIAN_POINT('Ctrl Pts',(4.77161885327615,17.9431634298683,-326.334055541009)) ;
#40968=CARTESIAN_POINT('Ctrl Pts',(4.52352632433165,18.0066273589065,-326.330714535729)) ;
#40969=CARTESIAN_POINT('Ctrl Pts',(4.44577410134282,18.0259815797391,-326.329674481122)) ;
#40970=CARTESIAN_POINT('Ctrl Pts',(4.30327980514069,18.0604734881682,-326.327782788929)) ;
#40971=CARTESIAN_POINT('Ctrl Pts',(4.23857722064267,18.0757678353135,-326.326929394153)) ;
#40972=CARTESIAN_POINT('Ctrl Pts',(4.07767718010205,18.1128898405443,-326.32482013969)) ;
#40973=CARTESIAN_POINT('Ctrl Pts',(3.98138524884317,18.1342990242823,-326.32356913125)) ;
#40974=CARTESIAN_POINT('Ctrl Pts',(3.54411157924823,18.2278700515585,-326.317930795708)) ;
#40975=CARTESIAN_POINT('Ctrl Pts',(3.20130899250581,18.2911890096435,-326.313626614084)) ;
#40976=CARTESIAN_POINT('Ctrl Pts',(2.4490191149513,18.4083467278719,-326.304275287859)) ;
#40977=CARTESIAN_POINT('Ctrl Pts',(2.03910579866791,18.4582494188925,-326.29923915226)) ;
#40978=CARTESIAN_POINT('Ctrl Pts',(1.35354318610097,18.5185922456493,-326.290766707481)) ;
#40979=CARTESIAN_POINT('Ctrl Pts',(1.0787129409124,18.5366317322611,-326.28735772443)) ;
#40980=CARTESIAN_POINT('Ctrl Pts',(0.587407543280188,18.5579166830495,-326.281210249343)) ;
#40981=CARTESIAN_POINT('Ctrl Pts',(0.371084524128882,18.5635022362768,-326.278485220141)) ;
#40982=CARTESIAN_POINT('Ctrl Pts',(0.0218245807144408,18.5664127883284,
-326.274047731639)) ;
#40983=CARTESIAN_POINT('Ctrl Pts',(-0.111072437788727,18.5660933691244,
-326.272350435225)) ;
#40984=CARTESIAN_POINT('Ctrl Pts',(-0.370170199780886,18.5626885605346,
-326.269022951226)) ;
#40985=CARTESIAN_POINT('Ctrl Pts',(-0.496365646296472,18.559742823209,-326.267393758474)) ;
#40986=CARTESIAN_POINT('Ctrl Pts',(-0.777119648939183,18.5503237724084,
-326.263749762074)) ;
#40987=CARTESIAN_POINT('Ctrl Pts',(-0.931647146692736,18.5432052382465,
-326.261730955827)) ;
#40988=CARTESIAN_POINT('Ctrl Pts',(-1.8009580869145,18.4922652173002,-326.250301564516)) ;
#40989=CARTESIAN_POINT('Ctrl Pts',(-2.51282418618556,18.4090474805044,-326.240639439739)) ;
#40990=CARTESIAN_POINT('Ctrl Pts',(-3.49464427836755,18.2362498565568,-326.227221123847)) ;
#40991=CARTESIAN_POINT('Ctrl Pts',(-3.77005337844767,18.1813103295154,-326.223450586582)) ;
#40992=CARTESIAN_POINT('Ctrl Pts',(-4.16710563498376,18.0926949732638,-326.218045736527)) ;
#40993=CARTESIAN_POINT('Ctrl Pts',(-4.28981836909148,18.0639928917663,-326.216379755157)) ;
#40994=CARTESIAN_POINT('Ctrl Pts',(-4.51156964292605,18.0097389750561,-326.213382695124)) ;
#40995=CARTESIAN_POINT('Ctrl Pts',(-4.61070742624884,17.9846138592863,-326.212047730927)) ;
#40996=CARTESIAN_POINT('Ctrl Pts',(-4.77440867459764,17.9416834694386,-326.209854408829)) ;
#40997=CARTESIAN_POINT('Ctrl Pts',(-4.83909239497691,17.9243456991353,-326.208990675937)) ;
#40998=CARTESIAN_POINT('Ctrl Pts',(-4.9791715631619,17.8859854668682,-326.207127255513)) ;
#40999=CARTESIAN_POINT('Ctrl Pts',(-5.05453060564233,17.8648354583893,-326.206129032033)) ;
#41000=CARTESIAN_POINT('Ctrl Pts',(-5.28793031347417,17.797735253399,-326.203047625619)) ;
#41001=CARTESIAN_POINT('Ctrl Pts',(-5.44549550112615,17.7501596065228,-326.200982006097)) ;
#41002=CARTESIAN_POINT('Ctrl Pts',(-6.21918421964404,17.5052783544626,-326.190870663147)) ;
#41003=CARTESIAN_POINT('Ctrl Pts',(-6.82533717852088,17.2779570472,-326.183031673085)) ;
#41004=CARTESIAN_POINT('Ctrl Pts',(-7.6708904691481,16.9094000598681,-326.171676439278)) ;
#41005=CARTESIAN_POINT('Ctrl Pts',(-7.92091349192079,16.793733953377,-326.168266732856)) ;
#41006=CARTESIAN_POINT('Ctrl Pts',(-8.36261070861343,16.5773361903279,-326.162118134227)) ;
#41007=CARTESIAN_POINT('Ctrl Pts',(-8.55527150335354,16.478733637576,-326.159392713031)) ;
#41008=CARTESIAN_POINT('Ctrl Pts',(-8.86339297025271,16.31417870092,-326.154954758)) ;
#41009=CARTESIAN_POINT('Ctrl Pts',(-8.97994602007168,16.2503147983607,-326.153257393324)) ;
#41010=CARTESIAN_POINT('Ctrl Pts',(-9.20584071920047,16.1233659137424,-326.149929885715)) ;
#41011=CARTESIAN_POINT('Ctrl Pts',(-9.31524462156906,16.0604062626797,-326.148300738834)) ;
#41012=CARTESIAN_POINT('Ctrl Pts',(-9.55726109582829,15.9178259398387,-326.144656989978)) ;
#41013=CARTESIAN_POINT('Ctrl Pts',(-9.68953786781783,15.8376538071998,-326.142638387349)) ;
#41014=CARTESIAN_POINT('Ctrl Pts',(-10.4286486151118,15.3769574820544,-326.131207300683)) ;
#41015=CARTESIAN_POINT('Ctrl Pts',(-11.0140633690426,14.9632193418172,-326.121543149781)) ;
#41016=CARTESIAN_POINT('Ctrl Pts',(-11.7936083460349,14.3416913768626,-326.10812379406)) ;
#41017=CARTESIAN_POINT('Ctrl Pts',(-12.009114379439,14.1617259365412,-326.104354183358)) ;
#41018=CARTESIAN_POINT('Ctrl Pts',(-12.3542122520213,13.8599966111326,-326.098264055128)) ;
#41019=CARTESIAN_POINT('Ctrl Pts',(-12.48628243131,13.7411359670686,-326.095920057442)) ;
#41020=CARTESIAN_POINT('Ctrl Pts',(-12.6756054536784,13.5657653318055,-326.092552832867)) ;
#41021=CARTESIAN_POINT('Ctrl Pts',(-12.7342291392633,13.5107501978132,-326.091509176399)) ;
#41022=CARTESIAN_POINT('Ctrl Pts',(-12.8406361853493,13.4095851697791,-326.089614595448)) ;
#41023=CARTESIAN_POINT('Ctrl Pts',(-12.8885325897359,13.3635564034161,-326.08876186636)) ;
#41024=CARTESIAN_POINT('Ctrl Pts',(-13.006591309621,13.2488760826904,-326.086659318651)) ;
#41025=CARTESIAN_POINT('Ctrl Pts',(-13.0764581698007,13.1799232442338,-326.085414273528)) ;
#41026=CARTESIAN_POINT('Ctrl Pts',(-13.3995577289955,12.8559523678614,-326.079644412894)) ;
#41027=CARTESIAN_POINT('Ctrl Pts',(-13.6458989686736,12.5941693338738,-326.075208682264)) ;
#41028=CARTESIAN_POINT('Ctrl Pts',(-14.2294065348734,11.9368517359364,-326.064416600158)) ;
#41029=CARTESIAN_POINT('Ctrl Pts',(-14.5578643461038,11.5339943484771,-326.058085891049)) ;
#41030=CARTESIAN_POINT('Ctrl Pts',(-14.9594024389937,10.9969801353638,-326.049785597036)) ;
#41031=CARTESIAN_POINT('Ctrl Pts',(-15.0483339890011,10.8749683917046,-326.047909099209)) ;
#41032=CARTESIAN_POINT('Ctrl Pts',(-15.2635443671719,10.5720099775238,-326.043266087132)) ;
#41033=CARTESIAN_POINT('Ctrl Pts',(-15.3881044935754,10.3898710992468,-326.040488655063)) ;
#41034=CARTESIAN_POINT('Ctrl Pts',(-15.582851568487,10.0939138656749,-326.035988783594)) ;
#41035=CARTESIAN_POINT('Ctrl Pts',(-15.6551069734793,9.98148214042663,-326.034282354213)) ;
#41036=CARTESIAN_POINT('Ctrl Pts',(-15.793012260236,9.76171556594236,-326.030951385076)) ;
#41037=CARTESIAN_POINT('Ctrl Pts',(-15.8587974654798,9.65447408914743,-326.029328000152)) ;
#41038=CARTESIAN_POINT('Ctrl Pts',(-16.0170810902115,9.39046023910958,-326.025335907065)) ;
#41039=CARTESIAN_POINT('Ctrl Pts',(-16.1083736941177,9.23298039244086,-326.022958417826)) ;
#41040=CARTESIAN_POINT('Ctrl Pts',(-16.381599723417,8.74527441109101,-326.015608539778)) ;
#41041=CARTESIAN_POINT('Ctrl Pts',(-16.555802027992,8.41082945303235,-326.010584770084)) ;
#41042=CARTESIAN_POINT('Ctrl Pts',(-16.939572203885,7.61585078792967,-325.998738922389)) ;
#41043=CARTESIAN_POINT('Ctrl Pts',(-17.140740743884,7.15159393811239,-325.991890758873)) ;
#41044=CARTESIAN_POINT('Ctrl Pts',(-17.3837722925309,6.52133204527432,-325.982861709737)) ;
#41045=CARTESIAN_POINT('Ctrl Pts',(-17.4426667779594,6.36212909056034,-325.980603879529)) ;
#41046=CARTESIAN_POINT('Ctrl Pts',(-17.5417503100744,6.08256443238945,-325.976691022803)) ;
#41047=CARTESIAN_POINT('Ctrl Pts',(-17.5829039898309,5.96255661439531,-325.975027910837)) ;
#41048=CARTESIAN_POINT('Ctrl Pts',(-17.6452860752128,5.77438083737191,-325.97245093015)) ;
#41049=CARTESIAN_POINT('Ctrl Pts',(-17.6673567496207,5.7064963182646,-325.971527512036)) ;
#41050=CARTESIAN_POINT('Ctrl Pts',(-17.7078934305089,5.57932481095569,-325.96981040179)) ;
#41051=CARTESIAN_POINT('Ctrl Pts',(-17.7264545574453,5.52006919564338,-325.969015484401)) ;
#41052=CARTESIAN_POINT('Ctrl Pts',(-17.7781449657395,5.35210023507433,-325.966775424559)) ;
#41053=CARTESIAN_POINT('Ctrl Pts',(-17.8105738322309,5.2431741507874,-325.965338421063)) ;
#41054=CARTESIAN_POINT('Ctrl Pts',(-17.9369822407852,4.80386800580374,-325.959594341586)) ;
#41055=CARTESIAN_POINT('Ctrl Pts',(-18.022785547168,4.47120586104699,-325.955360058512)) ;
#41056=CARTESIAN_POINT('Ctrl Pts',(-18.1100359699961,4.089427076147,-325.95055377847)) ;
#41057=CARTESIAN_POINT('Ctrl Pts',(-18.1205781502291,4.04245768659571,-325.949963407682)) ;
#41058=CARTESIAN_POINT('Ctrl Pts',(-18.2333454410775,3.53073114275622,-325.943539786307)) ;
#41059=CARTESIAN_POINT('Ctrl Pts',(-18.3178486685681,3.06224890478948,-325.937729187379)) ;
#41060=CARTESIAN_POINT('Ctrl Pts',(-18.4043699910721,2.44835224005511,-325.930046597674)) ;
#41061=CARTESIAN_POINT('Ctrl Pts',(-18.4228181606848,2.3054358417705,-325.928253731138)) ;
#41062=CARTESIAN_POINT('Ctrl Pts',(-18.4645012095539,1.94997549001014,-325.923778252274)) ;
#41063=CARTESIAN_POINT('Ctrl Pts',(-18.4857318945998,1.73721772416478,-325.921084958796)) ;
#41064=CARTESIAN_POINT('Ctrl Pts',(-18.51415571375,1.39214863794356,-325.916685232276)) ;
#41065=CARTESIAN_POINT('Ctrl Pts',(-18.5236154497839,1.26004374161199,-325.914993457558)) ;
#41066=CARTESIAN_POINT('Ctrl Pts',(-18.5393458383045,1.00157810739283,-325.911667751798)) ;
#41067=CARTESIAN_POINT('Ctrl Pts',(-18.5457399875305,0.875232013981004,
-325.910034715701)) ;
#41068=CARTESIAN_POINT('Ctrl Pts',(-18.5571323764447,0.593007407846611,
-325.906370108546)) ;
#41069=CARTESIAN_POINT('Ctrl Pts',(-18.5614588160241,0.437111364842863,
-325.90433437286)) ;
#41070=CARTESIAN_POINT('Ctrl Pts',(-18.5700970366831,-0.133194697888188,
-325.896846369808)) ;
#41071=CARTESIAN_POINT('Ctrl Pts',(-18.5624974019311,-0.547661784826543,
-325.891323016749)) ;
#41072=CARTESIAN_POINT('Ctrl Pts',(-18.5114109501745,-1.53275856261004,
-325.8780790217)) ;
#41073=CARTESIAN_POINT('Ctrl Pts',(-18.4554042895828,-2.10231683343467,
-325.870323690852)) ;
#41074=CARTESIAN_POINT('Ctrl Pts',(-18.3469444322849,-2.84912022771885,
-325.860292388118)) ;
#41075=CARTESIAN_POINT('Ctrl Pts',(-18.3180292749973,-3.02946525953145,
-325.857881615642)) ;
#41076=CARTESIAN_POINT('Ctrl Pts',(-18.2724276300795,-3.28929712620997,
-325.854438603977)) ;
#41077=CARTESIAN_POINT('Ctrl Pts',(-18.2578732486684,-3.3691470049838,-325.853384689805)) ;
#41078=CARTESIAN_POINT('Ctrl Pts',(-18.230483175355,-3.51402556500913,-325.851481682665)) ;
#41079=CARTESIAN_POINT('Ctrl Pts',(-18.2178219990464,-3.57908564931561,
-325.850630651104)) ;
#41080=CARTESIAN_POINT('Ctrl Pts',(-18.1858030504711,-3.73904358055901,
-325.848546263465)) ;
#41081=CARTESIAN_POINT('Ctrl Pts',(-18.1660505832882,-3.83386042159679,
-325.847317469275)) ;
#41082=CARTESIAN_POINT('Ctrl Pts',(-18.0768390809548,-4.24592222860317,
-325.841999027531)) ;
#41083=CARTESIAN_POINT('Ctrl Pts',(-17.9998046331222,-4.56146915516987,
-325.837981621989)) ;
#41084=CARTESIAN_POINT('Ctrl Pts',(-17.889963720349,-4.96512371569965,-325.832838182341)) ;
#41085=CARTESIAN_POINT('Ctrl Pts',(-17.8647119738382,-5.05522714890954,
-325.831689867123)) ;
#41086=CARTESIAN_POINT('Ctrl Pts',(-17.7417810987431,-5.48144268944366,
-325.826251268971)) ;
#41087=CARTESIAN_POINT('Ctrl Pts',(-17.6352910712944,-5.81493932203858,
-325.821974450875)) ;
#41088=CARTESIAN_POINT('Ctrl Pts',(-17.4288080493247,-6.40360223279718,
-325.814293693695)) ;
#41089=CARTESIAN_POINT('Ctrl Pts',(-17.3324737214144,-6.6599418875261,-325.810903726065)) ;
#41090=CARTESIAN_POINT('Ctrl Pts',(-17.1502374091235,-7.11409260197304,
-325.804785802981)) ;
#41091=CARTESIAN_POINT('Ctrl Pts',(-17.0664920831776,-7.31271526038314,
-325.802071096228)) ;
#41092=CARTESIAN_POINT('Ctrl Pts',(-16.9256125246196,-7.63123591231291,
-325.797645892108)) ;
#41093=CARTESIAN_POINT('Ctrl Pts',(-16.8706170308459,-7.75205790872377,
-325.795950392814)) ;
#41094=CARTESIAN_POINT('Ctrl Pts',(-16.7607708984117,-7.9866772665144,-325.792623516394)) ;
#41095=CARTESIAN_POINT('Ctrl Pts',(-16.7060451800202,-8.10052524579647,
-325.790993101869)) ;
#41096=CARTESIAN_POINT('Ctrl Pts',(-16.568180719477,-8.37998955989924,-325.786950548933)) ;
#41097=CARTESIAN_POINT('Ctrl Pts',(-16.4837161701132,-8.54493642082568,
-325.784529086427)) ;
#41098=CARTESIAN_POINT('Ctrl Pts',(-16.0971887345808,-9.27270188725517,
-325.77368933117)) ;
#41099=CARTESIAN_POINT('Ctrl Pts',(-15.7686699157909,-9.82097393334736,
-325.76508662222)) ;
#41100=CARTESIAN_POINT('Ctrl Pts',(-15.2393019446545,-10.6091816656868,
-325.752299203636)) ;
#41101=CARTESIAN_POINT('Ctrl Pts',(-15.0596028902879,-10.8627538175177,
-325.748119529675)) ;
#41102=CARTESIAN_POINT('Ctrl Pts',(-14.7604916413494,-11.2631308876633,
-325.741471638564)) ;
#41103=CARTESIAN_POINT('Ctrl Pts',(-14.6450524638065,-11.4128291603238,
-325.738974913005)) ;
#41104=CARTESIAN_POINT('Ctrl Pts',(-14.476208365781,-11.625000452875,-325.735434785477)) ;
#41105=CARTESIAN_POINT('Ctrl Pts',(-14.4246434895597,-11.688922294351,-325.734368059087)) ;
#41106=CARTESIAN_POINT('Ctrl Pts',(-14.330797302,-11.8036909810578,-325.732454144424)) ;
#41107=CARTESIAN_POINT('Ctrl Pts',(-14.2886653675355,-11.8546579073339,
-325.731604852189)) ;
#41108=CARTESIAN_POINT('Ctrl Pts',(-14.1851332911785,-11.9785466666369,
-325.729541349712)) ;
#41109=CARTESIAN_POINT('Ctrl Pts',(-14.1234420912199,-12.0512227706054,
-325.728331455586)) ;
#41110=CARTESIAN_POINT('Ctrl Pts',(-13.8648347674357,-12.351165157706,-325.723333613264)) ;
#41111=CARTESIAN_POINT('Ctrl Pts',(-13.6629711230557,-12.5741061212602,
-325.719607369629)) ;
#41112=CARTESIAN_POINT('Ctrl Pts',(-13.3635368286466,-12.8890770409518,
-325.714257690539)) ;
#41113=CARTESIAN_POINT('Ctrl Pts',(-13.2702451301722,-12.9851075370062,
-325.712614800457)) ;
#41114=CARTESIAN_POINT('Ctrl Pts',(-12.8433961009566,-13.4150829235332,
-325.705188382038)) ;
#41115=CARTESIAN_POINT('Ctrl Pts',(-12.4982168866682,-13.7372430895527,
-325.699423992928)) ;
#41116=CARTESIAN_POINT('Ctrl Pts',(-12.0326121885731,-14.139707253328,-325.691796667802)) ;
#41117=CARTESIAN_POINT('Ctrl Pts',(-11.9230029593247,-14.2322548341958,
-325.690011675223)) ;
#41118=CARTESIAN_POINT('Ctrl Pts',(-11.6478909787771,-14.4591343655779,
-325.685552069738)) ;
#41119=CARTESIAN_POINT('Ctrl Pts',(-11.481126753129,-14.5919038890302,-325.682866800028)) ;
#41120=CARTESIAN_POINT('Ctrl Pts',(-11.2071875306039,-14.8023969982428,
-325.678476618034)) ;
#41121=CARTESIAN_POINT('Ctrl Pts',(-11.1014024729739,-14.8818974701496,
-325.676786237508)) ;
#41122=CARTESIAN_POINT('Ctrl Pts',(-10.8927813662166,-15.0352198355038,
-325.67346093801)) ;
#41123=CARTESIAN_POINT('Ctrl Pts',(-10.790022231546,-15.1091343756911,-325.671826888349)) ;
#41124=CARTESIAN_POINT('Ctrl Pts',(-10.5587196351409,-15.2719469179462,
-325.668156886081)) ;
#41125=CARTESIAN_POINT('Ctrl Pts',(-10.4297933317919,-15.3602843058016,
-325.666116726378)) ;
#41126=CARTESIAN_POINT('Ctrl Pts',(-9.7132229859223,-15.8380803673515,-325.654809199395)) ;
#41127=CARTESIAN_POINT('Ctrl Pts',(-9.10488067770076,-16.1954509180499,
-325.645300089706)) ;
#41128=CARTESIAN_POINT('Ctrl Pts',(-8.10600976264098,-16.7081312894147,
-325.630186152228)) ;
#41129=CARTESIAN_POINT('Ctrl Pts',(-7.72798763877837,-16.8863037300734,
-325.624579423746)) ;
#41130=CARTESIAN_POINT('Ctrl Pts',(-7.25212406730502,-17.0912627823632,
-325.617780427003)) ;
#41131=CARTESIAN_POINT('Ctrl Pts',(-7.15965064798743,-17.1302063509282,
-325.616471214611)) ;
#41132=CARTESIAN_POINT('Ctrl Pts',(-7.00518674697434,-17.1937868704601,
-325.614307034721)) ;
#41133=CARTESIAN_POINT('Ctrl Pts',(-6.9433710771508,-17.2188427726664,-325.613447003777)) ;
#41134=CARTESIAN_POINT('Ctrl Pts',(-6.80784554966059,-17.272927196313,-325.611575351122)) ;
#41135=CARTESIAN_POINT('Ctrl Pts',(-6.73408234506195,-17.301818111114,-325.610565365285)) ;
#41136=CARTESIAN_POINT('Ctrl Pts',(-6.50115134899761,-17.3913351960528,
-325.607400274459)) ;
#41137=CARTESIAN_POINT('Ctrl Pts',(-6.34133275225464,-17.4502437766335,
-325.605264103372)) ;
#41138=CARTESIAN_POINT('Ctrl Pts',(-6.06650171124781,-17.5472712922293,
-325.601635355937)) ;
#41139=CARTESIAN_POINT('Ctrl Pts',(-5.95188532901854,-17.5864787233345,
-325.600135179089)) ;
#41140=CARTESIAN_POINT('Ctrl Pts',(-5.26415783401835,-17.8142399666871,
-325.591194184243)) ;
#41141=CARTESIAN_POINT('Ctrl Pts',(-4.68251674137203,-17.9758877990413,
-325.583869552335)) ;
#41142=CARTESIAN_POINT('Ctrl Pts',(-3.9358674414343,-18.1446891396433,-325.574408967758)) ;
#41143=CARTESIAN_POINT('Ctrl Pts',(-3.77723391141671,-18.1783745256108,
-325.57239660554)) ;
#41144=CARTESIAN_POINT('Ctrl Pts',(-3.51105965157956,-18.2312612622896,
-325.569010416946)) ;
#41145=CARTESIAN_POINT('Ctrl Pts',(-3.40375405195838,-18.2515995303417,
-325.567642728785)) ;
#41146=CARTESIAN_POINT('Ctrl Pts',(-3.12248502091476,-18.3023433694199,
-325.564048907471)) ;
#41147=CARTESIAN_POINT('Ctrl Pts',(-2.94825644327139,-18.3312157078248,
-325.561813873351)) ;
#41148=CARTESIAN_POINT('Ctrl Pts',(-2.64880250539709,-18.376460092909,-325.557953169476)) ;
#41149=CARTESIAN_POINT('Ctrl Pts',(-2.52377325041383,-18.394048189186,-325.556335531848)) ;
#41150=CARTESIAN_POINT('Ctrl Pts',(-2.2639905433933,-18.4278937074565,-325.552961679349)) ;
#41151=CARTESIAN_POINT('Ctrl Pts',(-2.12921855974028,-18.4439515270494,
-325.551204263126)) ;
#41152=CARTESIAN_POINT('Ctrl Pts',(-1.76313488556778,-18.4835036666961,
-325.546410945793)) ;
#41153=CARTESIAN_POINT('Ctrl Pts',(-1.53153869931223,-18.5041330874849,
-325.543357138461)) ;
#41154=CARTESIAN_POINT('Ctrl Pts',(-1.05099695682863,-18.5378537298776,
-325.53698145632)) ;
#41155=CARTESIAN_POINT('Ctrl Pts',(-0.802051533335079,-18.5502918724665,
-325.533656708231)) ;
#41156=CARTESIAN_POINT('Ctrl Pts',(-0.0245848552779535,-18.5734566824771,
-325.523229903037)) ;
#41157=CARTESIAN_POINT('Ctrl Pts',(0.504192435468138,-18.5666283059729,
-325.516069508624)) ;
#41158=CARTESIAN_POINT('Ctrl Pts',(1.15626000415832,-18.5303281581978,-325.507337090578)) ;
#41159=CARTESIAN_POINT('Ctrl Pts',(1.28049166112913,-18.5221580816199,-325.505678197775)) ;
#41160=CARTESIAN_POINT('Ctrl Pts',(1.56274218715176,-18.5007426625752,-325.501926275503)) ;
#41161=CARTESIAN_POINT('Ctrl Pts',(1.72069264647002,-18.4867211579014,-325.499838798793)) ;
#41162=CARTESIAN_POINT('Ctrl Pts',(1.95529386563328,-18.4628625149745,-325.496765555104)) ;
#41163=CARTESIAN_POINT('Ctrl Pts',(2.03209402876608,-18.4545674624936,-325.495763848179)) ;
#41164=CARTESIAN_POINT('Ctrl Pts',(2.17494325627519,-18.4382360315584,-325.493910226276)) ;
#41165=CARTESIAN_POINT('Ctrl Pts',(2.24100506531518,-18.430323448347,-325.493056967061)) ;
#41166=CARTESIAN_POINT('Ctrl Pts',(2.41002848499342,-18.4091563806101,-325.490882827947)) ;
#41167=CARTESIAN_POINT('Ctrl Pts',(2.51292415374054,-18.39539312406,-325.489567724326)) ;
#41168=CARTESIAN_POINT('Ctrl Pts',(2.87171676616319,-18.3443346741717,-325.485003955096)) ;
#41169=CARTESIAN_POINT('Ctrl Pts',(3.12694585899099,-18.3025567039776,-325.481796194505)) ;
#41170=CARTESIAN_POINT('Ctrl Pts',(3.9556834938046,-18.1490605227644,-325.471408792808)) ;
#41171=CARTESIAN_POINT('Ctrl Pts',(4.5248053677219,-18.0156034468714,-325.464310293688)) ;
#41172=CARTESIAN_POINT('Ctrl Pts',(5.24040308298934,-17.8117439215308,-325.455111551622)) ;
#41173=CARTESIAN_POINT('Ctrl Pts',(5.39354816743352,-17.7659698325353,-325.453127483824)) ;
#41174=CARTESIAN_POINT('Ctrl Pts',(5.76482770245515,-17.6497534952484,-325.448271818349)) ;
#41175=CARTESIAN_POINT('Ctrl Pts',(5.98228536587229,-17.5772380767641,-325.445389058572)) ;
#41176=CARTESIAN_POINT('Ctrl Pts',(6.32573835948047,-17.4555950540187,-325.440763757312)) ;
#41177=CARTESIAN_POINT('Ctrl Pts',(6.45263589382466,-17.4090853992907,-325.439038982128)) ;
#41178=CARTESIAN_POINT('Ctrl Pts',(6.69730699405274,-17.3163674331531,-325.435681260763)) ;
#41179=CARTESIAN_POINT('Ctrl Pts',(6.8151384586883,-17.2703326484286,-325.434049591425)) ;
#41180=CARTESIAN_POINT('Ctrl Pts',(7.09787392482434,-17.1565284471316,-325.43009847591)) ;
#41181=CARTESIAN_POINT('Ctrl Pts',(7.26229007903832,-17.0875810245551,-325.427771021031)) ;
#41182=CARTESIAN_POINT('Ctrl Pts',(7.79112692535068,-16.8568033234498,-325.420189384574)) ;
#41183=CARTESIAN_POINT('Ctrl Pts',(8.15133335726371,-16.6855997850491,-325.414874612666)) ;
#41184=CARTESIAN_POINT('Ctrl Pts',(8.94611242424129,-16.2759641295029,-325.402870992047)) ;
#41185=CARTESIAN_POINT('Ctrl Pts',(9.37721659556207,-16.0314610789527,-325.396164328099)) ;
#41186=CARTESIAN_POINT('Ctrl Pts',(9.90043763331762,-15.7063799550682,-325.387932106646)) ;
#41187=CARTESIAN_POINT('Ctrl Pts',(10.0022285476579,-15.6417537619149,-325.386326382459)) ;
#41188=CARTESIAN_POINT('Ctrl Pts',(10.2335904195664,-15.491682084193,-325.382672717367)) ;
#41189=CARTESIAN_POINT('Ctrl Pts',(10.3627341090871,-15.4055940681663,-325.380630349876)) ;
#41190=CARTESIAN_POINT('Ctrl Pts',(10.5540326016346,-15.2745792782623,-325.377609275737)) ;
#41191=CARTESIAN_POINT('Ctrl Pts',(10.6170130197322,-15.2308703245855,-325.376615370024)) ;
#41192=CARTESIAN_POINT('Ctrl Pts',(10.7343171680542,-15.1483790927794,-325.374766917203)) ;
#41193=CARTESIAN_POINT('Ctrl Pts',(10.7887058639316,-15.1096915909759,-325.373911133361)) ;
#41194=CARTESIAN_POINT('Ctrl Pts',(10.9282796977612,-15.0092727764472,-325.37171701207)) ;
#41195=CARTESIAN_POINT('Ctrl Pts',(11.0131509902948,-14.9471091433723,-325.370384679379)) ;
#41196=CARTESIAN_POINT('Ctrl Pts',(11.5711639756845,-14.5310618062259,-325.361622324033)) ;
#41197=CARTESIAN_POINT('Ctrl Pts',(12.0277115105238,-14.1554849378218,-325.354430083177)) ;
#41198=CARTESIAN_POINT('Ctrl Pts',(12.7329177717943,-13.5165619355861,-325.342766824898)) ;
#41199=CARTESIAN_POINT('Ctrl Pts',(12.9931457553622,-13.2666048576102,-325.338331924461)) ;
#41200=CARTESIAN_POINT('Ctrl Pts',(13.4264472849148,-12.8254195063637,-325.330638021702)) ;
#41201=CARTESIAN_POINT('Ctrl Pts',(13.603123235126,-12.6378760115532,-325.327406543785)) ;
#41202=CARTESIAN_POINT('Ctrl Pts',(13.8696971979593,-12.3428359670296,-325.322366760395)) ;
#41203=CARTESIAN_POINT('Ctrl Pts',(13.9623774654911,-12.23789669478,-325.320582564457)) ;
#41204=CARTESIAN_POINT('Ctrl Pts',(14.1355076593842,-12.0373391601769,-325.317186642055)) ;
#41205=CARTESIAN_POINT('Ctrl Pts',(14.2161965424819,-11.9419373076176,-325.31557709674)) ;
#41206=CARTESIAN_POINT('Ctrl Pts',(14.4002451370054,-11.7198198311237,-325.311842437595)) ;
#41207=CARTESIAN_POINT('Ctrl Pts',(14.5029060275426,-11.592538700461,-325.30971168009)) ;
#41208=CARTESIAN_POINT('Ctrl Pts',(14.8825971223937,-11.1088506580209,-325.301650051956)) ;
#41209=CARTESIAN_POINT('Ctrl Pts',(15.1482794231129,-10.7437371768272,-325.295632125791)) ;
#41210=CARTESIAN_POINT('Ctrl Pts',(15.4242032212069,-10.3339378917946,-325.288995507223)) ;
#41211=CARTESIAN_POINT('Ctrl Pts',(15.4478948784972,-10.298488295994,-325.288422384577)) ;
#41212=CARTESIAN_POINT('Ctrl Pts',(15.6055720106843,-10.0607891601424,-325.284586363474)) ;
#41213=CARTESIAN_POINT('Ctrl Pts',(15.7357042727936,-9.85601173424314,-325.281314707487)) ;
#41214=CARTESIAN_POINT('Ctrl Pts',(16.0060827453585,-9.41153047904062,-325.274312698051)) ;
#41215=CARTESIAN_POINT('Ctrl Pts',(16.1450402359084,-9.1711104506302,-325.270585120915)) ;
#41216=CARTESIAN_POINT('Ctrl Pts',(16.3634041503653,-8.77294935741677,-325.264552869295)) ;
#41217=CARTESIAN_POINT('Ctrl Pts',(16.4460449192951,-8.61703211764601,-325.262225213585)) ;
#41218=CARTESIAN_POINT('Ctrl Pts',(16.5629966772832,-8.38856799226436,-325.258876582447)) ;
#41219=CARTESIAN_POINT('Ctrl Pts',(16.5990797915779,-8.31693946047766,-325.257835477423)) ;
#41220=CARTESIAN_POINT('Ctrl Pts',(16.6642160099039,-8.18552516378484,-325.255942946683)) ;
#41221=CARTESIAN_POINT('Ctrl Pts',(16.6934142628742,-8.1258130469061,-325.255089749927)) ;
#41222=CARTESIAN_POINT('Ctrl Pts',(16.7650845084634,-7.97722653036488,-325.252982469829)) ;
#41223=CARTESIAN_POINT('Ctrl Pts',(16.8071710884756,-7.88816846525244,-325.251733214866)) ;
#41224=CARTESIAN_POINT('Ctrl Pts',(16.9939949698223,-7.48455263080776,-325.2461251409)) ;
#41225=CARTESIAN_POINT('Ctrl Pts',(17.1306243216637,-7.16631736648492,-325.241848381673)) ;
#41226=CARTESIAN_POINT('Ctrl Pts',(17.4104721685707,-6.46068100472641,-325.232523921038)) ;
#41227=CARTESIAN_POINT('Ctrl Pts',(17.5498269439641,-6.07194487904033,-325.227487689554)) ;
#41228=CARTESIAN_POINT('Ctrl Pts',(17.7607345986231,-5.41547361531304,-325.219000026489)) ;
#41229=CARTESIAN_POINT('Ctrl Pts',(17.8394638390499,-5.15020170113004,-325.215575541175)) ;
#41230=CARTESIAN_POINT('Ctrl Pts',(17.9693273399642,-4.67385171626183,-325.209403998361)) ;
#41231=CARTESIAN_POINT('Ctrl Pts',(18.0227423254854,-4.46344863832101,-325.206670579502)) ;
#41232=CARTESIAN_POINT('Ctrl Pts',(18.1029198227921,-4.12267946500903,-325.20222310564)) ;
#41233=CARTESIAN_POINT('Ctrl Pts',(18.1319916077016,-3.99287770389717,-325.200524347972)) ;
#41234=CARTESIAN_POINT('Ctrl Pts',(18.1859137182883,-3.73937923467862,-325.197196350214)) ;
#41235=CARTESIAN_POINT('Ctrl Pts',(18.2109030017392,-3.61571938034208,-325.195568130975)) ;
#41236=CARTESIAN_POINT('Ctrl Pts',(18.2636618278296,-3.34020713448863,-325.191929396364)) ;
#41237=CARTESIAN_POINT('Ctrl Pts',(18.2908017598256,-3.18824370926364,-325.189914919715)) ;
#41238=CARTESIAN_POINT('Ctrl Pts',(18.4338319645526,-2.32533783791376,-325.178435351717)) ;
#41239=CARTESIAN_POINT('Ctrl Pts',(18.5101644333385,-1.60846537411794,-325.168715140381)) ;
#41240=CARTESIAN_POINT('Ctrl Pts',(18.544654593745,-0.888979977948195,-325.159020379883)) ;
#41241=CARTESIAN_POINT('Ctrl Pts',(18.544654593743,-0.888979977990129,-324.862668413757)) ;
#41242=CARTESIAN_POINT('Ctrl Pts',(18.5381258541361,-1.02517339509664,-324.864435224152)) ;
#41243=CARTESIAN_POINT('Ctrl Pts',(18.5300969633876,-1.16129131229351,-324.866211571098)) ;
#41244=CARTESIAN_POINT('Ctrl Pts',(18.4922244160714,-1.70196523688201,-324.873308733905)) ;
#41245=CARTESIAN_POINT('Ctrl Pts',(18.4506251769581,-2.10558271819744,-324.8787015583)) ;
#41246=CARTESIAN_POINT('Ctrl Pts',(18.3400775793385,-2.9165921489683,-324.889674525018)) ;
#41247=CARTESIAN_POINT('Ctrl Pts',(18.2706864423052,-3.32369851936604,-324.895253226547)) ;
#41248=CARTESIAN_POINT('Ctrl Pts',(18.1186365610978,-4.06547361825138,-324.905427810891)) ;
#41249=CARTESIAN_POINT('Ctrl Pts',(18.0401208576654,-4.40080752377932,-324.91003043826)) ;
#41250=CARTESIAN_POINT('Ctrl Pts',(17.9272125024931,-4.82900114681951,-324.915838807011)) ;
#41251=CARTESIAN_POINT('Ctrl Pts',(17.901342354071,-4.92403717989873,-324.917123445081)) ;
#41252=CARTESIAN_POINT('Ctrl Pts',(17.8567493604272,-5.08285545398464,-324.919260077664)) ;
#41253=CARTESIAN_POINT('Ctrl Pts',(17.8384380204821,-5.14675104435503,-324.920116839305)) ;
#41254=CARTESIAN_POINT('Ctrl Pts',(17.797273715886,-5.28753069564596,-324.921997661633)) ;
#41255=CARTESIAN_POINT('Ctrl Pts',(17.7742648936657,-5.36436763180048,-324.923019910421)) ;
#41256=CARTESIAN_POINT('Ctrl Pts',(17.6990379175872,-5.60978628222489,-324.926274481705)) ;
#41257=CARTESIAN_POINT('Ctrl Pts',(17.6449136201815,-5.77777369483103,-324.928486348787)) ;
#41258=CARTESIAN_POINT('Ctrl Pts',(17.499473894113,-6.20806266031709,-324.934137004373)) ;
#41259=CARTESIAN_POINT('Ctrl Pts',(17.4046529861399,-6.46913312500787,-324.937551384741)) ;
#41260=CARTESIAN_POINT('Ctrl Pts',(17.2181084296283,-6.94891605348687,-324.943863349554)) ;
#41261=CARTESIAN_POINT('Ctrl Pts',(17.1279820158107,-7.16818835494682,-324.946762713302)) ;
#41262=CARTESIAN_POINT('Ctrl Pts',(17.0084701558398,-7.44382018113507,-324.950447884027)) ;
#41263=CARTESIAN_POINT('Ctrl Pts',(16.9829611138028,-7.50183629094492,-324.951225840286)) ;
#41264=CARTESIAN_POINT('Ctrl Pts',(16.7836550600635,-7.94889828041912,-324.957240520559)) ;
#41265=CARTESIAN_POINT('Ctrl Pts',(16.5968085535664,-8.33198690246369,-324.962514623405)) ;
#41266=CARTESIAN_POINT('Ctrl Pts',(16.3253925464621,-8.84303853742481,-324.969800174043)) ;
#41267=CARTESIAN_POINT('Ctrl Pts',(16.2521793193965,-8.97688362698648,-324.971731869571)) ;
#41268=CARTESIAN_POINT('Ctrl Pts',(16.1156130648748,-9.2193998176518,-324.975278018854)) ;
#41269=CARTESIAN_POINT('Ctrl Pts',(16.0527892801765,-9.32835857630667,-324.976888520089)) ;
#41270=CARTESIAN_POINT('Ctrl Pts',(15.9208979907835,-9.55182635565259,-324.980228375585)) ;
#41271=CARTESIAN_POINT('Ctrl Pts',(15.851690659593,-9.66624449981995,-324.981958715949)) ;
#41272=CARTESIAN_POINT('Ctrl Pts',(15.6648100359974,-9.96780269544494,-324.986573771121)) ;
#41273=CARTESIAN_POINT('Ctrl Pts',(15.5450203621148,-10.1536055521247,-324.989474091266)) ;
#41274=CARTESIAN_POINT('Ctrl Pts',(15.337645955908,-10.4629841408862,-324.994397037497)) ;
#41275=CARTESIAN_POINT('Ctrl Pts',(15.2518152073156,-10.5877076560748,-324.996408000453)) ;
#41276=CARTESIAN_POINT('Ctrl Pts',(14.8630810511037,-11.1380526088268,-325.00539307083)) ;
#41277=CARTESIAN_POINT('Ctrl Pts',(14.543819364428,-11.5518271631589,-325.012456914511)) ;
#41278=CARTESIAN_POINT('Ctrl Pts',(13.9807375303385,-12.221194882475,-325.024214133831)) ;
#41279=CARTESIAN_POINT('Ctrl Pts',(13.7463096200732,-12.4842940911381,-325.028926108407)) ;
#41280=CARTESIAN_POINT('Ctrl Pts',(13.4361921249088,-12.8130074460888,-325.034855195076)) ;
#41281=CARTESIAN_POINT('Ctrl Pts',(13.367264649142,-12.8849002508042,-325.036154522666)) ;
#41282=CARTESIAN_POINT('Ctrl Pts',(13.2512826114673,-13.0039395803706,-325.038307588683)) ;
#41283=CARTESIAN_POINT('Ctrl Pts',(13.2045468541549,-13.0513937137986,-325.03916627127)) ;
#41284=CARTESIAN_POINT('Ctrl Pts',(13.1013934351152,-13.1550114603232,-325.04104144792)) ;
#41285=CARTESIAN_POINT('Ctrl Pts',(13.0448679648698,-13.2110656748541,-325.042056236811)) ;
#41286=CARTESIAN_POINT('Ctrl Pts',(12.8645682258735,-13.3875768209156,-325.045256092971)) ;
#41287=CARTESIAN_POINT('Ctrl Pts',(12.7394726213125,-13.5066711770952,-325.047421642113)) ;
#41288=CARTESIAN_POINT('Ctrl Pts',(12.4158267578886,-13.8062937648796,-325.052911163064)) ;
#41289=CARTESIAN_POINT('Ctrl Pts',(12.2149909927262,-13.9842946556543,-325.056212358608)) ;
#41290=CARTESIAN_POINT('Ctrl Pts',(11.4385647355043,-14.6429501066623,-325.068701015128)) ;
#41291=CARTESIAN_POINT('Ctrl Pts',(10.8378996366233,-15.0929348587716,-325.077838873132)) ;
#41292=CARTESIAN_POINT('Ctrl Pts',(10.0745518696503,-15.5956680629472,-325.089354048055)) ;
#41293=CARTESIAN_POINT('Ctrl Pts',(9.93623689516225,-15.6841529562926,-325.091435334465)) ;
#41294=CARTESIAN_POINT('Ctrl Pts',(9.69056454589318,-15.8367638556577,-325.095126126287)) ;
#41295=CARTESIAN_POINT('Ctrl Pts',(9.58369889118122,-15.9016617417581,-325.096729632167)) ;
#41296=CARTESIAN_POINT('Ctrl Pts',(9.35609379009608,-16.0367550127542,-325.100141568057)) ;
#41297=CARTESIAN_POINT('Ctrl Pts',(9.23520129563525,-16.1066774756576,-325.101951922738)) ;
#41298=CARTESIAN_POINT('Ctrl Pts',(8.89090976266209,-16.3006599966445,-325.107102603623)) ;
#41299=CARTESIAN_POINT('Ctrl Pts',(8.66572263367698,-16.4214811621469,-325.110465842043)) ;
#41300=CARTESIAN_POINT('Ctrl Pts',(8.26984674924257,-16.6234719390595,-325.116362134229)) ;
#41301=CARTESIAN_POINT('Ctrl Pts',(8.10027912422241,-16.7067549975803,-325.118882558934)) ;
#41302=CARTESIAN_POINT('Ctrl Pts',(7.60594996510282,-16.9402491682121,-325.126205223727)) ;
#41303=CARTESIAN_POINT('Ctrl Pts',(7.27807995788663,-17.0836784241801,-325.131032586518)) ;
#41304=CARTESIAN_POINT('Ctrl Pts',(6.90056669914075,-17.2359829292881,-325.136512491861)) ;
#41305=CARTESIAN_POINT('Ctrl Pts',(6.85478891652288,-17.2542399780111,-325.137175669494)) ;
#41306=CARTESIAN_POINT('Ctrl Pts',(6.49016627604845,-17.397978288492,-325.142446342933)) ;
#41307=CARTESIAN_POINT('Ctrl Pts',(6.16797525620258,-17.5147934272467,-325.147034723616)) ;
#41308=CARTESIAN_POINT('Ctrl Pts',(5.734919285191,-17.6583720232006,-325.153038767898)) ;
#41309=CARTESIAN_POINT('Ctrl Pts',(5.6267763662319,-17.6931283130446,-325.154524629484)) ;
#41310=CARTESIAN_POINT('Ctrl Pts',(5.45904281214665,-17.7453432039354,-325.156804844848)) ;
#41311=CARTESIAN_POINT('Ctrl Pts',(5.39967217022753,-17.7634989323192,-325.157607240794)) ;
#41312=CARTESIAN_POINT('Ctrl Pts',(5.27183163679566,-17.8018928247677,-325.159324037637)) ;
#41313=CARTESIAN_POINT('Ctrl Pts',(5.20333379095375,-17.8220345199068,-325.160237184869)) ;
#41314=CARTESIAN_POINT('Ctrl Pts',(5.01272906233195,-17.8768890326417,-325.162761517157)) ;
#41315=CARTESIAN_POINT('Ctrl Pts',(4.89037967544262,-17.9107454017938,-325.16436301573)) ;
#41316=CARTESIAN_POINT('Ctrl Pts',(4.60350095171625,-17.986971412684,-325.168083219911)) ;
#41317=CARTESIAN_POINT('Ctrl Pts',(4.43871803237274,-18.0283427960947,-325.170193471739)) ;
#41318=CARTESIAN_POINT('Ctrl Pts',(3.78020831113551,-18.1840963547799,-325.178554893562)) ;
#41319=CARTESIAN_POINT('Ctrl Pts',(3.28245640292659,-18.2805037230435,-325.184721444914)) ;
#41320=CARTESIAN_POINT('Ctrl Pts',(2.41451156324132,-18.4120156269892,-325.195516034648)) ;
#41321=CARTESIAN_POINT('Ctrl Pts',(2.04605487618976,-18.4565935155754,-325.200109836829)) ;
#41322=CARTESIAN_POINT('Ctrl Pts',(1.49315527545507,-18.5067253303527,-325.207081930661)) ;
#41323=CARTESIAN_POINT('Ctrl Pts',(1.30956260823679,-18.5206220401048,-325.209409581076)) ;
#41324=CARTESIAN_POINT('Ctrl Pts',(0.999897604728933,-18.5394339867642,
-325.21336141677)) ;
#41325=CARTESIAN_POINT('Ctrl Pts',(0.873926774540049,-18.545798977377,-325.214976158995)) ;
#41326=CARTESIAN_POINT('Ctrl Pts',(0.614946778249287,-18.5562400667901,
-325.21831153593)) ;
#41327=CARTESIAN_POINT('Ctrl Pts',(0.481938917505182,-18.5601707905231,
-325.220033018631)) ;
#41328=CARTESIAN_POINT('Ctrl Pts',(0.131602864138187,-18.5667556402194,
-325.224590087067)) ;
#41329=CARTESIAN_POINT('Ctrl Pts',(-0.0857493167577347,-18.5670240241271,
-325.227440556212)) ;
#41330=CARTESIAN_POINT('Ctrl Pts',(-0.580212184113941,-18.5589517324173,
-325.233974174773)) ;
#41331=CARTESIAN_POINT('Ctrl Pts',(-0.857232122236112,-18.548220622205,
-325.237669859553)) ;
#41332=CARTESIAN_POINT('Ctrl Pts',(-1.54599096097788,-18.5060763017575,
-325.246920353621)) ;
#41333=CARTESIAN_POINT('Ctrl Pts',(-1.95711882222,-18.4671230458694,-325.25249888158)) ;
#41334=CARTESIAN_POINT('Ctrl Pts',(-2.70907867008816,-18.370482242093,-325.262686461108)) ;
#41335=CARTESIAN_POINT('Ctrl Pts',(-3.05025879526739,-18.3169224265755,
-325.267302063434)) ;
#41336=CARTESIAN_POINT('Ctrl Pts',(-3.48655755233183,-18.235901715154,-325.273122568471)) ;
#41337=CARTESIAN_POINT('Ctrl Pts',(-3.58322389406087,-18.2171540449279,
-325.274406851151)) ;
#41338=CARTESIAN_POINT('Ctrl Pts',(-3.74488205907087,-18.1844652169232,
-325.27654308744)) ;
#41339=CARTESIAN_POINT('Ctrl Pts',(-3.8099563325229,-18.1709424533239,-325.277399803896)) ;
#41340=CARTESIAN_POINT('Ctrl Pts',(-3.95341210292426,-18.1403271116726,
-325.279280769134)) ;
#41341=CARTESIAN_POINT('Ctrl Pts',(-4.03175811277579,-18.1230753879647,
-325.280303203378)) ;
#41342=CARTESIAN_POINT('Ctrl Pts',(-4.28218568938222,-18.0662271788778,
-325.283559146377)) ;
#41343=CARTESIAN_POINT('Ctrl Pts',(-4.45381534758566,-18.0246832926122,
-325.285772175941)) ;
#41344=CARTESIAN_POINT('Ctrl Pts',(-4.89402441204554,-17.9114568438308,
-325.291426913013)) ;
#41345=CARTESIAN_POINT('Ctrl Pts',(-5.16163387062843,-17.8361794505509,
-325.294844170377)) ;
#41346=CARTESIAN_POINT('Ctrl Pts',(-5.65180806111612,-17.6863394776365,
-325.301129018385)) ;
#41347=CARTESIAN_POINT('Ctrl Pts',(-5.87484368838931,-17.6135104430597,
-325.303998537316)) ;
#41348=CARTESIAN_POINT('Ctrl Pts',(-6.18086110857364,-17.507125514711,-325.307972468968)) ;
#41349=CARTESIAN_POINT('Ctrl Pts',(-6.26507008961982,-17.4771675221502,
-325.309069857811)) ;
#41350=CARTESIAN_POINT('Ctrl Pts',(-6.68374446566345,-17.3248061396228,
-325.314549079391)) ;
#41351=CARTESIAN_POINT('Ctrl Pts',(-7.01485493331593,-17.1934044746438,
-325.31895796167)) ;
#41352=CARTESIAN_POINT('Ctrl Pts',(-7.51600863644812,-16.9776327487746,
-325.325804512307)) ;
#41353=CARTESIAN_POINT('Ctrl Pts',(-7.68887982183782,-16.9000451625378,
-325.328198292907)) ;
#41354=CARTESIAN_POINT('Ctrl Pts',(-7.97556951367066,-16.7660643561651,
-325.332227300152)) ;
#41355=CARTESIAN_POINT('Ctrl Pts',(-8.09005146554495,-16.7111247465066,
-325.333852164385)) ;
#41356=CARTESIAN_POINT('Ctrl Pts',(-8.32213421134901,-16.5968049626977,
-325.337179926963)) ;
#41357=CARTESIAN_POINT('Ctrl Pts',(-8.4396847228047,-16.5373387980106,-325.338883377208)) ;
#41358=CARTESIAN_POINT('Ctrl Pts',(-8.74276016887112,-16.3799465676584,
-325.3433224931)) ;
#41359=CARTESIAN_POINT('Ctrl Pts',(-8.92727581063615,-16.2801182826145,
-325.346071612035)) ;
#41360=CARTESIAN_POINT('Ctrl Pts',(-9.23215653176139,-16.1084270001712,
-325.35069006627)) ;
#41361=CARTESIAN_POINT('Ctrl Pts',(-9.35347079505296,-16.0382891442111,
-325.352548253763)) ;
#41362=CARTESIAN_POINT('Ctrl Pts',(-9.8632502919117,-15.7358086830335,-325.360439330944)) ;
#41363=CARTESIAN_POINT('Ctrl Pts',(-10.2439437333666,-15.4906745086136,
-325.366541656486)) ;
#41364=CARTESIAN_POINT('Ctrl Pts',(-10.7846995607814,-15.113814549437,-325.375418303177)) ;
#41365=CARTESIAN_POINT('Ctrl Pts',(-10.9521215306519,-14.9929373009771,
-325.378196399511)) ;
#41366=CARTESIAN_POINT('Ctrl Pts',(-11.2393775048666,-14.7781613737659,
-325.382997414465)) ;
#41367=CARTESIAN_POINT('Ctrl Pts',(-11.3601376206761,-14.6855348424388,
-325.38502658867)) ;
#41368=CARTESIAN_POINT('Ctrl Pts',(-11.6005257561328,-14.4964105542178,
-325.389078154469)) ;
#41369=CARTESIAN_POINT('Ctrl Pts',(-11.7201218887997,-14.3998909655259,
-325.391100128609)) ;
#41370=CARTESIAN_POINT('Ctrl Pts',(-11.8973539200183,-14.253185784914,-325.394097570721)) ;
#41371=CARTESIAN_POINT('Ctrl Pts',(-11.9559006636398,-14.2041111886541,
-325.39508790761)) ;
#41372=CARTESIAN_POINT('Ctrl Pts',(-12.0657119565852,-14.1109060521385,
-325.396944301609)) ;
#41373=CARTESIAN_POINT('Ctrl Pts',(-12.1170413620737,-14.0668540637558,
-325.397811436519)) ;
#41374=CARTESIAN_POINT('Ctrl Pts',(-12.2486894644291,-13.952615625416,-325.400035199504)) ;
#41375=CARTESIAN_POINT('Ctrl Pts',(-12.328646205604,-13.8820156740331,-325.401385665571)) ;
#41376=CARTESIAN_POINT('Ctrl Pts',(-12.4604768780668,-13.7635748947493,
-325.40361593333)) ;
#41377=CARTESIAN_POINT('Ctrl Pts',(-12.5126943527993,-13.7161203682864,
-325.404500298253)) ;
#41378=CARTESIAN_POINT('Ctrl Pts',(-12.7189120803986,-13.5265548491555,
-325.407999261578)) ;
#41379=CARTESIAN_POINT('Ctrl Pts',(-12.8707723011009,-13.3821385130273,
-325.410590421761)) ;
#41380=CARTESIAN_POINT('Ctrl Pts',(-13.6203377077586,-12.6447510124986,
-325.42353187591)) ;
#41381=CARTESIAN_POINT('Ctrl Pts',(-14.1796623771319,-12.0141793892542,
-325.43373397788)) ;
#41382=CARTESIAN_POINT('Ctrl Pts',(-14.7870252244975,-11.2277076553842,
-325.446247094295)) ;
#41383=CARTESIAN_POINT('Ctrl Pts',(-14.8783144395675,-11.1064527881372,
-325.448169146537)) ;
#41384=CARTESIAN_POINT('Ctrl Pts',(-15.0424183123088,-10.8828271875925,
-325.451703619779)) ;
#41385=CARTESIAN_POINT('Ctrl Pts',(-15.1157004314686,-10.7808105767237,
-325.45331218965)) ;
#41386=CARTESIAN_POINT('Ctrl Pts',(-15.2650328854429,-10.5684074850552,
-325.456654401007)) ;
#41387=CARTESIAN_POINT('Ctrl Pts',(-15.3409343614486,-10.4579251583357,
-325.458389094974)) ;
#41388=CARTESIAN_POINT('Ctrl Pts',(-15.539843769457,-10.1615664245743,-325.463032692592)) ;
#41389=CARTESIAN_POINT('Ctrl Pts',(-15.6607120034706,-9.9742807182039,-325.465957561625)) ;
#41390=CARTESIAN_POINT('Ctrl Pts',(-15.8589564007482,-9.65460991424466,
-325.470930512323)) ;
#41391=CARTESIAN_POINT('Ctrl Pts',(-15.938117947845,-9.52336006474313,-325.472966855059)) ;
#41392=CARTESIAN_POINT('Ctrl Pts',(-16.2863959273451,-8.92940731252562,
-325.482150944488)) ;
#41393=CARTESIAN_POINT('Ctrl Pts',(-16.5370516564231,-8.4561769104291,-325.489392466822)) ;
#41394=CARTESIAN_POINT('Ctrl Pts',(-16.9113094864143,-7.66910562441568,
-325.501100341607)) ;
#41395=CARTESIAN_POINT('Ctrl Pts',(-17.0474329218596,-7.36156241601446,
-325.505593215)) ;
#41396=CARTESIAN_POINT('Ctrl Pts',(-17.2125897247166,-6.9592373934995,-325.511297848511)) ;
#41397=CARTESIAN_POINT('Ctrl Pts',(-17.2493225080383,-6.8676854314611,-325.512584509882)) ;
#41398=CARTESIAN_POINT('Ctrl Pts',(-17.3095885474437,-6.71394548982351,
-325.514723399839)) ;
#41399=CARTESIAN_POINT('Ctrl Pts',(-17.3335204846647,-6.65191606726594,
-325.51558041992)) ;
#41400=CARTESIAN_POINT('Ctrl Pts',(-17.3855572453533,-6.51485366349033,
-325.517460434453)) ;
#41401=CARTESIAN_POINT('Ctrl Pts',(-17.4135105333851,-6.43976474069617,
-325.518481631983)) ;
#41402=CARTESIAN_POINT('Ctrl Pts',(-17.5012921923567,-6.19921189782354,
-325.521728438355)) ;
#41403=CARTESIAN_POINT('Ctrl Pts',(-17.5592549674642,-6.03307730220059,
-325.523933726129)) ;
#41404=CARTESIAN_POINT('Ctrl Pts',(-17.7021711792304,-5.60392871880256,
-325.529561316627)) ;
#41405=CARTESIAN_POINT('Ctrl Pts',(-17.7836289662406,-5.33979613123601,
-325.532959447996)) ;
#41406=CARTESIAN_POINT('Ctrl Pts',(-18.0567477392945,-4.37847840775305,
-325.545213854333)) ;
#41407=CARTESIAN_POINT('Ctrl Pts',(-18.2135431528933,-3.67206450362121,
-325.554030734353)) ;
#41408=CARTESIAN_POINT('Ctrl Pts',(-18.3533975978218,-2.80557189399373,
-325.565076709102)) ;
#41409=CARTESIAN_POINT('Ctrl Pts',(-18.3761401969136,-2.6525286818328,-325.567035056102)) ;
#41410=CARTESIAN_POINT('Ctrl Pts',(-18.4139599137766,-2.37413450448275,
-325.570613628627)) ;
#41411=CARTESIAN_POINT('Ctrl Pts',(-18.4296764458473,-2.24887980999691,
-325.572229619995)) ;
#41412=CARTESIAN_POINT('Ctrl Pts',(-18.4593126680716,-1.991464982837,-325.575563840464)) ;
#41413=CARTESIAN_POINT('Ctrl Pts',(-18.4730932747754,-1.85929603731072,
-325.577282878659)) ;
#41414=CARTESIAN_POINT('Ctrl Pts',(-18.5055748957073,-1.51161755220164,
-325.581823957283)) ;
#41415=CARTESIAN_POINT('Ctrl Pts',(-18.5219304598692,-1.29590957569516,
-325.584660684272)) ;
#41416=CARTESIAN_POINT('Ctrl Pts',(-18.5505246958422,-0.80517143329906,
-325.591154405314)) ;
#41417=CARTESIAN_POINT('Ctrl Pts',(-18.560423163618,-0.530055751092466,
-325.594823690902)) ;
#41418=CARTESIAN_POINT('Ctrl Pts',(-18.5698672744087,0.157962337761502,
-325.604046528953)) ;
#41419=CARTESIAN_POINT('Ctrl Pts',(-18.5617640737465,0.570821060204457,
-325.609624394886)) ;
#41420=CARTESIAN_POINT('Ctrl Pts',(-18.5214388544416,1.33132601610996,-325.619859256568)) ;
#41421=CARTESIAN_POINT('Ctrl Pts',(-18.493163371486,1.67899838666721,-325.62452207147)) ;
#41422=CARTESIAN_POINT('Ctrl Pts',(-18.4443478998066,2.12373811586512,-325.630390765951)) ;
#41423=CARTESIAN_POINT('Ctrl Pts',(-18.4328019756894,2.22172104464914,-325.631677623332)) ;
#41424=CARTESIAN_POINT('Ctrl Pts',(-18.4121687533959,2.38557367432853,-325.63381673208)) ;
#41425=CARTESIAN_POINT('Ctrl Pts',(-18.4035076200842,2.45149490573154,-325.634673777305)) ;
#41426=CARTESIAN_POINT('Ctrl Pts',(-18.3836298094674,2.5967427108578,-325.636553714106)) ;
#41427=CARTESIAN_POINT('Ctrl Pts',(-18.3722534244905,2.67604592783782,-325.637574810206)) ;
#41428=CARTESIAN_POINT('Ctrl Pts',(-18.3342604818384,2.92922020051268,-325.640820868344)) ;
#41429=CARTESIAN_POINT('Ctrl Pts',(-18.3056861670504,3.10278786620846,-325.643025522238)) ;
#41430=CARTESIAN_POINT('Ctrl Pts',(-18.2259071860437,3.54783274017972,-325.648650893665)) ;
#41431=CARTESIAN_POINT('Ctrl Pts',(-18.1711019587516,3.81862068013037,-325.652047462569)) ;
#41432=CARTESIAN_POINT('Ctrl Pts',(-17.9516045826797,4.79099721518068,-325.664271022509)) ;
#41433=CARTESIAN_POINT('Ctrl Pts',(-17.7521453722084,5.48407657751811,-325.67305864834)) ;
#41434=CARTESIAN_POINT('Ctrl Pts',(-17.461219862357,6.31066888090055,-325.684084726484)) ;
#41435=CARTESIAN_POINT('Ctrl Pts',(-17.4076840449076,6.45687826317527,-325.686055130276)) ;
#41436=CARTESIAN_POINT('Ctrl Pts',(-17.3073481493258,6.72057948834217,-325.689648438801)) ;
#41437=CARTESIAN_POINT('Ctrl Pts',(-17.2611745620122,6.83829959181913,-325.691266981231)) ;
#41438=CARTESIAN_POINT('Ctrl Pts',(-17.1641515887554,7.07841532204329,-325.694599045026)) ;
#41439=CARTESIAN_POINT('Ctrl Pts',(-17.1131869204801,7.20075666827623,-325.696313298285)) ;
#41440=CARTESIAN_POINT('Ctrl Pts',(-16.9763933074534,7.51947447615887,-325.700823085113)) ;
#41441=CARTESIAN_POINT('Ctrl Pts',(-16.888466523612,7.71492866839115,-325.703632922743)) ;
#41442=CARTESIAN_POINT('Ctrl Pts',(-16.6815209950024,8.1544508698707,-325.710048888708)) ;
#41443=CARTESIAN_POINT('Ctrl Pts',(-16.5604920599986,8.39751832532395,-325.71366684079)) ;
#41444=CARTESIAN_POINT('Ctrl Pts',(-16.269939377822,8.95031764018592,-325.722035117324)) ;
#41445=CARTESIAN_POINT('Ctrl Pts',(-16.0968238486783,9.25804379237521,-325.726798254232)) ;
#41446=CARTESIAN_POINT('Ctrl Pts',(-15.7595083869069,9.81955282186625,-325.735615246477)) ;
#41447=CARTESIAN_POINT('Ctrl Pts',(-15.5976807776198,10.074625401159,-325.739670530999)) ;
#41448=CARTESIAN_POINT('Ctrl Pts',(-15.3382866896946,10.4622406009242,-325.745857163054)) ;
#41449=CARTESIAN_POINT('Ctrl Pts',(-15.2450603609048,10.5976248148503,-325.748022524744)) ;
#41450=CARTESIAN_POINT('Ctrl Pts',(-15.1048265182354,10.7955933523002,-325.751185508893)) ;
#41451=CARTESIAN_POINT('Ctrl Pts',(-15.0592014357155,10.8591469331221,-325.752200384815)) ;
#41452=CARTESIAN_POINT('Ctrl Pts',(-14.9737728473272,10.9765710545287,-325.754073031483)) ;
#41453=CARTESIAN_POINT('Ctrl Pts',(-14.9340769898321,11.0305181134235,-325.754932221792)) ;
#41454=CARTESIAN_POINT('Ctrl Pts',(-14.8329871159042,11.1663542586281,-325.757093821876)) ;
#41455=CARTESIAN_POINT('Ctrl Pts',(-14.7712062298641,11.2479527368217,-325.758390778703)) ;
#41456=CARTESIAN_POINT('Ctrl Pts',(-14.6317768379482,11.4289771895086,-325.761269214318)) ;
#41457=CARTESIAN_POINT('Ctrl Pts',(-14.5537832529012,11.5281310768763,-325.762846647535)) ;
#41458=CARTESIAN_POINT('Ctrl Pts',(-14.2986261011356,11.8457976594216,-325.76791479526)) ;
#41459=CARTESIAN_POINT('Ctrl Pts',(-14.117505119151,12.0610812194131,-325.771372333612)) ;
#41460=CARTESIAN_POINT('Ctrl Pts',(-13.4589551961165,12.8086777878847,-325.783587056471)) ;
#41461=CARTESIAN_POINT('Ctrl Pts',(-12.9557499349095,13.3174413803227,-325.792309977594)) ;
#41462=CARTESIAN_POINT('Ctrl Pts',(-12.3094244624844,13.899515673893,-325.803256205789)) ;
#41463=CARTESIAN_POINT('Ctrl Pts',(-12.1930951745481,14.0016747762227,-325.805215728218)) ;
#41464=CARTESIAN_POINT('Ctrl Pts',(-11.9796012462123,14.1844842552587,-325.808795735595)) ;
#41465=CARTESIAN_POINT('Ctrl Pts',(-11.8828654969847,14.2656211618479,-325.810411973914)) ;
#41466=CARTESIAN_POINT('Ctrl Pts',(-11.6826602031754,14.4300934928543,-325.813745973816)) ;
#41467=CARTESIAN_POINT('Ctrl Pts',(-11.5791085836803,14.5133177454427,-325.815464536894)) ;
#41468=CARTESIAN_POINT('Ctrl Pts',(-11.3047788072906,14.7289911341839,-325.8200025081)) ;
#41469=CARTESIAN_POINT('Ctrl Pts',(-11.1325659111102,14.8595820833543,-325.822836564644)) ;
#41470=CARTESIAN_POINT('Ctrl Pts',(-10.7362149370299,15.1493811813869,-325.829322545224)) ;
#41471=CARTESIAN_POINT('Ctrl Pts',(-10.5107415592983,15.3066773929509,-325.832986713787)) ;
#41472=CARTESIAN_POINT('Ctrl Pts',(-9.93812633263931,15.687528927325,-325.84220420679)) ;
#41473=CARTESIAN_POINT('Ctrl Pts',(-9.58686388451546,15.9046206879937,-325.847781960742)) ;
#41474=CARTESIAN_POINT('Ctrl Pts',(-8.92549894526548,16.2834896103077,-325.858025443599)) ;
#41475=CARTESIAN_POINT('Ctrl Pts',(-8.61749731967721,16.4485654731905,-325.862696858116)) ;
#41476=CARTESIAN_POINT('Ctrl Pts',(-8.21673224209315,16.649010649223,-325.868574635706)) ;
#41477=CARTESIAN_POINT('Ctrl Pts',(-8.12809221670241,16.6924642067723,-325.869862255838)) ;
#41478=CARTESIAN_POINT('Ctrl Pts',(-7.97917238073115,16.7640009843189,-325.872002216173)) ;
#41479=CARTESIAN_POINT('Ctrl Pts',(-7.91908071659601,16.7924709773137,-325.872859359421)) ;
#41480=CARTESIAN_POINT('Ctrl Pts',(-7.78628312513224,16.8545159433535,-325.874738994611)) ;
#41481=CARTESIAN_POINT('Ctrl Pts',(-7.71351042958043,16.8879445009117,-325.875759696696)) ;
#41482=CARTESIAN_POINT('Ctrl Pts',(-7.48039670501084,16.9932054979515,-325.87900284983)) ;
#41483=CARTESIAN_POINT('Ctrl Pts',(-7.31925117855927,17.0632332907562,-325.881205042867)) ;
#41484=CARTESIAN_POINT('Ctrl Pts',(-6.90270747874475,17.2372608558067,-325.886821804599)) ;
#41485=CARTESIAN_POINT('Ctrl Pts',(-6.64594224773445,17.3378771588116,-325.89021231274)) ;
#41486=CARTESIAN_POINT('Ctrl Pts',(-5.70570197653486,17.6823637375105,-325.902491483921)) ;
#41487=CARTESIAN_POINT('Ctrl Pts',(-5.01032331176097,17.8918328446128,-325.911339965105)) ;
#41488=CARTESIAN_POINT('Ctrl Pts',(-4.15456818780093,18.0957954099149,-325.922412700275)) ;
#41489=CARTESIAN_POINT('Ctrl Pts',(-4.00422148437912,18.1296568792157,-325.924363519327)) ;
#41490=CARTESIAN_POINT('Ctrl Pts',(-3.7301157846588,18.1878156227027,-325.927932911874)) ;
#41491=CARTESIAN_POINT('Ctrl Pts',(-3.60649741989119,18.2127311845243,-325.929547330984)) ;
#41492=CARTESIAN_POINT('Ctrl Pts',(-3.35188800928146,18.2613543962448,-325.932883018432)) ;
#41493=CARTESIAN_POINT('Ctrl Pts',(-3.22087646518749,18.2849165255167,-325.934605144949)) ;
#41494=CARTESIAN_POINT('Ctrl Pts',(-2.87505134035548,18.3432802830131,-325.939166425339)) ;
#41495=CARTESIAN_POINT('Ctrl Pts',(-2.65985995226683,18.3757175784956,-325.942020514635)) ;
#41496=CARTESIAN_POINT('Ctrl Pts',(-1.60793750064242,18.515415673222,-325.956040791013)) ;
#41497=CARTESIAN_POINT('Ctrl Pts',(-0.765136275296041,18.5693466268616,
-325.967534556341)) ;
#41498=CARTESIAN_POINT('Ctrl Pts',(0.295082724962301,18.5648694388514,-325.981678250055)) ;
#41499=CARTESIAN_POINT('Ctrl Pts',(0.511731969816002,18.5601611468255,-325.984548649932)) ;
#41500=CARTESIAN_POINT('Ctrl Pts',(0.814739961412343,18.5482665054331,-325.988514389729)) ;
#41501=CARTESIAN_POINT('Ctrl Pts',(0.90120589264641,18.5442664866913,-325.989640448845)) ;
#41502=CARTESIAN_POINT('Ctrl Pts',(1.05329278231821,18.5361645476409,-325.991609363401)) ;
#41503=CARTESIAN_POINT('Ctrl Pts',(1.11892560309099,18.5323184553841,-325.992455060869)) ;
#41504=CARTESIAN_POINT('Ctrl Pts',(1.27232474320629,18.5225113674957,-325.994422431458)) ;
#41505=CARTESIAN_POINT('Ctrl Pts',(1.36007170207535,18.5162750737467,-325.995540980881)) ;
#41506=CARTESIAN_POINT('Ctrl Pts',(1.68044435934408,18.4912161368036,-325.999604860392)) ;
#41507=CARTESIAN_POINT('Ctrl Pts',(1.91275426063009,18.4686312162562,-326.002513243689)) ;
#41508=CARTESIAN_POINT('Ctrl Pts',(2.59861765013032,18.3888723596994,-326.011053437748)) ;
#41509=CARTESIAN_POINT('Ctrl Pts',(3.05055412035333,18.3193220662031,-326.016623781821)) ;
#41510=CARTESIAN_POINT('Ctrl Pts',(3.96392214500717,18.1440207739935,-326.028037463384)) ;
#41511=CARTESIAN_POINT('Ctrl Pts',(4.42480514575666,18.0371634867906,-326.033880074358)) ;
#41512=CARTESIAN_POINT('Ctrl Pts',(5.02725505875044,17.8730006537474,-326.041743520987)) ;
#41513=CARTESIAN_POINT('Ctrl Pts',(5.17291381020615,17.8313882920061,-326.043661981945)) ;
#41514=CARTESIAN_POINT('Ctrl Pts',(5.43833184222175,17.7520367247879,-326.047192114981)) ;
#41515=CARTESIAN_POINT('Ctrl Pts',(5.55824886622087,17.7148562114734,-326.048799973626)) ;
#41516=CARTESIAN_POINT('Ctrl Pts',(5.80551322754323,17.635433503348,-326.052143108107)) ;
#41517=CARTESIAN_POINT('Ctrl Pts',(5.93279840900113,17.5930213908802,-326.053879461481)) ;
#41518=CARTESIAN_POINT('Ctrl Pts',(6.27095080348051,17.4762600228415,-326.058533947658)) ;
#41519=CARTESIAN_POINT('Ctrl Pts',(6.48095324191959,17.3994750828928,-326.061468184024)) ;
#41520=CARTESIAN_POINT('Ctrl Pts',(6.83316032424528,17.2634333509648,-326.066460258774)) ;
#41521=CARTESIAN_POINT('Ctrl Pts',(6.97610744357938,17.2061656373489,-326.068506329929)) ;
#41522=CARTESIAN_POINT('Ctrl Pts',(7.61734833547387,16.9399658512253,-326.077768270067)) ;
#41523=CARTESIAN_POINT('Ctrl Pts',(8.10708972261343,16.7111200423497,-326.085079526092)) ;
#41524=CARTESIAN_POINT('Ctrl Pts',(8.87959769809157,16.3081814868363,-326.096781403116)) ;
#41525=CARTESIAN_POINT('Ctrl Pts',(9.16890049363321,16.1473001833487,-326.101201819958)) ;
#41526=CARTESIAN_POINT('Ctrl Pts',(9.53794795938075,15.9289553766288,-326.106825278383)) ;
#41527=CARTESIAN_POINT('Ctrl Pts',(9.62175274208957,15.8784742616224,-326.108101129311)) ;
#41528=CARTESIAN_POINT('Ctrl Pts',(9.76175127797173,15.7926286273999,-326.110227982068)) ;
#41529=CARTESIAN_POINT('Ctrl Pts',(9.81816133616834,15.7576208543033,-326.111083645231)) ;
#41530=CARTESIAN_POINT('Ctrl Pts',(9.94262275716697,15.6794529767418,-326.112968092511)) ;
#41531=CARTESIAN_POINT('Ctrl Pts',(10.0105832149865,15.6361509541529,-326.113994998619)) ;
#41532=CARTESIAN_POINT('Ctrl Pts',(10.2284840755446,15.495309239534,-326.117284190863)) ;
#41533=CARTESIAN_POINT('Ctrl Pts',(10.3772976687841,15.3960445636133,-326.119525417212)) ;
#41534=CARTESIAN_POINT('Ctrl Pts',(10.7584463457597,15.1337659764524,-326.125279728585)) ;
#41535=CARTESIAN_POINT('Ctrl Pts',(10.988519753648,14.9675473755151,-326.128767328313)) ;
#41536=CARTESIAN_POINT('Ctrl Pts',(11.7795489237345,14.3679882462425,-326.14093556031)) ;
#41537=CARTESIAN_POINT('Ctrl Pts',(12.3194259018141,13.9078612343114,-326.14958450643)) ;
#41538=CARTESIAN_POINT('Ctrl Pts',(12.9441869791235,13.3104004566808,-326.160461660875)) ;
#41539=CARTESIAN_POINT('Ctrl Pts',(13.0553449789335,13.2013902395014,-326.162431908843)) ;
#41540=CARTESIAN_POINT('Ctrl Pts',(13.2542764973676,13.0013323334899,-326.166025026664)) ;
#41541=CARTESIAN_POINT('Ctrl Pts',(13.3425159324755,12.9107612654248,-326.167643535874)) ;
#41542=CARTESIAN_POINT('Ctrl Pts',(13.5108770362846,12.7343818556155,-326.170780775693)) ;
#41543=CARTESIAN_POINT('Ctrl Pts',(13.5911236568056,12.6487010098442,-326.172298275558)) ;
#41544=CARTESIAN_POINT('Ctrl Pts',(13.6754495458126,12.5569355938576,-326.173916846399)) ;
#41545=CARTESIAN_POINT('Ctrl Pts',(13.6803437417049,12.5516033596181,-326.174010873231)) ;
#41546=CARTESIAN_POINT('Ctrl Pts',(13.6901452324564,12.5409120767852,-326.174199351987)) ;
#41547=CARTESIAN_POINT('Ctrl Pts',(13.6950525009698,12.53555300731,-326.174293804089)) ;
#41548=CARTESIAN_POINT('Ctrl Pts',(13.7049530641626,12.5247281694731,-326.174484540396)) ;
#41549=CARTESIAN_POINT('Ctrl Pts',(13.7099462383262,12.5192622926547,-326.174580825599)) ;
#41550=CARTESIAN_POINT('Ctrl Pts',(13.7200913125024,12.5081434384684,-326.174776641318)) ;
#41551=CARTESIAN_POINT('Ctrl Pts',(13.7252429912914,12.5024902611718,-326.174876173678)) ;
#41552=CARTESIAN_POINT('Ctrl Pts',(13.7357813666331,12.4909116471868,-326.175079977581)) ;
#41553=CARTESIAN_POINT('Ctrl Pts',(13.7411677257626,12.4849859055675,-326.175184251938)) ;
#41554=CARTESIAN_POINT('Ctrl Pts',(13.7522590624025,12.4727680256151,-326.175399188141)) ;
#41555=CARTESIAN_POINT('Ctrl Pts',(13.7579635594468,12.466475453678,-326.175509853983)) ;
#41556=CARTESIAN_POINT('Ctrl Pts',(13.7697860319488,12.4534162081856,-326.175739455722)) ;
#41557=CARTESIAN_POINT('Ctrl Pts',(13.7759033422313,12.4466489355743,-326.17585839713)) ;
#41558=CARTESIAN_POINT('Ctrl Pts',(13.7886620368946,12.4325137051817,-326.176106758803)) ;
#41559=CARTESIAN_POINT('Ctrl Pts',(13.795302509049,12.4251449279689,-326.176236186588)) ;
#41560=CARTESIAN_POINT('Ctrl Pts',(13.8092391290691,12.4096548408105,-326.176508166153)) ;
#41561=CARTESIAN_POINT('Ctrl Pts',(13.8165340253887,12.4015324100333,-326.176650728187)) ;
#41562=CARTESIAN_POINT('Ctrl Pts',(13.8319384075838,12.384350089389,-326.176952191856)) ;
#41563=CARTESIAN_POINT('Ctrl Pts',(13.8400461661024,12.3752886579605,-326.17711110754)) ;
#41564=CARTESIAN_POINT('Ctrl Pts',(13.8572700143265,12.3560007622214,-326.177449227903)) ;
#41565=CARTESIAN_POINT('Ctrl Pts',(13.8663836983411,12.3457721595809,-326.17762845198)) ;
#41566=CARTESIAN_POINT('Ctrl Pts',(13.8858566889508,12.3238681851777,-326.178012067424)) ;
#41567=CARTESIAN_POINT('Ctrl Pts',(13.8962126102776,12.312189818289,-326.178216485804)) ;
#41568=CARTESIAN_POINT('Ctrl Pts',(13.9184604434533,12.2870371229628,-326.178656519844)) ;
#41569=CARTESIAN_POINT('Ctrl Pts',(13.9303475428202,12.2735585594862,-326.178892173418)) ;
#41570=CARTESIAN_POINT('Ctrl Pts',(14.0709232952275,12.1136949919324,-326.181685407731)) ;
#41571=CARTESIAN_POINT('Ctrl Pts',(14.1973184996401,11.9653096903167,-326.184260854254)) ;
#41572=CARTESIAN_POINT('Ctrl Pts',(14.5752261720363,11.5072337821234,-326.192152766329)) ;
#41573=CARTESIAN_POINT('Ctrl Pts',(14.8191138747671,11.1914034092077,-326.197516448595)) ;
#41574=CARTESIAN_POINT('Ctrl Pts',(15.3527935327658,10.4522321093359,-326.209796607689)) ;
#41575=CARTESIAN_POINT('Ctrl Pts',(15.6355986834255,10.0242446196427,-326.216716594901)) ;
#41576=CARTESIAN_POINT('Ctrl Pts',(15.9584584533486,9.48866599888211,-326.224944745217)) ;
#41577=CARTESIAN_POINT('Ctrl Pts',(16.0157134685856,9.3917038281846,-326.226417450865)) ;
#41578=CARTESIAN_POINT('Ctrl Pts',(16.1030809785081,9.24062317281765,-326.228682473268)) ;
#41579=CARTESIAN_POINT('Ctrl Pts',(16.1338107161249,9.18686483055236,-326.229482666142)) ;
#41580=CARTESIAN_POINT('Ctrl Pts',(16.1872010205725,9.09237017134847,-326.230878448429)) ;
#41581=CARTESIAN_POINT('Ctrl Pts',(16.2099781651642,9.05170039844211,-326.231475721017)) ;
#41582=CARTESIAN_POINT('Ctrl Pts',(16.2791371337427,8.92711524405567,-326.233295431394)) ;
#41583=CARTESIAN_POINT('Ctrl Pts',(16.3250223182117,8.84292591551947,-326.2345113965)) ;
#41584=CARTESIAN_POINT('Ctrl Pts',(16.4264597894673,8.65332964535442,-326.237222982068)) ;
#41585=CARTESIAN_POINT('Ctrl Pts',(16.4816537271513,8.54773570252579,-326.238714808704)) ;
#41586=CARTESIAN_POINT('Ctrl Pts',(16.6516040885121,8.21482915009749,-326.24337048646)) ;
#41587=CARTESIAN_POINT('Ctrl Pts',(16.7627030274991,7.9856824519716,-326.246506423549)) ;
#41588=CARTESIAN_POINT('Ctrl Pts',(17.1742306399231,7.09042940512117,-326.258599155768)) ;
#41589=CARTESIAN_POINT('Ctrl Pts',(17.4399499969237,6.40909758995289,-326.267493369391)) ;
#41590=CARTESIAN_POINT('Ctrl Pts',(17.721280986405,5.53934572549684,-326.278974606326)) ;
#41591=CARTESIAN_POINT('Ctrl Pts',(17.7751477760869,5.3639791436072,-326.281294064475)) ;
#41592=CARTESIAN_POINT('Ctrl Pts',(17.8616219345275,5.06683764801474,-326.28523637947)) ;
#41593=CARTESIAN_POINT('Ctrl Pts',(17.8956040020969,4.94547664341804,-326.28684990559)) ;
#41594=CARTESIAN_POINT('Ctrl Pts',(17.9585426420398,4.71155510929684,-326.28996734179)) ;
#41595=CARTESIAN_POINT('Ctrl Pts',(17.9876831053392,4.59905010126032,-326.291469934847)) ;
#41596=CARTESIAN_POINT('Ctrl Pts',(18.0329229160626,4.41737842835324,-326.293901735486)) ;
#41597=CARTESIAN_POINT('Ctrl Pts',(18.0496851019182,4.34838001882996,-326.294826577833)) ;
#41598=CARTESIAN_POINT('Ctrl Pts',(18.0821235892296,4.21143305954911,-326.296664634176)) ;
#41599=CARTESIAN_POINT('Ctrl Pts',(18.0978137127823,4.14348895498113,-326.297577744657)) ;
#41600=CARTESIAN_POINT('Ctrl Pts',(18.1497936019229,3.91246756272262,-326.300686340654)) ;
#41601=CARTESIAN_POINT('Ctrl Pts',(18.1842648154924,3.74898962828245,-326.302892678332)) ;
#41602=CARTESIAN_POINT('Ctrl Pts',(18.3068415174889,3.12615040494634,-326.311318420687)) ;
#41603=CARTESIAN_POINT('Ctrl Pts',(18.3797837939384,2.66398362450672,-326.317615691143)) ;
#41604=CARTESIAN_POINT('Ctrl Pts',(18.4898188667436,1.74174464653576,-326.330126728078)) ;
#41605=CARTESIAN_POINT('Ctrl Pts',(18.5273692870419,1.28205479994996,-326.336335596783)) ;
#41606=CARTESIAN_POINT('Ctrl Pts',(18.5528417082755,0.706901559720696,-326.343913581851)) ;
#41607=CARTESIAN_POINT('Ctrl Pts',(18.5568534445105,0.592313741152011,-326.345413679559)) ;
#41608=CARTESIAN_POINT('Ctrl Pts',(18.561405495324,0.415454051365691,-326.3477103568)) ;
#41609=CARTESIAN_POINT('Ctrl Pts',(18.5626943817849,0.353204375563594,-326.34851515907)) ;
#41610=CARTESIAN_POINT('Ctrl Pts',(18.564615155673,0.230651730128177,-326.35009177426)) ;
#41611=CARTESIAN_POINT('Ctrl Pts',(18.5652664147311,0.170349815297605,-326.350863819058)) ;
#41612=CARTESIAN_POINT('Ctrl Pts',(18.566054124091,0.0374567727573222,-326.352558003735)) ;
#41613=CARTESIAN_POINT('Ctrl Pts',(18.5660586650683,-0.0351341711078605,
-326.353478666443)) ;
#41614=CARTESIAN_POINT('Ctrl Pts',(18.564125770088,-0.368260060632838,-326.357685219006)) ;
#41615=CARTESIAN_POINT('Ctrl Pts',(18.5571299447306,-0.628736687137649,
-326.360922991914)) ;
#41616=CARTESIAN_POINT('Ctrl Pts',(18.5446545937382,-0.888979978089834,
-326.364137692133)) ;
#41617=CARTESIAN_POINT('Origin',(0.,0.,-315.477129595899)) ;
#41618=CARTESIAN_POINT('',(18.5446545937613,-0.888979977608419,-328.159979993775)) ;
#41619=CARTESIAN_POINT('',(18.5446545920456,-0.888980013399066,-327.863308833241)) ;
#41620=CARTESIAN_POINT('',(18.544654593745,-0.888979977948782,-315.477129595899)) ;
#41621=CARTESIAN_POINT('Ctrl Pts',(18.5446545937776,-0.888979977268111,
-328.159979993775)) ;
#41622=CARTESIAN_POINT('Ctrl Pts',(18.5514236661009,-0.74777307568927,-328.158107862953)) ;
#41623=CARTESIAN_POINT('Ctrl Pts',(18.5565798363497,-0.606490695771115,
-328.156227426047)) ;
#41624=CARTESIAN_POINT('Ctrl Pts',(18.5745103188236,0.108944031999928,-328.146674608869)) ;
#41625=CARTESIAN_POINT('Ctrl Pts',(18.5622535103131,0.683406818439957,-328.138893899993)) ;
#41626=CARTESIAN_POINT('Ctrl Pts',(18.50367512622,1.54705962925855,-328.127288829815)) ;
#41627=CARTESIAN_POINT('Ctrl Pts',(18.4771190513928,1.8372421840355,-328.123407637824)) ;
#41628=CARTESIAN_POINT('Ctrl Pts',(18.4339502100328,2.21162630830476,-328.118469203763)) ;
#41629=CARTESIAN_POINT('Ctrl Pts',(18.4235685762218,2.29650434744372,-328.117354249426)) ;
#41630=CARTESIAN_POINT('Ctrl Pts',(18.4040025166416,2.44779182979563,-328.115377077128)) ;
#41631=CARTESIAN_POINT('Ctrl Pts',(18.3950440658625,2.51422897316266,-328.114512357129)) ;
#41632=CARTESIAN_POINT('Ctrl Pts',(18.3748785500496,2.6578991651199,-328.112650837349)) ;
#41633=CARTESIAN_POINT('Ctrl Pts',(18.3635439724568,2.73511288519702,-328.111655459563)) ;
#41634=CARTESIAN_POINT('Ctrl Pts',(18.3269994879263,2.97358868234219,-328.108594002804)) ;
#41635=CARTESIAN_POINT('Ctrl Pts',(18.3001495906628,3.13459167957558,-328.106545167952)) ;
#41636=CARTESIAN_POINT('Ctrl Pts',(18.1816729970637,3.79151512853311,-328.09822646062)) ;
#41637=CARTESIAN_POINT('Ctrl Pts',(18.0719816867557,4.2839584596961,-328.092080765508)) ;
#41638=CARTESIAN_POINT('Ctrl Pts',(17.8184540203618,5.23733927215678,-328.079987070465)) ;
#41639=CARTESIAN_POINT('Ctrl Pts',(17.6764208224042,5.6983481810062,-328.074046866786)) ;
#41640=CARTESIAN_POINT('Ctrl Pts',(17.4551371864372,6.32827613392892,-328.065663781168)) ;
#41641=CARTESIAN_POINT('Ctrl Pts',(17.3910537002965,6.50231836059139,-328.063319523851)) ;
#41642=CARTESIAN_POINT('Ctrl Pts',(17.2789487160083,6.79326078428456,-328.059348359552)) ;
#41643=CARTESIAN_POINT('Ctrl Pts',(17.2323217200021,6.9106836781064,-328.057731124369)) ;
#41644=CARTESIAN_POINT('Ctrl Pts',(17.1342673365167,7.15045407075271,-328.054397987917)) ;
#41645=CARTESIAN_POINT('Ctrl Pts',(17.0827192780376,7.27274450139638,-328.052681315549)) ;
#41646=CARTESIAN_POINT('Ctrl Pts',(16.9441070096523,7.59197598657199,-328.048155710286)) ;
#41647=CARTESIAN_POINT('Ctrl Pts',(16.8549201960559,7.78797320661865,-328.045332280427)) ;
#41648=CARTESIAN_POINT('Ctrl Pts',(16.6447984289805,8.22921202532305,-328.038877061763)) ;
#41649=CARTESIAN_POINT('Ctrl Pts',(16.5218144660265,8.47342266383326,-328.035233214282)) ;
#41650=CARTESIAN_POINT('Ctrl Pts',(16.228930238702,9.02436785952236,-328.026871083059)) ;
#41651=CARTESIAN_POINT('Ctrl Pts',(16.0556437906125,9.32918507153438,-328.022140903281)) ;
#41652=CARTESIAN_POINT('Ctrl Pts',(15.8248668895879,9.70963443683454,-328.016151596367)) ;
#41653=CARTESIAN_POINT('Ctrl Pts',(15.775286849698,9.78998150088528,-328.014881854905)) ;
#41654=CARTESIAN_POINT('Ctrl Pts',(15.553944201941,10.1426312612573,-328.009291616065)) ;
#41655=CARTESIAN_POINT('Ctrl Pts',(15.3757280793041,10.4108182152703,-328.004993680335)) ;
#41656=CARTESIAN_POINT('Ctrl Pts',(15.1343471417449,10.7543302332678,-327.999487668842)) ;
#41657=CARTESIAN_POINT('Ctrl Pts',(15.0774330586572,10.8339787047613,-327.998211034885)) ;
#41658=CARTESIAN_POINT('Ctrl Pts',(14.9808635069289,10.9668881851245,-327.996083312137)) ;
#41659=CARTESIAN_POINT('Ctrl Pts',(14.9415474705939,11.0203932369666,-327.995227552588)) ;
#41660=CARTESIAN_POINT('Ctrl Pts',(14.8539018102926,11.1383386770644,-327.99334343574)) ;
#41661=CARTESIAN_POINT('Ctrl Pts',(14.8054382242945,11.2026776480181,-327.99231695049)) ;
#41662=CARTESIAN_POINT('Ctrl Pts',(14.6481407455602,11.4086979942674,-327.989030902338)) ;
#41663=CARTESIAN_POINT('Ctrl Pts',(14.537679882563,11.5491246878927,-327.986792343972)) ;
#41664=CARTESIAN_POINT('Ctrl Pts',(14.2468988310866,11.9080056549176,-327.981047502236)) ;
#41665=CARTESIAN_POINT('Ctrl Pts',(14.0635753022643,12.1239669706998,-327.977566604872)) ;
#41666=CARTESIAN_POINT('Ctrl Pts',(13.403508753563,12.8664228830841,-327.965387487122)) ;
#41667=CARTESIAN_POINT('Ctrl Pts',(12.9015675410471,13.3696835895997,-327.956721520582)) ;
#41668=CARTESIAN_POINT('Ctrl Pts',(12.2561133616275,13.9465535668615,-327.945828610059)) ;
#41669=CARTESIAN_POINT('Ctrl Pts',(12.1388948400138,14.0486975587308,-327.943860965151)) ;
#41670=CARTESIAN_POINT('Ctrl Pts',(11.9240769158918,14.2311934087864,-327.940271031904)) ;
#41671=CARTESIAN_POINT('Ctrl Pts',(11.8269133605756,14.312043754912,-327.938653076501)) ;
#41672=CARTESIAN_POINT('Ctrl Pts',(11.6261370864121,14.4756699593801,-327.935320539035)) ;
#41673=CARTESIAN_POINT('Ctrl Pts',(11.5224478176042,14.5583405837799,-327.933605207558)) ;
#41674=CARTESIAN_POINT('Ctrl Pts',(11.2485385094423,14.7719667413822,-327.929088370955)) ;
#41675=CARTESIAN_POINT('Ctrl Pts',(11.0769165555979,14.901091885372,-327.926272475912)) ;
#41676=CARTESIAN_POINT('Ctrl Pts',(10.6826588486031,15.1871482129532,-327.919839029859)) ;
#41677=CARTESIAN_POINT('Ctrl Pts',(10.4587320854737,15.3422160614638,-327.916209550792)) ;
#41678=CARTESIAN_POINT('Ctrl Pts',(9.93780994252413,15.6862451419727,-327.907843862582)) ;
#41679=CARTESIAN_POINT('Ctrl Pts',(9.63868924464666,15.8717995960812,-327.903095249167)) ;
#41680=CARTESIAN_POINT('Ctrl Pts',(9.25188533949489,16.0967775020261,-327.897072193654)) ;
#41681=CARTESIAN_POINT('Ctrl Pts',(9.16892475941206,16.1441768774129,-327.895787195699)) ;
#41682=CARTESIAN_POINT('Ctrl Pts',(8.8047346771958,16.3485434805822,-327.890180201155)) ;
#41683=CARTESIAN_POINT('Ctrl Pts',(8.51981320106167,16.4988184557095,-327.88588078533)) ;
#41684=CARTESIAN_POINT('Ctrl Pts',(8.1435958069966,16.6848998438459,-327.880376650738)) ;
#41685=CARTESIAN_POINT('Ctrl Pts',(8.05572434380301,16.7275025273885,-327.879103198085)) ;
#41686=CARTESIAN_POINT('Ctrl Pts',(7.90757405298156,16.7978920354829,-327.876979007491)) ;
#41687=CARTESIAN_POINT('Ctrl Pts',(7.84747501658886,16.8260524228929,-327.876123637079)) ;
#41688=CARTESIAN_POINT('Ctrl Pts',(7.71397949505441,16.887733126861,-327.874238166229)) ;
#41689=CARTESIAN_POINT('Ctrl Pts',(7.64051302451444,16.9210983851681,-327.873209962154)) ;
#41690=CARTESIAN_POINT('Ctrl Pts',(7.40287570612491,17.0271596825096,-327.869911056702)) ;
#41691=CARTESIAN_POINT('Ctrl Pts',(7.23786693920372,17.0979536186422,-327.867661586251)) ;
#41692=CARTESIAN_POINT('Ctrl Pts',(6.80785986210398,17.2750995957218,-327.861877950311)) ;
#41693=CARTESIAN_POINT('Ctrl Pts',(6.54138851891774,17.3777518282403,-327.858369578704)) ;
#41694=CARTESIAN_POINT('Ctrl Pts',(5.60989529042941,17.712126532224,-327.846237293141)) ;
#41695=CARTESIAN_POINT('Ctrl Pts',(4.93413579302475,17.91213708527,-327.837643330999)) ;
#41696=CARTESIAN_POINT('Ctrl Pts',(4.09639306218631,18.1090730846715,-327.826816509335)) ;
#41697=CARTESIAN_POINT('Ctrl Pts',(3.94368560732016,18.1429409920813,-327.824837290935)) ;
#41698=CARTESIAN_POINT('Ctrl Pts',(3.66662818428516,18.2007243418371,-327.821233184179)) ;
#41699=CARTESIAN_POINT('Ctrl Pts',(3.54242670584466,18.2253049848144,-327.819612752121)) ;
#41700=CARTESIAN_POINT('Ctrl Pts',(3.28796509167005,18.2729659013395,-327.816282120425)) ;
#41701=CARTESIAN_POINT('Ctrl Pts',(3.15769011973695,18.2959282443259,-327.814571244279)) ;
#41702=CARTESIAN_POINT('Ctrl Pts',(2.81714043964998,18.3522080712358,-327.810083543326)) ;
#41703=CARTESIAN_POINT('Ctrl Pts',(2.60651869309998,18.3833044201638,-327.807292682273)) ;
#41704=CARTESIAN_POINT('Ctrl Pts',(2.12879192037522,18.4454610256195,-327.800931345266)) ;
#41705=CARTESIAN_POINT('Ctrl Pts',(1.86145305566809,18.4743546468227,-327.797349368403)) ;
#41706=CARTESIAN_POINT('Ctrl Pts',(1.23914259885147,18.5279676283469,-327.788981354838)) ;
#41707=CARTESIAN_POINT('Ctrl Pts',(0.883899345031587,18.5483093678236,-327.7841813309)) ;
#41708=CARTESIAN_POINT('Ctrl Pts',(0.269479611282192,18.5657996939309,-327.775907362587)) ;
#41709=CARTESIAN_POINT('Ctrl Pts',(0.0105411719020318,18.5677523316723,
-327.772429441677)) ;
#41710=CARTESIAN_POINT('Ctrl Pts',(-0.440783130971584,18.5617145082437,
-327.766421026055)) ;
#41711=CARTESIAN_POINT('Ctrl Pts',(-0.633161600439865,18.556148357681,-327.763877001331)) ;
#41712=CARTESIAN_POINT('Ctrl Pts',(-0.909954411501939,18.5438303156014,
-327.76025674032)) ;
#41713=CARTESIAN_POINT('Ctrl Pts',(-0.994463280493784,18.5394903548087,
-327.759156825267)) ;
#41714=CARTESIAN_POINT('Ctrl Pts',(-1.13808604847684,18.5311297471719,-327.757298415554)) ;
#41715=CARTESIAN_POINT('Ctrl Pts',(-1.19721552606026,18.5274036106528,-327.756536556009)) ;
#41716=CARTESIAN_POINT('Ctrl Pts',(-1.34324105043619,18.5174996096544,-327.754662929474)) ;
#41717=CARTESIAN_POINT('Ctrl Pts',(-1.43011325053917,18.5109930698828,-327.753554964077)) ;
#41718=CARTESIAN_POINT('Ctrl Pts',(-1.74237073753988,18.4853943899725,-327.74959179762)) ;
#41719=CARTESIAN_POINT('Ctrl Pts',(-1.96744886835411,18.4627952071018,-327.746771216131)) ;
#41720=CARTESIAN_POINT('Ctrl Pts',(-2.61838087987808,18.3853991413432,-327.738658448875)) ;
#41721=CARTESIAN_POINT('Ctrl Pts',(-3.04281762954468,18.3199367309319,-327.733421447103)) ;
#41722=CARTESIAN_POINT('Ctrl Pts',(-3.68005324412878,18.1988956026787,-327.725468024274)) ;
#41723=CARTESIAN_POINT('Ctrl Pts',(-3.89476143282105,18.1541572735682,-327.72277308522)) ;
#41724=CARTESIAN_POINT('Ctrl Pts',(-4.43106801412754,18.0324556873001,-327.715976066692)) ;
#41725=CARTESIAN_POINT('Ctrl Pts',(-4.75149681272042,17.9506852016331,-327.711854687536)) ;
#41726=CARTESIAN_POINT('Ctrl Pts',(-5.21696865942547,17.8185637507548,-327.705742772273)) ;
#41727=CARTESIAN_POINT('Ctrl Pts',(-5.36384335339008,17.7749025460605,-327.703795964642)) ;
#41728=CARTESIAN_POINT('Ctrl Pts',(-5.6285406238717,17.6926368101363,-327.700251909802)) ;
#41729=CARTESIAN_POINT('Ctrl Pts',(-5.74654908214465,17.6546605871006,-327.698658995785)) ;
#41730=CARTESIAN_POINT('Ctrl Pts',(-6.00544154793853,17.5684757775857,-327.695135170074)) ;
#41731=CARTESIAN_POINT('Ctrl Pts',(-6.1461438274027,17.5197484370892,-327.693200820047)) ;
#41732=CARTESIAN_POINT('Ctrl Pts',(-6.58379266741056,17.3622628878616,-327.687123796617)) ;
#41733=CARTESIAN_POINT('Ctrl Pts',(-6.87855595940369,17.2476075337035,-327.682942521881)) ;
#41734=CARTESIAN_POINT('Ctrl Pts',(-7.65372471160755,16.9230530811344,-327.671735681111)) ;
#41735=CARTESIAN_POINT('Ctrl Pts',(-8.12841371961347,16.7002429983047,-327.664647659642)) ;
#41736=CARTESIAN_POINT('Ctrl Pts',(-8.90430989177654,16.2951241194049,-327.652883440994)) ;
#41737=CARTESIAN_POINT('Ctrl Pts',(-9.21091004192311,16.1238004760479,-327.648187767002)) ;
#41738=CARTESIAN_POINT('Ctrl Pts',(-9.59746848012484,15.8931713417723,-327.642282942083)) ;
#41739=CARTESIAN_POINT('Ctrl Pts',(-9.68206310077038,15.8417786463616,-327.640991805535)) ;
#41740=CARTESIAN_POINT('Ctrl Pts',(-9.82282137187132,15.7547169280661,-327.638847915492)) ;
#41741=CARTESIAN_POINT('Ctrl Pts',(-9.87921149240667,15.7194181034803,-327.637990316585)) ;
#41742=CARTESIAN_POINT('Ctrl Pts',(-10.002938726135,15.641039165701,-327.636112053575)) ;
#41743=CARTESIAN_POINT('Ctrl Pts',(-10.0701896683495,15.5978257910775,-327.635093153589)) ;
#41744=CARTESIAN_POINT('Ctrl Pts',(-10.2835872461133,15.4587477193681,-327.631863255471)) ;
#41745=CARTESIAN_POINT('Ctrl Pts',(-10.4286603605162,15.361252910214,-327.629672287387)) ;
#41746=CARTESIAN_POINT('Ctrl Pts',(-10.7971234600206,15.1060055067624,-327.624094693858)) ;
#41747=CARTESIAN_POINT('Ctrl Pts',(-11.0184440805897,14.945339333836,-327.620731730159)) ;
#41748=CARTESIAN_POINT('Ctrl Pts',(-11.8173135761429,14.338011808623,-327.608425168961)) ;
#41749=CARTESIAN_POINT('Ctrl Pts',(-12.3719260776933,13.8622843655092,-327.599524322198)) ;
#41750=CARTESIAN_POINT('Ctrl Pts',(-13.0077152623174,13.2483016791433,-327.588398909745)) ;
#41751=CARTESIAN_POINT('Ctrl Pts',(-13.1170167730301,13.1400922604503,-327.586451876793)) ;
#41752=CARTESIAN_POINT('Ctrl Pts',(-13.313418804879,12.9407597892092,-327.582887094733)) ;
#41753=CARTESIAN_POINT('Ctrl Pts',(-13.4009600068065,12.850083853392,-327.581273459958)) ;
#41754=CARTESIAN_POINT('Ctrl Pts',(-13.5791245074397,12.6617386793108,-327.577936997862)) ;
#41755=CARTESIAN_POINT('Ctrl Pts',(-13.6696334386174,12.5639711223193,-327.576213287411)) ;
#41756=CARTESIAN_POINT('Ctrl Pts',(-13.905629483459,12.3034795878385,-327.571641644171)) ;
#41757=CARTESIAN_POINT('Ctrl Pts',(-14.0493126197095,12.1391497210655,-327.568778647713)) ;
#41758=CARTESIAN_POINT('Ctrl Pts',(-14.3699548662752,11.7591120740141,-327.562208563336)) ;
#41759=CARTESIAN_POINT('Ctrl Pts',(-14.5450165075369,11.5418722048661,-327.558488714931)) ;
#41760=CARTESIAN_POINT('Ctrl Pts',(-14.9668816152219,10.9935178336856,-327.549212789759)) ;
#41761=CARTESIAN_POINT('Ctrl Pts',(-15.2076600057518,10.6579574189557,-327.543633533081)) ;
#41762=CARTESIAN_POINT('Ctrl Pts',(-15.624455592337,10.0341752891427,-327.533553618611)) ;
#41763=CARTESIAN_POINT('Ctrl Pts',(-15.804183263217,9.74864495568453,-327.529045062872)) ;
#41764=CARTESIAN_POINT('Ctrl Pts',(-16.0272596668256,9.37184924323189,-327.52329879195)) ;
#41765=CARTESIAN_POINT('Ctrl Pts',(-16.0777832992068,9.28490683275527,-327.521986682754)) ;
#41766=CARTESIAN_POINT('Ctrl Pts',(-16.1606556660085,9.13959302190165,-327.519819237928)) ;
#41767=CARTESIAN_POINT('Ctrl Pts',(-16.1934004430646,9.08145001032745,-327.518958803865)) ;
#41768=CARTESIAN_POINT('Ctrl Pts',(-16.264277714269,8.95399507604674,-327.517088144213)) ;
#41769=CARTESIAN_POINT('Ctrl Pts',(-16.3022820381042,8.88461354037111,-327.516079534554)) ;
#41770=CARTESIAN_POINT('Ctrl Pts',(-16.4203865304267,8.66569004043984,-327.512924339698)) ;
#41771=CARTESIAN_POINT('Ctrl Pts',(-16.4988813123755,8.51529173302976,-327.510796523704)) ;
#41772=CARTESIAN_POINT('Ctrl Pts',(-16.6928172863068,8.13095293246788,-327.505436187141)) ;
#41773=CARTESIAN_POINT('Ctrl Pts',(-16.8054095773649,7.89561611429601,-327.502225172456)) ;
#41774=CARTESIAN_POINT('Ctrl Pts',(-17.2278258307727,6.96269073945524,-327.489659864137)) ;
#41775=CARTESIAN_POINT('Ctrl Pts',(-17.4994703596249,6.24864647875538,-327.480364867702)) ;
#41776=CARTESIAN_POINT('Ctrl Pts',(-17.7750465603044,5.36367383838616,-327.468686402988)) ;
#41777=CARTESIAN_POINT('Ctrl Pts',(-17.8216310066909,5.20679800042396,-327.466611903218)) ;
#41778=CARTESIAN_POINT('Ctrl Pts',(-17.9001204887222,4.92907708628152,-327.462928705667)) ;
#41779=CARTESIAN_POINT('Ctrl Pts',(-17.9328905953612,4.80848721286577,-327.46132592238)) ;
#41780=CARTESIAN_POINT('Ctrl Pts',(-17.999772577633,4.55217191135093,-327.45791093117)) ;
#41781=CARTESIAN_POINT('Ctrl Pts',(-18.0335723387819,4.41637301256079,-327.456096748898)) ;
#41782=CARTESIAN_POINT('Ctrl Pts',(-18.125137586258,4.02989561841148,-327.450919595292)) ;
#41783=CARTESIAN_POINT('Ctrl Pts',(-18.1792328514543,3.77838109901227,-327.447533319043)) ;
#41784=CARTESIAN_POINT('Ctrl Pts',(-18.3858176098867,2.71036293994219,-327.433098767163)) ;
#41785=CARTESIAN_POINT('Ctrl Pts',(-18.4886508985518,1.88524103443056,-327.42176657293)) ;
#41786=CARTESIAN_POINT('Ctrl Pts',(-18.5459508936432,0.8794732821184,-327.408380839249)) ;
#41787=CARTESIAN_POINT('Ctrl Pts',(-18.5534860873437,0.702795843586862,
-327.406047453231)) ;
#41788=CARTESIAN_POINT('Ctrl Pts',(-18.560801208355,0.444719893812653,-327.402677620649)) ;
#41789=CARTESIAN_POINT('Ctrl Pts',(-18.5625716581819,0.363387863963918,
-327.401621231686)) ;
#41790=CARTESIAN_POINT('Ctrl Pts',(-18.5648043497484,0.216436144751031,
-327.39972427871)) ;
#41791=CARTESIAN_POINT('Ctrl Pts',(-18.5654533534118,0.150820847200539,
-327.398881658952)) ;
#41792=CARTESIAN_POINT('Ctrl Pts',(-18.5661951426942,-0.010814504401239,
-327.396816064613)) ;
#41793=CARTESIAN_POINT('Ctrl Pts',(-18.5658909149383,-0.106834464789306,
-327.39559759206)) ;
#41794=CARTESIAN_POINT('Ctrl Pts',(-18.5613098599187,-0.526097339364414,
-327.390307267628)) ;
#41795=CARTESIAN_POINT('Ctrl Pts',(-18.5493358889197,-0.849200302216394,
-327.386307360137)) ;
#41796=CARTESIAN_POINT('Ctrl Pts',(-18.4903713354712,-1.78154877808444,
-327.37481959073)) ;
#41797=CARTESIAN_POINT('Ctrl Pts',(-18.4217384227802,-2.38899615268031,
-327.367391771039)) ;
#41798=CARTESIAN_POINT('Ctrl Pts',(-18.278030612562,-3.26908998607008,-327.3563214251)) ;
#41799=CARTESIAN_POINT('Ctrl Pts',(-18.2264960909448,-3.54516462091775,
-327.352806162819)) ;
#41800=CARTESIAN_POINT('Ctrl Pts',(-18.1391487804232,-3.96061068414821,
-327.347431129771)) ;
#41801=CARTESIAN_POINT('Ctrl Pts',(-18.1079456588277,-4.1009095832651,-327.345601253152)) ;
#41802=CARTESIAN_POINT('Ctrl Pts',(-18.0469886325038,-4.36071836482692,
-327.342183470692)) ;
#41803=CARTESIAN_POINT('Ctrl Pts',(-18.0176685178356,-4.48032191818991,
-327.340598530517)) ;
#41804=CARTESIAN_POINT('Ctrl Pts',(-17.9476992302533,-4.75394180504,-327.33694539926)) ;
#41805=CARTESIAN_POINT('Ctrl Pts',(-17.9062535225901,-4.9077443926778,-327.33487202255)) ;
#41806=CARTESIAN_POINT('Ctrl Pts',(-17.7516327893757,-5.45347992247736,
-327.327444334254)) ;
#41807=CARTESIAN_POINT('Ctrl Pts',(-17.6275265602583,-5.84219272007735,
-327.322020430568)) ;
#41808=CARTESIAN_POINT('Ctrl Pts',(-17.352243789891,-6.61548316633229,-327.311015217826)) ;
#41809=CARTESIAN_POINT('Ctrl Pts',(-17.2008326364957,-6.99973844019897,
-327.30543590737)) ;
#41810=CARTESIAN_POINT('Ctrl Pts',(-16.9040824459968,-7.68491421727396,
-327.295403607562)) ;
#41811=CARTESIAN_POINT('Ctrl Pts',(-16.7631922313316,-7.98757139911168,
-327.290942221022)) ;
#41812=CARTESIAN_POINT('Ctrl Pts',(-16.568632917638,-8.37766884585339,-327.285219499371)) ;
#41813=CARTESIAN_POINT('Ctrl Pts',(-16.5222925780093,-8.46869411787894,
-327.283886265325)) ;
#41814=CARTESIAN_POINT('Ctrl Pts',(-16.4443388788663,-8.61874122268755,
-327.281694909126)) ;
#41815=CARTESIAN_POINT('Ctrl Pts',(-16.4131531957676,-8.67798269406289,
-327.280831432953)) ;
#41816=CARTESIAN_POINT('Ctrl Pts',(-16.3447854262572,-8.80616968498797,
-327.278967499968)) ;
#41817=CARTESIAN_POINT('Ctrl Pts',(-16.3074861233423,-8.8750510708676,-327.27796851838)) ;
#41818=CARTESIAN_POINT('Ctrl Pts',(-16.1902920340095,-9.08824247517432,
-327.274881778293)) ;
#41819=CARTESIAN_POINT('Ctrl Pts',(-16.1089091245678,-9.23172542978836,
-327.272811669052)) ;
#41820=CARTESIAN_POINT('Ctrl Pts',(-15.7696201586022,-9.81176136129259,
-327.264439331465)) ;
#41821=CARTESIAN_POINT('Ctrl Pts',(-15.4957938578941,-10.2387477706868,
-327.258261456983)) ;
#41822=CARTESIAN_POINT('Ctrl Pts',(-15.1886577808932,-10.6770767949344,
-327.251699502731)) ;
#41823=CARTESIAN_POINT('Ctrl Pts',(-15.1724285996487,-10.7001263758161,
-327.25135379923)) ;
#41824=CARTESIAN_POINT('Ctrl Pts',(-15.1283131277772,-10.7624794407218,
-327.25041679795)) ;
#41825=CARTESIAN_POINT('Ctrl Pts',(-15.1003262046303,-10.8017114531394,
-327.249825284613)) ;
#41826=CARTESIAN_POINT('Ctrl Pts',(-14.8081418481186,-11.2079400880309,
-327.24367873995)) ;
#41827=CARTESIAN_POINT('Ctrl Pts',(-14.5307733859594,-11.5652760229603,
-327.238082952568)) ;
#41828=CARTESIAN_POINT('Ctrl Pts',(-14.1367958958321,-12.0362658004772,
-327.230343472799)) ;
#41829=CARTESIAN_POINT('Ctrl Pts',(-14.0313367934658,-12.1590410930342,
-327.228291120769)) ;
#41830=CARTESIAN_POINT('Ctrl Pts',(-13.8417648553699,-12.3739892405408,
-327.224632574078)) ;
#41831=CARTESIAN_POINT('Ctrl Pts',(-13.7583026999586,-12.4667225364614,
-327.223032017125)) ;
#41832=CARTESIAN_POINT('Ctrl Pts',(-13.5785951187415,-12.662389588663,-327.219606332395)) ;
#41833=CARTESIAN_POINT('Ctrl Pts',(-13.482099601088,-12.7650830692869,-327.217779062408)) ;
#41834=CARTESIAN_POINT('Ctrl Pts',(-13.2020702005939,-13.0563813268648,
-327.212510596744)) ;
#41835=CARTESIAN_POINT('Ctrl Pts',(-13.0156833401025,-13.2421953495966,
-327.209044717675)) ;
#41836=CARTESIAN_POINT('Ctrl Pts',(-12.5552806087895,-13.6820687703149,
-327.2005905873)) ;
#41837=CARTESIAN_POINT('Ctrl Pts',(-12.2774229119273,-13.931940381478,-327.195574786715)) ;
#41838=CARTESIAN_POINT('Ctrl Pts',(-11.5712185273036,-14.5294710303161,
-327.18311892877)) ;
#41839=CARTESIAN_POINT('Ctrl Pts',(-11.1345579301039,-14.8667497180024,
-327.175663153653)) ;
#41840=CARTESIAN_POINT('Ctrl Pts',(-10.5900922646953,-15.249836031741,-327.166901032792)) ;
#41841=CARTESIAN_POINT('Ctrl Pts',(-10.4960458064753,-15.3147176160413,
-327.165406303006)) ;
#41842=CARTESIAN_POINT('Ctrl Pts',(-10.3498883158809,-15.4135712760725,
-327.163115835329)) ;
#41843=CARTESIAN_POINT('Ctrl Pts',(-10.2981954558067,-15.4481564596052,
-327.162311942901)) ;
#41844=CARTESIAN_POINT('Ctrl Pts',(-10.1869326175048,-15.5217903759263,
-327.160595785637)) ;
#41845=CARTESIAN_POINT('Ctrl Pts',(-10.1273097168511,-15.560757389801,-327.159684743718)) ;
#41846=CARTESIAN_POINT('Ctrl Pts',(-9.96153345483602,-15.6677453926956,
-327.157173408724)) ;
#41847=CARTESIAN_POINT('Ctrl Pts',(-9.85490913579416,-15.7350297256176,
-327.155582643134)) ;
#41848=CARTESIAN_POINT('Ctrl Pts',(-9.60441023937502,-15.8895598517041,
-327.151893241897)) ;
#41849=CARTESIAN_POINT('Ctrl Pts',(-9.46001842968493,-15.9759462870097,
-327.149802871131)) ;
#41850=CARTESIAN_POINT('Ctrl Pts',(-8.88572465180983,-16.3090175303576,
-327.141597846437)) ;
#41851=CARTESIAN_POINT('Ctrl Pts',(-8.44719131233928,-16.5404085669056,
-327.135565105366)) ;
#41852=CARTESIAN_POINT('Ctrl Pts',(-7.64130406698794,-16.9252150392383,
-327.124589088361)) ;
#41853=CARTESIAN_POINT('Ctrl Pts',(-7.27727737228563,-17.0848958171024,
-327.119670921124)) ;
#41854=CARTESIAN_POINT('Ctrl Pts',(-6.74251446880614,-17.2992757539046,
-327.11242913343)) ;
#41855=CARTESIAN_POINT('Ctrl Pts',(-6.57566939725639,-17.3633814336151,
-327.110167814012)) ;
#41856=CARTESIAN_POINT('Ctrl Pts',(-6.2891347346609,-17.4687521912117,-327.106276837682)) ;
#41857=CARTESIAN_POINT('Ctrl Pts',(-6.16990099998421,-17.5112204150779,
-327.104655563008)) ;
#41858=CARTESIAN_POINT('Ctrl Pts',(-5.92261114097204,-17.5964599248182,
-327.101287654776)) ;
#41859=CARTESIAN_POINT('Ctrl Pts',(-5.79450390610891,-17.6390603216107,
-327.099539962321)) ;
#41860=CARTESIAN_POINT('Ctrl Pts',(-5.44847080802769,-17.7499525848289,
-327.094810899392)) ;
#41861=CARTESIAN_POINT('Ctrl Pts',(-5.22973104848556,-17.8156269541973,
-327.091812466516)) ;
#41862=CARTESIAN_POINT('Ctrl Pts',(-4.85678299514989,-17.9201401541632,
-327.086688671639)) ;
#41863=CARTESIAN_POINT('Ctrl Pts',(-4.70318576815724,-17.9610636587855,
-327.084575261249)) ;
#41864=CARTESIAN_POINT('Ctrl Pts',(-3.98942674238782,-18.1414495858339,
-327.07474776227)) ;
#41865=CARTESIAN_POINT('Ctrl Pts',(-3.42348088469581,-18.2567109658516,
-327.066926043834)) ;
#41866=CARTESIAN_POINT('Ctrl Pts',(-2.56878330767499,-18.3896339221145,
-327.055331943312)) ;
#41867=CARTESIAN_POINT('Ctrl Pts',(-2.28348873981796,-18.4272342807755,
-327.051499995821)) ;
#41868=CARTESIAN_POINT('Ctrl Pts',(-1.91256883872709,-18.4673730273998,
-327.046611292322)) ;
#41869=CARTESIAN_POINT('Ctrl Pts',(-1.82763975579113,-18.4759713965464,
-327.045498301421)) ;
#41870=CARTESIAN_POINT('Ctrl Pts',(-1.675941986275,-18.4902733337497,-327.043523483468)) ;
#41871=CARTESIAN_POINT('Ctrl Pts',(-1.60919600971362,-18.4962017111698,
-327.042659173489)) ;
#41872=CARTESIAN_POINT('Ctrl Pts',(-1.46455463878849,-18.5082598894619,
-327.040796877442)) ;
#41873=CARTESIAN_POINT('Ctrl Pts',(-1.38664982029901,-18.5142595510569,
-327.039800330669)) ;
#41874=CARTESIAN_POINT('Ctrl Pts',(-1.14533825512362,-18.5313119635857,
-327.036730692307)) ;
#41875=CARTESIAN_POINT('Ctrl Pts',(-0.981821245929157,-18.5406944316804,
-327.034674975439)) ;
#41876=CARTESIAN_POINT('Ctrl Pts',(-0.313506704967963,-18.5701756938317,
-327.026338916175)) ;
#41877=CARTESIAN_POINT('Ctrl Pts',(0.191887371361827,-18.5718306373701,
-327.020182809343)) ;
#41878=CARTESIAN_POINT('Ctrl Pts',(1.22062211292943,-18.5331983854704,-327.007562259969)) ;
#41879=CARTESIAN_POINT('Ctrl Pts',(1.74345568850655,-18.4913417950225,-327.001099473812)) ;
#41880=CARTESIAN_POINT('Ctrl Pts',(2.41291219286764,-18.4090988322846,-326.992603213681)) ;
#41881=CARTESIAN_POINT('Ctrl Pts',(2.56178206666474,-18.3889732618692,-326.990700301306)) ;
#41882=CARTESIAN_POINT('Ctrl Pts',(2.83557243895069,-18.3485705150837,-326.987172986941)) ;
#41883=CARTESIAN_POINT('Ctrl Pts',(2.96056149595839,-18.3288184719743,-326.985552074971)) ;
#41884=CARTESIAN_POINT('Ctrl Pts',(3.21852982610359,-18.2853440999976,-326.982183619128)) ;
#41885=CARTESIAN_POINT('Ctrl Pts',(3.35147185961615,-18.2614451620175,-326.980435002656)) ;
#41886=CARTESIAN_POINT('Ctrl Pts',(3.70883502945817,-18.193168289506,-326.975699847009)) ;
#41887=CARTESIAN_POINT('Ctrl Pts',(3.93271592844854,-18.1460897939941,-326.972696166128)) ;
#41888=CARTESIAN_POINT('Ctrl Pts',(4.31098450706341,-18.0592166810187,-326.967561551573)) ;
#41889=CARTESIAN_POINT('Ctrl Pts',(4.46583391836849,-18.0215488203166,-326.965442583824)) ;
#41890=CARTESIAN_POINT('Ctrl Pts',(5.18238885029603,-17.837440716041,-326.955566115804)) ;
#41891=CARTESIAN_POINT('Ctrl Pts',(5.73751336929836,-17.6667026820205,-326.947699876506)) ;
#41892=CARTESIAN_POINT('Ctrl Pts',(6.55027754241457,-17.3743663462364,-326.936124556613)) ;
#41893=CARTESIAN_POINT('Ctrl Pts',(6.8146020496616,-17.2724040391494,-326.932352769708)) ;
#41894=CARTESIAN_POINT('Ctrl Pts',(7.15545619310193,-17.1318779350348,-326.927521645893)) ;
#41895=CARTESIAN_POINT('Ctrl Pts',(7.23419666587833,-17.0987775451559,-326.926407967078)) ;
#41896=CARTESIAN_POINT('Ctrl Pts',(7.37430694715388,-17.0387378622034,-326.924432324568)) ;
#41897=CARTESIAN_POINT('Ctrl Pts',(7.43576460007991,-17.0120073988872,-326.923567871249)) ;
#41898=CARTESIAN_POINT('Ctrl Pts',(7.56852706755423,-16.9534066570074,-326.921705848671)) ;
#41899=CARTESIAN_POINT('Ctrl Pts',(7.63977811235016,-16.9214180749242,-326.920709712633)) ;
#41900=CARTESIAN_POINT('Ctrl Pts',(7.85963152476459,-16.8210419030549,-326.917642951098)) ;
#41901=CARTESIAN_POINT('Ctrl Pts',(8.00753364832913,-16.751139168346,-326.915589654346)) ;
#41902=CARTESIAN_POINT('Ctrl Pts',(8.60806260536747,-16.4575410123078,-326.907259696739)) ;
#41903=CARTESIAN_POINT('Ctrl Pts',(9.05239930101172,-16.2173816356411,-326.901107251101)) ;
#41904=CARTESIAN_POINT('Ctrl Pts',(9.89992404181671,-15.7136065167819,-326.889020299012)) ;
#41905=CARTESIAN_POINT('Ctrl Pts',(10.3037426475419,-15.4518222876854,-326.883093875213)) ;
#41906=CARTESIAN_POINT('Ctrl Pts',(10.8485254486814,-15.0677932309612,-326.874725006155)) ;
#41907=CARTESIAN_POINT('Ctrl Pts',(10.9985043757455,-14.9586696802507,-326.872380608035)) ;
#41908=CARTESIAN_POINT('Ctrl Pts',(11.2478581320256,-14.7714640001729,-326.868409279703)) ;
#41909=CARTESIAN_POINT('Ctrl Pts',(11.3481163179081,-14.6945812205917,-326.866792023233)) ;
#41910=CARTESIAN_POINT('Ctrl Pts',(11.5520577639608,-14.5348571101698,-326.863458904786)) ;
#41911=CARTESIAN_POINT('Ctrl Pts',(11.6556532728351,-14.4519153234459,-326.861742272353)) ;
#41912=CARTESIAN_POINT('Ctrl Pts',(11.763731802875,-14.3634662190082,-326.859926218642)) ;
#41913=CARTESIAN_POINT('Ctrl Pts',(11.7691105724771,-14.3590593037066,-326.859835772614)) ;
#41914=CARTESIAN_POINT('Ctrl Pts',(11.7800085429609,-14.3501201783384,-326.859652385209)) ;
#41915=CARTESIAN_POINT('Ctrl Pts',(11.7855276071371,-14.3455878034463,-326.859559442508)) ;
#41916=CARTESIAN_POINT('Ctrl Pts',(11.7967823836165,-14.336334258935,-326.859369766371)) ;
#41917=CARTESIAN_POINT('Ctrl Pts',(11.8025178801671,-14.3316128289402,-326.859273030844)) ;
#41918=CARTESIAN_POINT('Ctrl Pts',(11.8142881235422,-14.3219117701261,-326.859074357513)) ;
#41919=CARTESIAN_POINT('Ctrl Pts',(11.8203225595079,-14.3169317664967,-326.858972416703)) ;
#41920=CARTESIAN_POINT('Ctrl Pts',(11.8327834897189,-14.3066349592115,-326.858761738745)) ;
#41921=CARTESIAN_POINT('Ctrl Pts',(11.839209552689,-14.3013176364348,-326.85865299744)) ;
#41922=CARTESIAN_POINT('Ctrl Pts',(11.8525610819794,-14.2902545875103,-326.858426865741)) ;
#41923=CARTESIAN_POINT('Ctrl Pts',(11.8594859585686,-14.2845081531149,-326.85830946969)) ;
#41924=CARTESIAN_POINT('Ctrl Pts',(11.873962138257,-14.2724776774405,-326.858063825591)) ;
#41925=CARTESIAN_POINT('Ctrl Pts',(11.8815126369119,-14.2661926726326,-326.85793556987)) ;
#41926=CARTESIAN_POINT('Ctrl Pts',(11.897393025874,-14.2529525485445,-326.857665540604)) ;
#41927=CARTESIAN_POINT('Ctrl Pts',(11.9057218138867,-14.2459961130658,-326.857523756618)) ;
#41928=CARTESIAN_POINT('Ctrl Pts',(12.0403021745294,-14.1333903992495,-326.855230131147)) ;
#41929=CARTESIAN_POINT('Ctrl Pts',(12.1651490286888,-14.0260739208042,-326.853065065705)) ;
#41930=CARTESIAN_POINT('Ctrl Pts',(12.5064518450368,-13.7247098460763,-326.847044538442)) ;
#41931=CARTESIAN_POINT('Ctrl Pts',(12.7198026667733,-13.5272176649301,-326.843164512395)) ;
#41932=CARTESIAN_POINT('Ctrl Pts',(13.1628326807557,-13.0973663741485,-326.834881612142)) ;
#41933=CARTESIAN_POINT('Ctrl Pts',(13.3911950303763,-12.8637889274182,-326.830474597117)) ;
#41934=CARTESIAN_POINT('Ctrl Pts',(13.7269862903283,-12.5016923535573,-326.823828835522)) ;
#41935=CARTESIAN_POINT('Ctrl Pts',(13.8390341276396,-12.3775441339682,-326.821581974367)) ;
#41936=CARTESIAN_POINT('Ctrl Pts',(14.0543795370975,-12.1323627985403,-326.817216788125)) ;
#41937=CARTESIAN_POINT('Ctrl Pts',(14.1578288525864,-12.0114817374491,-326.815097712751)) ;
#41938=CARTESIAN_POINT('Ctrl Pts',(14.3503056822411,-11.7806298485435,-326.811123284633)) ;
#41939=CARTESIAN_POINT('Ctrl Pts',(14.4396548652993,-11.6709417049327,-326.809264867421)) ;
#41940=CARTESIAN_POINT('Ctrl Pts',(14.5739290938495,-11.5021994631817,-326.80645799936)) ;
#41941=CARTESIAN_POINT('Ctrl Pts',(14.6197681828415,-11.4438795879201,-326.805497219165)) ;
#41942=CARTESIAN_POINT('Ctrl Pts',(14.6922250685337,-11.3505487071763,-326.803975518865)) ;
#41943=CARTESIAN_POINT('Ctrl Pts',(14.7190700372476,-11.315715207371,-326.803411103947)) ;
#41944=CARTESIAN_POINT('Ctrl Pts',(14.7465703595737,-11.2797678911374,-326.802832107947)) ;
#41945=CARTESIAN_POINT('Ctrl Pts',(14.7473496241855,-11.2787490489783,-326.802815700517)) ;
#41946=CARTESIAN_POINT('Ctrl Pts',(14.7499434648194,-11.2753570281298,-326.802761084904)) ;
#41947=CARTESIAN_POINT('Ctrl Pts',(14.7517575736512,-11.2729834921988,-326.80272288356)) ;
#41948=CARTESIAN_POINT('Ctrl Pts',(14.7552181175223,-11.2684535348797,-326.802650004615)) ;
#41949=CARTESIAN_POINT('Ctrl Pts',(14.7568646529083,-11.266297190255,-326.802615325555)) ;
#41950=CARTESIAN_POINT('Ctrl Pts',(14.8120457641581,-11.1939977526916,-326.801453005475)) ;
#41951=CARTESIAN_POINT('Ctrl Pts',(14.8650801360856,-11.1234741867984,-326.800332600198)) ;
#41952=CARTESIAN_POINT('Ctrl Pts',(15.0667076902149,-10.8513384060217,-326.796055070246)) ;
#41953=CARTESIAN_POINT('Ctrl Pts',(15.2117186656336,-10.6471048429403,-326.792940333628)) ;
#41954=CARTESIAN_POINT('Ctrl Pts',(15.6654335182437,-9.97989396203828,-326.782978132254)) ;
#41955=CARTESIAN_POINT('Ctrl Pts',(15.9574719049475,-9.50595512145185,-326.776216220472)) ;
#41956=CARTESIAN_POINT('Ctrl Pts',(16.4067733843464,-8.69758742689565,-326.764815534732)) ;
#41957=CARTESIAN_POINT('Ctrl Pts',(16.5761363768627,-8.37030118178966,-326.760236085769)) ;
#41958=CARTESIAN_POINT('Ctrl Pts',(16.8046679886038,-7.89449467826937,-326.753577494318)) ;
#41959=CARTESIAN_POINT('Ctrl Pts',(16.8718333958693,-7.74991291513527,-326.751554341734)) ;
#41960=CARTESIAN_POINT('Ctrl Pts',(16.9880338624197,-7.49110480250484,-326.747930339098)) ;
#41961=CARTESIAN_POINT('Ctrl Pts',(17.0377995300502,-7.3772171443979,-326.746334788592)) ;
#41962=CARTESIAN_POINT('Ctrl Pts',(17.1375013357732,-7.14266054272902,-326.743046238123)) ;
#41963=CARTESIAN_POINT('Ctrl Pts',(17.1873153957241,-7.02194710112931,-326.741352487818)) ;
#41964=CARTESIAN_POINT('Ctrl Pts',(17.2512928246325,-6.86215134762048,-326.739108567134)) ;
#41965=CARTESIAN_POINT('Ctrl Pts',(17.2666043842565,-6.82353268289879,-326.738566132553)) ;
#41966=CARTESIAN_POINT('Ctrl Pts',(17.3969646713326,-6.49149080947905,-326.733901199319)) ;
#41967=CARTESIAN_POINT('Ctrl Pts',(17.504653881744,-6.19523401088165,-326.729730585535)) ;
#41968=CARTESIAN_POINT('Ctrl Pts',(17.7802828379706,-5.37229208113595,-326.718150431057)) ;
#41969=CARTESIAN_POINT('Ctrl Pts',(17.9323257840963,-4.84062702754272,-326.710668038348)) ;
#41970=CARTESIAN_POINT('Ctrl Pts',(18.1335910854552,-3.99587740362943,-326.699012057862)) ;
#41971=CARTESIAN_POINT('Ctrl Pts',(18.1989139221187,-3.68696279482137,-326.694799579853)) ;
#41972=CARTESIAN_POINT('Ctrl Pts',(18.2739658323541,-3.28117010923824,-326.689388751037)) ;
#41973=CARTESIAN_POINT('Ctrl Pts',(18.2908558466787,-3.18567056729326,-326.688124258517)) ;
#41974=CARTESIAN_POINT('Ctrl Pts',(18.318030577803,-3.02467354618739,-326.686009986932)) ;
#41975=CARTESIAN_POINT('Ctrl Pts',(18.3287141013367,-2.95924546727753,-326.685155683198)) ;
#41976=CARTESIAN_POINT('Ctrl Pts',(18.3488092341081,-2.83189371192019,-326.683502828001)) ;
#41977=CARTESIAN_POINT('Ctrl Pts',(18.358258345277,-2.76997704770864,-326.682703671237)) ;
#41978=CARTESIAN_POINT('Ctrl Pts',(18.3794314212705,-2.62636838494424,-326.68085926728)) ;
#41979=CARTESIAN_POINT('Ctrl Pts',(18.390924367199,-2.54464363024246,-326.679816501654)) ;
#41980=CARTESIAN_POINT('Ctrl Pts',(18.4717828128968,-1.94048590755105,-326.672150349244)) ;
#41981=CARTESIAN_POINT('Ctrl Pts',(18.5194196832725,-1.41539532641382,-326.665715364132)) ;
#41982=CARTESIAN_POINT('Ctrl Pts',(18.5446545943314,-0.888979965716119,
-326.659259832385)) ;
#41983=CARTESIAN_POINT('Ctrl Pts',(18.5446545937382,-0.888979978089846,
-326.364137692133)) ;
#41984=CARTESIAN_POINT('Ctrl Pts',(18.5026962120991,-1.76425694043673,-326.374949702051)) ;
#41985=CARTESIAN_POINT('Ctrl Pts',(18.3988248501205,-2.63545455372144,-326.385538532625)) ;
#41986=CARTESIAN_POINT('Ctrl Pts',(18.2084207684801,-3.62851206867422,-326.398258197816)) ;
#41987=CARTESIAN_POINT('Ctrl Pts',(18.1815835253599,-3.76067908291487,-326.399963143586)) ;
#41988=CARTESIAN_POINT('Ctrl Pts',(18.128961717625,-4.00608682932487,-326.403153455714)) ;
#41989=CARTESIAN_POINT('Ctrl Pts',(18.1035499750231,-4.11940079429492,-326.404636346405)) ;
#41990=CARTESIAN_POINT('Ctrl Pts',(18.0483068395658,-4.35534687042108,-326.407745495943)) ;
#41991=CARTESIAN_POINT('Ctrl Pts',(18.0182847216749,-4.47792829015448,-326.409372954154)) ;
#41992=CARTESIAN_POINT('Ctrl Pts',(17.9433558844881,-4.77090422569198,-326.413292452849)) ;
#41993=CARTESIAN_POINT('Ctrl Pts',(17.8972686136077,-4.94098406780114,-326.415592169263)) ;
#41994=CARTESIAN_POINT('Ctrl Pts',(17.7373329291751,-5.49958319063575,-326.423224370962)) ;
#41995=CARTESIAN_POINT('Ctrl Pts',(17.6131984992922,-5.88503457085696,-326.428620443018)) ;
#41996=CARTESIAN_POINT('Ctrl Pts',(17.309708388988,-6.73148591367984,-326.440692778461)) ;
#41997=CARTESIAN_POINT('Ctrl Pts',(17.1243324833767,-7.19000303772743,-326.447385220849)) ;
#41998=CARTESIAN_POINT('Ctrl Pts',(16.8517138762357,-7.79374650243736,-326.456238127008)) ;
#41999=CARTESIAN_POINT('Ctrl Pts',(16.7804723441072,-7.94597339193071,-326.458473238092)) ;
#42000=CARTESIAN_POINT('Ctrl Pts',(16.6666552553487,-8.18081494621922,-326.461915464164)) ;
#42001=CARTESIAN_POINT('Ctrl Pts',(16.625509751875,-8.26411254194308,-326.46313522741)) ;
#42002=CARTESIAN_POINT('Ctrl Pts',(16.5807153724435,-8.35310854842434,-326.464435810253)) ;
#42003=CARTESIAN_POINT('Ctrl Pts',(16.5776867415473,-8.35911759594778,-326.464523613226)) ;
#42004=CARTESIAN_POINT('Ctrl Pts',(16.5722108395581,-8.36996754564659,-326.464682126233)) ;
#42005=CARTESIAN_POINT('Ctrl Pts',(16.5697647126626,-8.37480902426757,-326.464752849388)) ;
#42006=CARTESIAN_POINT('Ctrl Pts',(16.565283052362,-8.38366966755605,-326.464882267086)) ;
#42007=CARTESIAN_POINT('Ctrl Pts',(16.563248177161,-8.38768916456408,-326.464940969271)) ;
#42008=CARTESIAN_POINT('Ctrl Pts',(16.5594714288274,-8.39514265672645,-326.465049810981)) ;
#42009=CARTESIAN_POINT('Ctrl Pts',(16.5577299500929,-8.39857685139204,-326.465099955133)) ;
#42010=CARTESIAN_POINT('Ctrl Pts',(16.5544564280303,-8.40502725870876,-326.465194131407)) ;
#42011=CARTESIAN_POINT('Ctrl Pts',(16.5529246284303,-8.4080435948383,-326.465238166413)) ;
#42012=CARTESIAN_POINT('Ctrl Pts',(16.5500087060112,-8.41378158479565,-326.465321927329)) ;
#42013=CARTESIAN_POINT('Ctrl Pts',(16.5486247360639,-8.41650331614191,-326.465361655061)) ;
#42014=CARTESIAN_POINT('Ctrl Pts',(16.5459564834907,-8.4217475301289,-326.465438196262)) ;
#42015=CARTESIAN_POINT('Ctrl Pts',(16.5446722953049,-8.42427006070976,-326.465475010864)) ;
#42016=CARTESIAN_POINT('Ctrl Pts',(16.5421637659266,-8.42919477846355,-326.465546878501)) ;
#42017=CARTESIAN_POINT('Ctrl Pts',(16.5409394782403,-8.43159699281256,-326.465581932181)) ;
#42018=CARTESIAN_POINT('Ctrl Pts',(16.5385146740669,-8.43635221858807,-326.465651316676)) ;
#42019=CARTESIAN_POINT('Ctrl Pts',(16.5373141785866,-8.43870524068253,-326.465685647746)) ;
#42020=CARTESIAN_POINT('Ctrl Pts',(16.5349005514442,-8.44343355928576,-326.465754630053)) ;
#42021=CARTESIAN_POINT('Ctrl Pts',(16.533687409984,-8.44580885085371,-326.465789281171)) ;
#42022=CARTESIAN_POINT('Ctrl Pts',(16.5017146899841,-8.50837710952026,-326.466701971268)) ;
#42023=CARTESIAN_POINT('Ctrl Pts',(16.4706270833373,-8.56840196580296,-326.467575970412)) ;
#42024=CARTESIAN_POINT('Ctrl Pts',(16.4101781619319,-8.68357387096116,-326.469248870667)) ;
#42025=CARTESIAN_POINT('Ctrl Pts',(16.3808649389626,-8.73874512399434,-326.470048445458)) ;
#42026=CARTESIAN_POINT('Ctrl Pts',(16.296372807625,-8.89585116376364,-326.47232155885)) ;
#42027=CARTESIAN_POINT('Ctrl Pts',(16.2405169806811,-8.99741867849112,-326.473786568648)) ;
#42028=CARTESIAN_POINT('Ctrl Pts',(15.9975510284008,-9.42958993405747,-326.480013466453)) ;
#42029=CARTESIAN_POINT('Ctrl Pts',(15.8012688538205,-9.75493255524212,-326.484685869259)) ;
#42030=CARTESIAN_POINT('Ctrl Pts',(15.3341720318717,-10.4780241237083,-326.495240181844)) ;
#42031=CARTESIAN_POINT('Ctrl Pts',(15.0575995565262,-10.8717301703389,-326.501111465497)) ;
#42032=CARTESIAN_POINT('Ctrl Pts',(14.6367784555695,-11.4238652213471,-326.509713084837)) ;
#42033=CARTESIAN_POINT('Ctrl Pts',(14.5045911362948,-11.59123875736,-326.512371249507)) ;
#42034=CARTESIAN_POINT('Ctrl Pts',(14.2614378024571,-11.8884415061596,-326.517195995861)) ;
#42035=CARTESIAN_POINT('Ctrl Pts',(14.1515081331023,-12.019087614111,-326.519354620518)) ;
#42036=CARTESIAN_POINT('Ctrl Pts',(13.9687765969683,-12.2302722403605,-326.522910025976)) ;
#42037=CARTESIAN_POINT('Ctrl Pts',(13.897042669628,-12.3117213944365,-326.524297759316)) ;
#42038=CARTESIAN_POINT('Ctrl Pts',(13.7401835510086,-12.486706904515,-326.527315879451)) ;
#42039=CARTESIAN_POINT('Ctrl Pts',(13.6548084335803,-12.5800119206167,-326.528948397727)) ;
#42040=CARTESIAN_POINT('Ctrl Pts',(13.4621564747937,-12.7862860172731,-326.532610243105)) ;
#42041=CARTESIAN_POINT('Ctrl Pts',(13.3543976250305,-12.8987918442656,-326.53464371311)) ;
#42042=CARTESIAN_POINT('Ctrl Pts',(12.7490140392894,-13.5151248703991,-326.545985127595)) ;
#42043=CARTESIAN_POINT('Ctrl Pts',(12.2242964354032,-13.9915162817371,-326.555537600353)) ;
#42044=CARTESIAN_POINT('Ctrl Pts',(11.4527875671398,-14.6153630220403,-326.568893310128)) ;
#42045=CARTESIAN_POINT('Ctrl Pts',(11.2278484966696,-14.7888673594368,-326.572708144822)) ;
#42046=CARTESIAN_POINT('Ctrl Pts',(10.8548365340942,-15.0631687530199,-326.578860392525)) ;
#42047=CARTESIAN_POINT('Ctrl Pts',(10.7091298846897,-15.1671047458488,-326.581221826115)) ;
#42048=CARTESIAN_POINT('Ctrl Pts',(10.4956586715981,-15.3147688324228,-326.584608868726)) ;
#42049=CARTESIAN_POINT('Ctrl Pts',(10.4290762321194,-15.3601876391559,-326.585655229476)) ;
#42050=CARTESIAN_POINT('Ctrl Pts',(10.3071154311353,-15.4422238713289,-326.58755200359)) ;
#42051=CARTESIAN_POINT('Ctrl Pts',(10.2518325376521,-15.4789804643998,-326.588404257032)) ;
#42052=CARTESIAN_POINT('Ctrl Pts',(10.1146168702492,-15.5691551216043,-326.590501884071)) ;
#42053=CARTESIAN_POINT('Ctrl Pts',(10.0324568471083,-15.6222237624314,-326.591742541342)) ;
#42054=CARTESIAN_POINT('Ctrl Pts',(9.67087666360603,-15.8517460809997,-326.59714376199)) ;
#42055=CARTESIAN_POINT('Ctrl Pts',(9.38719244648079,-16.0213709846403,-326.601229792122)) ;
#42056=CARTESIAN_POINT('Ctrl Pts',(8.62781128111609,-16.4483355053427,-326.611937772282)) ;
#42057=CARTESIAN_POINT('Ctrl Pts',(8.14513905944076,-16.6926204848564,-326.618519881164)) ;
#42058=CARTESIAN_POINT('Ctrl Pts',(7.51214651626492,-16.9789835706538,-326.627116045082)) ;
#42059=CARTESIAN_POINT('Ctrl Pts',(7.37101364914425,-17.0407272758858,-326.62902978514)) ;
#42060=CARTESIAN_POINT('Ctrl Pts',(7.0231418137628,-17.1877861238651,-326.633746779964)) ;
#42061=CARTESIAN_POINT('Ctrl Pts',(6.81559850700049,-17.2711357330323,-326.636561044861)) ;
#42062=CARTESIAN_POINT('Ctrl Pts',(6.48121165108943,-17.3984596098192,-326.641104776613)) ;
#42063=CARTESIAN_POINT('Ctrl Pts',(6.3553090705216,-17.4448430149358,-326.642817627475)) ;
#42064=CARTESIAN_POINT('Ctrl Pts',(6.1106503911945,-17.5319768345413,-326.646151410397)) ;
#42065=CARTESIAN_POINT('Ctrl Pts',(5.99196181511737,-17.5728954211767,-326.647771078563)) ;
#42066=CARTESIAN_POINT('Ctrl Pts',(5.72918665287508,-17.6605169583859,-326.651362753569)) ;
#42067=CARTESIAN_POINT('Ctrl Pts',(5.58492510840863,-17.7066668343848,-326.653338352609)) ;
#42068=CARTESIAN_POINT('Ctrl Pts',(4.9892194111868,-17.8892311497806,-326.66151084462)) ;
#42069=CARTESIAN_POINT('Ctrl Pts',(4.53322359772509,-18.0101855339538,-326.66780567846)) ;
#42070=CARTESIAN_POINT('Ctrl Pts',(3.82116789865146,-18.1703017263502,-326.677617122839)) ;
#42071=CARTESIAN_POINT('Ctrl Pts',(3.56806143119564,-18.2216938428152,-326.681100049528)) ;
#42072=CARTESIAN_POINT('Ctrl Pts',(3.04089049258729,-18.3173280946925,-326.688310880042)) ;
#42073=CARTESIAN_POINT('Ctrl Pts',(2.76673857958043,-18.3607374976121,-326.692036801902)) ;
#42074=CARTESIAN_POINT('Ctrl Pts',(2.31690557091818,-18.4216602786168,-326.698066771517)) ;
#42075=CARTESIAN_POINT('Ctrl Pts',(2.14176562914686,-18.4428430298319,-326.700393780918)) ;
#42076=CARTESIAN_POINT('Ctrl Pts',(1.88660611214707,-18.4700202503915,-326.703741676239)) ;
#42077=CARTESIAN_POINT('Ctrl Pts',(1.80680769534469,-18.477997095145,-326.704782679929)) ;
#42078=CARTESIAN_POINT('Ctrl Pts',(1.66077834452336,-18.4916395416229,-326.706675129455)) ;
#42079=CARTESIAN_POINT('Ctrl Pts',(1.59456405899212,-18.4974669374542,-326.707528344996)) ;
#42080=CARTESIAN_POINT('Ctrl Pts',(1.43014041887756,-18.5110481265793,-326.70963581415)) ;
#42081=CARTESIAN_POINT('Ctrl Pts',(1.33189791211798,-18.5183760722902,-326.710885237192)) ;
#42082=CARTESIAN_POINT('Ctrl Pts',(0.887849653158683,-18.5479458957626,
-326.716496754199)) ;
#42083=CARTESIAN_POINT('Ctrl Pts',(0.541519906217356,-18.5612858197278,
-326.720776662602)) ;
#42084=CARTESIAN_POINT('Ctrl Pts',(-0.333091452918507,-18.5704733806766,
-326.731520456152)) ;
#42085=CARTESIAN_POINT('Ctrl Pts',(-0.861198435910072,-18.5534840155664,
-326.737953188577)) ;
#42086=CARTESIAN_POINT('Ctrl Pts',(-1.60943875228085,-18.4973938370672,
-326.747239588024)) ;
#42087=CARTESIAN_POINT('Ctrl Pts',(-1.83069987676984,-18.4768073435676,
-326.750006020787)) ;
#42088=CARTESIAN_POINT('Ctrl Pts',(-2.23688642803872,-18.4316471665521,
-326.755136618579)) ;
#42089=CARTESIAN_POINT('Ctrl Pts',(-2.42191376619061,-18.4082484695159,
-326.757493638808)) ;
#42090=CARTESIAN_POINT('Ctrl Pts',(-2.73306140678452,-18.3641280738278,
-326.761495834665)) ;
#42091=CARTESIAN_POINT('Ctrl Pts',(-2.85937722285068,-18.344884475177,-326.763131325918)) ;
#42092=CARTESIAN_POINT('Ctrl Pts',(-3.11651859208449,-18.3029898389316,
-326.766483647797)) ;
#42093=CARTESIAN_POINT('Ctrl Pts',(-3.24732008033496,-18.2802362515444,
-326.768201065447)) ;
#42094=CARTESIAN_POINT('Ctrl Pts',(-3.58989884209959,-18.2168499665864,
-326.772731545598)) ;
#42095=CARTESIAN_POINT('Ctrl Pts',(-3.80123163847965,-18.1739273185073,
-326.775559164704)) ;
#42096=CARTESIAN_POINT('Ctrl Pts',(-4.29407840478718,-18.0648551749294,
-326.782226721592)) ;
#42097=CARTESIAN_POINT('Ctrl Pts',(-4.57488985058449,-17.9957907359514,
-326.786082570072)) ;
#42098=CARTESIAN_POINT('Ctrl Pts',(-5.35702463897054,-17.7839369634897,
-326.79694886986)) ;
#42099=CARTESIAN_POINT('Ctrl Pts',(-5.85411482890597,-17.6265556957852,
-326.804008011476)) ;
#42100=CARTESIAN_POINT('Ctrl Pts',(-6.57716100012093,-17.3636702188845,
-326.814294057897)) ;
#42101=CARTESIAN_POINT('Ctrl Pts',(-6.80867522810172,-17.2742013523003,
-326.817589055323)) ;
#42102=CARTESIAN_POINT('Ctrl Pts',(-7.12125133463936,-17.146145616605,-326.822009364928)) ;
#42103=CARTESIAN_POINT('Ctrl Pts',(-7.20392927243562,-17.1115730763335,
-326.823175777074)) ;
#42104=CARTESIAN_POINT('Ctrl Pts',(-7.34684338374057,-17.0505928598623,
-326.825185104049)) ;
#42105=CARTESIAN_POINT('Ctrl Pts',(-7.40719534712128,-17.0244612744748,
-326.82603136068)) ;
#42106=CARTESIAN_POINT('Ctrl Pts',(-7.54526879173654,-16.9638041328658,
-326.827962184028)) ;
#42107=CARTESIAN_POINT('Ctrl Pts',(-7.62289428577533,-16.9290641954369,
-326.829044106759)) ;
#42108=CARTESIAN_POINT('Ctrl Pts',(-7.87580453842161,-16.8137863853595,
-326.832561264233)) ;
#42109=CARTESIAN_POINT('Ctrl Pts',(-8.05007343311089,-16.731049808631,-326.83497250127)) ;
#42110=CARTESIAN_POINT('Ctrl Pts',(-8.82008018878329,-16.3506623567819,
-326.845629698817)) ;
#42111=CARTESIAN_POINT('Ctrl Pts',(-9.40083792657956,-16.0238018113441,
-326.853694057912)) ;
#42112=CARTESIAN_POINT('Ctrl Pts',(-10.105358910533,-15.5757751482347,-326.864003435448)) ;
#42113=CARTESIAN_POINT('Ctrl Pts',(-10.2466955456567,-15.4831611917713,
-326.866098384733)) ;
#42114=CARTESIAN_POINT('Ctrl Pts',(-10.5838325823997,-15.255606349652,-326.871169956836)) ;
#42115=CARTESIAN_POINT('Ctrl Pts',(-10.778343027701,-15.1188081045015,-326.8741579211)) ;
#42116=CARTESIAN_POINT('Ctrl Pts',(-11.0804064847131,-14.8975756927966,
-326.87890846046)) ;
#42117=CARTESIAN_POINT('Ctrl Pts',(-11.1897462746621,-14.8156251178051,
-326.880651442179)) ;
#42118=CARTESIAN_POINT('Ctrl Pts',(-11.398079710107,-14.6558565226824,-326.884019278324)) ;
#42119=CARTESIAN_POINT('Ctrl Pts',(-11.4972059978724,-14.5782236805645,
-326.885642564963)) ;
#42120=CARTESIAN_POINT('Ctrl Pts',(-11.7314942634099,-14.3908598995086,
-326.889529925693)) ;
#42121=CARTESIAN_POINT('Ctrl Pts',(-11.8659174741564,-14.2802243910504,
-326.891801338814)) ;
#42122=CARTESIAN_POINT('Ctrl Pts',(-12.5338390519738,-13.7145556238068,
-326.903294233929)) ;
#42123=CARTESIAN_POINT('Ctrl Pts',(-13.0428104244999,-13.2314491202778,
-326.91275138245)) ;
#42124=CARTESIAN_POINT('Ctrl Pts',(-13.7196024215848,-12.5119602908376,
-326.926048790745)) ;
#42125=CARTESIAN_POINT('Ctrl Pts',(-13.9111127046318,-12.2986822287112,
-326.929898613203)) ;
#42126=CARTESIAN_POINT('Ctrl Pts',(-14.2147134096491,-11.94440493153,-326.936098814283)) ;
#42127=CARTESIAN_POINT('Ctrl Pts',(-14.3298250477942,-11.8060578002989,
-326.938473634115)) ;
#42128=CARTESIAN_POINT('Ctrl Pts',(-14.4936486020641,-11.6032396571846,
-326.941875877965)) ;
#42129=CARTESIAN_POINT('Ctrl Pts',(-14.5439796222735,-11.5400899958964,
-326.9429243025)) ;
#42130=CARTESIAN_POINT('Ctrl Pts',(-14.6349155734363,-11.4244539798501,
-326.944822764228)) ;
#42131=CARTESIAN_POINT('Ctrl Pts',(-14.6756540450582,-11.3720746094886,
-326.945674668497)) ;
#42132=CARTESIAN_POINT('Ctrl Pts',(-14.7755808518664,-11.2421627898323,
-326.947768605728)) ;
#42133=CARTESIAN_POINT('Ctrl Pts',(-14.8344406618585,-11.1643801436847,
-326.949005965313)) ;
#42134=CARTESIAN_POINT('Ctrl Pts',(-15.0972407780093,-10.8113447057897,
-326.95455682066)) ;
#42135=CARTESIAN_POINT('Ctrl Pts',(-15.2941525851511,-10.530942562824,-326.958789604085)) ;
#42136=CARTESIAN_POINT('Ctrl Pts',(-15.8466543919673,-9.69597122318395,
-326.971090584124)) ;
#42137=CARTESIAN_POINT('Ctrl Pts',(-16.1806276098271,-9.12773818663991,
-326.979100068229)) ;
#42138=CARTESIAN_POINT('Ctrl Pts',(-16.5930126794276,-8.33203864512454,
-326.990274897359)) ;
#42139=CARTESIAN_POINT('Ctrl Pts',(-16.698268692159,-8.11903689758766,-326.993260292732)) ;
#42140=CARTESIAN_POINT('Ctrl Pts',(-16.8575634849551,-7.7804699637858,-326.998007775332)) ;
#42141=CARTESIAN_POINT('Ctrl Pts',(-16.9143530068844,-7.65622764805146,
-326.999750314675)) ;
#42142=CARTESIAN_POINT('Ctrl Pts',(-17.0208454958791,-7.41627759587268,
-327.003117885688)) ;
#42143=CARTESIAN_POINT('Ctrl Pts',(-17.0707525642146,-7.30066857292239,
-327.004741356466)) ;
#42144=CARTESIAN_POINT('Ctrl Pts',(-17.1868844039221,-7.02394788102239,
-327.008630155542)) ;
#42145=CARTESIAN_POINT('Ctrl Pts',(-17.2520254418457,-6.86239443382043,
-327.010902837924)) ;
#42146=CARTESIAN_POINT('Ctrl Pts',(-17.5677373359511,-6.04649045394342,
-327.022390462494)) ;
#42147=CARTESIAN_POINT('Ctrl Pts',(-17.7833957758326,-5.37924426551951,
-327.031840621406)) ;
#42148=CARTESIAN_POINT('Ctrl Pts',(-18.0334467181512,-4.42397398597466,
-327.045133693862)) ;
#42149=CARTESIAN_POINT('Ctrl Pts',(-18.0996311539107,-4.14488827056821,
-327.048986028345)) ;
#42150=CARTESIAN_POINT('Ctrl Pts',(-18.1967973663554,-3.6882892700022,-327.055189668817)) ;
#42151=CARTESIAN_POINT('Ctrl Pts',(-18.2317072643957,-3.51166093957875,
-327.057565446302)) ;
#42152=CARTESIAN_POINT('Ctrl Pts',(-18.2785483351576,-3.25510259237579,
-327.060968777187)) ;
#42153=CARTESIAN_POINT('Ctrl Pts',(-18.2925353483904,-3.17555864058567,
-327.062017348951)) ;
#42154=CARTESIAN_POINT('Ctrl Pts',(-18.3170676758039,-3.03050062812811,
-327.06391593152)) ;
#42155=CARTESIAN_POINT('Ctrl Pts',(-18.327781604383,-2.96501665321094,-327.064767811325)) ;
#42156=CARTESIAN_POINT('Ctrl Pts',(-18.3533745148706,-2.80315071780301,
-327.06686148744)) ;
#42157=CARTESIAN_POINT('Ctrl Pts',(-18.3678455800112,-2.70670626748359,
-327.068098613414)) ;
#42158=CARTESIAN_POINT('Ctrl Pts',(-18.4266432688807,-2.29263347197853,
-327.073373475872)) ;
#42159=CARTESIAN_POINT('Ctrl Pts',(-18.4634958561383,-1.97399900787125,
-327.077341255139)) ;
#42160=CARTESIAN_POINT('Ctrl Pts',(-18.5030135767353,-1.5323345106877,-327.082793833516)) ;
#42161=CARTESIAN_POINT('Ctrl Pts',(-18.5127382627211,-1.40999379632923,
-327.084299084285)) ;
#42162=CARTESIAN_POINT('Ctrl Pts',(-18.5533492189315,-0.825817260896462,
-327.091475289535)) ;
#42163=CARTESIAN_POINT('Ctrl Pts',(-18.5681703565681,-0.363029938491348,
-327.097130875431)) ;
#42164=CARTESIAN_POINT('Ctrl Pts',(-18.5640843027216,0.396896815357878,
-327.106551427455)) ;
#42165=CARTESIAN_POINT('Ctrl Pts',(-18.5553570354474,0.693886034294105,
-327.110265519233)) ;
#42166=CARTESIAN_POINT('Ctrl Pts',(-18.5317084776999,1.13650706957426,-327.115873980792)) ;
#42167=CARTESIAN_POINT('Ctrl Pts',(-18.5221858862663,1.28237956002616,-327.117734058904)) ;
#42168=CARTESIAN_POINT('Ctrl Pts',(-18.5013960050624,1.55185211176864,-327.121193869744)) ;
#42169=CARTESIAN_POINT('Ctrl Pts',(-18.4906101098028,1.67548107396545,-327.122790386258)) ;
#42170=CARTESIAN_POINT('Ctrl Pts',(-18.4634203347717,1.95476438800068,-327.126418548748)) ;
#42171=CARTESIAN_POINT('Ctrl Pts',(-18.4462860008254,2.11033811174323,-327.128454808903)) ;
#42172=CARTESIAN_POINT('Ctrl Pts',(-18.3832618999616,2.62292537810659,-327.135213831997)) ;
#42173=CARTESIAN_POINT('Ctrl Pts',(-18.3289574902738,2.97882054939017,-327.139988317052)) ;
#42174=CARTESIAN_POINT('Ctrl Pts',(-18.1620591775996,3.89342281347032,-327.15242546214)) ;
#42175=CARTESIAN_POINT('Ctrl Pts',(-18.034028215192,4.44892790261231,-327.160149022747)) ;
#42176=CARTESIAN_POINT('Ctrl Pts',(-17.8326523521079,5.16941109731806,-327.170157496103)) ;
#42177=CARTESIAN_POINT('Ctrl Pts',(-17.7821766148177,5.34045840603847,-327.172531939782)) ;
#42178=CARTESIAN_POINT('Ctrl Pts',(-17.6902536574805,5.63619382684467,-327.176620549269)) ;
#42179=CARTESIAN_POINT('Ctrl Pts',(-17.6499325210346,5.76121839637051,-327.178343767465)) ;
#42180=CARTESIAN_POINT('Ctrl Pts',(-17.5853805816548,5.9543354302579,-327.180991748596)) ;
#42181=CARTESIAN_POINT('Ctrl Pts',(-17.5620733474982,6.02273196921081,-327.18192688721)) ;
#42182=CARTESIAN_POINT('Ctrl Pts',(-17.5181663749925,6.14915747970571,-327.183649224433)) ;
#42183=CARTESIAN_POINT('Ctrl Pts',(-17.4976761029815,6.20722336074041,-327.184437803244)) ;
#42184=CARTESIAN_POINT('Ctrl Pts',(-17.4396190547559,6.36917498239749,-327.186631602611)) ;
#42185=CARTESIAN_POINT('Ctrl Pts',(-17.4014133526989,6.47282906581619,-327.188029224547)) ;
#42186=CARTESIAN_POINT('Ctrl Pts',(-17.1330418640408,7.18138225824297,-327.197556223597)) ;
#42187=CARTESIAN_POINT('Ctrl Pts',(-16.8723068090042,7.77422948273606,-327.205409134126)) ;
#42188=CARTESIAN_POINT('Ctrl Pts',(-16.414745052828,8.68259534562688,-327.217892846295)) ;
#42189=CARTESIAN_POINT('Ctrl Pts',(-16.2385086945559,9.00789386068396,-327.222456063144)) ;
#42190=CARTESIAN_POINT('Ctrl Pts',(-15.9450883743921,9.51286031466355,-327.229758971463)) ;
#42191=CARTESIAN_POINT('Ctrl Pts',(-15.8343081786906,9.69613525615551,-327.232456441772)) ;
#42192=CARTESIAN_POINT('Ctrl Pts',(-15.6498904154397,9.98964390931654,-327.236861137074)) ;
#42193=CARTESIAN_POINT('Ctrl Pts',(-15.5781992798387,10.1010772983335,-327.238553637698)) ;
#42194=CARTESIAN_POINT('Ctrl Pts',(-15.4357616099646,10.317352218216,-327.241879561534)) ;
#42195=CARTESIAN_POINT('Ctrl Pts',(-15.3651243927596,10.422257222664,-327.243512076517)) ;
#42196=CARTESIAN_POINT('Ctrl Pts',(-15.205097691635,10.6547534424509,-327.247173904312)) ;
#42197=CARTESIAN_POINT('Ctrl Pts',(-15.1151630069123,10.78195779568,-327.24920735989)) ;
#42198=CARTESIAN_POINT('Ctrl Pts',(-14.6075830372634,11.4810490383051,-327.260548850363)) ;
#42199=CARTESIAN_POINT('Ctrl Pts',(-14.1590846361893,12.029808121566,-327.270101419741)) ;
#42200=CARTESIAN_POINT('Ctrl Pts',(-13.4883170949134,12.7608965101675,-327.283457187197)) ;
#42201=CARTESIAN_POINT('Ctrl Pts',(-13.2915129389356,12.9657572823715,-327.287271985153)) ;
#42202=CARTESIAN_POINT('Ctrl Pts',(-12.9631718759001,13.2922046179026,-327.293424182454)) ;
#42203=CARTESIAN_POINT('Ctrl Pts',(-12.8344393436325,13.4165455918345,-327.295785601942)) ;
#42204=CARTESIAN_POINT('Ctrl Pts',(-12.6451545137902,13.5941554587708,-327.299172628531)) ;
#42205=CARTESIAN_POINT('Ctrl Pts',(-12.5860213624277,13.6489216278637,-327.300218987101)) ;
#42206=CARTESIAN_POINT('Ctrl Pts',(-12.4775341519483,13.7480925256658,-327.302115759438)) ;
#42207=CARTESIAN_POINT('Ctrl Pts',(-12.4282950909574,13.7926207710403,-327.302968013255)) ;
#42208=CARTESIAN_POINT('Ctrl Pts',(-12.3059240241778,13.9020969497038,-327.305065644221)) ;
#42209=CARTESIAN_POINT('Ctrl Pts',(-12.2325155889292,13.9667329069638,-327.306306304998)) ;
#42210=CARTESIAN_POINT('Ctrl Pts',(-11.9088512763747,14.247209345247,-327.311707597338)) ;
#42211=CARTESIAN_POINT('Ctrl Pts',(-11.6533681354822,14.4569265386785,-327.315793693139)) ;
#42212=CARTESIAN_POINT('Ctrl Pts',(-11.3160158334268,14.7190913095114,-327.321045077913)) ;
#42213=CARTESIAN_POINT('Ctrl Pts',(-11.2391450643087,14.7778713471007,-327.322232242831)) ;
#42214=CARTESIAN_POINT('Ctrl Pts',(-10.7836140355556,15.1205875912917,-327.32921989856)) ;
#42215=CARTESIAN_POINT('Ctrl Pts',(-10.3946676928102,15.3905615276053,-327.334999765208)) ;
#42216=CARTESIAN_POINT('Ctrl Pts',(-9.74255522591668,15.8071961913074,-327.344589915789)) ;
#42217=CARTESIAN_POINT('Ctrl Pts',(-9.48538686340759,15.962840262847,-327.348346524811)) ;
#42218=CARTESIAN_POINT('Ctrl Pts',(-9.09725479145342,16.185053954308,-327.354004734061)) ;
#42219=CARTESIAN_POINT('Ctrl Pts',(-8.96909631280644,16.2564241915321,-327.355871064678)) ;
#42220=CARTESIAN_POINT('Ctrl Pts',(-8.73100961321056,16.3853398486178,-327.359336627715)) ;
#42221=CARTESIAN_POINT('Ctrl Pts',(-8.62132429740078,16.4433165185368,-327.360932561846)) ;
#42222=CARTESIAN_POINT('Ctrl Pts',(-8.37255369134558,16.5716364457552,-327.364551483376)) ;
#42223=CARTESIAN_POINT('Ctrl Pts',(-8.23314714668496,16.6413364176688,-327.36657898461)) ;
#42224=CARTESIAN_POINT('Ctrl Pts',(-7.77101354237626,16.8651637331876,-327.373298307512)) ;
#42225=CARTESIAN_POINT('Ctrl Pts',(-7.4447110436268,17.011721713048,-327.37804117831)) ;
#42226=CARTESIAN_POINT('Ctrl Pts',(-6.4915130660272,17.4071678944539,-327.39184386748)) ;
#42227=CARTESIAN_POINT('Ctrl Pts',(-5.85503157798774,17.63144458984,-327.401011812333)) ;
#42228=CARTESIAN_POINT('Ctrl Pts',(-5.03320326071529,17.8716098370464,-327.412392217371)) ;
#42229=CARTESIAN_POINT('Ctrl Pts',(-4.85790180804087,17.9200547838885,-327.414792555504)) ;
#42230=CARTESIAN_POINT('Ctrl Pts',(-4.60349059050028,17.9863543319882,-327.418223744202)) ;
#42231=CARTESIAN_POINT('Ctrl Pts',(-4.52493135780387,18.0062784607028,-327.419276073064)) ;
#42232=CARTESIAN_POINT('Ctrl Pts',(-4.3818718642458,18.0415657378047,-327.421177759206)) ;
#42233=CARTESIAN_POINT('Ctrl Pts',(-4.31741515098008,18.0570989285555,-327.422029034469)) ;
#42234=CARTESIAN_POINT('Ctrl Pts',(-4.15840922618506,18.094517135811,-327.424116140612)) ;
#42235=CARTESIAN_POINT('Ctrl Pts',(-4.06376897908579,18.1160067176638,-327.425347377813)) ;
#42236=CARTESIAN_POINT('Ctrl Pts',(-3.64925344153182,18.2067174105727,-327.430699812288)) ;
#42237=CARTESIAN_POINT('Ctrl Pts',(-3.32774746855397,18.2682157669594,-327.434747644332)) ;
#42238=CARTESIAN_POINT('Ctrl Pts',(-2.94221135230492,18.3314459983211,-327.439550610788)) ;
#42239=CARTESIAN_POINT('Ctrl Pts',(-2.87958670530254,18.341387636713,-327.44032914674)) ;
#42240=CARTESIAN_POINT('Ctrl Pts',(-2.32333073306962,18.4267739161208,-327.447233298347)) ;
#42241=CARTESIAN_POINT('Ctrl Pts',(-1.82689297607741,18.482595183797,-327.453323740944)) ;
#42242=CARTESIAN_POINT('Ctrl Pts',(-1.18129924394719,18.528920723854,-327.461339653355)) ;
#42243=CARTESIAN_POINT('Ctrl Pts',(-1.0336666203417,18.5377426983824,-327.463178642747)) ;
#42244=CARTESIAN_POINT('Ctrl Pts',(-0.668600962928266,18.5551830542013,
-327.467746756184)) ;
#42245=CARTESIAN_POINT('Ctrl Pts',(-0.451092023478368,18.5617445615631,
-327.47048669689)) ;
#42246=CARTESIAN_POINT('Ctrl Pts',(-0.100421704298765,18.5661555636103,
-327.474941933505)) ;
#42247=CARTESIAN_POINT('Ctrl Pts',(0.0326889975123691,18.5663983663657,
-327.476641827251)) ;
#42248=CARTESIAN_POINT('Ctrl Pts',(0.291888208747056,18.5640836707535,-327.479970235944)) ;
#42249=CARTESIAN_POINT('Ctrl Pts',(0.417970888513894,18.5616729187842,-327.481597709921)) ;
#42250=CARTESIAN_POINT('Ctrl Pts',(0.698066611530982,18.5534620337248,-327.485232405255)) ;
#42251=CARTESIAN_POINT('Ctrl Pts',(0.852051747604905,18.5470282836666,-327.487243556183)) ;
#42252=CARTESIAN_POINT('Ctrl Pts',(1.73037390432249,18.4993690987665,-327.498787336571)) ;
#42253=CARTESIAN_POINT('Ctrl Pts',(2.45188011015524,18.417630848513,-327.508579452566)) ;
#42254=CARTESIAN_POINT('Ctrl Pts',(3.43850796223524,18.246841682233,-327.522054971141)) ;
#42255=CARTESIAN_POINT('Ctrl Pts',(3.70919064984514,18.1937481957733,-327.525757320784)) ;
#42256=CARTESIAN_POINT('Ctrl Pts',(4.15022834907698,18.0969881956845,-327.53175477119)) ;
#42257=CARTESIAN_POINT('Ctrl Pts',(4.32132374179857,18.0568972530956,-327.534072555319)) ;
#42258=CARTESIAN_POINT('Ctrl Pts',(4.56953163687006,17.9950074706845,-327.537409945969)) ;
#42259=CARTESIAN_POINT('Ctrl Pts',(4.64711278089576,17.9751288194487,-327.538449501795)) ;
#42260=CARTESIAN_POINT('Ctrl Pts',(4.78886740905989,17.937827898694,-327.540340796771)) ;
#42261=CARTESIAN_POINT('Ctrl Pts',(4.85308038608426,17.9205616972291,-327.541194286532)) ;
#42262=CARTESIAN_POINT('Ctrl Pts',(5.01238333547499,17.8768077733177,-327.543304483155)) ;
#42263=CARTESIAN_POINT('Ctrl Pts',(5.1073574751163,17.8499059529265,-327.544556327861)) ;
#42264=CARTESIAN_POINT('Ctrl Pts',(5.5229852149516,17.7285889158883,-327.550015502966)) ;
#42265=CARTESIAN_POINT('Ctrl Pts',(5.84127073784943,17.6262811682561,-327.554146905572)) ;
#42266=CARTESIAN_POINT('Ctrl Pts',(6.21423960057419,17.4951837852178,-327.559005076501)) ;
#42267=CARTESIAN_POINT('Ctrl Pts',(6.2717580172002,17.4746468023733,-327.559754739108)) ;
#42268=CARTESIAN_POINT('Ctrl Pts',(6.79328737485886,17.2855278087406,-327.566559205747)) ;
#42269=CARTESIAN_POINT('Ctrl Pts',(7.2505034418735,17.0987843074423,-327.572582062372)) ;
#42270=CARTESIAN_POINT('Ctrl Pts',(7.97917523155449,16.7666803996104,-327.582500772623)) ;
#42271=CARTESIAN_POINT('Ctrl Pts',(8.25541536673911,16.6324058853837,-327.586337238701)) ;
#42272=CARTESIAN_POINT('Ctrl Pts',(8.65932541936638,16.4235311542488,-327.592088721186)) ;
#42273=CARTESIAN_POINT('Ctrl Pts',(8.7896400763428,16.3541590899349,-327.59396659497)) ;
#42274=CARTESIAN_POINT('Ctrl Pts',(9.02787781480226,16.2236648296563,-327.597442929561)) ;
#42275=CARTESIAN_POINT('Ctrl Pts',(9.1360425072938,16.1630011321562,-327.599037941398)) ;
#42276=CARTESIAN_POINT('Ctrl Pts',(9.37775044366371,16.0242387259504,-327.602640619275)) ;
#42277=CARTESIAN_POINT('Ctrl Pts',(9.51094167171217,15.9455454139893,-327.604652621432)) ;
#42278=CARTESIAN_POINT('Ctrl Pts',(9.92438533091768,15.6942473979743,-327.610982267279)) ;
#42279=CARTESIAN_POINT('Ctrl Pts',(10.2010407735134,15.5158496992859,-327.61534141355)) ;
#42280=CARTESIAN_POINT('Ctrl Pts',(10.6465809743406,15.2114793249099,-327.622547823724)) ;
#42281=CARTESIAN_POINT('Ctrl Pts',(10.8183237480652,15.0898197753552,-327.625372646545)) ;
#42282=CARTESIAN_POINT('Ctrl Pts',(11.3376586949367,14.708508028158,-327.634040386302)) ;
#42283=CARTESIAN_POINT('Ctrl Pts',(11.6782493725886,14.439570795678,-327.639904276368)) ;
#42284=CARTESIAN_POINT('Ctrl Pts',(12.1825226967449,14.0118645377211,-327.648730915036)) ;
#42285=CARTESIAN_POINT('Ctrl Pts',(12.3532230572227,13.8616047963072,-327.651744912699)) ;
#42286=CARTESIAN_POINT('Ctrl Pts',(12.5855486714897,13.6493984568164,-327.655859633654)) ;
#42287=CARTESIAN_POINT('Ctrl Pts',(12.6495613593273,13.5900960644816,-327.656994698044)) ;
#42288=CARTESIAN_POINT('Ctrl Pts',(12.7563363115265,13.4897699886671,-327.658888432341)) ;
#42289=CARTESIAN_POINT('Ctrl Pts',(12.7993244058282,13.4489890031938,-327.659650881673)) ;
#42290=CARTESIAN_POINT('Ctrl Pts',(12.9031332530454,13.3495614185935,-327.661492099007)) ;
#42291=CARTESIAN_POINT('Ctrl Pts',(12.9637502358049,13.2907041824549,-327.66256748137)) ;
#42292=CARTESIAN_POINT('Ctrl Pts',(13.1588941240561,13.0986201928476,-327.666034089572)) ;
#42293=CARTESIAN_POINT('Ctrl Pts',(13.2917855787146,12.9637487588066,-327.668402144939)) ;
#42294=CARTESIAN_POINT('Ctrl Pts',(13.9816952881079,12.2417973267069,-327.680800581413)) ;
#42295=CARTESIAN_POINT('Ctrl Pts',(14.5019485357546,11.6207960967083,-327.690558961953)) ;
#42296=CARTESIAN_POINT('Ctrl Pts',(15.1321367858446,10.7600761107374,-327.703831788143)) ;
#42297=CARTESIAN_POINT('Ctrl Pts',(15.2799114300906,10.5491756989865,-327.707061586475)) ;
#42298=CARTESIAN_POINT('Ctrl Pts',(15.5011751572282,10.2189853926499,-327.712099378994)) ;
#42299=CARTESIAN_POINT('Ctrl Pts',(15.577781184385,10.1018229548233,-327.71388329619)) ;
#42300=CARTESIAN_POINT('Ctrl Pts',(15.7202469001488,9.87845886226319,-327.717279008874)) ;
#42301=CARTESIAN_POINT('Ctrl Pts',(15.7863736765702,9.77243665554591,-327.718888627197)) ;
#42302=CARTESIAN_POINT('Ctrl Pts',(15.9365768448127,9.52610988181825,-327.722623930781)) ;
#42303=CARTESIAN_POINT('Ctrl Pts',(16.0198794350881,9.38534569325051,-327.724755266258)) ;
#42304=CARTESIAN_POINT('Ctrl Pts',(16.3262567709777,8.85166503843979,-327.732822955998)) ;
#42305=CARTESIAN_POINT('Ctrl Pts',(16.5368235853489,8.45175116541721,-327.738846542318)) ;
#42306=CARTESIAN_POINT('Ctrl Pts',(16.7506682402526,8.00695656437228,-327.745476492103)) ;
#42307=CARTESIAN_POINT('Ctrl Pts',(16.7686183518665,7.96929598443489,-327.746037275166)) ;
#42308=CARTESIAN_POINT('Ctrl Pts',(16.977320344606,7.52759762502785,-327.75260701353)) ;
#42309=CARTESIAN_POINT('Ctrl Pts',(17.1535540572944,7.1168613365757,-327.758648384927)) ;
#42310=CARTESIAN_POINT('Ctrl Pts',(17.3980817636596,6.48494469835063,-327.76769570092)) ;
#42311=CARTESIAN_POINT('Ctrl Pts',(17.4773452329137,6.26818640182485,-327.770755396221)) ;
#42312=CARTESIAN_POINT('Ctrl Pts',(17.5811133620001,5.96712970882221,-327.774920111553)) ;
#42313=CARTESIAN_POINT('Ctrl Pts',(17.6090920645608,5.88405138501024,-327.776060534989)) ;
#42314=CARTESIAN_POINT('Ctrl Pts',(17.6550017536798,5.74446918030818,-327.777959924947)) ;
#42315=CARTESIAN_POINT('Ctrl Pts',(17.6732523491538,5.68807212539553,-327.778722732515)) ;
#42316=CARTESIAN_POINT('Ctrl Pts',(17.7167530087117,5.55141791192916,-327.780559848186)) ;
#42317=CARTESIAN_POINT('Ctrl Pts',(17.7417281824127,5.47107476944672,-327.781630828508)) ;
#42318=CARTESIAN_POINT('Ctrl Pts',(17.8190216128348,5.21633203255912,-327.785001496962)) ;
#42319=CARTESIAN_POINT('Ctrl Pts',(17.869321017044,5.04133094593128,-327.787280094054)) ;
#42320=CARTESIAN_POINT('Ctrl Pts',(18.1493968771512,4.00998616637852,-327.800557620631)) ;
#42321=CARTESIAN_POINT('Ctrl Pts',(18.3201663051196,3.13880782650356,-327.811224976039)) ;
#42322=CARTESIAN_POINT('Ctrl Pts',(18.4545114030542,2.04275991416404,-327.825026810529)) ;
#42323=CARTESIAN_POINT('Ctrl Pts',(18.4771878039784,1.82630496046092,-327.827767140321)) ;
#42324=CARTESIAN_POINT('Ctrl Pts',(18.5075934141066,1.47689012193679,-327.83222284008)) ;
#42325=CARTESIAN_POINT('Ctrl Pts',(18.5177065724591,1.344158342134,-327.833922801622)) ;
#42326=CARTESIAN_POINT('Ctrl Pts',(18.5346187715303,1.08549871134924,-327.83725123519)) ;
#42327=CARTESIAN_POINT('Ctrl Pts',(18.5415639066461,0.959587567914242,-327.838878665049)) ;
#42328=CARTESIAN_POINT('Ctrl Pts',(18.5541448691738,0.679672026233069,-327.842513120881)) ;
#42329=CARTESIAN_POINT('Ctrl Pts',(18.5591470564903,0.525648485061498,-327.844524074546)) ;
#42330=CARTESIAN_POINT('Ctrl Pts',(18.5706458829459,-0.0487728198690466,
-327.852064087765)) ;
#42331=CARTESIAN_POINT('Ctrl Pts',(18.5647775975318,-0.469202087608817,
-327.857666110766)) ;
#42332=CARTESIAN_POINT('Ctrl Pts',(18.5446545920453,-0.888980013405447,
-327.863308832765)) ;
#42333=CARTESIAN_POINT('Origin',(0.,0.,-315.477129595899)) ;
#42334=CARTESIAN_POINT('',(18.5446545937453,-0.888979977940784,-329.658408769442)) ;
#42335=CARTESIAN_POINT('',(18.5446545935817,-0.888979981355556,-329.363119887734)) ;
#42336=CARTESIAN_POINT('',(18.544654593745,-0.888979977948782,-315.477129595899)) ;
#42337=CARTESIAN_POINT('Ctrl Pts',(18.5446545937457,-0.888979977932787,
-329.658408769442)) ;
#42338=CARTESIAN_POINT('Ctrl Pts',(18.5464056157976,-0.852452609550874,
-329.657945483223)) ;
#42339=CARTESIAN_POINT('Ctrl Pts',(18.548048719277,-0.81591999982208,-329.657483285843)) ;
#42340=CARTESIAN_POINT('Ctrl Pts',(18.5630941390681,-0.457833654916934,
-329.652963311734)) ;
#42341=CARTESIAN_POINT('Ctrl Pts',(18.5682412777646,-0.13598693597125,-329.648982036948)) ;
#42342=CARTESIAN_POINT('Ctrl Pts',(18.5640719297102,0.280542107439365,-329.643860347317)) ;
#42343=CARTESIAN_POINT('Ctrl Pts',(18.5623991451796,0.375244544935029,-329.642698014782)) ;
#42344=CARTESIAN_POINT('Ctrl Pts',(18.5511258441397,0.820486321522968,-329.63723744753)) ;
#42345=CARTESIAN_POINT('Ctrl Pts',(18.5323198928692,1.17072082538506,-329.632952652673)) ;
#42346=CARTESIAN_POINT('Ctrl Pts',(18.48122711744,1.79260822178519,-329.625269663356)) ;
#42347=CARTESIAN_POINT('Ctrl Pts',(18.4528354240194,2.06447680806557,-329.621885679587)) ;
#42348=CARTESIAN_POINT('Ctrl Pts',(18.3913704034129,2.5491836723963,-329.615777062905)) ;
#42349=CARTESIAN_POINT('Ctrl Pts',(18.3605761713517,2.76226087358939,-329.613065611654)) ;
#42350=CARTESIAN_POINT('Ctrl Pts',(18.3048216159088,3.10573890129734,-329.608644281449)) ;
#42351=CARTESIAN_POINT('Ctrl Pts',(18.2821560091663,3.23649194477292,-329.606949348729)) ;
#42352=CARTESIAN_POINT('Ctrl Pts',(18.2351779117158,3.49123882555864,-329.603622658193)) ;
#42353=CARTESIAN_POINT('Ctrl Pts',(18.2109975284144,3.61524978047479,-329.601991852761)) ;
#42354=CARTESIAN_POINT('Ctrl Pts',(18.1481982967582,3.92068907093482,-329.597946527125)) ;
#42355=CARTESIAN_POINT('Ctrl Pts',(18.1081227649738,4.10180374629958,-329.595522652821)) ;
#42356=CARTESIAN_POINT('Ctrl Pts',(17.9544386770753,4.75013842607234,-329.586757648808)) ;
#42357=CARTESIAN_POINT('Ctrl Pts',(17.8254049329426,5.2135036140851,-329.580322648283)) ;
#42358=CARTESIAN_POINT('Ctrl Pts',(17.5242735712885,6.15218208866002,-329.567056188216)) ;
#42359=CARTESIAN_POINT('Ctrl Pts',(17.3504621607203,6.62653542863033,-329.560226365094)) ;
#42360=CARTESIAN_POINT('Ctrl Pts',(17.0950067691068,7.24444783859639,-329.551357988226)) ;
#42361=CARTESIAN_POINT('Ctrl Pts',(17.0304862722755,7.39485080357388,-329.549202283536)) ;
#42362=CARTESIAN_POINT('Ctrl Pts',(16.9322439963063,7.6157543493639,-329.546050403293)) ;
#42363=CARTESIAN_POINT('Ctrl Pts',(16.9000521322515,7.6869264995685,-329.545037139498)) ;
#42364=CARTESIAN_POINT('Ctrl Pts',(16.8394093829016,7.81877752980614,-329.543165636627)) ;
#42365=CARTESIAN_POINT('Ctrl Pts',(16.8110773286262,7.87950946866018,-329.542306000018)) ;
#42366=CARTESIAN_POINT('Ctrl Pts',(16.7458959506702,8.01727887965723,-329.540360393077)) ;
#42367=CARTESIAN_POINT('Ctrl Pts',(16.7088426612801,8.09421823106599,-329.539276952249)) ;
#42368=CARTESIAN_POINT('Ctrl Pts',(16.5463595160849,8.42573605378673,-329.534616865767)) ;
#42369=CARTESIAN_POINT('Ctrl Pts',(16.4156321655984,8.67767610317607,-329.531096045575)) ;
#42370=CARTESIAN_POINT('Ctrl Pts',(16.0002642668367,9.43517719972528,-329.520451921263)) ;
#42371=CARTESIAN_POINT('Ctrl Pts',(15.6976608899925,9.9304818258345,-329.513402326031)) ;
#42372=CARTESIAN_POINT('Ctrl Pts',(15.2830317075343,10.5427141580516,-329.504260368031)) ;
#42373=CARTESIAN_POINT('Ctrl Pts',(15.1920033812151,10.673467720669,-329.502282615644)) ;
#42374=CARTESIAN_POINT('Ctrl Pts',(14.966220685514,10.9890421840235,-329.497439347552)) ;
#42375=CARTESIAN_POINT('Ctrl Pts',(14.8297121852846,11.17257561876,-329.49456268219)) ;
#42376=CARTESIAN_POINT('Ctrl Pts',(14.6072544258106,11.4604039708628,-329.489944638299)) ;
#42377=CARTESIAN_POINT('Ctrl Pts',(14.5234973425004,11.5663635561837,-329.488220922475)) ;
#42378=CARTESIAN_POINT('Ctrl Pts',(14.359042603586,11.769809148002,-329.484863735291)) ;
#42379=CARTESIAN_POINT('Ctrl Pts',(14.2784896241219,11.8674026590362,-329.483231523347)) ;
#42380=CARTESIAN_POINT('Ctrl Pts',(14.1001314241273,12.0790464822641,-329.479643353384)) ;
#42381=CARTESIAN_POINT('Ctrl Pts',(14.0019267739386,12.1927485263665,-329.477684121172)) ;
#42382=CARTESIAN_POINT('Ctrl Pts',(13.5549776628183,12.6977074958631,-329.468840954069)) ;
#42383=CARTESIAN_POINT('Ctrl Pts',(13.1911404705956,13.0752822146579,-329.461831737615)) ;
#42384=CARTESIAN_POINT('Ctrl Pts',(12.4461530609739,13.7856100631217,-329.447979225795)) ;
#42385=CARTESIAN_POINT('Ctrl Pts',(12.0664070907128,14.1191922952866,-329.441145797908)) ;
#42386=CARTESIAN_POINT('Ctrl Pts',(11.5461471190198,14.539870063039,-329.432271616335)) ;
#42387=CARTESIAN_POINT('Ctrl Pts',(11.4174068721334,14.6411801169166,-329.430113706025)) ;
#42388=CARTESIAN_POINT('Ctrl Pts',(11.2253013397838,14.7882796570412,-329.426959289101)) ;
#42389=CARTESIAN_POINT('Ctrl Pts',(11.162960688388,14.8353939642875,-329.425945656568)) ;
#42390=CARTESIAN_POINT('Ctrl Pts',(11.0466133096676,14.922175567033,-329.424073892906)) ;
#42391=CARTESIAN_POINT('Ctrl Pts',(10.9926858132041,14.9619466604146,-329.423214359202)) ;
#42392=CARTESIAN_POINT('Ctrl Pts',(10.8695786363941,15.0517123522689,-329.421269395023)) ;
#42393=CARTESIAN_POINT('Ctrl Pts',(10.8002670835109,15.1015236125255,-329.420186488422)) ;
#42394=CARTESIAN_POINT('Ctrl Pts',(10.4970057537607,15.3163088751214,-329.415495752473)) ;
#42395=CARTESIAN_POINT('Ctrl Pts',(10.2596010859597,15.4763378610795,-329.411944833104)) ;
#42396=CARTESIAN_POINT('Ctrl Pts',(9.53167290427586,15.9429044066923,-329.401293244489)) ;
#42397=CARTESIAN_POINT('Ctrl Pts',(9.03043783209601,16.2320726682406,-329.394264483782)) ;
#42398=CARTESIAN_POINT('Ctrl Pts',(8.3751603521555,16.5703499645443,-329.385146734879)) ;
#42399=CARTESIAN_POINT('Ctrl Pts',(8.23286420762254,16.6415070152318,-329.383171694541)) ;
#42400=CARTESIAN_POINT('Ctrl Pts',(7.88400204667147,16.8103903565124,-329.378333753632)) ;
#42401=CARTESIAN_POINT('Ctrl Pts',(7.67651260857948,16.906148766256,-329.375459708821)) ;
#42402=CARTESIAN_POINT('Ctrl Pts',(7.34368745221428,17.0523601169786,-329.370844785587)) ;
#42403=CARTESIAN_POINT('Ctrl Pts',(7.21947736706305,17.1053172270247,-329.369121525399)) ;
#42404=CARTESIAN_POINT('Ctrl Pts',(6.97774843408016,17.2052766012387,-329.36576456597)) ;
#42405=CARTESIAN_POINT('Ctrl Pts',(6.86030474969144,17.2524414162647,-329.364132118633)) ;
#42406=CARTESIAN_POINT('Ctrl Pts',(6.60233316493429,17.3529908531503,-329.360542624641)) ;
#42407=CARTESIAN_POINT('Ctrl Pts',(6.46162055661302,17.4058770093359,-329.358582293492)) ;
#42408=CARTESIAN_POINT('Ctrl Pts',(5.88015319146191,17.6163958362378,-329.350472649438)) ;
#42409=CARTESIAN_POINT('Ctrl Pts',(5.43415750933693,17.7590409006545,-329.34422669434)) ;
#42410=CARTESIAN_POINT('Ctrl Pts',(4.72798379895485,17.9558037517669,-329.334373393803)) ;
#42411=CARTESIAN_POINT('Ctrl Pts',(4.47122392841441,18.0214559813872,-329.330799308776)) ;
#42412=CARTESIAN_POINT('Ctrl Pts',(3.94290922258713,18.1445573024967,-329.323498428541)) ;
#42413=CARTESIAN_POINT('Ctrl Pts',(3.67129333729694,18.201458688249,-329.319773261476)) ;
#42414=CARTESIAN_POINT('Ctrl Pts',(3.22509943348238,18.2845384068916,-329.313744332418)) ;
#42415=CARTESIAN_POINT('Ctrl Pts',(3.05124300540132,18.3143530439589,-329.311417617706)) ;
#42416=CARTESIAN_POINT('Ctrl Pts',(2.79776490737793,18.3541123904302,-329.30807005776)) ;
#42417=CARTESIAN_POINT('Ctrl Pts',(2.71846207337928,18.3660255389394,-329.307029100146)) ;
#42418=CARTESIAN_POINT('Ctrl Pts',(2.57328881674885,18.3868731004828,-329.305136687279)) ;
#42419=CARTESIAN_POINT('Ctrl Pts',(2.507443016451,18.3959682338385,-329.304283462929)) ;
#42420=CARTESIAN_POINT('Ctrl Pts',(2.34388534797976,18.417665624753,-329.302175906683)) ;
#42421=CARTESIAN_POINT('Ctrl Pts',(2.24611929529175,18.4298441051964,-329.300926406365)) ;
#42422=CARTESIAN_POINT('Ctrl Pts',(1.80395475097615,18.4813528207075,-329.295313348593)) ;
#42423=CARTESIAN_POINT('Ctrl Pts',(1.45859197412777,18.5118115108392,-329.291032032854)) ;
#42424=CARTESIAN_POINT('Ctrl Pts',(0.70047964845604,18.5573237698163,-329.281703112689)) ;
#42425=CARTESIAN_POINT('Ctrl Pts',(0.287669937373465,18.568311270573,-329.276666901431)) ;
#42426=CARTESIAN_POINT('Ctrl Pts',(-0.401620203831488,18.5636643251038,
-329.26818172439)) ;
#42427=CARTESIAN_POINT('Ctrl Pts',(-0.678001836750486,18.5556257005605,
-329.264759766599)) ;
#42428=CARTESIAN_POINT('Ctrl Pts',(-1.17076365192046,18.5302692686968,-329.258592146341)) ;
#42429=CARTESIAN_POINT('Ctrl Pts',(-1.38721458448472,18.5153234418784,-329.255860093777)) ;
#42430=CARTESIAN_POINT('Ctrl Pts',(-1.73585090042897,18.485102340234,-329.251414246141)) ;
#42431=CARTESIAN_POINT('Ctrl Pts',(-1.86822093544779,18.4721936258859,-329.249715726479)) ;
#42432=CARTESIAN_POINT('Ctrl Pts',(-2.12587391853036,18.4442695105792,-329.246387813588)) ;
#42433=CARTESIAN_POINT('Ctrl Pts',(-2.25116517340885,18.429396978869,-329.244759436983)) ;
#42434=CARTESIAN_POINT('Ctrl Pts',(-2.55914005515718,18.3896517289511,-329.240731392047)) ;
#42435=CARTESIAN_POINT('Ctrl Pts',(-2.74162325887527,18.3633327660953,-329.238322556326)) ;
#42436=CARTESIAN_POINT('Ctrl Pts',(-3.55913171485046,18.2329685694546,-329.227434458451)) ;
#42437=CARTESIAN_POINT('Ctrl Pts',(-4.18887996161352,18.0986695754916,-329.218767089537)) ;
#42438=CARTESIAN_POINT('Ctrl Pts',(-5.10880081888335,17.851893967093,-329.205939961591)) ;
#42439=CARTESIAN_POINT('Ctrl Pts',(-5.40517869083605,17.7644028235072,-329.201784448889)) ;
#42440=CARTESIAN_POINT('Ctrl Pts',(-5.87852276361185,17.6117278472674,-329.195169087521)) ;
#42441=CARTESIAN_POINT('Ctrl Pts',(-6.05692033955571,17.5511738601811,-329.19268103426)) ;
#42442=CARTESIAN_POINT('Ctrl Pts',(-6.31163349007251,17.4603697318797,-329.18915068319)) ;
#42443=CARTESIAN_POINT('Ctrl Pts',(-6.38871801374282,17.4323122577922,-329.18808522974)) ;
#42444=CARTESIAN_POINT('Ctrl Pts',(-6.52761399040505,17.3807114214591,-329.186172416622)) ;
#42445=CARTESIAN_POINT('Ctrl Pts',(-6.58949019849059,17.3573469414404,-329.18532296933)) ;
#42446=CARTESIAN_POINT('Ctrl Pts',(-6.7403769903966,17.2994489114451,-329.183257475283)) ;
#42447=CARTESIAN_POINT('Ctrl Pts',(-6.82924856698833,17.2645584554089,-329.182045768209)) ;
#42448=CARTESIAN_POINT('Ctrl Pts',(-7.1986597147558,17.1162310874814,-329.177022338809)) ;
#42449=CARTESIAN_POINT('Ctrl Pts',(-7.47667439477461,16.9966293456523,-329.173273115701)) ;
#42450=CARTESIAN_POINT('Ctrl Pts',(-7.86038173036401,16.8203216160385,-329.168075559127)) ;
#42451=CARTESIAN_POINT('Ctrl Pts',(-7.96863608411152,16.7693070575595,-329.166606680282)) ;
#42452=CARTESIAN_POINT('Ctrl Pts',(-8.3931139416433,16.5642345309535,-329.16082698426)) ;
#42453=CARTESIAN_POINT('Ctrl Pts',(-8.70542577721187,16.4022495177638,-329.156528976738)) ;
#42454=CARTESIAN_POINT('Ctrl Pts',(-9.25116814710385,16.0992122255411,-329.148842393761)) ;
#42455=CARTESIAN_POINT('Ctrl Pts',(-9.48644819297611,15.9617056333788,-329.145468430242)) ;
#42456=CARTESIAN_POINT('Ctrl Pts',(-9.90166242926357,15.7066143058814,-329.13937540489)) ;
#42457=CARTESIAN_POINT('Ctrl Pts',(-10.0827427968709,15.5909893617076,-329.136669412829)) ;
#42458=CARTESIAN_POINT('Ctrl Pts',(-10.372297608971,15.3989457461736,-329.132254578447)) ;
#42459=CARTESIAN_POINT('Ctrl Pts',(-10.4820310121135,15.3244612819719,-329.130560595582)) ;
#42460=CARTESIAN_POINT('Ctrl Pts',(-10.6947658527859,15.1767077278296,-329.12723421047)) ;
#42461=CARTESIAN_POINT('Ctrl Pts',(-10.7978358104002,15.103549776777,-329.125602743423)) ;
#42462=CARTESIAN_POINT('Ctrl Pts',(-11.0259778671037,14.9380879582892,-329.12194652051)) ;
#42463=CARTESIAN_POINT('Ctrl Pts',(-11.1506539870435,14.8452543036172,-329.119917665964)) ;
#42464=CARTESIAN_POINT('Ctrl Pts',(-11.8386155483028,14.3194423654408,-329.108551088841)) ;
#42465=CARTESIAN_POINT('Ctrl Pts',(-12.3778508949711,13.8559751316625,-329.098966796857)) ;
#42466=CARTESIAN_POINT('Ctrl Pts',(-13.0929840002629,13.1661854156127,-329.085592315766)) ;
#42467=CARTESIAN_POINT('Ctrl Pts',(-13.2922505309425,12.9649814718804,-329.081789784805)) ;
#42468=CARTESIAN_POINT('Ctrl Pts',(-13.6095902916943,12.629546918324,-329.075654422096)) ;
#42469=CARTESIAN_POINT('Ctrl Pts',(-13.7304644292381,12.4980298455889,-329.073297717164)) ;
#42470=CARTESIAN_POINT('Ctrl Pts',(-13.9030628198843,12.3047076648567,-329.069916047151)) ;
#42471=CARTESIAN_POINT('Ctrl Pts',(-13.9563120411438,12.2442778768537,-329.068870417922)) ;
#42472=CARTESIAN_POINT('Ctrl Pts',(-14.0527384690571,12.133402226157,-329.066974238976)) ;
#42473=CARTESIAN_POINT('Ctrl Pts',(-14.0960413757827,12.083067722556,-329.066121858766)) ;
#42474=CARTESIAN_POINT('Ctrl Pts',(-14.2025233464681,11.9579435874088,-329.064022909729)) ;
#42475=CARTESIAN_POINT('Ctrl Pts',(-14.2653826326845,11.882884440652,-329.062781072598)) ;
#42476=CARTESIAN_POINT('Ctrl Pts',(-14.5322876758576,11.559007637291,-329.057488347771)) ;
#42477=CARTESIAN_POINT('Ctrl Pts',(-14.7304400882219,11.305404830605,-329.053507742861)) ;
#42478=CARTESIAN_POINT('Ctrl Pts',(-14.9781817664607,10.9707573718264,-329.048388273981)) ;
#42479=CARTESIAN_POINT('Ctrl Pts',(-15.0338802013486,10.8943055051733,-329.047227507275)) ;
#42480=CARTESIAN_POINT('Ctrl Pts',(-15.2932833251524,10.5324699147148,-329.041769034841)) ;
#42481=CARTESIAN_POINT('Ctrl Pts',(-15.4894613038502,10.2417784519133,-329.037484771849)) ;
#42482=CARTESIAN_POINT('Ctrl Pts',(-15.8237208744952,9.71488938933557,-329.02980192998)) ;
#42483=CARTESIAN_POINT('Ctrl Pts',(-15.9650364158651,9.48086652552187,-329.026417545776)) ;
#42484=CARTESIAN_POINT('Ctrl Pts',(-16.2083253132601,9.05709892187497,-329.020308306214)) ;
#42485=CARTESIAN_POINT('Ctrl Pts',(-16.3122615459554,8.86853840066222,-329.017596637)) ;
#42486=CARTESIAN_POINT('Ctrl Pts',(-16.4749233654184,8.56090003707979,-329.013175047433)) ;
#42487=CARTESIAN_POINT('Ctrl Pts',(-16.5356923678803,8.44292527474377,-329.011480076782)) ;
#42488=CARTESIAN_POINT('Ctrl Pts',(-16.6518382379373,8.2113789844864,-329.008153373888)) ;
#42489=CARTESIAN_POINT('Ctrl Pts',(-16.7073309067011,8.09787351404136,-329.006522594713)) ;
#42490=CARTESIAN_POINT('Ctrl Pts',(-16.8414186598449,7.81636214904177,-329.002477455215)) ;
#42491=CARTESIAN_POINT('Ctrl Pts',(-16.9186628695807,7.64772817650856,-329.000053742808)) ;
#42492=CARTESIAN_POINT('Ctrl Pts',(-17.1870954909235,7.03772613870586,-328.991286762151)) ;
#42493=CARTESIAN_POINT('Ctrl Pts',(-17.3636423636545,6.59012611138508,-328.984849540912)) ;
#42494=CARTESIAN_POINT('Ctrl Pts',(-17.6894863660748,5.65963865569467,-328.971581794006)) ;
#42495=CARTESIAN_POINT('Ctrl Pts',(-17.8368548722474,5.17648975658616,-328.964752948045)) ;
#42496=CARTESIAN_POINT('Ctrl Pts',(-18.0056575068686,4.52963178282796,-328.955886144614)) ;
#42497=CARTESIAN_POINT('Ctrl Pts',(-18.0448740885557,4.37078775806497,-328.953731037755)) ;
#42498=CARTESIAN_POINT('Ctrl Pts',(-18.0997033642613,4.13537640533821,-328.950579845134)) ;
#42499=CARTESIAN_POINT('Ctrl Pts',(-18.1169404239192,4.0591956822157,-328.949566681338)) ;
#42500=CARTESIAN_POINT('Ctrl Pts',(-18.1480733524763,3.91745125482738,-328.947695249101)) ;
#42501=CARTESIAN_POINT('Ctrl Pts',(-18.1620958938704,3.85191685695051,-328.946835584497)) ;
#42502=CARTESIAN_POINT('Ctrl Pts',(-18.1931811372667,3.70269549523105,-328.944889802918)) ;
#42503=CARTESIAN_POINT('Ctrl Pts',(-18.2100218289735,3.61896377970072,-328.943806216979)) ;
#42504=CARTESIAN_POINT('Ctrl Pts',(-18.2802550542846,3.25685693041649,-328.939150435351)) ;
#42505=CARTESIAN_POINT('Ctrl Pts',(-18.3278466238248,2.97739495370585,-328.935633908894)) ;
#42506=CARTESIAN_POINT('Ctrl Pts',(-18.4533248128601,2.12275947188802,-328.924990978)) ;
#42507=CARTESIAN_POINT('Ctrl Pts',(-18.5106590836004,1.54492913503653,-328.91793853273)) ;
#42508=CARTESIAN_POINT('Ctrl Pts',(-18.549120541585,0.806236216037114,-328.908793263879)) ;
#42509=CARTESIAN_POINT('Ctrl Pts',(-18.555356898997,0.64700848545377,-328.906815141501)) ;
#42510=CARTESIAN_POINT('Ctrl Pts',(-18.5655517874979,0.259055709987912,
-328.901971146802)) ;
#42511=CARTESIAN_POINT('Ctrl Pts',(-18.5673343449506,0.0302998911234719,
-328.899094124089)) ;
#42512=CARTESIAN_POINT('Ctrl Pts',(-18.5634460026754,-0.333489004622157,
-328.894475654654)) ;
#42513=CARTESIAN_POINT('Ctrl Pts',(-18.5605286509434,-0.468528060685627,
-328.892751876703)) ;
#42514=CARTESIAN_POINT('Ctrl Pts',(-18.5520246752332,-0.72999434392318,
-328.88939465837)) ;
#42515=CARTESIAN_POINT('Ctrl Pts',(-18.5466184483464,-0.856420089644797,
-328.887762478429)) ;
#42516=CARTESIAN_POINT('Ctrl Pts',(-18.5319681614582,-1.13279424658688,
-328.884174488593)) ;
#42517=CARTESIAN_POINT('Ctrl Pts',(-18.5221956767152,-1.28270572131308,
-328.882215405908)) ;
#42518=CARTESIAN_POINT('Ctrl Pts',(-18.4701576356817,-1.95514396538228,
-328.873370955207)) ;
#42519=CARTESIAN_POINT('Ctrl Pts',(-18.4075919403145,-2.47585677836037,
-328.866360241071)) ;
#42520=CARTESIAN_POINT('Ctrl Pts',(-18.2416270395859,-3.49181508586461,
-328.852506770226)) ;
#42521=CARTESIAN_POINT('Ctrl Pts',(-18.1398605465809,-3.9868771384187,-328.845673908469)) ;
#42522=CARTESIAN_POINT('Ctrl Pts',(-17.9785332538672,-4.63612643559636,
-328.836800638558)) ;
#42523=CARTESIAN_POINT('Ctrl Pts',(-17.9369337740724,-4.79455245330044,
-328.834643074665)) ;
#42524=CARTESIAN_POINT('Ctrl Pts',(-17.8724007767717,-5.0277127184577,-328.831489056131)) ;
#42525=CARTESIAN_POINT('Ctrl Pts',(-17.8510829284046,-5.10288575321948,
-328.830475481492)) ;
#42526=CARTESIAN_POINT('Ctrl Pts',(-17.8106031098457,-5.24227110247202,
-328.828603758811)) ;
#42527=CARTESIAN_POINT('Ctrl Pts',(-17.7915668699794,-5.30651842072874,
-328.827744208984)) ;
#42528=CARTESIAN_POINT('Ctrl Pts',(-17.7474909134409,-5.45237121802005,
-328.825799144012)) ;
#42529=CARTESIAN_POINT('Ctrl Pts',(-17.7222353661028,-5.53390994477335,
-328.824716153623)) ;
#42530=CARTESIAN_POINT('Ctrl Pts',(-17.6094535757236,-5.88933954250445,
-328.820009324466)) ;
#42531=CARTESIAN_POINT('Ctrl Pts',(-17.5161334821473,-6.16135082649842,
-328.81644294422)) ;
#42532=CARTESIAN_POINT('Ctrl Pts',(-17.2165290404984,-6.97273345663403,
-328.805788189731)) ;
#42533=CARTESIAN_POINT('Ctrl Pts',(-16.9913657990118,-7.5047567311333,-328.798770765493)) ;
#42534=CARTESIAN_POINT('Ctrl Pts',(-16.6730612774619,-8.16876965722278,
-328.789666193618)) ;
#42535=CARTESIAN_POINT('Ctrl Pts',(-16.6025068884232,-8.31122945310268,
-328.787692634373)) ;
#42536=CARTESIAN_POINT('Ctrl Pts',(-16.426152040784,-8.65610698255043,-328.78285760357)) ;
#42537=CARTESIAN_POINT('Ctrl Pts',(-16.3184293129125,-8.85751226058293,
-328.779984990748)) ;
#42538=CARTESIAN_POINT('Ctrl Pts',(-16.1411606873682,-9.17472926637017,
-328.775371772794)) ;
#42539=CARTESIAN_POINT('Ctrl Pts',(-16.0740194161147,-9.29185800541385,
-328.773648761616)) ;
#42540=CARTESIAN_POINT('Ctrl Pts',(-15.9414694901437,-9.51735619637811,
-328.770291926144)) ;
#42541=CARTESIAN_POINT('Ctrl Pts',(-15.8762182696884,-9.62580967363088,
-328.768659349646)) ;
#42542=CARTESIAN_POINT('Ctrl Pts',(-15.7310325555191,-9.86162882263915,
-328.765069129831)) ;
#42543=CARTESIAN_POINT('Ctrl Pts',(-15.6506493638892,-9.98870775917945,
-328.763108196374)) ;
#42544=CARTESIAN_POINT('Ctrl Pts',(-15.3136145829547,-10.5074729380746,
-328.754995433068)) ;
#42545=CARTESIAN_POINT('Ctrl Pts',(-15.0437335571463,-10.8903561710446,
-328.748746886634)) ;
#42546=CARTESIAN_POINT('Ctrl Pts',(-14.5991096858575,-11.4730356627758,
-328.738895259044)) ;
#42547=CARTESIAN_POINT('Ctrl Pts',(-14.4340709491049,-11.6799891570014,
-328.735325465672)) ;
#42548=CARTESIAN_POINT('Ctrl Pts',(-14.0870600507345,-12.0965380945556,
-328.728028813372)) ;
#42549=CARTESIAN_POINT('Ctrl Pts',(-13.9046982746158,-12.3057247224738,
-328.724303599432)) ;
#42550=CARTESIAN_POINT('Ctrl Pts',(-13.5988577892126,-12.6410710945822,
-328.718274605746)) ;
#42551=CARTESIAN_POINT('Ctrl Pts',(-13.4781475948639,-12.7696965190413,
-328.715947872727)) ;
#42552=CARTESIAN_POINT('Ctrl Pts',(-13.2999185419667,-12.9542694479112,
-328.712600291941)) ;
#42553=CARTESIAN_POINT('Ctrl Pts',(-13.2438410796647,-13.0115949688152,
-328.711559331459)) ;
#42554=CARTESIAN_POINT('Ctrl Pts',(-13.1406053442828,-13.1157694752277,
-328.709666916299)) ;
#42555=CARTESIAN_POINT('Ctrl Pts',(-13.0935636344892,-13.1627318245329,
-328.708813692487)) ;
#42556=CARTESIAN_POINT('Ctrl Pts',(-12.9761752210364,-13.2786701949695,
-328.706706141617)) ;
#42557=CARTESIAN_POINT('Ctrl Pts',(-12.9055297468071,-13.347340840367,-328.705456646075)) ;
#42558=CARTESIAN_POINT('Ctrl Pts',(-12.5857859767026,-13.6532345523095,
-328.699877049147)) ;
#42559=CARTESIAN_POINT('Ctrl Pts',(-12.3306698682767,-13.8840701561186,
-328.695627838695)) ;
#42560=CARTESIAN_POINT('Ctrl Pts',(-11.7555642434101,-14.3760796811826,
-328.686330342133)) ;
#42561=CARTESIAN_POINT('Ctrl Pts',(-11.4329749027445,-14.6339346302631,
-328.681293973119)) ;
#42562=CARTESIAN_POINT('Ctrl Pts',(-10.8794061765004,-15.0469328399117,
-328.67279305177)) ;
#42563=CARTESIAN_POINT('Ctrl Pts',(-10.6530545787562,-15.2080273029687,
-328.669355118658)) ;
#42564=CARTESIAN_POINT('Ctrl Pts',(-10.2430598536589,-15.4861743613712,
-328.663162715513)) ;
#42565=CARTESIAN_POINT('Ctrl Pts',(-10.0608111167187,-15.6051898722756,
-328.660422037533)) ;
#42566=CARTESIAN_POINT('Ctrl Pts',(-9.76379299575491,-15.7917879317515,
-328.655965923129)) ;
#42567=CARTESIAN_POINT('Ctrl Pts',(-9.65031544826297,-15.8613880676517,
-328.654265900731)) ;
#42568=CARTESIAN_POINT('Ctrl Pts',(-9.42790727304879,-15.9945291958675,
-328.650937444367)) ;
#42569=CARTESIAN_POINT('Ctrl Pts',(-9.31905829555421,-16.0581926809078,
-328.649310053635)) ;
#42570=CARTESIAN_POINT('Ctrl Pts',(-9.07577720059422,-16.1971759899021,
-328.645675811051)) ;
#42571=CARTESIAN_POINT('Ctrl Pts',(-8.94103888968603,-16.2719410434213,
-328.643665033185)) ;
#42572=CARTESIAN_POINT('Ctrl Pts',(-8.16624016252996,-16.6893404449532,
-328.632115243328)) ;
#42573=CARTESIAN_POINT('Ctrl Pts',(-7.50745051015065,-16.99587423295,-328.62231632661)) ;
#42574=CARTESIAN_POINT('Ctrl Pts',(-6.57620695891841,-17.3644442820637,
-328.608837855675)) ;
#42575=CARTESIAN_POINT('Ctrl Pts',(-6.31777513304963,-17.4601300357293,
-328.605139102085)) ;
#42576=CARTESIAN_POINT('Ctrl Pts',(-5.89130357674038,-17.607324679776,-328.599146616342)) ;
#42577=CARTESIAN_POINT('Ctrl Pts',(-5.72449280064397,-17.6622626685687,
-328.596830243184)) ;
#42578=CARTESIAN_POINT('Ctrl Pts',(-5.48052838521918,-17.7387913681375,
-328.593494459601)) ;
#42579=CARTESIAN_POINT('Ctrl Pts',(-5.40397488888692,-17.762262412417,-328.592455125585)) ;
#42580=CARTESIAN_POINT('Ctrl Pts',(-5.26357100298485,-17.8043180596652,
-328.590564006756)) ;
#42581=CARTESIAN_POINT('Ctrl Pts',(-5.19976818953087,-17.8230561925155,
-328.589710474263)) ;
#42582=CARTESIAN_POINT('Ctrl Pts',(-5.04098000197888,-17.8687651904691,
-328.587599856457)) ;
#42583=CARTESIAN_POINT('Ctrl Pts',(-4.9458775032724,-17.895321862883,-328.586347638173)) ;
#42584=CARTESIAN_POINT('Ctrl Pts',(-4.52888527505385,-18.0081858549682,
-328.580900799466)) ;
#42585=CARTESIAN_POINT('Ctrl Pts',(-4.20491615651792,-18.0865762584199,
-328.576781596143)) ;
#42586=CARTESIAN_POINT('Ctrl Pts',(-3.35359937336498,-18.2684572519014,
-328.566083595378)) ;
#42587=CARTESIAN_POINT('Ctrl Pts',(-2.82356143339785,-18.3578501042474,
-328.559542363239)) ;
#42588=CARTESIAN_POINT('Ctrl Pts',(-2.13801239771499,-18.4430740797816,
-328.550994189361)) ;
#42589=CARTESIAN_POINT('Ctrl Pts',(-1.98540137606864,-18.4601262139273,
-328.549086367512)) ;
#42590=CARTESIAN_POINT('Ctrl Pts',(-1.61052370376827,-18.497311003647,-328.544381103787)) ;
#42591=CARTESIAN_POINT('Ctrl Pts',(-1.38807211177403,-18.515333011359,-328.541572665903)) ;
#42592=CARTESIAN_POINT('Ctrl Pts',(-1.03152679946578,-18.5377569132546,
-328.537035873159)) ;
#42593=CARTESIAN_POINT('Ctrl Pts',(-0.897616386720214,-18.5447233377103,
-328.53532403784)) ;
#42594=CARTESIAN_POINT('Ctrl Pts',(-0.638166876905006,-18.5554038820657,
-328.53199071814)) ;
#42595=CARTESIAN_POINT('Ctrl Pts',(-0.512642296336732,-18.5592959999148,
-328.530370480575)) ;
#42596=CARTESIAN_POINT('Ctrl Pts',(-0.206612362929484,-18.5656779127097,
-328.52640140547)) ;
#42597=CARTESIAN_POINT('Ctrl Pts',(-0.0260916677088571,-18.5668092061987,
-328.524044032784)) ;
#42598=CARTESIAN_POINT('Ctrl Pts',(0.546633240945437,-18.562045578941,-328.516515573085)) ;
#42599=CARTESIAN_POINT('Ctrl Pts',(0.938647088542706,-18.5463550145626,
-328.5112870223)) ;
#42600=CARTESIAN_POINT('Ctrl Pts',(1.42083879473946,-18.511726954916,-328.504797286631)) ;
#42601=CARTESIAN_POINT('Ctrl Pts',(1.51176001042452,-18.5045237549564,-328.503571157027)) ;
#42602=CARTESIAN_POINT('Ctrl Pts',(2.02827754624916,-18.4597705925993,-328.496595098937)) ;
#42603=CARTESIAN_POINT('Ctrl Pts',(2.45253075023639,-18.4082083095043,-328.490821385096)) ;
#42604=CARTESIAN_POINT('Ctrl Pts',(3.09753698460728,-18.307120845082,-328.482107449655)) ;
#42605=CARTESIAN_POINT('Ctrl Pts',(3.31979263256119,-18.2681248689671,-328.479117246763)) ;
#42606=CARTESIAN_POINT('Ctrl Pts',(3.62673095271924,-18.2084842618855,-328.475028604905)) ;
#42607=CARTESIAN_POINT('Ctrl Pts',(3.71206171352296,-18.1912801743966,-328.473896372299)) ;
#42608=CARTESIAN_POINT('Ctrl Pts',(3.85525920304587,-18.1613596856957,-328.472005614508)) ;
#42609=CARTESIAN_POINT('Ctrl Pts',(3.91319157136291,-18.1489652844169,-328.471243342477)) ;
#42610=CARTESIAN_POINT('Ctrl Pts',(4.05378445159341,-18.1181815250775,-328.469399898643)) ;
#42611=CARTESIAN_POINT('Ctrl Pts',(4.13638026507514,-18.0995035425218,-328.468322143613)) ;
#42612=CARTESIAN_POINT('Ctrl Pts',(4.40666692614469,-18.0364348928172,-328.464808567297)) ;
#42613=CARTESIAN_POINT('Ctrl Pts',(4.59379440455133,-17.9896845511195,-328.462396952489)) ;
#42614=CARTESIAN_POINT('Ctrl Pts',(5.55815924320325,-17.7327274188438,-328.450009668671)) ;
#42615=CARTESIAN_POINT('Ctrl Pts',(6.32185088266296,-17.4750383503712,-328.440298918956)) ;
#42616=CARTESIAN_POINT('Ctrl Pts',(7.30456042364226,-17.0705660517323,-328.42707676386)) ;
#42617=CARTESIAN_POINT('Ctrl Pts',(7.5406545988373,-16.9675972416591,-328.423846330296)) ;
#42618=CARTESIAN_POINT('Ctrl Pts',(7.90165322635368,-16.8011300932219,-328.418807784695)) ;
#42619=CARTESIAN_POINT('Ctrl Pts',(8.02810946329015,-16.7410738751505,-328.417023761954)) ;
#42620=CARTESIAN_POINT('Ctrl Pts',(8.26612797264323,-16.6247177409206,-328.413627969681)) ;
#42621=CARTESIAN_POINT('Ctrl Pts',(8.37782473529209,-16.5687103987615,-328.41201837882)) ;
#42622=CARTESIAN_POINT('Ctrl Pts',(8.63439394422414,-16.4368028183087,-328.408283318582)) ;
#42623=CARTESIAN_POINT('Ctrl Pts',(8.77884580640209,-16.3601073304837,-328.406152201459)) ;
#42624=CARTESIAN_POINT('Ctrl Pts',(9.31834730278332,-16.0644606446752,-328.398086808872)) ;
#42625=CARTESIAN_POINT('Ctrl Pts',(9.70637582814352,-15.8330274582888,-328.392065368304)) ;
#42626=CARTESIAN_POINT('Ctrl Pts',(10.4874606551575,-15.3276480093299,-328.37956772038)) ;
#42627=CARTESIAN_POINT('Ctrl Pts',(10.8791377499119,-15.052175458738,-328.373090201535)) ;
#42628=CARTESIAN_POINT('Ctrl Pts',(11.4494675720051,-14.6171521429595,-328.363506708102)) ;
#42629=CARTESIAN_POINT('Ctrl Pts',(11.6363972174771,-14.4687837996989,-328.360340819286)) ;
#42630=CARTESIAN_POINT('Ctrl Pts',(11.8887125632867,-14.2604648310821,-328.356060377687)) ;
#42631=CARTESIAN_POINT('Ctrl Pts',(11.9566057895535,-14.2035883365874,-328.354907897514)) ;
#42632=CARTESIAN_POINT('Ctrl Pts',(12.0741854825223,-14.1036472968745,-328.352912770747)) ;
#42633=CARTESIAN_POINT('Ctrl Pts',(12.124054816179,-14.0608007229688,-328.35206695204)) ;
#42634=CARTESIAN_POINT('Ctrl Pts',(12.2386179580455,-13.9613080939858,-328.350124700544)) ;
#42635=CARTESIAN_POINT('Ctrl Pts',(12.3031477988333,-13.9044758076888,-328.349031065243)) ;
#42636=CARTESIAN_POINT('Ctrl Pts',(12.5170677159015,-13.7134185429096,-328.345402700363)) ;
#42637=CARTESIAN_POINT('Ctrl Pts',(12.6646746446081,-13.5772180047355,-328.342894194451)) ;
#42638=CARTESIAN_POINT('Ctrl Pts',(13.0723537452098,-13.188608507693,-328.335910739251)) ;
#42639=CARTESIAN_POINT('Ctrl Pts',(13.3272877573692,-12.9309407435477,-328.331477571104)) ;
#42640=CARTESIAN_POINT('Ctrl Pts',(13.6716924255063,-12.5618316713683,-328.325294185121)) ;
#42641=CARTESIAN_POINT('Ctrl Pts',(13.7676658131387,-12.4565712281782,-328.323549083842)) ;
#42642=CARTESIAN_POINT('Ctrl Pts',(14.1714561070906,-12.0033395108717,-328.316097143368)) ;
#42643=CARTESIAN_POINT('Ctrl Pts',(14.4673645688335,-11.6449855591653,-328.31035414592)) ;
#42644=CARTESIAN_POINT('Ctrl Pts',(14.8405968572803,-11.1567769770391,-328.302612721226)) ;
#42645=CARTESIAN_POINT('Ctrl Pts',(14.930227647745,-11.0365433854141,-328.300712988741)) ;
#42646=CARTESIAN_POINT('Ctrl Pts',(15.0927541056352,-10.8129214907698,-328.297189505664)) ;
#42647=CARTESIAN_POINT('Ctrl Pts',(15.1660687413496,-10.7098485767933,-328.29556921202)) ;
#42648=CARTESIAN_POINT('Ctrl Pts',(15.3155519383036,-10.495077127003,-328.292199800722)) ;
#42649=CARTESIAN_POINT('Ctrl Pts',(15.3915652597502,-10.3832795332514,-328.290449586867)) ;
#42650=CARTESIAN_POINT('Ctrl Pts',(15.5932737224311,-10.0795314522182,-328.285703892322)) ;
#42651=CARTESIAN_POINT('Ctrl Pts',(15.7166426708738,-9.88606506816518,-328.282691132402)) ;
#42652=CARTESIAN_POINT('Ctrl Pts',(15.91994059827,-9.55382711934579,-328.277537781082)) ;
#42653=CARTESIAN_POINT('Ctrl Pts',(16.0017178072763,-9.41621730906551,-328.27540918009)) ;
#42654=CARTESIAN_POINT('Ctrl Pts',(16.374593806261,-8.7698752602981,-328.265446911579)) ;
#42655=CARTESIAN_POINT('Ctrl Pts',(16.6432759292471,-8.24859979153521,-328.257502542392)) ;
#42656=CARTESIAN_POINT('Ctrl Pts',(16.9967428638843,-7.47496883062772,-328.246107920495)) ;
#42657=CARTESIAN_POINT('Ctrl Pts',(17.1014849951204,-7.23212544342308,-328.24258742481)) ;
#42658=CARTESIAN_POINT('Ctrl Pts',(17.2385552231785,-6.89468411734399,-328.237808681688)) ;
#42659=CARTESIAN_POINT('Ctrl Pts',(17.2753603700098,-6.80193938442706,-328.23650690668)) ;
#42660=CARTESIAN_POINT('Ctrl Pts',(17.3354922338592,-6.64677723454865,-328.234351092859)) ;
#42661=CARTESIAN_POINT('Ctrl Pts',(17.3592337645261,-6.58452289402169,-328.233492080366)) ;
#42662=CARTESIAN_POINT('Ctrl Pts',(17.4105707678609,-6.44770087281997,-328.231617795872)) ;
#42663=CARTESIAN_POINT('Ctrl Pts',(17.4380233350864,-6.37308113836966,-328.230604211704)) ;
#42664=CARTESIAN_POINT('Ctrl Pts',(17.5233819428517,-6.13638381895745,-328.227413109422)) ;
#42665=CARTESIAN_POINT('Ctrl Pts',(17.5795141043454,-5.97367601426046,-328.2252549615)) ;
#42666=CARTESIAN_POINT('Ctrl Pts',(17.7955709324368,-5.31796640424708,-328.216661298885)) ;
#42667=CARTESIAN_POINT('Ctrl Pts',(17.9370832417971,-4.81914500214567,-328.210350747289)) ;
#42668=CARTESIAN_POINT('Ctrl Pts',(18.0812017706597,-4.21604149813619,-328.202745004273)) ;
#42669=CARTESIAN_POINT('Ctrl Pts',(18.1040479370264,-4.11683272308126,-328.201494912535)) ;
#42670=CARTESIAN_POINT('Ctrl Pts',(18.1918934735261,-3.72048715949355,-328.196500223587)) ;
#42671=CARTESIAN_POINT('Ctrl Pts',(18.2504025878971,-3.42196110445181,-328.19273633045)) ;
#42672=CARTESIAN_POINT('Ctrl Pts',(18.3367832991858,-2.91560824751373,-328.18630929247)) ;
#42673=CARTESIAN_POINT('Ctrl Pts',(18.3685167968437,-2.70850211029244,-328.183668784849)) ;
#42674=CARTESIAN_POINT('Ctrl Pts',(18.4144768576802,-2.37041822269271,-328.179331821818)) ;
#42675=CARTESIAN_POINT('Ctrl Pts',(18.4308266120378,-2.23974793885727,-328.177649199558)) ;
#42676=CARTESIAN_POINT('Ctrl Pts',(18.460382338211,-1.98123652937086,-328.174306576125)) ;
#42677=CARTESIAN_POINT('Ctrl Pts',(18.4736538075379,-1.85341015449862,-328.172647099705)) ;
#42678=CARTESIAN_POINT('Ctrl Pts',(18.503350011706,-1.53526125336713,-328.168499772076)) ;
#42679=CARTESIAN_POINT('Ctrl Pts',(18.5181665293139,-1.34480369755538,-328.166001802841)) ;
#42680=CARTESIAN_POINT('Ctrl Pts',(18.5355446920298,-1.06579525390036,-328.162321368704)) ;
#42681=CARTESIAN_POINT('Ctrl Pts',(18.54041586422,-0.977402413736633,-328.161152304525)) ;
#42682=CARTESIAN_POINT('Ctrl Pts',(18.5446545937776,-0.888979977268102,
-328.159979993775)) ;
#42683=CARTESIAN_POINT('Ctrl Pts',(18.5446545920453,-0.888980013405418,
-327.863308832765)) ;
#42684=CARTESIAN_POINT('Ctrl Pts',(18.5300411021301,-1.19382615029684,-327.86740662328)) ;
#42685=CARTESIAN_POINT('Ctrl Pts',(18.5079099903433,-1.49832879568963,-327.871525005959)) ;
#42686=CARTESIAN_POINT('Ctrl Pts',(18.4515131040269,-2.07657284262969,-327.879343913353)) ;
#42687=CARTESIAN_POINT('Ctrl Pts',(18.4186468305415,-2.35030632805528,-327.88304433689)) ;
#42688=CARTESIAN_POINT('Ctrl Pts',(18.3548778686956,-2.7971084657546,-327.88903912823)) ;
#42689=CARTESIAN_POINT('Ctrl Pts',(18.3275911514274,-2.97064978009094,-327.891356156708)) ;
#42690=CARTESIAN_POINT('Ctrl Pts',(18.28428621462,-3.22269909291187,-327.894692686652)) ;
#42691=CARTESIAN_POINT('Ctrl Pts',(18.2702161846501,-3.30153182803569,-327.895732123652)) ;
#42692=CARTESIAN_POINT('Ctrl Pts',(18.2435298564916,-3.44565515112731,-327.89762332415)) ;
#42693=CARTESIAN_POINT('Ctrl Pts',(18.2310719907671,-3.51097352680301,-327.89847683669)) ;
#42694=CARTESIAN_POINT('Ctrl Pts',(18.1992467755902,-3.67309989608745,-327.900587258458)) ;
#42695=CARTESIAN_POINT('Ctrl Pts',(18.179457648151,-3.76982303372699,-327.901839302926)) ;
#42696=CARTESIAN_POINT('Ctrl Pts',(18.0861215898884,-4.20818612488769,-327.907490334085)) ;
#42697=CARTESIAN_POINT('Ctrl Pts',(18.0037089712388,-4.54786642968076,-327.911805742765)) ;
#42698=CARTESIAN_POINT('Ctrl Pts',(17.8031390693265,-5.28329039476061,-327.921168085715)) ;
#42699=CARTESIAN_POINT('Ctrl Pts',(17.6812663451557,-5.67782869885497,-327.926204200426)) ;
#42700=CARTESIAN_POINT('Ctrl Pts',(17.4565186356168,-6.32771602072079,-327.934670107157)) ;
#42701=CARTESIAN_POINT('Ctrl Pts',(17.360937536812,-6.585429403447,-327.938072408383)) ;
#42702=CARTESIAN_POINT('Ctrl Pts',(17.1800510866933,-7.04180633717154,-327.944209502882)) ;
#42703=CARTESIAN_POINT('Ctrl Pts',(17.096930504747,-7.24128157937077,-327.946930908755)) ;
#42704=CARTESIAN_POINT('Ctrl Pts',(16.957118206431,-7.5609713981056,-327.951364084896)) ;
#42705=CARTESIAN_POINT('Ctrl Pts',(16.9025846175058,-7.6821077535088,-327.953060750205)) ;
#42706=CARTESIAN_POINT('Ctrl Pts',(16.7936939753774,-7.91721434561734,-327.956388017307)) ;
#42707=CARTESIAN_POINT('Ctrl Pts',(16.7394649849125,-8.03123603800784,-327.958017635552)) ;
#42708=CARTESIAN_POINT('Ctrl Pts',(16.6029471078683,-8.31088734902738,-327.962054531688)) ;
#42709=CARTESIAN_POINT('Ctrl Pts',(16.5193384520843,-8.47585736883879,-327.964471072519)) ;
#42710=CARTESIAN_POINT('Ctrl Pts',(16.060666427503,-9.34829690839901,-327.977436107054)) ;
#42711=CARTESIAN_POINT('Ctrl Pts',(15.6425934124493,-10.0321942133913,-327.988297401468)) ;
#42712=CARTESIAN_POINT('Ctrl Pts',(15.0601413375938,-10.8596144489829,-328.001872417451)) ;
#42713=CARTESIAN_POINT('Ctrl Pts',(14.9356630150683,-11.0301882844288,-328.004693081071)) ;
#42714=CARTESIAN_POINT('Ctrl Pts',(14.7192684500912,-11.3163343740757,-328.009441228138)) ;
#42715=CARTESIAN_POINT('Ctrl Pts',(14.6288336241622,-11.4330011058988,-328.011381841904)) ;
#42716=CARTESIAN_POINT('Ctrl Pts',(14.4901743610848,-11.6075414027722,-328.014284714688)) ;
#42717=CARTESIAN_POINT('Ctrl Pts',(14.4429732637068,-11.6662202000395,-328.015260555245)) ;
#42718=CARTESIAN_POINT('Ctrl Pts',(14.3529034727887,-11.7768074282067,-328.017098137781)) ;
#42719=CARTESIAN_POINT('Ctrl Pts',(14.3101069772804,-11.8287729536979,-328.017960861672)) ;
#42720=CARTESIAN_POINT('Ctrl Pts',(14.1974279317006,-11.9640866670007,-328.020206721017)) ;
#42721=CARTESIAN_POINT('Ctrl Pts',(14.1270938372403,-12.0470556327372,-328.021583259906)) ;
#42722=CARTESIAN_POINT('Ctrl Pts',(13.6621538989957,-12.5858465790156,-328.03053504908)) ;
#42723=CARTESIAN_POINT('Ctrl Pts',(13.2462722157463,-13.022836119876,-328.03786763444)) ;
#42724=CARTESIAN_POINT('Ctrl Pts',(12.7464603394436,-13.499256330604,-328.046333525624)) ;
#42725=CARTESIAN_POINT('Ctrl Pts',(12.6826256525536,-13.5592470113239,-328.047408414561)) ;
#42726=CARTESIAN_POINT('Ctrl Pts',(12.3091365662166,-13.905300165218,-328.053665206647)) ;
#42727=CARTESIAN_POINT('Ctrl Pts',(11.9902360437277,-14.1812007319378,-328.058883035034)) ;
#42728=CARTESIAN_POINT('Ctrl Pts',(11.5425052184215,-14.5426526229642,-328.066125984913)) ;
#42729=CARTESIAN_POINT('Ctrl Pts',(11.421592132145,-14.6378073872467,-328.068073750817)) ;
#42730=CARTESIAN_POINT('Ctrl Pts',(11.1994958747663,-14.8081625993823,-328.071639424932)) ;
#42731=CARTESIAN_POINT('Ctrl Pts',(11.0987027881309,-14.8838564823262,-328.073253211064)) ;
#42732=CARTESIAN_POINT('Ctrl Pts',(10.8898248611445,-15.0374185680877,-328.076589520777)) ;
#42733=CARTESIAN_POINT('Ctrl Pts',(10.7816570062692,-15.1151617534979,-328.078312922642)) ;
#42734=CARTESIAN_POINT('Ctrl Pts',(10.494166538148,-15.3171326791413,-328.082882547602)) ;
#42735=CARTESIAN_POINT('Ctrl Pts',(10.313475159575,-15.4393754637695,-328.08574380936)) ;
#42736=CARTESIAN_POINT('Ctrl Pts',(9.89710472921494,-15.710490149969,-328.092308838859)) ;
#42737=CARTESIAN_POINT('Ctrl Pts',(9.66014276590698,-15.8572956107436,-328.096025335753)) ;
#42738=CARTESIAN_POINT('Ctrl Pts',(9.0641721815128,-16.2082003149744,-328.105297726627)) ;
#42739=CARTESIAN_POINT('Ctrl Pts',(8.70148898974456,-16.4057631244973,-328.110876874917)) ;
#42740=CARTESIAN_POINT('Ctrl Pts',(8.02863736007048,-16.7436889677968,-328.120993598246)) ;
#42741=CARTESIAN_POINT('Ctrl Pts',(7.72061629001675,-16.8879312833566,-328.12553866059)) ;
#42742=CARTESIAN_POINT('Ctrl Pts',(7.31758164856354,-17.0633348633018,-328.131305388436)) ;
#42743=CARTESIAN_POINT('Ctrl Pts',(7.22603793407603,-17.1023031682322,-328.13260332491)) ;
#42744=CARTESIAN_POINT('Ctrl Pts',(7.07270743065675,-17.1661219642137,-328.134754830337)) ;
#42745=CARTESIAN_POINT('Ctrl Pts',(7.01109226694358,-17.1913792044578,-328.135613326673)) ;
#42746=CARTESIAN_POINT('Ctrl Pts',(6.87547202374067,-17.2461221661343,-328.137489016636)) ;
#42747=CARTESIAN_POINT('Ctrl Pts',(6.80141049907751,-17.2754641200991,-328.138504495179)) ;
#42748=CARTESIAN_POINT('Ctrl Pts',(6.56586482811938,-17.3670339241863,-328.141709372429)) ;
#42749=CARTESIAN_POINT('Ctrl Pts',(6.40369816402056,-17.427481122392,-328.143879167906)) ;
#42750=CARTESIAN_POINT('Ctrl Pts',(5.98718969388352,-17.5761349162628,-328.149383342238)) ;
#42751=CARTESIAN_POINT('Ctrl Pts',(5.73173121889971,-17.6610933021273,-328.152694798589)) ;
#42752=CARTESIAN_POINT('Ctrl Pts',(4.8028988737558,-17.9477208913343,-328.164617420204)) ;
#42753=CARTESIAN_POINT('Ctrl Pts',(4.1200536227653,-18.1166685940836,-328.173183881467)) ;
#42754=CARTESIAN_POINT('Ctrl Pts',(3.24703152559254,-18.2807459702496,-328.184337347047)) ;
#42755=CARTESIAN_POINT('Ctrl Pts',(3.06428077691759,-18.3122655649673,-328.186681402715)) ;
#42756=CARTESIAN_POINT('Ctrl Pts',(2.75628331494997,-18.3606471141197,-328.190652331906)) ;
#42757=CARTESIAN_POINT('Ctrl Pts',(2.6312811088735,-18.378977660206,-328.192269536412)) ;
#42758=CARTESIAN_POINT('Ctrl Pts',(2.37460497552077,-18.4139447946416,-328.195602698083)) ;
#42759=CARTESIAN_POINT('Ctrl Pts',(2.24292011651937,-18.4304482034063,-328.197319427269)) ;
#42760=CARTESIAN_POINT('Ctrl Pts',(1.89712336973055,-18.4700242269768,-328.201845405104)) ;
#42761=CARTESIAN_POINT('Ctrl Pts',(1.68276749404526,-18.4907859576921,-328.204669155278)) ;
#42762=CARTESIAN_POINT('Ctrl Pts',(1.19551382079149,-18.5294364864431,-328.211125300394)) ;
#42763=CARTESIAN_POINT('Ctrl Pts',(0.922484303747169,-18.5450341628335,
-328.214769759589)) ;
#42764=CARTESIAN_POINT('Ctrl Pts',(0.298923316332265,-18.5668520646512,
-328.223131731931)) ;
#42765=CARTESIAN_POINT('Ctrl Pts',(-0.0516405535188888,-18.5691864029257,
-328.227861119503)) ;
#42766=CARTESIAN_POINT('Ctrl Pts',(-0.496303570331408,-18.5595546361347,
-328.233847674073)) ;
#42767=CARTESIAN_POINT('Ctrl Pts',(-0.590530806398523,-18.5567954911413,
-328.235115459867)) ;
#42768=CARTESIAN_POINT('Ctrl Pts',(-1.00686034382319,-18.5414303397882,
-328.240709138117)) ;
#42769=CARTESIAN_POINT('Ctrl Pts',(-1.32862416231878,-18.5211545368095,
-328.245012417834)) ;
#42770=CARTESIAN_POINT('Ctrl Pts',(-1.74706959872887,-18.4838254727084,
-328.250521759801)) ;
#42771=CARTESIAN_POINT('Ctrl Pts',(-1.84437221848916,-18.4743700149249,
-328.251796631625)) ;
#42772=CARTESIAN_POINT('Ctrl Pts',(-2.00761282017689,-18.4572044637966,
-328.253922397132)) ;
#42773=CARTESIAN_POINT('Ctrl Pts',(-2.07359224684668,-18.4499084302036,
-328.254777940366)) ;
#42774=CARTESIAN_POINT('Ctrl Pts',(-2.21961930991149,-18.4329674747788,
-328.256662803563)) ;
#42775=CARTESIAN_POINT('Ctrl Pts',(-2.29964595744679,-18.4231546783294,
-328.257690238041)) ;
#42776=CARTESIAN_POINT('Ctrl Pts',(-2.55727460430077,-18.3898596861652,
-328.260983381068)) ;
#42777=CARTESIAN_POINT('Ctrl Pts',(-2.73460166564056,-18.3643281012017,
-328.263227960304)) ;
#42778=CARTESIAN_POINT('Ctrl Pts',(-3.19250922378791,-18.2916189331276,
-328.268994186409)) ;
#42779=CARTESIAN_POINT('Ctrl Pts',(-3.47242460788392,-18.2405511455486,
-328.272490222804)) ;
#42780=CARTESIAN_POINT('Ctrl Pts',(-4.44341021501702,-18.0402427783326,
-328.284644224652)) ;
#42781=CARTESIAN_POINT('Ctrl Pts',(-5.12704238812446,-17.857986721414,-328.293271213128)) ;
#42782=CARTESIAN_POINT('Ctrl Pts',(-5.94677606926052,-17.588481445232,-328.304128174259)) ;
#42783=CARTESIAN_POINT('Ctrl Pts',(-6.09432117181592,-17.5379039377096,
-328.306101912922)) ;
#42784=CARTESIAN_POINT('Ctrl Pts',(-6.36035732933423,-17.4429458067768,
-328.309699304335)) ;
#42785=CARTESIAN_POINT('Ctrl Pts',(-6.47906545194072,-17.3992015503873,
-328.31131855925)) ;
#42786=CARTESIAN_POINT('Ctrl Pts',(-6.72110733833275,-17.307187933771,-328.314650067024)) ;
#42787=CARTESIAN_POINT('Ctrl Pts',(-6.84439038447217,-17.2588052376531,
-328.316363030721)) ;
#42788=CARTESIAN_POINT('Ctrl Pts',(-7.16528736218257,-17.1288893906088,
-328.320864384644)) ;
#42789=CARTESIAN_POINT('Ctrl Pts',(-7.36202910186227,-17.0452551167199,
-328.323666976467)) ;
#42790=CARTESIAN_POINT('Ctrl Pts',(-7.68887080011427,-16.8996011641234,
-328.32839244557)) ;
#42791=CARTESIAN_POINT('Ctrl Pts',(-7.81977206796812,-16.8394304662703,
-328.330303983716)) ;
#42792=CARTESIAN_POINT('Ctrl Pts',(-8.37980858284826,-16.5740629583676,
-328.338559108074)) ;
#42793=CARTESIAN_POINT('Ctrl Pts',(-8.80167077259434,-16.3539397399262,
-328.344978545542)) ;
#42794=CARTESIAN_POINT('Ctrl Pts',(-9.25795781762861,-16.0930795496178,
-328.352053823519)) ;
#42795=CARTESIAN_POINT('Ctrl Pts',(-9.30120339852626,-16.0681239627868,
-328.352725684207)) ;
#42796=CARTESIAN_POINT('Ctrl Pts',(-9.64002042099114,-15.8707777536731,
-328.35799855157)) ;
#42797=CARTESIAN_POINT('Ctrl Pts',(-9.93087616425577,-15.690419993574,-328.362580423341)) ;
#42798=CARTESIAN_POINT('Ctrl Pts',(-10.3113965535809,-15.4396403800449,
-328.368577700864)) ;
#42799=CARTESIAN_POINT('Ctrl Pts',(-10.4056364256555,-15.3762844857714,
-328.37006310627)) ;
#42800=CARTESIAN_POINT('Ctrl Pts',(-10.5504878085151,-15.2769617446286,
-328.372342794491)) ;
#42801=CARTESIAN_POINT('Ctrl Pts',(-10.6015100480348,-15.2415989272808,
-328.373145113702)) ;
#42802=CARTESIAN_POINT('Ctrl Pts',(-10.7108373304059,-15.1650111078859,
-328.374861945164)) ;
#42803=CARTESIAN_POINT('Ctrl Pts',(-10.7690838588645,-15.1237042776915,
-328.37577520215)) ;
#42804=CARTESIAN_POINT('Ctrl Pts',(-10.930250398835,-15.0080062587773,-328.378300212675)) ;
#42805=CARTESIAN_POINT('Ctrl Pts',(-11.0326477365926,-14.9328935456325,
-328.379902271404)) ;
#42806=CARTESIAN_POINT('Ctrl Pts',(-11.2702824385203,-14.7548000481966,
-328.383624085673)) ;
#42807=CARTESIAN_POINT('Ctrl Pts',(-11.4048922717077,-14.6510007545022,
-328.385735377501)) ;
#42808=CARTESIAN_POINT('Ctrl Pts',(-11.935562562396,-14.2300485528917,-328.394105085832)) ;
#42809=CARTESIAN_POINT('Ctrl Pts',(-12.3199746369712,-13.898566895034,-328.400278739922)) ;
#42810=CARTESIAN_POINT('Ctrl Pts',(-12.9586844536724,-13.3004572974636,
-328.411038976111)) ;
#42811=CARTESIAN_POINT('Ctrl Pts',(-13.2195184557534,-13.0412422003547,
-328.415590473488)) ;
#42812=CARTESIAN_POINT('Ctrl Pts',(-13.5999938872799,-12.6399766178496,
-328.42253362296)) ;
#42813=CARTESIAN_POINT('Ctrl Pts',(-13.7254835432438,-12.5035972417051,
-328.424876205074)) ;
#42814=CARTESIAN_POINT('Ctrl Pts',(-13.9330405005951,-12.271138408274,-328.428845417767)) ;
#42815=CARTESIAN_POINT('Ctrl Pts',(-14.0162068410048,-12.1760585233152,
-328.430462399685)) ;
#42816=CARTESIAN_POINT('Ctrl Pts',(-14.1847665037495,-11.9793371741802,
-328.433795751021)) ;
#42817=CARTESIAN_POINT('Ctrl Pts',(-14.2700530545605,-11.8776136347428,
-328.435512899211)) ;
#42818=CARTESIAN_POINT('Ctrl Pts',(-14.4909285692868,-11.6083563393389,
-328.440041617174)) ;
#42819=CARTESIAN_POINT('Ctrl Pts',(-14.6247038614405,-11.4393611890232,
-328.442867721984)) ;
#42820=CARTESIAN_POINT('Ctrl Pts',(-14.9216640739547,-11.0504928091501,
-328.449330678095)) ;
#42821=CARTESIAN_POINT('Ctrl Pts',(-15.0829884461214,-10.829261710037,-328.452979634677)) ;
#42822=CARTESIAN_POINT('Ctrl Pts',(-15.4393140253402,-10.3172006602097,
-328.461340421536)) ;
#42823=CARTESIAN_POINT('Ctrl Pts',(-15.6310996846999,-10.0242590429054,
-328.466063967434)) ;
#42824=CARTESIAN_POINT('Ctrl Pts',(-15.8635246395246,-9.64633854319791,
-328.472035762359)) ;
#42825=CARTESIAN_POINT('Ctrl Pts',(-15.9119573890841,-9.56623611115411,
-328.473294653642)) ;
#42826=CARTESIAN_POINT('Ctrl Pts',(-16.1136842163482,-9.22683130098725,
-328.478595920781)) ;
#42827=CARTESIAN_POINT('Ctrl Pts',(-16.2612618798849,-8.96418415413755,
-328.482618768823)) ;
#42828=CARTESIAN_POINT('Ctrl Pts',(-16.4531047761469,-8.6024161426674,-328.488001709626)) ;
#42829=CARTESIAN_POINT('Ctrl Pts',(-16.5029879489438,-8.50632759046972,
-328.489416548204)) ;
#42830=CARTESIAN_POINT('Ctrl Pts',(-16.5824833880533,-8.34986614679401,
-328.4916929519)) ;
#42831=CARTESIAN_POINT('Ctrl Pts',(-16.612613124818,-8.28975905493632,-328.492560953636)) ;
#42832=CARTESIAN_POINT('Ctrl Pts',(-16.6758754122883,-8.16182435190642,
-328.494393726641)) ;
#42833=CARTESIAN_POINT('Ctrl Pts',(-16.7089221054919,-8.09395574551899,
-328.495357447176)) ;
#42834=CARTESIAN_POINT('Ctrl Pts',(-16.805792235911,-7.89189005093344,-328.498203958701)) ;
#42835=CARTESIAN_POINT('Ctrl Pts',(-16.8684195068632,-7.75712606026524,
-328.500072767121)) ;
#42836=CARTESIAN_POINT('Ctrl Pts',(-16.9758350311224,-7.51853089790636,
-328.503340405499)) ;
#42837=CARTESIAN_POINT('Ctrl Pts',(-17.0213051862685,-7.41501528383948,
-328.504744662579)) ;
#42838=CARTESIAN_POINT('Ctrl Pts',(-17.238453484798,-6.90813943944556,-328.511567805263)) ;
#42839=CARTESIAN_POINT('Ctrl Pts',(-17.3967545149665,-6.4992001338689,-328.516913380959)) ;
#42840=CARTESIAN_POINT('Ctrl Pts',(-17.5875866470013,-5.94911710476848,
-328.524054601083)) ;
#42841=CARTESIAN_POINT('Ctrl Pts',(-17.6331593371579,-5.81264915114521,
-328.52582193637)) ;
#42842=CARTESIAN_POINT('Ctrl Pts',(-17.6970635788206,-5.61361622194164,
-328.528397919647)) ;
#42843=CARTESIAN_POINT('Ctrl Pts',(-17.7166590866234,-5.55146261848974,
-328.529202109731)) ;
#42844=CARTESIAN_POINT('Ctrl Pts',(-17.8322655254533,-5.17793192505153,
-328.534035291402)) ;
#42845=CARTESIAN_POINT('Ctrl Pts',(-17.9203926605644,-4.86417506054375,
-328.538096889836)) ;
#42846=CARTESIAN_POINT('Ctrl Pts',(-18.0379962809472,-4.39874661896167,
-328.544159415084)) ;
#42847=CARTESIAN_POINT('Ctrl Pts',(-18.073911256405,-4.24876610931386,-328.54611846898)) ;
#42848=CARTESIAN_POINT('Ctrl Pts',(-18.1353247548754,-3.97742002685228,
-328.549675052812)) ;
#42849=CARTESIAN_POINT('Ctrl Pts',(-18.1614837852016,-3.85621325964894,
-328.55126809418)) ;
#42850=CARTESIAN_POINT('Ctrl Pts',(-18.2162043384155,-3.58975088525467,
-328.554780569166)) ;
#42851=CARTESIAN_POINT('Ctrl Pts',(-18.2442467337896,-3.44439732723533,
-328.556703304959)) ;
#42852=CARTESIAN_POINT('Ctrl Pts',(-18.3256220108535,-2.99368643591197,
-328.562686016426)) ;
#42853=CARTESIAN_POINT('Ctrl Pts',(-18.3730482421428,-2.68731802043421,
-328.566782804346)) ;
#42854=CARTESIAN_POINT('Ctrl Pts',(-18.4772598861388,-1.88105690670342,
-328.577619199434)) ;
#42855=CARTESIAN_POINT('Ctrl Pts',(-18.5214383058594,-1.37979326884387,
-328.584415474029)) ;
#42856=CARTESIAN_POINT('Ctrl Pts',(-18.5478080794076,-0.822400084664782,
-328.591921380662)) ;
#42857=CARTESIAN_POINT('Ctrl Pts',(-18.5501637490318,-0.767431648842084,
-328.5926609585)) ;
#42858=CARTESIAN_POINT('Ctrl Pts',(-18.5648983072,-0.3837440720037,-328.597817545063)) ;
#42859=CARTESIAN_POINT('Ctrl Pts',(-18.5687832443194,-0.0547564736898822,
-328.602210508713)) ;
#42860=CARTESIAN_POINT('Ctrl Pts',(-18.5624825356949,0.371876246913001,
-328.607805992132)) ;
#42861=CARTESIAN_POINT('Ctrl Pts',(-18.560267922656,0.469579078038605,-328.609080423994)) ;
#42862=CARTESIAN_POINT('Ctrl Pts',(-18.5552539304723,0.633606287483184,
-328.611205701108)) ;
#42863=CARTESIAN_POINT('Ctrl Pts',(-18.5528700633289,0.699941283239329,
-328.612061190616)) ;
#42864=CARTESIAN_POINT('Ctrl Pts',(-18.5468021102246,0.846837874634305,
-328.613946241504)) ;
#42865=CARTESIAN_POINT('Ctrl Pts',(-18.5429487651842,0.927390973420635,
-328.614973914033)) ;
#42866=CARTESIAN_POINT('Ctrl Pts',(-18.5288384642232,1.18692122152031,-328.618268838595)) ;
#42867=CARTESIAN_POINT('Ctrl Pts',(-18.5165140650109,1.36577593317995,-328.620514929925)) ;
#42868=CARTESIAN_POINT('Ctrl Pts',(-18.4779088790104,1.82825102881213,-328.626286534595)) ;
#42869=CARTESIAN_POINT('Ctrl Pts',(-18.4476883614047,2.11149541768433,-328.629786380863)) ;
#42870=CARTESIAN_POINT('Ctrl Pts',(-18.3199193544384,3.09412571405806,-328.641933780138)) ;
#42871=CARTESIAN_POINT('Ctrl Pts',(-18.189005040234,3.78855569794481,-328.650550674341)) ;
#42872=CARTESIAN_POINT('Ctrl Pts',(-17.9812435580324,4.62533750497072,-328.661398396789)) ;
#42873=CARTESIAN_POINT('Ctrl Pts',(-17.9417187268702,4.77635802261492,-328.66337378415)) ;
#42874=CARTESIAN_POINT('Ctrl Pts',(-17.8667146293908,5.04886320284028,-328.666973195146)) ;
#42875=CARTESIAN_POINT('Ctrl Pts',(-17.831888752175,5.17051784308506,-328.668592803368)) ;
#42876=CARTESIAN_POINT('Ctrl Pts',(-17.7580880797287,5.41870219075343,-328.671924042578)) ;
#42877=CARTESIAN_POINT('Ctrl Pts',(-17.7189980363364,5.54519018662917,-328.67363637404)) ;
#42878=CARTESIAN_POINT('Ctrl Pts',(-17.6133418642507,5.87454422732882,-328.678133593473)) ;
#42879=CARTESIAN_POINT('Ctrl Pts',(-17.5446234386492,6.07669891100858,-328.680932632896)) ;
#42880=CARTESIAN_POINT('Ctrl Pts',(-17.4238113801289,6.41295368059579,-328.685650970359)) ;
#42881=CARTESIAN_POINT('Ctrl Pts',(-17.3736182306027,6.54771467256947,-328.687558941679)) ;
#42882=CARTESIAN_POINT('Ctrl Pts',(-17.1512422601802,7.12419421678658,-328.695789179788)) ;
#42883=CARTESIAN_POINT('Ctrl Pts',(-16.9637408314788,7.55981149840204,-328.7021868489)) ;
#42884=CARTESIAN_POINT('Ctrl Pts',(-16.7276368943837,8.05519971772877,-328.70957449565)) ;
#42885=CARTESIAN_POINT('Ctrl Pts',(-16.6950941938299,8.12243242048359,-328.710579445948)) ;
#42886=CARTESIAN_POINT('Ctrl Pts',(-16.5080197939169,8.50305073414986,-328.716279204931)) ;
#42887=CARTESIAN_POINT('Ctrl Pts',(-16.3450707909111,8.81222168432377,-328.720951089118)) ;
#42888=CARTESIAN_POINT('Ctrl Pts',(-16.1250190204767,9.20260868500017,-328.726829367449)) ;
#42889=CARTESIAN_POINT('Ctrl Pts',(-16.0758584792548,9.28821937813447,-328.728117033713)) ;
#42890=CARTESIAN_POINT('Ctrl Pts',(-15.9924461305286,9.43083176086942,-328.730257045562)) ;
#42891=CARTESIAN_POINT('Ctrl Pts',(-15.9585666988887,9.48804879271938,-328.731114194747)) ;
#42892=CARTESIAN_POINT('Ctrl Pts',(-15.883209712241,9.61376937102261,-328.73299381174)) ;
#42893=CARTESIAN_POINT('Ctrl Pts',(-15.8415949268799,9.68218893011981,-328.73401449003)) ;
#42894=CARTESIAN_POINT('Ctrl Pts',(-15.7072750772852,9.89984208749577,-328.737257467807)) ;
#42895=CARTESIAN_POINT('Ctrl Pts',(-15.6128938346539,10.0480301556232,-328.739459512306)) ;
#42896=CARTESIAN_POINT('Ctrl Pts',(-15.365026618945,10.4252804577153,-328.745075754619)) ;
#42897=CARTESIAN_POINT('Ctrl Pts',(-15.2085154515834,10.6523036836069,-328.748465897187)) ;
#42898=CARTESIAN_POINT('Ctrl Pts',(-14.6219127355575,11.463889924009,-328.760745400854)) ;
#42899=CARTESIAN_POINT('Ctrl Pts',(-14.1627020257357,12.0265945057044,-328.769594546679)) ;
#42900=CARTESIAN_POINT('Ctrl Pts',(-13.5674789939611,12.6744530893621,-328.780667958738)) ;
#42901=CARTESIAN_POINT('Ctrl Pts',(-13.4618098873805,12.7866305894679,-328.782618738671)) ;
#42902=CARTESIAN_POINT('Ctrl Pts',(-13.2671565738272,12.9881852914467,-328.786188083558)) ;
#42903=CARTESIAN_POINT('Ctrl Pts',(-13.1786347926589,13.0779962405622,-328.78780249454)) ;
#42904=CARTESIAN_POINT('Ctrl Pts',(-12.9948032493127,13.2607430577359,-328.791138189861)) ;
#42905=CARTESIAN_POINT('Ctrl Pts',(-12.8993950554435,13.3535697501581,-328.792860332634)) ;
#42906=CARTESIAN_POINT('Ctrl Pts',(-12.6454029647254,13.595427120094,-328.79742171938)) ;
#42907=CARTESIAN_POINT('Ctrl Pts',(-12.4851830147489,13.7427093233366,-328.80027590009)) ;
#42908=CARTESIAN_POINT('Ctrl Pts',(-11.6792555938629,14.4578291143289,-328.814511544614)) ;
#42909=CARTESIAN_POINT('Ctrl Pts',(-10.9972362895098,14.9831443320925,-328.826236017318)) ;
#42910=CARTESIAN_POINT('Ctrl Pts',(-10.1132759228889,15.5710261995572,-328.840382677265)) ;
#42911=CARTESIAN_POINT('Ctrl Pts',(-9.94346552073621,15.6800095821046,-328.843052746969)) ;
#42912=CARTESIAN_POINT('Ctrl Pts',(-9.69877822552249,15.8314749290872,-328.846815580553)) ;
#42913=CARTESIAN_POINT('Ctrl Pts',(-9.6253302380238,15.8762374426617,-328.847934382164)) ;
#42914=CARTESIAN_POINT('Ctrl Pts',(-9.49519481938215,15.9543128166624,-328.849896042747)) ;
#42915=CARTESIAN_POINT('Ctrl Pts',(-9.43863672459305,15.9878378433132,-328.850741656057)) ;
#42916=CARTESIAN_POINT('Ctrl Pts',(-9.30549724544581,16.0658040537127,-328.852716157355)) ;
#42917=CARTESIAN_POINT('Ctrl Pts',(-9.22877381539913,16.1099991549433,-328.853841827688)) ;
#42918=CARTESIAN_POINT('Ctrl Pts',(-8.94431747867649,16.2711559596593,-328.857975609634)) ;
#42919=CARTESIAN_POINT('Ctrl Pts',(-8.73465328176057,16.3846624589636,-328.860945111996)) ;
#42920=CARTESIAN_POINT('Ctrl Pts',(-8.09849647217279,16.7133785583656,-328.869797976526)) ;
#42921=CARTESIAN_POINT('Ctrl Pts',(-7.66582690318696,16.9161983608373,-328.87561514106)) ;
#42922=CARTESIAN_POINT('Ctrl Pts',(-6.80882715397221,17.2782896736915,-328.887041281656)) ;
#42923=CARTESIAN_POINT('Ctrl Pts',(-6.3855329231001,17.4391625152545,-328.892641207699)) ;
#42924=CARTESIAN_POINT('Ctrl Pts',(-5.80178697817189,17.63690869026,-328.900406749879)) ;
#42925=CARTESIAN_POINT('Ctrl Pts',(-5.64610285607817,17.6873627971359,-328.902481363536)) ;
#42926=CARTESIAN_POINT('Ctrl Pts',(-5.37039885622113,17.7727018436518,-328.90616468816)) ;
#42927=CARTESIAN_POINT('Ctrl Pts',(-5.25065557123506,17.8084454885514,-328.907767483206)) ;
#42928=CARTESIAN_POINT('Ctrl Pts',(-4.99607695718351,17.8816468937493,-328.911182421605)) ;
#42929=CARTESIAN_POINT('Ctrl Pts',(-4.86116049450667,17.9187945791184,-328.912996538463)) ;
#42930=CARTESIAN_POINT('Ctrl Pts',(-4.47709968718839,18.0198844211697,-328.918173239851)) ;
#42931=CARTESIAN_POINT('Ctrl Pts',(-4.22702904635217,18.0801792353798,-328.921559122564)) ;
#42932=CARTESIAN_POINT('Ctrl Pts',(-3.16194626012095,18.3136769929548,-328.93602764114)) ;
#42933=CARTESIAN_POINT('Ctrl Pts',(-2.33702352660584,18.4371087597631,-328.947396428164)) ;
#42934=CARTESIAN_POINT('Ctrl Pts',(-1.33002530105114,18.5190961091707,-328.960818447185)) ;
#42935=CARTESIAN_POINT('Ctrl Pts',(-1.15324428054706,18.5309448172915,-328.96315568684)) ;
#42936=CARTESIAN_POINT('Ctrl Pts',(-0.896116445282131,18.5444850363538,
-328.966515224425)) ;
#42937=CARTESIAN_POINT('Ctrl Pts',(-0.815885649505258,18.5481880672469,
-328.967557827648)) ;
#42938=CARTESIAN_POINT('Ctrl Pts',(-0.675949258570448,18.5537370841316,
-328.96936493221)) ;
#42939=CARTESIAN_POINT('Ctrl Pts',(-0.616254274080633,18.5558157420915,
-328.970132091641)) ;
#42940=CARTESIAN_POINT('Ctrl Pts',(-0.463829799070343,18.5603870144338,
-328.972081981578)) ;
#42941=CARTESIAN_POINT('Ctrl Pts',(-0.371089758064073,18.5624728049455,
-328.973260042188)) ;
#42942=CARTESIAN_POINT('Ctrl Pts',(0.00228856765034612,18.5680710652833,
-328.977975801849)) ;
#42943=CARTESIAN_POINT('Ctrl Pts',(0.282975029303099,18.5659148470277,-328.981459516529)) ;
#42944=CARTESIAN_POINT('Ctrl Pts',(1.27669570988853,18.5357400067762,-328.993713250721)) ;
#42945=CARTESIAN_POINT('Ctrl Pts',(1.98804470223297,18.4729881337875,-329.00236209498)) ;
#42946=CARTESIAN_POINT('Ctrl Pts',(2.93652311281207,18.3338868430283,-329.014301394551)) ;
#42947=CARTESIAN_POINT('Ctrl Pts',(3.17830329243401,18.2935224223884,-329.017378159301)) ;
#42948=CARTESIAN_POINT('Ctrl Pts',(3.55594556526066,18.2227633116825,-329.022249201092)) ;
#42949=CARTESIAN_POINT('Ctrl Pts',(3.69238576582513,18.1956076805139,-329.024022479073)) ;
#42950=CARTESIAN_POINT('Ctrl Pts',(3.9509737619485,18.1411126930506,-329.027410377427)) ;
#42951=CARTESIAN_POINT('Ctrl Pts',(4.0731755640644,18.1140664728138,-329.029022974264)) ;
#42952=CARTESIAN_POINT('Ctrl Pts',(4.35900190358412,18.0477675329933,-329.032822590077)) ;
#42953=CARTESIAN_POINT('Ctrl Pts',(4.5223847500422,18.0075219441354,-329.035016032389)) ;
#42954=CARTESIAN_POINT('Ctrl Pts',(5.25148165400773,17.8173771320086,-329.044899707635)) ;
#42955=CARTESIAN_POINT('Ctrl Pts',(5.81046424766624,17.6430011113935,-329.052747661673)) ;
#42956=CARTESIAN_POINT('Ctrl Pts',(6.85645229004998,17.2615900142105,-329.067742915159)) ;
#42957=CARTESIAN_POINT('Ctrl Pts',(7.34468565292565,17.0595727237352,-329.074874526586)) ;
#42958=CARTESIAN_POINT('Ctrl Pts',(7.9245127595969,16.7901449959315,-329.083284559573)) ;
#42959=CARTESIAN_POINT('Ctrl Pts',(8.02496124031148,16.7423674732572,-329.084738960207)) ;
#42960=CARTESIAN_POINT('Ctrl Pts',(8.18044979104515,16.6666897480717,-329.08698287885)) ;
#42961=CARTESIAN_POINT('Ctrl Pts',(8.2357903151535,16.6394129657847,-329.087780043204)) ;
#42962=CARTESIAN_POINT('Ctrl Pts',(8.35545007685986,16.5796906765487,-329.089499641702)) ;
#42963=CARTESIAN_POINT('Ctrl Pts',(8.41971851920079,16.5471456448645,-329.090420707702)) ;
#42964=CARTESIAN_POINT('Ctrl Pts',(8.59963278005804,16.4547189241417,-329.09299416176)) ;
#42965=CARTESIAN_POINT('Ctrl Pts',(8.71484042633788,16.3939932674618,-329.094636252659)) ;
#42966=CARTESIAN_POINT('Ctrl Pts',(8.98435137553112,16.2482908982507,-329.098473780236)) ;
#42967=CARTESIAN_POINT('Ctrl Pts',(9.13810320178457,16.1623202780274,-329.100660024386)) ;
#42968=CARTESIAN_POINT('Ctrl Pts',(9.76896591725543,15.797692010374,-329.109657145919)) ;
#42969=CARTESIAN_POINT('Ctrl Pts',(10.2347432684803,15.4999935391241,-329.116372281035)) ;
#42970=CARTESIAN_POINT('Ctrl Pts',(10.9929088910055,14.9663225903865,-329.127799103793)) ;
#42971=CARTESIAN_POINT('Ctrl Pts',(11.2926693610923,14.7414543228634,-329.132454969548)) ;
#42972=CARTESIAN_POINT('Ctrl Pts',(11.7095960125738,14.4085083748425,-329.13918631324)) ;
#42973=CARTESIAN_POINT('Ctrl Pts',(11.8324933234658,14.3077550305541,-329.141203265931)) ;
#42974=CARTESIAN_POINT('Ctrl Pts',(12.0491469448274,14.1254378499473,-329.144820629031)) ;
#42975=CARTESIAN_POINT('Ctrl Pts',(12.1434064800096,14.0444870166558,-329.146415818328)) ;
#42976=CARTESIAN_POINT('Ctrl Pts',(12.3454699763002,13.8673981785719,-329.1498828556)) ;
#42977=CARTESIAN_POINT('Ctrl Pts',(12.4529789662129,13.7709359146698,-329.151757431808)) ;
#42978=CARTESIAN_POINT('Ctrl Pts',(12.7695739339482,13.4801320824121,-329.157367841748)) ;
#42979=CARTESIAN_POINT('Ctrl Pts',(12.975314933628,13.282212964119,-329.161133860241)) ;
#42980=CARTESIAN_POINT('Ctrl Pts',(13.4793091616763,12.7744895006594,-329.170651052562)) ;
#42981=CARTESIAN_POINT('Ctrl Pts',(13.7715163973202,12.4589201957367,-329.176441162765)) ;
#42982=CARTESIAN_POINT('Ctrl Pts',(14.3510761117434,11.7876983772191,-329.188386762579)) ;
#42983=CARTESIAN_POINT('Ctrl Pts',(14.6367837320738,11.4310009021824,-329.1945385908)) ;
#42984=CARTESIAN_POINT('Ctrl Pts',(14.9782260159731,10.9709034303299,-329.202082268983)) ;
#42985=CARTESIAN_POINT('Ctrl Pts',(15.0465334193819,10.8770312487457,-329.203601530243)) ;
#42986=CARTESIAN_POINT('Ctrl Pts',(15.1502571554111,10.7316408090449,-329.205920398291)) ;
#42987=CARTESIAN_POINT('Ctrl Pts',(15.186301185109,10.6805740789779,-329.206728472808)) ;
#42988=CARTESIAN_POINT('Ctrl Pts',(15.2626087439176,10.5712952550637,-329.208443205451)) ;
#42989=CARTESIAN_POINT('Ctrl Pts',(15.3027986705916,10.5130329543827,-329.209348722788)) ;
#42990=CARTESIAN_POINT('Ctrl Pts',(15.4123644716266,10.3522387090938,-329.211825935384)) ;
#42991=CARTESIAN_POINT('Ctrl Pts',(15.4810495936202,10.2492403841038,-329.213388516475)) ;
#42992=CARTESIAN_POINT('Ctrl Pts',(15.6383142709665,10.0082225836565,-329.216997455965)) ;
#42993=CARTESIAN_POINT('Ctrl Pts',(15.7261055415446,9.8697009649993,-329.219036032986)) ;
#42994=CARTESIAN_POINT('Ctrl Pts',(16.0572964014171,9.33149048201659,-329.226850446068)) ;
#42995=CARTESIAN_POINT('Ctrl Pts',(16.2873872022798,8.92381653580239,-329.23255105411)) ;
#42996=CARTESIAN_POINT('Ctrl Pts',(16.7140540836628,8.09625673332628,-329.243981840361)) ;
#42997=CARTESIAN_POINT('Ctrl Pts',(16.910802054966,7.67683199633442,-329.249707312655)) ;
#42998=CARTESIAN_POINT('Ctrl Pts',(17.1501885421993,7.11252366918415,-329.257429386254)) ;
#42999=CARTESIAN_POINT('Ctrl Pts',(17.2070433723845,6.97385247009293,-329.259327983806)) ;
#43000=CARTESIAN_POINT('Ctrl Pts',(17.3087674904143,6.71692346791216,-329.262850100218)) ;
#43001=CARTESIAN_POINT('Ctrl Pts',(17.354119337829,6.59886618032869,-329.264470173927)) ;
#43002=CARTESIAN_POINT('Ctrl Pts',(17.445462819266,6.35362995455593,-329.267839930924)) ;
#43003=CARTESIAN_POINT('Ctrl Pts',(17.4912782154418,6.22639324986314,-329.269590718873)) ;
#43004=CARTESIAN_POINT('Ctrl Pts',(17.6111456056611,5.88173459720228,-329.274340204026)) ;
#43005=CARTESIAN_POINT('Ctrl Pts',(17.6825596771967,5.66342073081232,-329.277356230039)) ;
#43006=CARTESIAN_POINT('Ctrl Pts',(17.7969144682316,5.29056127808998,-329.282516327658)) ;
#43007=CARTESIAN_POINT('Ctrl Pts',(17.8419366818134,5.13668167059828,-329.284648400138)) ;
#43008=CARTESIAN_POINT('Ctrl Pts',(18.042799180619,4.41563673193793,-329.29464188041)) ;
#43009=CARTESIAN_POINT('Ctrl Pts',(18.1736234602727,3.84185607541159,-329.302614709956)) ;
#43010=CARTESIAN_POINT('Ctrl Pts',(18.3199072260667,3.02243807143412,-329.3137642967)) ;
#43011=CARTESIAN_POINT('Ctrl Pts',(18.3580764716915,2.78121579374912,-329.317016213756)) ;
#43012=CARTESIAN_POINT('Ctrl Pts',(18.4063010161381,2.43193968077421,-329.32165132707)) ;
#43013=CARTESIAN_POINT('Ctrl Pts',(18.4201852004245,2.32444078064242,-329.32306785437)) ;
#43014=CARTESIAN_POINT('Ctrl Pts',(18.4411578397834,2.15005124098106,-329.325346212118)) ;
#43015=CARTESIAN_POINT('Ctrl Pts',(18.4488255373903,2.0832328580525,-329.326214500059)) ;
#43016=CARTESIAN_POINT('Ctrl Pts',(18.4643232872109,1.94137997269128,-329.328046987204)) ;
#43017=CARTESIAN_POINT('Ctrl Pts',(18.4720594048526,1.86633652293836,-329.329010144397)) ;
#43018=CARTESIAN_POINT('Ctrl Pts',(18.4936505815662,1.64359201073278,-329.331852937352)) ;
#43019=CARTESIAN_POINT('Ctrl Pts',(18.5061930156225,1.49576960810489,-329.333718644129)) ;
#43020=CARTESIAN_POINT('Ctrl Pts',(18.5324048286394,1.13565786237487,-329.338227834286)) ;
#43021=CARTESIAN_POINT('Ctrl Pts',(18.5441999416556,0.923253083740634,-329.340857311212)) ;
#43022=CARTESIAN_POINT('Ctrl Pts',(18.5727651835436,0.177568840775042,-329.350039598519)) ;
#43023=CARTESIAN_POINT('Ctrl Pts',(18.5701969915469,-0.356150271044903,
-329.35653102772)) ;
#43024=CARTESIAN_POINT('Ctrl Pts',(18.5446545934183,-0.888979984762296,
-329.363119887734)) ;
#43025=CARTESIAN_POINT('Origin',(0.,0.,-315.477129595899)) ;
#43026=CARTESIAN_POINT('',(18.5446545937517,-0.888979977808743,-331.160160528407)) ;
#43027=CARTESIAN_POINT('',(18.544654593742,-0.888979978010901,-330.86430516735)) ;
#43028=CARTESIAN_POINT('',(18.544654593745,-0.888979977948782,-315.477129595899)) ;
#43029=CARTESIAN_POINT('',(4.76165266723923E-5,-18.5659499999389,-330.021951923812)) ;
#43030=CARTESIAN_POINT('Ctrl Pts',(18.5446545937584,-0.888979977668659,
-331.160160528407)) ;
#43031=CARTESIAN_POINT('Ctrl Pts',(18.5481227871158,-0.8166313877202,-331.15924327645)) ;
#43032=CARTESIAN_POINT('Ctrl Pts',(18.5511676134064,-0.744262185559457,
-331.158323422676)) ;
#43033=CARTESIAN_POINT('Ctrl Pts',(18.558360962383,-0.545618593590704,-331.155791736724)) ;
#43034=CARTESIAN_POINT('Ctrl Pts',(18.5616441554253,-0.419317843523367,
-331.154174480573)) ;
#43035=CARTESIAN_POINT('Ctrl Pts',(18.5657321922503,-0.160305871188285,
-331.150841361856)) ;
#43036=CARTESIAN_POINT('Ctrl Pts',(18.566403744436,-0.0275996911559258,
-331.149124728823)) ;
#43037=CARTESIAN_POINT('Ctrl Pts',(18.5644336733073,0.320401348695704,-331.144599380799)) ;
#43038=CARTESIAN_POINT('Ctrl Pts',(18.5594698156593,0.5356627145399,-331.141776171986)) ;
#43039=CARTESIAN_POINT('Ctrl Pts',(18.5397085601776,1.02393110241196,-331.135321592516)) ;
#43040=CARTESIAN_POINT('Ctrl Pts',(18.5226226293287,1.29679563580841,-331.131678167029)) ;
#43041=CARTESIAN_POINT('Ctrl Pts',(18.4698853880767,1.91852915750099,-331.123315926543)) ;
#43042=CARTESIAN_POINT('Ctrl Pts',(18.4303631454727,2.26696589651703,-331.118585200598)) ;
#43043=CARTESIAN_POINT('Ctrl Pts',(18.3676904974804,2.70765197174233,-331.112593889649)) ;
#43044=CARTESIAN_POINT('Ctrl Pts',(18.3536677345799,2.8011272923186,-331.111322693582)) ;
#43045=CARTESIAN_POINT('Ctrl Pts',(18.2887605515523,3.2123665089465,-331.105732855716)) ;
#43046=CARTESIAN_POINT('Ctrl Pts',(18.2303329455754,3.52888403516724,-331.101436761758)) ;
#43047=CARTESIAN_POINT('Ctrl Pts',(18.1434367596884,3.93951637247554,-331.095932209225)) ;
#43048=CARTESIAN_POINT('Ctrl Pts',(18.1224078808916,4.03514799492262,-331.094655267207)) ;
#43049=CARTESIAN_POINT('Ctrl Pts',(18.0858508053869,4.19534371405165,-331.092527202141)) ;
#43050=CARTESIAN_POINT('Ctrl Pts',(18.0707309758703,4.25999885758617,-331.091671404628)) ;
#43051=CARTESIAN_POINT('Ctrl Pts',(18.0365054747331,4.40289173015556,-331.089787417524)) ;
#43052=CARTESIAN_POINT('Ctrl Pts',(18.0172369557155,4.48108891154186,-331.08876109764)) ;
#43053=CARTESIAN_POINT('Ctrl Pts',(17.9536095144795,4.73226078727507,-331.085476283827)) ;
#43054=CARTESIAN_POINT('Ctrl Pts',(17.907263607486,4.90472191333748,-331.083238772763)) ;
#43055=CARTESIAN_POINT('Ctrl Pts',(17.7810499760305,5.34872538204143,-331.077497645468)) ;
#43056=CARTESIAN_POINT('Ctrl Pts',(17.6974479174435,5.61915821806239,-331.074019376348)) ;
#43057=CARTESIAN_POINT('Ctrl Pts',(17.3823049679693,6.56164169255582,-331.061836096526)) ;
#43058=CARTESIAN_POINT('Ctrl Pts',(17.1183917639599,7.22221092963999,-331.053163563286)) ;
#43059=CARTESIAN_POINT('Ctrl Pts',(16.7514236715618,8.00677534518241,-331.042264547455)) ;
#43060=CARTESIAN_POINT('Ctrl Pts',(16.683822211145,8.14670011640386,-331.040297880446)) ;
#43061=CARTESIAN_POINT('Ctrl Pts',(16.5580696337901,8.39885716748686,-331.036709143154)) ;
#43062=CARTESIAN_POINT('Ctrl Pts',(16.5005137505024,8.51137577795021,-331.035091395404)) ;
#43063=CARTESIAN_POINT('Ctrl Pts',(16.3802080948564,8.74075938453084,-331.031758687381)) ;
#43064=CARTESIAN_POINT('Ctrl Pts',(16.3173457164775,8.85755725670296,-331.030042971464)) ;
#43065=CARTESIAN_POINT('Ctrl Pts',(16.1493586234133,9.1618177944381,-331.025523620874)) ;
#43066=CARTESIAN_POINT('Ctrl Pts',(16.0422210325689,9.34814598392815,-331.022705565621)) ;
#43067=CARTESIAN_POINT('Ctrl Pts',(15.7918845169414,9.76653565176752,-331.016265880712)) ;
#43068=CARTESIAN_POINT('Ctrl Pts',(15.6467596053445,9.99738709261697,-331.012632285647)) ;
#43069=CARTESIAN_POINT('Ctrl Pts',(15.3029980488245,10.5183805756114,-331.004267580816)) ;
#43070=CARTESIAN_POINT('Ctrl Pts',(15.1010977328267,10.8062447754485,-330.999524212466)) ;
#43071=CARTESIAN_POINT('Ctrl Pts',(14.8301535264014,11.1701152944837,-330.993417828854)) ;
#43072=CARTESIAN_POINT('Ctrl Pts',(14.768485087998,11.2515233423899,-330.992044398152)) ;
#43073=CARTESIAN_POINT('Ctrl Pts',(14.5129480704408,11.5831352791013,-330.986424909322)) ;
#43074=CARTESIAN_POINT('Ctrl Pts',(14.3133677336897,11.82887101243,-330.982201151328)) ;
#43075=CARTESIAN_POINT('Ctrl Pts',(14.0444958234674,12.1431486907464,-330.976778100764)) ;
#43076=CARTESIAN_POINT('Ctrl Pts',(13.9808111620209,12.2164169195587,-330.975512336279)) ;
#43077=CARTESIAN_POINT('Ctrl Pts',(13.8726664350371,12.3388825131193,-330.973396659304)) ;
#43078=CARTESIAN_POINT('Ctrl Pts',(13.8285121955437,12.3883471933111,-330.972542206843)) ;
#43079=CARTESIAN_POINT('Ctrl Pts',(13.7298114853869,12.497733460438,-330.970653355)) ;
#43080=CARTESIAN_POINT('Ctrl Pts',(13.6751359040282,12.5575365061447,-330.969620911739)) ;
#43081=CARTESIAN_POINT('Ctrl Pts',(13.4965550335862,12.7503151345888,-330.966290078243)) ;
#43082=CARTESIAN_POINT('Ctrl Pts',(13.3710880204971,12.8818298064171,-330.964013486387)) ;
#43083=CARTESIAN_POINT('Ctrl Pts',(13.0395948188231,13.2192394990963,-330.958132687744)) ;
#43084=CARTESIAN_POINT('Ctrl Pts',(12.8306187566375,13.4221663202339,-330.954555309347)) ;
#43085=CARTESIAN_POINT('Ctrl Pts',(12.110658413272,14.0891006456218,-330.942526560241)) ;
#43086=CARTESIAN_POINT('Ctrl Pts',(11.5786033490314,14.5295130016241,-330.934099782661)) ;
#43087=CARTESIAN_POINT('Ctrl Pts',(10.88187683553,15.043607686256,-330.923210606501)) ;
#43088=CARTESIAN_POINT('Ctrl Pts',(10.739010985984,15.1459241576935,-330.920986416848)) ;
#43089=CARTESIAN_POINT('Ctrl Pts',(10.4911360566456,15.3181745940061,-330.917138160645)) ;
#43090=CARTESIAN_POINT('Ctrl Pts',(10.3868269519003,15.3890946604943,-330.915521982655)) ;
#43091=CARTESIAN_POINT('Ctrl Pts',(10.1685346175898,15.53428171424,-330.912145433226)) ;
#43092=CARTESIAN_POINT('Ctrl Pts',(10.054441419404,15.6083699444631,-330.910383799769)) ;
#43093=CARTESIAN_POINT('Ctrl Pts',(9.74165779318092,15.8066281923907,-330.905562511127)) ;
#43094=CARTESIAN_POINT('Ctrl Pts',(9.5414149554891,15.9283015948812,-330.902484577182)) ;
#43095=CARTESIAN_POINT('Ctrl Pts',(9.07062412638347,16.2023036967203,-330.895273673872)) ;
#43096=CARTESIAN_POINT('Ctrl Pts',(8.79845109259639,16.3517009799672,-330.891123625488)) ;
#43097=CARTESIAN_POINT('Ctrl Pts',(8.15395552397445,16.6847159826388,-330.88137809388)) ;
#43098=CARTESIAN_POINT('Ctrl Pts',(7.77896601033168,16.8628119159217,-330.875768151297)) ;
#43099=CARTESIAN_POINT('Ctrl Pts',(7.13421472922153,17.14294025996,-330.86634533474)) ;
#43100=CARTESIAN_POINT('Ctrl Pts',(6.86747076873449,17.2515293928735,-330.862510163059)) ;
#43101=CARTESIAN_POINT('Ctrl Pts',(6.51851579755499,17.3842094617561,-330.857618278281)) ;
#43102=CARTESIAN_POINT('Ctrl Pts',(6.43851423539279,17.413997854622,-330.856505231405)) ;
#43103=CARTESIAN_POINT('Ctrl Pts',(6.29535314917866,17.4661821340035,-330.854530346371)) ;
#43104=CARTESIAN_POINT('Ctrl Pts',(6.23227244016171,17.4887898347052,-330.853666024741)) ;
#43105=CARTESIAN_POINT('Ctrl Pts',(6.09537792271287,17.537017191739,-330.851803751006)) ;
#43106=CARTESIAN_POINT('Ctrl Pts',(6.02152211482329,17.5625133579141,-330.850807237702)) ;
#43107=CARTESIAN_POINT('Ctrl Pts',(5.79237513587827,17.6400030567689,-330.847737833842)) ;
#43108=CARTESIAN_POINT('Ctrl Pts',(5.63655520357092,17.6904087898536,-330.845682314259)) ;
#43109=CARTESIAN_POINT('Ctrl Pts',(4.99743586894677,17.8878540050492,-330.83734675238)) ;
#43110=CARTESIAN_POINT('Ctrl Pts',(4.50889759314673,18.0172009728816,-330.831190943995)) ;
#43111=CARTESIAN_POINT('Ctrl Pts',(3.5037655121286,18.239875513533,-330.818569888844)) ;
#43112=CARTESIAN_POINT('Ctrl Pts',(2.98726399128732,18.3315488636272,-330.812106284076)) ;
#43113=CARTESIAN_POINT('Ctrl Pts',(2.31869805305841,18.4212025245819,-330.80360924413)) ;
#43114=CARTESIAN_POINT('Ctrl Pts',(2.16958182819799,18.4393594715001,-330.801706411908)) ;
#43115=CARTESIAN_POINT('Ctrl Pts',(1.89447760420637,18.4694738764635,-330.798179194162)) ;
#43116=CARTESIAN_POINT('Ctrl Pts',(1.76855599578412,18.4819566145575,-330.796558297825)) ;
#43117=CARTESIAN_POINT('Ctrl Pts',(1.5079741875116,18.5051008575434,-330.793189818168)) ;
#43118=CARTESIAN_POINT('Ctrl Pts',(1.37330536849315,18.5155819837578,-330.791441161656)) ;
#43119=CARTESIAN_POINT('Ctrl Pts',(1.01026884317501,18.5398542148108,-330.786705741932)) ;
#43120=CARTESIAN_POINT('Ctrl Pts',(0.781741177960401,18.5508953388265,-330.783701833575)) ;
#43121=CARTESIAN_POINT('Ctrl Pts',(0.393762692635999,18.5624581118883,-330.77856674986)) ;
#43122=CARTESIAN_POINT('Ctrl Pts',(0.234402720213039,18.5651543353626,-330.776447541044)) ;
#43123=CARTESIAN_POINT('Ctrl Pts',(-0.505578151244105,18.5681447403556,
-330.766568940198)) ;
#43124=CARTESIAN_POINT('Ctrl Pts',(-1.08597317809753,18.5432539875002,-330.758700760651)) ;
#43125=CARTESIAN_POINT('Ctrl Pts',(-1.94616852480889,18.4658347306011,-330.747126442984)) ;
#43126=CARTESIAN_POINT('Ctrl Pts',(-2.22747569809587,18.4340168386924,-330.743357457767)) ;
#43127=CARTESIAN_POINT('Ctrl Pts',(-2.59258420454397,18.3842406262605,-330.738528940324)) ;
#43128=CARTESIAN_POINT('Ctrl Pts',(-2.67714234873171,18.3721176006886,-330.737415156243)) ;
#43129=CARTESIAN_POINT('Ctrl Pts',(-2.82788844212664,18.3494424454694,-330.735439387527)) ;
#43130=CARTESIAN_POINT('Ctrl Pts',(-2.89410860984592,18.3391146595194,-330.734574912243)) ;
#43131=CARTESIAN_POINT('Ctrl Pts',(-3.0373689639651,18.3159763113108,-330.73271293137)) ;
#43132=CARTESIAN_POINT('Ctrl Pts',(-3.11438704382568,18.3030377758217,-330.731716858073)) ;
#43133=CARTESIAN_POINT('Ctrl Pts',(-3.35243871359538,18.2615005751385,-330.728650535774)) ;
#43134=CARTESIAN_POINT('Ctrl Pts',(-3.51317791850914,18.2312596836872,-330.726597608503)) ;
#43135=CARTESIAN_POINT('Ctrl Pts',(-4.16834361696844,18.0990127242423,-330.71826858247)) ;
#43136=CARTESIAN_POINT('Ctrl Pts',(-4.65891161228077,17.9789848134266,-330.712116695807)) ;
#43137=CARTESIAN_POINT('Ctrl Pts',(-5.60631444422846,17.705797534222,-330.700029043485)) ;
#43138=CARTESIAN_POINT('Ctrl Pts',(-6.0632929631573,17.5545579600269,-330.69410133502)) ;
#43139=CARTESIAN_POINT('Ctrl Pts',(-6.68754920369072,17.3206691725551,-330.68573120314)) ;
#43140=CARTESIAN_POINT('Ctrl Pts',(-6.86023510701914,17.2530017405025,-330.683386882274)) ;
#43141=CARTESIAN_POINT('Ctrl Pts',(-7.1488047929945,17.1349073837524,-330.679415643943)) ;
#43142=CARTESIAN_POINT('Ctrl Pts',(-7.26524002350625,17.0858639923686,-330.677798399152)) ;
#43143=CARTESIAN_POINT('Ctrl Pts',(-7.50293288297232,16.982876916992,-330.674465270829)) ;
#43144=CARTESIAN_POINT('Ctrl Pts',(-7.62413098073381,16.9288138081309,-330.672748616487)) ;
#43145=CARTESIAN_POINT('Ctrl Pts',(-7.94042244954395,16.7836393492035,-330.668223129106)) ;
#43146=CARTESIAN_POINT('Ctrl Pts',(-8.13452843294813,16.6904255608455,-330.665399800544)) ;
#43147=CARTESIAN_POINT('Ctrl Pts',(-8.5713127002809,16.4712427019942,-330.6589448748)) ;
#43148=CARTESIAN_POINT('Ctrl Pts',(-8.81291808194992,16.3432466794557,-330.655301220707)) ;
#43149=CARTESIAN_POINT('Ctrl Pts',(-9.35769946137628,16.0390419219058,-330.646939039377)) ;
#43150=CARTESIAN_POINT('Ctrl Pts',(-9.65888775124047,15.8594858701113,-330.642208609274)) ;
#43151=CARTESIAN_POINT('Ctrl Pts',(-10.0345449264861,15.6208620217748,-330.636218394612)) ;
#43152=CARTESIAN_POINT('Ctrl Pts',(-10.1138912993197,15.5696058067745,-330.634947997204)) ;
#43153=CARTESIAN_POINT('Ctrl Pts',(-10.4618678354267,15.3410371631397,-330.629358139101)) ;
#43154=CARTESIAN_POINT('Ctrl Pts',(-10.7262523806301,15.1573615927871,-330.625061231587)) ;
#43155=CARTESIAN_POINT('Ctrl Pts',(-11.0646575803404,14.9089717355814,-330.619555972283)) ;
#43156=CARTESIAN_POINT('Ctrl Pts',(-11.1431273433813,14.8504140895884,-330.618279106394)) ;
#43157=CARTESIAN_POINT('Ctrl Pts',(-11.2740289729751,14.7511077164518,-330.616151125927)) ;
#43158=CARTESIAN_POINT('Ctrl Pts',(-11.3267119954395,14.7106935102792,-330.6152953378)) ;
#43159=CARTESIAN_POINT('Ctrl Pts',(-11.4428152845252,14.6206348775338,-330.613411318656)) ;
#43160=CARTESIAN_POINT('Ctrl Pts',(-11.506131481596,14.5708587327633,-330.612384957924)) ;
#43161=CARTESIAN_POINT('Ctrl Pts',(-11.7088004846587,14.4093853266332,-330.609099839252)) ;
#43162=CARTESIAN_POINT('Ctrl Pts',(-11.8468663500648,14.2960887015532,-330.606862069528)) ;
#43163=CARTESIAN_POINT('Ctrl Pts',(-12.1994926333109,13.998107423612,-330.601120024997)) ;
#43164=CARTESIAN_POINT('Ctrl Pts',(-12.4115023274802,13.8104758185935,-330.597641106901)) ;
#43165=CARTESIAN_POINT('Ctrl Pts',(-13.1403739580981,13.1350693645033,-330.585458849114)) ;
#43166=CARTESIAN_POINT('Ctrl Pts',(-13.6334491296713,12.6225409245384,-330.576787931616)) ;
#43167=CARTESIAN_POINT('Ctrl Pts',(-14.1970743797401,11.9650211676568,-330.565890419424)) ;
#43168=CARTESIAN_POINT('Ctrl Pts',(-14.2967337182456,11.8457611567692,-330.563923513226)) ;
#43169=CARTESIAN_POINT('Ctrl Pts',(-14.4747024500922,11.6272723275276,-330.560334483434)) ;
#43170=CARTESIAN_POINT('Ctrl Pts',(-14.5535182835272,11.5284681686224,-330.558716684917)) ;
#43171=CARTESIAN_POINT('Ctrl Pts',(-14.7129634481555,11.3243453046729,-330.555384018751)) ;
#43172=CARTESIAN_POINT('Ctrl Pts',(-14.7934854104544,11.2189517939363,-330.553668396983)) ;
#43173=CARTESIAN_POINT('Ctrl Pts',(-15.0014874186071,10.9405688843869,-330.549149662067)) ;
#43174=CARTESIAN_POINT('Ctrl Pts',(-15.1271054431131,10.7662134915783,-330.546332135851)) ;
#43175=CARTESIAN_POINT('Ctrl Pts',(-15.4051392015674,10.3658323904254,-330.539893979086)) ;
#43176=CARTESIAN_POINT('Ctrl Pts',(-15.5556604518152,10.1385513002385,-330.536261392284)) ;
#43177=CARTESIAN_POINT('Ctrl Pts',(-15.8887788265828,9.61066354740706,-330.527896443821)) ;
#43178=CARTESIAN_POINT('Ctrl Pts',(-16.0679484860358,9.30801684241158,-330.523151787894)) ;
#43179=CARTESIAN_POINT('Ctrl Pts',(-16.4345551275127,8.6465942956125,-330.512972881649)) ;
#43180=CARTESIAN_POINT('Ctrl Pts',(-16.6190757736095,8.28640553254775,-330.50754460659)) ;
#43181=CARTESIAN_POINT('Ctrl Pts',(-16.8359631109392,7.82659694602327,-330.500867992627)) ;
#43182=CARTESIAN_POINT('Ctrl Pts',(-16.8794570831303,7.73234778411225,-330.499512656652)) ;
#43183=CARTESIAN_POINT('Ctrl Pts',(-16.9495285523412,7.57709757966394,-330.497304656267)) ;
#43184=CARTESIAN_POINT('Ctrl Pts',(-16.976572543636,7.51630963893987,-330.496446285057)) ;
#43185=CARTESIAN_POINT('Ctrl Pts',(-17.0343102757226,7.3846286654148,-330.49460094204)) ;
#43186=CARTESIAN_POINT('Ctrl Pts',(-17.0648894297572,7.31368688606125,-330.493615351778)) ;
#43187=CARTESIAN_POINT('Ctrl Pts',(-17.1568918581588,7.09652822671324,-330.490621677507)) ;
#43188=CARTESIAN_POINT('Ctrl Pts',(-17.216885234924,6.94971323560982,-330.488629773962)) ;
#43189=CARTESIAN_POINT('Ctrl Pts',(-17.320615197322,6.68627671113947,-330.485099226433)) ;
#43190=CARTESIAN_POINT('Ctrl Pts',(-17.3650732086083,6.56994973935645,-330.483555222653)) ;
#43191=CARTESIAN_POINT('Ctrl Pts',(-17.5921832066087,5.95728908999621,-330.475484419714)) ;
#43192=CARTESIAN_POINT('Ctrl Pts',(-17.7547359256516,5.45376538662723,-330.469052942221)) ;
#43193=CARTESIAN_POINT('Ctrl Pts',(-17.9615360641349,4.7052188834405,-330.459493536434)) ;
#43194=CARTESIAN_POINT('Ctrl Pts',(-18.0227157703569,4.4651515706854,-330.456429312891)) ;
#43195=CARTESIAN_POINT('Ctrl Pts',(-18.1321167239935,3.99689883884166,-330.450430420117)) ;
#43196=CARTESIAN_POINT('Ctrl Pts',(-18.180878700416,3.76888665422343,-330.44749929868)) ;
#43197=CARTESIAN_POINT('Ctrl Pts',(-18.2512334933319,3.40667383168276,-330.442816414543)) ;
#43198=CARTESIAN_POINT('Ctrl Pts',(-18.2756693639819,3.27305054294396,-330.441083248898)) ;
#43199=CARTESIAN_POINT('Ctrl Pts',(-18.3199766457208,3.01477764874225,-330.437721076734)) ;
#43200=CARTESIAN_POINT('Ctrl Pts',(-18.3400476331296,2.89016977562543,-330.436093483044)) ;
#43201=CARTESIAN_POINT('Ctrl Pts',(-18.385101952996,2.59106107712134,-330.43217295651)) ;
#43202=CARTESIAN_POINT('Ctrl Pts',(-18.4088736582348,2.41639024584107,-330.429872336945)) ;
#43203=CARTESIAN_POINT('Ctrl Pts',(-18.4549308116001,2.03768160184106,-330.424861169367)) ;
#43204=CARTESIAN_POINT('Ctrl Pts',(-18.4763275208731,1.83355902970655,-330.422145656844)) ;
#43205=CARTESIAN_POINT('Ctrl Pts',(-18.5332057502782,1.18785921698701,-330.41351900801)) ;
#43206=CARTESIAN_POINT('Ctrl Pts',(-18.556270749547,0.745345250572032,-330.407549723034)) ;
#43207=CARTESIAN_POINT('Ctrl Pts',(-18.5661659217633,0.137972571028798,
-330.39936793353)) ;
#43208=CARTESIAN_POINT('Ctrl Pts',(-18.5666596468405,-0.0265151922384639,
-330.39715378097)) ;
#43209=CARTESIAN_POINT('Ctrl Pts',(-18.5617637765965,-0.502418275354446,
-330.390766967386)) ;
#43210=CARTESIAN_POINT('Ctrl Pts',(-18.5507239721748,-0.813719501713166,
-330.386612423732)) ;
#43211=CARTESIAN_POINT('Ctrl Pts',(-18.5260150512544,-1.22089003075575,
-330.381264624084)) ;
#43212=CARTESIAN_POINT('Ctrl Pts',(-18.519421025374,-1.31713745310965,-330.380006904576)) ;
#43213=CARTESIAN_POINT('Ctrl Pts',(-18.5070346377355,-1.47937691227361,
-330.377900100957)) ;
#43214=CARTESIAN_POINT('Ctrl Pts',(-18.5016387044778,-1.54539716995087,
-330.377046573637)) ;
#43215=CARTESIAN_POINT('Ctrl Pts',(-18.4888248747068,-1.69247737064019,
-330.375154013099)) ;
#43216=CARTESIAN_POINT('Ctrl Pts',(-18.4812269988148,-1.77352009874664,
-330.374117000095)) ;
#43217=CARTESIAN_POINT('Ctrl Pts',(-18.4547007146308,-2.03775298220845,
-330.370751393486)) ;
#43218=CARTESIAN_POINT('Ctrl Pts',(-18.43357950976,-2.22071212794997,-330.36844522484)) ;
#43219=CARTESIAN_POINT('Ctrl Pts',(-18.3712162345436,-2.69842144769139,
-330.362457231648)) ;
#43220=CARTESIAN_POINT('Ctrl Pts',(-18.3256029734356,-2.99254746964278,
-330.358803398109)) ;
#43221=CARTESIAN_POINT('Ctrl Pts',(-18.152853151092,-3.95334343820715,-330.346840201097)) ;
#43222=CARTESIAN_POINT('Ctrl Pts',(-17.9962387990633,-4.6141510789431,-330.338550169864)) ;
#43223=CARTESIAN_POINT('Ctrl Pts',(-17.7537576672823,-5.43412654378801,
-330.327798057687)) ;
#43224=CARTESIAN_POINT('Ctrl Pts',(-17.7013031497934,-5.60263413637229,
-330.325564522393)) ;
#43225=CARTESIAN_POINT('Ctrl Pts',(-17.6072185883051,-5.89035562974297,
-330.321705540435)) ;
#43226=CARTESIAN_POINT('Ctrl Pts',(-17.5667600813921,-6.00993977097595,
-330.320088106029)) ;
#43227=CARTESIAN_POINT('Ctrl Pts',(-17.4802659474733,-6.25725448271785,
-330.316713889588)) ;
#43228=CARTESIAN_POINT('Ctrl Pts',(-17.4340424561258,-6.3849114972118,-330.314955897886)) ;
#43229=CARTESIAN_POINT('Ctrl Pts',(-17.3047896226676,-6.73000167159116,
-330.310158767569)) ;
#43230=CARTESIAN_POINT('Ctrl Pts',(-17.2190653054668,-6.94639878461507,
-330.307101672136)) ;
#43231=CARTESIAN_POINT('Ctrl Pts',(-17.0662084342514,-7.31202987185582,
-330.301856478411)) ;
#43232=CARTESIAN_POINT('Ctrl Pts',(-17.0011300618483,-7.46209271586618,
-330.299680484895)) ;
#43233=CARTESIAN_POINT('Ctrl Pts',(-16.6818399371303,-8.17247081362076,
-330.289277685478)) ;
#43234=CARTESIAN_POINT('Ctrl Pts',(-16.4018621393915,-8.72077856422216,
-330.280929701705)) ;
#43235=CARTESIAN_POINT('Ctrl Pts',(-16.0733130669516,-9.29220270212986,
-330.272116864638)) ;
#43236=CARTESIAN_POINT('Ctrl Pts',(-16.0513112420454,-9.33015709506135,
-330.271531033282)) ;
#43237=CARTESIAN_POINT('Ctrl Pts',(-15.9224575611999,-9.55063221266623,
-330.268125851353)) ;
#43238=CARTESIAN_POINT('Ctrl Pts',(-15.8126274595549,-9.7313947390057,-330.265325370099)) ;
#43239=CARTESIAN_POINT('Ctrl Pts',(-15.6538431031587,-9.98293976836074,
-330.261435821128)) ;
#43240=CARTESIAN_POINT('Ctrl Pts',(-15.6074488623538,-10.055318510847,-330.26031757548)) ;
#43241=CARTESIAN_POINT('Ctrl Pts',(-15.5246894087672,-10.1824771507967,
-330.258356467414)) ;
#43242=CARTESIAN_POINT('Ctrl Pts',(-15.4885329145412,-10.2373907971327,
-330.257510857388)) ;
#43243=CARTESIAN_POINT('Ctrl Pts',(-15.402977510373,-10.3658396011438,-330.255535795351)) ;
#43244=CARTESIAN_POINT('Ctrl Pts',(-15.3533425793521,-10.439215415613,-330.254409568327)) ;
#43245=CARTESIAN_POINT('Ctrl Pts',(-15.1679775989655,-10.7090605002199,
-330.250270245683)) ;
#43246=CARTESIAN_POINT('Ctrl Pts',(-15.0289857881028,-10.9032613399288,
-330.247295892746)) ;
#43247=CARTESIAN_POINT('Ctrl Pts',(-14.5998346278338,-11.4790724443462,
-330.238417635867)) ;
#43248=CARTESIAN_POINT('Ctrl Pts',(-14.2986049567674,-11.8521800859017,
-330.232580318352)) ;
#43249=CARTESIAN_POINT('Ctrl Pts',(-13.6866204068814,-12.5528596604249,
-330.221153965526)) ;
#43250=CARTESIAN_POINT('Ctrl Pts',(-13.3776906313024,-12.8815859226233,
-330.215574760798)) ;
#43251=CARTESIAN_POINT('Ctrl Pts',(-12.9408872331305,-13.3137019414541,
-330.207832918695)) ;
#43252=CARTESIAN_POINT('Ctrl Pts',(-12.8231616266427,-13.4271273008815,
-330.20576051094)) ;
#43253=CARTESIAN_POINT('Ctrl Pts',(-12.6128424213714,-13.6244748728398,
-330.202079650693)) ;
#43254=CARTESIAN_POINT('Ctrl Pts',(-12.5208706443765,-13.7090447428699,
-330.200477086502)) ;
#43255=CARTESIAN_POINT('Ctrl Pts',(-12.3415802175801,-13.8705964389887,
-330.197365757672)) ;
#43256=CARTESIAN_POINT('Ctrl Pts',(-12.2543773493398,-13.9476981462261,
-330.195858143505)) ;
#43257=CARTESIAN_POINT('Ctrl Pts',(-12.0613442653694,-14.1151633935476,
-330.192533040218)) ;
#43258=CARTESIAN_POINT('Ctrl Pts',(-11.9552114711779,-14.2051674303664,
-330.19071268553)) ;
#43259=CARTESIAN_POINT('Ctrl Pts',(-11.507816985023,-14.5760066319688,-330.183072911309)) ;
#43260=CARTESIAN_POINT('Ctrl Pts',(-11.1575957720371,-14.8458033078795,
-330.177169594897)) ;
#43261=CARTESIAN_POINT('Ctrl Pts',(-10.2802959771581,-15.4730464530979,
-330.162670534322)) ;
#43262=CARTESIAN_POINT('Ctrl Pts',(-9.74381415641788,-15.8163756113584,
-330.154035235311)) ;
#43263=CARTESIAN_POINT('Ctrl Pts',(-9.09445342691111,-16.1863430845461,
-330.14420122367)) ;
#43264=CARTESIAN_POINT('Ctrl Pts',(-8.99765519925968,-16.2403505675189,
-330.142751260244)) ;
#43265=CARTESIAN_POINT('Ctrl Pts',(-8.84060289792843,-16.3261409772042,
-330.140427907386)) ;
#43266=CARTESIAN_POINT('Ctrl Pts',(-8.78064740648805,-16.3584647800832,
-330.139547754509)) ;
#43267=CARTESIAN_POINT('Ctrl Pts',(-8.66699183473694,-16.4189350337465,
-330.137893068336)) ;
#43268=CARTESIAN_POINT('Ctrl Pts',(-8.61332917160136,-16.4471497742988,
-330.137117508219)) ;
#43269=CARTESIAN_POINT('Ctrl Pts',(-8.51851504977828,-16.4964098206519,
-330.135756444397)) ;
#43270=CARTESIAN_POINT('Ctrl Pts',(-8.47742141704833,-16.5175652487354,
-330.135169581176)) ;
#43271=CARTESIAN_POINT('Ctrl Pts',(-8.25302042359775,-16.6320311936333,
-330.131980365758)) ;
#43272=CARTESIAN_POINT('Ctrl Pts',(-8.06825073589355,-16.7224441421848,
-330.129410400277)) ;
#43273=CARTESIAN_POINT('Ctrl Pts',(-7.55652235598144,-16.9623910329631,
-330.122401888033)) ;
#43274=CARTESIAN_POINT('Ctrl Pts',(-7.22666328815681,-17.1055277045896,
-330.118003464492)) ;
#43275=CARTESIAN_POINT('Ctrl Pts',(-6.77224408864678,-17.2872231012085,
-330.112009214102)) ;
#43276=CARTESIAN_POINT('Ctrl Pts',(-6.65112866273107,-17.334181839662,-330.110417930318)) ;
#43277=CARTESIAN_POINT('Ctrl Pts',(-6.08298750655138,-17.5476296909381,
-330.102970501915)) ;
#43278=CARTESIAN_POINT('Ctrl Pts',(-5.63014569610861,-17.6981214484734,
-330.097078592974)) ;
#43279=CARTESIAN_POINT('Ctrl Pts',(-5.02651697669581,-17.8732083462247,
-330.089163627025)) ;
#43280=CARTESIAN_POINT('Ctrl Pts',(-4.88051007119133,-17.9136280764974,
-330.087245015188)) ;
#43281=CARTESIAN_POINT('Ctrl Pts',(-4.6126268096025,-17.9842691166204,-330.083714699708)) ;
#43282=CARTESIAN_POINT('Ctrl Pts',(-4.49090713243562,-18.0150496757352,
-330.082106811078)) ;
#43283=CARTESIAN_POINT('Ctrl Pts',(-4.25599254292782,-18.0719262563996,
-330.078995453635)) ;
#43284=CARTESIAN_POINT('Ctrl Pts',(-4.14284643128943,-18.0981992073007,
-330.077493245856)) ;
#43285=CARTESIAN_POINT('Ctrl Pts',(-3.89958097867066,-18.1522855413034,
-330.074255462553)) ;
#43286=CARTESIAN_POINT('Ctrl Pts',(-3.76939409285071,-18.1797654081152,
-330.072517815642)) ;
#43287=CARTESIAN_POINT('Ctrl Pts',(-3.44614278234465,-18.2443758006867,
-330.068191690622)) ;
#43288=CARTESIAN_POINT('Ctrl Pts',(-3.25276274937905,-18.279843619488,-330.065593379781)) ;
#43289=CARTESIAN_POINT('Ctrl Pts',(-2.59873184162833,-18.3890922535926,
-330.056779016735)) ;
#43290=CARTESIAN_POINT('Ctrl Pts',(-2.1358748411174,-18.4485814695994,-330.05049265788)) ;
#43291=CARTESIAN_POINT('Ctrl Pts',(-1.25835765446653,-18.5278958790408,
-330.038625383331)) ;
#43292=CARTESIAN_POINT('Ctrl Pts',(-0.844309466275273,-18.5513754769053,
-330.033048159475)) ;
#43293=CARTESIAN_POINT('Ctrl Pts',(-0.347385170617471,-18.5628829276712,
-330.026490566988)) ;
#43294=CARTESIAN_POINT('Ctrl Pts',(-0.264935466496756,-18.5642427333547,
-330.025407121129)) ;
#43295=CARTESIAN_POINT('Ctrl Pts',(-0.121638931265175,-18.5656512218572,
-330.023533604446)) ;
#43296=CARTESIAN_POINT('Ctrl Pts',(-0.0607958602491681,-18.5659501559856,
-330.022741094051)) ;
#43297=CARTESIAN_POINT('Ctrl Pts',(4.7616526672392E-5,-18.5659499999389,
-330.021951923812)) ;
#43298=CARTESIAN_POINT('Ctrl Pts',(4.7616526672392E-5,-18.5659499999389,
-330.021951923812)) ;
#43299=CARTESIAN_POINT('Ctrl Pts',(0.0581026652593616,-18.5659498510438,
-330.021198920875)) ;
#43300=CARTESIAN_POINT('Ctrl Pts',(0.116157458008613,-18.5656773981162,
-330.020448967975)) ;
#43301=CARTESIAN_POINT('Ctrl Pts',(0.238776255328645,-18.5645267771815,
-330.018872109095)) ;
#43302=CARTESIAN_POINT('Ctrl Pts',(0.303338885232825,-18.5635840853691,
-330.018045992598)) ;
#43303=CARTESIAN_POINT('Ctrl Pts',(0.482556376936524,-18.5600320868817,
-330.015762822773)) ;
#43304=CARTESIAN_POINT('Ctrl Pts',(0.5971940506329,-18.5566972020742,-330.014313757867)) ;
#43305=CARTESIAN_POINT('Ctrl Pts',(1.14093747068827,-18.5358354727858,-330.007480944841)) ;
#43306=CARTESIAN_POINT('Ctrl Pts',(1.56938204509395,-18.5044853166008,-330.002213255011)) ;
#43307=CARTESIAN_POINT('Ctrl Pts',(2.44542892588963,-18.4097366682375,-329.991418195119)) ;
#43308=CARTESIAN_POINT('Ctrl Pts',(2.89258184393477,-18.3447948133597,-329.985894367478)) ;
#43309=CARTESIAN_POINT('Ctrl Pts',(3.61850126273996,-18.2121630512013,-329.976739501948)) ;
#43310=CARTESIAN_POINT('Ctrl Pts',(3.89885481970043,-18.1542106685303,-329.973158524709)) ;
#43311=CARTESIAN_POINT('Ctrl Pts',(4.29470509939096,-18.0627908734934,-329.968016979546)) ;
#43312=CARTESIAN_POINT('Ctrl Pts',(4.41138966644285,-18.0346485188035,-329.966490890444)) ;
#43313=CARTESIAN_POINT('Ctrl Pts',(4.64822465796194,-17.9750918739856,-329.963370685704)) ;
#43314=CARTESIAN_POINT('Ctrl Pts',(4.76834929538207,-17.9435995635043,-329.961776120625)) ;
#43315=CARTESIAN_POINT('Ctrl Pts',(5.02813844237762,-17.8726992907168,-329.958300786899)) ;
#43316=CARTESIAN_POINT('Ctrl Pts',(5.16767517679351,-17.8328542112097,-329.956417181022)) ;
#43317=CARTESIAN_POINT('Ctrl Pts',(5.58452383535151,-17.7085185091262,-329.950739043784)) ;
#43318=CARTESIAN_POINT('Ctrl Pts',(5.86033803906599,-17.6191648989292,-329.946913172611)) ;
#43319=CARTESIAN_POINT('Ctrl Pts',(6.72237998229648,-17.3174128455323,-329.934758298425)) ;
#43320=CARTESIAN_POINT('Ctrl Pts',(7.30006480442918,-17.0819270201348,-329.926308519757)) ;
#43321=CARTESIAN_POINT('Ctrl Pts',(8.05186736080542,-16.7303489825553,-329.915177829223)) ;
#43322=CARTESIAN_POINT('Ctrl Pts',(8.23745903168308,-16.6397540236598,-329.912420321007)) ;
#43323=CARTESIAN_POINT('Ctrl Pts',(8.55107951538355,-16.4801298182743,-329.907764321705)) ;
#43324=CARTESIAN_POINT('Ctrl Pts',(8.6798791879029,-16.4126578317965,-329.905853311936)) ;
#43325=CARTESIAN_POINT('Ctrl Pts',(8.86300255001428,-16.3139696930125,-329.903144822235)) ;
#43326=CARTESIAN_POINT('Ctrl Pts',(8.91798132454375,-16.2839807925675,-329.902332775988)) ;
#43327=CARTESIAN_POINT('Ctrl Pts',(9.01563574848838,-16.2300710019763,-329.900893132544)) ;
#43328=CARTESIAN_POINT('Ctrl Pts',(9.05837042646113,-16.206258602737,-329.900264126856)) ;
#43329=CARTESIAN_POINT('Ctrl Pts',(9.17226394750052,-16.1422041985057,-329.898590273108)) ;
#43330=CARTESIAN_POINT('Ctrl Pts',(9.24325189405584,-16.1016606831915,-329.897549499824)) ;
#43331=CARTESIAN_POINT('Ctrl Pts',(9.46753213888617,-15.9715949959989,-329.894265852192)) ;
#43332=CARTESIAN_POINT('Ctrl Pts',(9.61980960301441,-15.8803424053068,-329.892043158918)) ;
#43333=CARTESIAN_POINT('Ctrl Pts',(10.3521323389,-15.4270971778075,-329.881337231818)) ;
#43334=CARTESIAN_POINT('Ctrl Pts',(10.9131900849732,-15.0354334319154,-329.873063366174)) ;
#43335=CARTESIAN_POINT('Ctrl Pts',(11.6438500729911,-14.4628854509154,-329.861603724857)) ;
#43336=CARTESIAN_POINT('Ctrl Pts',(11.8333358846869,-14.3082655017375,-329.858567017114)) ;
#43337=CARTESIAN_POINT('Ctrl Pts',(12.0306921794034,-14.1406206601484,-329.855322535427)) ;
#43338=CARTESIAN_POINT('Ctrl Pts',(12.041661690836,-14.1312805751333,-329.855141929022)) ;
#43339=CARTESIAN_POINT('Ctrl Pts',(12.0836251204874,-14.0954661102493,-329.854449981767)) ;
#43340=CARTESIAN_POINT('Ctrl Pts',(12.1145426859745,-14.0689024598871,-329.853937986846)) ;
#43341=CARTESIAN_POINT('Ctrl Pts',(12.1575910910589,-14.0316691538331,-329.853221990606)) ;
#43342=CARTESIAN_POINT('Ctrl Pts',(12.1697958698784,-14.0210851529195,-329.853018645106)) ;
#43343=CARTESIAN_POINT('Ctrl Pts',(12.2028188356677,-13.9923719908037,-329.852467486175)) ;
#43344=CARTESIAN_POINT('Ctrl Pts',(12.2236104255492,-13.9742123079998,-329.852119436267)) ;
#43345=CARTESIAN_POINT('Ctrl Pts',(12.2585847206205,-13.9435274616503,-329.851532203737)) ;
#43346=CARTESIAN_POINT('Ctrl Pts',(12.2727889219539,-13.9310268646438,-329.85129321652)) ;
#43347=CARTESIAN_POINT('Ctrl Pts',(12.2966591671877,-13.9099546955302,-329.850890761112)) ;
#43348=CARTESIAN_POINT('Ctrl Pts',(12.3063354200097,-13.9013947082963,-329.850727386348)) ;
#43349=CARTESIAN_POINT('Ctrl Pts',(12.3226114437513,-13.886965997204,-329.850452188024)) ;
#43350=CARTESIAN_POINT('Ctrl Pts',(12.3292159764595,-13.8811026509773,-329.850340408218)) ;
#43351=CARTESIAN_POINT('Ctrl Pts',(12.3403420934771,-13.871210945365,-329.850151917511)) ;
#43352=CARTESIAN_POINT('Ctrl Pts',(12.3448658953132,-13.8671850821132,-329.850075227037)) ;
#43353=CARTESIAN_POINT('Ctrl Pts',(12.352498368207,-13.8603860271048,-329.849945749256)) ;
#43354=CARTESIAN_POINT('Ctrl Pts',(12.3556080771553,-13.8576140009978,-329.849892971526)) ;
#43355=CARTESIAN_POINT('Ctrl Pts',(12.3682870472663,-13.8463041777819,-329.849677685319)) ;
#43356=CARTESIAN_POINT('Ctrl Pts',(12.3778483932976,-13.837757514125,-329.849515103857)) ;
#43357=CARTESIAN_POINT('Ctrl Pts',(12.3958108145418,-13.8216678128162,-329.849209232247)) ;
#43358=CARTESIAN_POINT('Ctrl Pts',(12.4042138795492,-13.8141270049219,-329.84906596065)) ;
#43359=CARTESIAN_POINT('Ctrl Pts',(12.4200538272188,-13.7998863229697,-329.848795548557)) ;
#43360=CARTESIAN_POINT('Ctrl Pts',(12.4274921805692,-13.7931880904947,-329.848668421808)) ;
#43361=CARTESIAN_POINT('Ctrl Pts',(12.44156817291,-13.7804920388692,-329.848427581942)) ;
#43362=CARTESIAN_POINT('Ctrl Pts',(12.4482069009987,-13.7744954312095,-329.848313879026)) ;
#43363=CARTESIAN_POINT('Ctrl Pts',(12.4608243461033,-13.7630818172029,-329.848097559047)) ;
#43364=CARTESIAN_POINT('Ctrl Pts',(12.4668038715921,-13.7576657074776,-329.847994949569)) ;
#43365=CARTESIAN_POINT('Ctrl Pts',(12.5589035044516,-13.6741347357994,-329.846413063903)) ;
#43366=CARTESIAN_POINT('Ctrl Pts',(12.6442914143989,-13.5952165335229,-329.844926974883)) ;
#43367=CARTESIAN_POINT('Ctrl Pts',(12.8209046404516,-13.4288817663955,-329.841811320343)) ;
#43368=CARTESIAN_POINT('Ctrl Pts',(12.9119903220531,-13.3413255400172,-329.840180553971)) ;
#43369=CARTESIAN_POINT('Ctrl Pts',(13.1345664331528,-13.1229593516729,-329.836135505242)) ;
#43370=CARTESIAN_POINT('Ctrl Pts',(13.2650038142331,-12.9910958420024,-329.833711871784)) ;
#43371=CARTESIAN_POINT('Ctrl Pts',(13.8012711460205,-12.4324664276529,-329.823525269086)) ;
#43372=CARTESIAN_POINT('Ctrl Pts',(14.1886518877783,-11.9884688715057,-329.815609336336)) ;
#43373=CARTESIAN_POINT('Ctrl Pts',(14.8664346895102,-11.1326729274872,-329.800903558876)) ;
#43374=CARTESIAN_POINT('Ctrl Pts',(15.162494743099,-10.7259552186097,-329.794126680316)) ;
#43375=CARTESIAN_POINT('Ctrl Pts',(15.4983300701611,-10.2228507244519,-329.786185897481)) ;
#43376=CARTESIAN_POINT('Ctrl Pts',(15.5542824790199,-10.1375149078137,-329.784853978497)) ;
#43377=CARTESIAN_POINT('Ctrl Pts',(15.6457670103106,-9.99544667370517,-329.782664115815)) ;
#43378=CARTESIAN_POINT('Ctrl Pts',(15.6817008837568,-9.93897565042121,-329.781800834034)) ;
#43379=CARTESIAN_POINT('Ctrl Pts',(15.759047724917,-9.81595931507566,-329.779936507707)) ;
#43380=CARTESIAN_POINT('Ctrl Pts',(15.8003461959506,-9.7493437000599,-329.778936946909)) ;
#43381=CARTESIAN_POINT('Ctrl Pts',(15.9273908721902,-9.54148938379758,-329.775846126354)) ;
#43382=CARTESIAN_POINT('Ctrl Pts',(16.0116744449906,-9.39936600444508,-329.773772581667)) ;
#43383=CARTESIAN_POINT('Ctrl Pts',(16.2439874308812,-8.99543324050806,-329.767967151885)) ;
#43384=CARTESIAN_POINT('Ctrl Pts',(16.3875685923579,-8.73112495555433,-329.764270297603)) ;
#43385=CARTESIAN_POINT('Ctrl Pts',(16.6855842090126,-8.14925691006487,-329.756255354711)) ;
#43386=CARTESIAN_POINT('Ctrl Pts',(16.837509005625,-7.83054270386208,-329.751942058568)) ;
#43387=CARTESIAN_POINT('Ctrl Pts',(17.0900461926661,-7.25937569696008,-329.744251505353)) ;
#43388=CARTESIAN_POINT('Ctrl Pts',(17.1943769443528,-7.00868144164467,-329.740889332834)) ;
#43389=CARTESIAN_POINT('Ctrl Pts',(17.3711546394092,-6.55617371373322,-329.734814665826)) ;
#43390=CARTESIAN_POINT('Ctrl Pts',(17.4456748971035,-6.35522261017884,-329.732115110044)) ;
#43391=CARTESIAN_POINT('Ctrl Pts',(17.5606215531586,-6.02798756042791,-329.727707933453)) ;
#43392=CARTESIAN_POINT('Ctrl Pts',(17.6032034765254,-5.90248173779442,-329.726015070028)) ;
#43393=CARTESIAN_POINT('Ctrl Pts',(17.683780503254,-5.65635886994195,-329.722689034744)) ;
#43394=CARTESIAN_POINT('Ctrl Pts',(17.7218943056158,-5.53578817508473,-329.721056777729)) ;
#43395=CARTESIAN_POINT('Ctrl Pts',(17.8041825674143,-5.26591146070652,-329.717396328597)) ;
#43396=CARTESIAN_POINT('Ctrl Pts',(17.847716531822,-5.11642012616933,-329.715364004563)) ;
#43397=CARTESIAN_POINT('Ctrl Pts',(18.0789428804612,-4.28352440615334,-329.704016506059)) ;
#43398=CARTESIAN_POINT('Ctrl Pts',(18.2292645469026,-3.59035695091203,-329.694456307325)) ;
#43399=CARTESIAN_POINT('Ctrl Pts',(18.3837779290755,-2.60993597128431,-329.681095997685)) ;
#43400=CARTESIAN_POINT('Ctrl Pts',(18.4215284173503,-2.32859352472789,-329.677284112108)) ;
#43401=CARTESIAN_POINT('Ctrl Pts',(18.4725323277506,-1.8687023086486,-329.671135910529)) ;
#43402=CARTESIAN_POINT('Ctrl Pts',(18.4896798658008,-1.69063229974774,-329.668775609301)) ;
#43403=CARTESIAN_POINT('Ctrl Pts',(18.5108156395543,-1.43202569187897,-329.665389853047)) ;
#43404=CARTESIAN_POINT('Ctrl Pts',(18.5168568829587,-1.3516672756189,-329.664343667278)) ;
#43405=CARTESIAN_POINT('Ctrl Pts',(18.5269206635785,-1.20503845468096,-329.662447035533)) ;
#43406=CARTESIAN_POINT('Ctrl Pts',(18.5311112587994,-1.13878112914995,-329.661594751771)) ;
#43407=CARTESIAN_POINT('Ctrl Pts',(18.5384852197741,-1.01134464217916,-329.659963993967)) ;
#43408=CARTESIAN_POINT('Ctrl Pts',(18.5417213276837,-0.950169664203256,
-329.659184854324)) ;
#43409=CARTESIAN_POINT('Ctrl Pts',(18.5446545937457,-0.888979977932787,
-329.658408769442)) ;
#43410=CARTESIAN_POINT('',(0.00032989125932316,-18.5659499970691,-329.726459838768)) ;
#43411=CARTESIAN_POINT('Ctrl Pts',(18.5446545934183,-0.888979984762294,
-329.363119887734)) ;
#43412=CARTESIAN_POINT('Ctrl Pts',(18.5408622451644,-0.96809063930157,-329.364098153425)) ;
#43413=CARTESIAN_POINT('Ctrl Pts',(18.5365634497327,-1.04718169001174,-329.365078387839)) ;
#43414=CARTESIAN_POINT('Ctrl Pts',(18.5141807712173,-1.41547560454857,-329.369655233095)) ;
#43415=CARTESIAN_POINT('Ctrl Pts',(18.4898347200062,-1.70425125395901,-329.373279960535)) ;
#43416=CARTESIAN_POINT('Ctrl Pts',(18.4431703167598,-2.13659056960382,-329.37878366536)) ;
#43417=CARTESIAN_POINT('Ctrl Pts',(18.4259100571044,-2.28065540668142,-329.380630363209)) ;
#43418=CARTESIAN_POINT('Ctrl Pts',(18.3907460732578,-2.54762235048005,-329.384078074143)) ;
#43419=CARTESIAN_POINT('Ctrl Pts',(18.3732943572848,-2.67057581453395,-329.385676047891)) ;
#43420=CARTESIAN_POINT('Ctrl Pts',(18.3308417048764,-2.949525227007,-329.389325115095)) ;
#43421=CARTESIAN_POINT('Ctrl Pts',(18.3050805528528,-3.10539571131417,-329.391381048006)) ;
#43422=CARTESIAN_POINT('Ctrl Pts',(18.2081303414711,-3.64879827313908,-329.398607346969)) ;
#43423=CARTESIAN_POINT('Ctrl Pts',(18.1265978036808,-4.03437604046755,-329.403842006204)) ;
#43424=CARTESIAN_POINT('Ctrl Pts',(17.9485203504936,-4.7613847840793,-329.413870855483)) ;
#43425=CARTESIAN_POINT('Ctrl Pts',(17.8543368150823,-5.10321706153174,-329.418654063231)) ;
#43426=CARTESIAN_POINT('Ctrl Pts',(17.6323803865769,-5.82716373825359,-329.428846450934)) ;
#43427=CARTESIAN_POINT('Ctrl Pts',(17.5018397243408,-6.20824311980329,-329.434250036758)) ;
#43428=CARTESIAN_POINT('Ctrl Pts',(17.3215687159364,-6.68347970674238,-329.440927766862)) ;
#43429=CARTESIAN_POINT('Ctrl Pts',(17.2832861438352,-6.78186286289523,-329.442306665114)) ;
#43430=CARTESIAN_POINT('Ctrl Pts',(17.2194123042543,-6.94195949883317,-329.444541639566)) ;
#43431=CARTESIAN_POINT('Ctrl Pts',(17.1943233599385,-7.00387078842446,-329.445403710302)) ;
#43432=CARTESIAN_POINT('Ctrl Pts',(17.1397825667695,-7.13640014674348,-329.447243459347)) ;
#43433=CARTESIAN_POINT('Ctrl Pts',(17.1102272531836,-7.20697418172087,-329.448219892867)) ;
#43434=CARTESIAN_POINT('Ctrl Pts',(17.0197339364188,-7.41936528193663,-329.451151262843)) ;
#43435=CARTESIAN_POINT('Ctrl Pts',(16.9574627643747,-7.5606071966991,-329.453090967853)) ;
#43436=CARTESIAN_POINT('Ctrl Pts',(16.8438312279553,-7.80987524298405,-329.456509141171)) ;
#43437=CARTESIAN_POINT('Ctrl Pts',(16.7931746230104,-7.91821241632929,-329.457993013658)) ;
#43438=CARTESIAN_POINT('Ctrl Pts',(16.5307112216416,-8.46568258809532,-329.465497704621)) ;
#43439=CARTESIAN_POINT('Ctrl Pts',(16.3027122899162,-8.89684035838738,-329.471433302715)) ;
#43440=CARTESIAN_POINT('Ctrl Pts',(15.8350492080014,-9.70273384665809,-329.482881216423)) ;
#43441=CARTESIAN_POINT('Ctrl Pts',(15.5983736394179,-10.0788176905777,-329.488380041022)) ;
#43442=CARTESIAN_POINT('Ctrl Pts',(15.2573006164766,-10.5799581722552,-329.496020389316)) ;
#43443=CARTESIAN_POINT('Ctrl Pts',(15.1644146667849,-10.71266842273,-329.498074432208)) ;
#43444=CARTESIAN_POINT('Ctrl Pts',(14.9969256411102,-10.9454232012221,-329.501734853121)) ;
#43445=CARTESIAN_POINT('Ctrl Pts',(14.9230281291423,-11.0459630247471,-329.503335572336)) ;
#43446=CARTESIAN_POINT('Ctrl Pts',(14.7635751202562,-11.2583828097293,-329.506760399129)) ;
#43447=CARTESIAN_POINT('Ctrl Pts',(14.6777486453076,-11.3700496240256,-329.508586635772)) ;
#43448=CARTESIAN_POINT('Ctrl Pts',(14.4282213567211,-11.6871695425115,-329.513847846711)) ;
#43449=CARTESIAN_POINT('Ctrl Pts',(14.2614199290215,-11.8901389645837,-329.517307393516)) ;
#43450=CARTESIAN_POINT('Ctrl Pts',(13.8478150729277,-12.3721973315111,-329.525740166454)) ;
#43451=CARTESIAN_POINT('Ctrl Pts',(13.5968094094343,-12.6475302784091,-329.530740737127)) ;
#43452=CARTESIAN_POINT('Ctrl Pts',(12.9525789206509,-13.3128391874652,-329.543210139689)) ;
#43453=CARTESIAN_POINT('Ctrl Pts',(12.5498690664016,-13.6931287579334,-329.550695420131)) ;
#43454=CARTESIAN_POINT('Ctrl Pts',(12.0443866403451,-14.129411549508,-329.559483518768)) ;
#43455=CARTESIAN_POINT('Ctrl Pts',(11.9573178130261,-14.2031711619817,-329.560976326904)) ;
#43456=CARTESIAN_POINT('Ctrl Pts',(11.8217686141987,-14.3158706151252,-329.563264572234)) ;
#43457=CARTESIAN_POINT('Ctrl Pts',(11.7737633769682,-14.3553774103229,-329.564068139585)) ;
#43458=CARTESIAN_POINT('Ctrl Pts',(11.6852601174995,-14.4274702281463,-329.56553638596)) ;
#43459=CARTESIAN_POINT('Ctrl Pts',(11.6448219553146,-14.4601287281136,-329.566202234305)) ;
#43460=CARTESIAN_POINT('Ctrl Pts',(11.6027696879068,-14.4938000039432,-329.566889777625)) ;
#43461=CARTESIAN_POINT('Ctrl Pts',(11.6012920412161,-14.4949827857548,-329.566913930527)) ;
#43462=CARTESIAN_POINT('Ctrl Pts',(11.5985031978816,-14.4972144148642,-329.566959503895)) ;
#43463=CARTESIAN_POINT('Ctrl Pts',(11.5971920397567,-14.498263310301,-329.566980925055)) ;
#43464=CARTESIAN_POINT('Ctrl Pts',(11.5947213763297,-14.5002392329097,-329.567021280542)) ;
#43465=CARTESIAN_POINT('Ctrl Pts',(11.593561902115,-14.5011662988934,-329.567040215427)) ;
#43466=CARTESIAN_POINT('Ctrl Pts',(11.591380316082,-14.5029101728699,-329.567075834827)) ;
#43467=CARTESIAN_POINT('Ctrl Pts',(11.5903582291015,-14.503727011892,-329.567092519788)) ;
#43468=CARTESIAN_POINT('Ctrl Pts',(11.5884377861092,-14.5052614730656,-329.567123864329)) ;
#43469=CARTESIAN_POINT('Ctrl Pts',(11.5875394497845,-14.5059791198048,-329.567138524261)) ;
#43470=CARTESIAN_POINT('Ctrl Pts',(11.5858536540197,-14.5073255814309,-329.567166030456)) ;
#43471=CARTESIAN_POINT('Ctrl Pts',(11.5850662100155,-14.5079544156838,-329.567178876995)) ;
#43472=CARTESIAN_POINT('Ctrl Pts',(11.5835902053199,-14.5091329215075,-329.567202953596)) ;
#43473=CARTESIAN_POINT('Ctrl Pts',(11.5829016567055,-14.5096826081705,-329.567214183872)) ;
#43474=CARTESIAN_POINT('Ctrl Pts',(11.5816123601113,-14.5107117376571,-329.567235209894)) ;
#43475=CARTESIAN_POINT('Ctrl Pts',(11.5810116214779,-14.5111911921957,-329.567245005806)) ;
#43476=CARTESIAN_POINT('Ctrl Pts',(11.5798877933608,-14.5120880145999,-329.567263329552)) ;
#43477=CARTESIAN_POINT('Ctrl Pts',(11.5793647110713,-14.5125053914999,-329.567271857514)) ;
#43478=CARTESIAN_POINT('Ctrl Pts',(11.577465670889,-14.5140205022649,-329.567302815329)) ;
#43479=CARTESIAN_POINT('Ctrl Pts',(11.5760895794684,-14.5151180687207,-329.567325242815)) ;
#43480=CARTESIAN_POINT('Ctrl Pts',(11.5733669855694,-14.517288968156,-329.567369605065)) ;
#43481=CARTESIAN_POINT('Ctrl Pts',(11.5720204897817,-14.5183623095612,-329.567391539946)) ;
#43482=CARTESIAN_POINT('Ctrl Pts',(11.5693572559227,-14.5204846655185,-329.567434914938)) ;
#43483=CARTESIAN_POINT('Ctrl Pts',(11.5680405245102,-14.5215336882859,-329.567456355163)) ;
#43484=CARTESIAN_POINT('Ctrl Pts',(11.4845382318516,-14.5880403127953,-329.56881570979)) ;
#43485=CARTESIAN_POINT('Ctrl Pts',(11.4017985477145,-14.6527993397419,-329.570143862139)) ;
#43486=CARTESIAN_POINT('Ctrl Pts',(11.2043066797621,-14.8046874128438,-329.573275054533)) ;
#43487=CARTESIAN_POINT('Ctrl Pts',(11.0890811110369,-14.8911899379376,-329.575071240062)) ;
#43488=CARTESIAN_POINT('Ctrl Pts',(10.6832227542838,-15.1885540654725,-329.581310355411)) ;
#43489=CARTESIAN_POINT('Ctrl Pts',(10.3874896551477,-15.3923189396957,-329.585703482952)) ;
#43490=CARTESIAN_POINT('Ctrl Pts',(9.60774151246282,-15.8968659738502,-329.597078987408)) ;
#43491=CARTESIAN_POINT('Ctrl Pts',(9.11545812249566,-16.1841733378255,-329.60406949261)) ;
#43492=CARTESIAN_POINT('Ctrl Pts',(8.4473955127139,-16.5339047066207,-329.613539078241)) ;
#43493=CARTESIAN_POINT('Ctrl Pts',(8.28277959068855,-16.6169810102456,-329.615870096179)) ;
#43494=CARTESIAN_POINT('Ctrl Pts',(8.00458619126559,-16.75221506323,-329.619810181734)) ;
#43495=CARTESIAN_POINT('Ctrl Pts',(7.89167016808338,-16.805702946464,-329.621409602688)) ;
#43496=CARTESIAN_POINT('Ctrl Pts',(7.66964847227156,-16.9081427045649,-329.624555744414)) ;
#43497=CARTESIAN_POINT('Ctrl Pts',(7.56059265222892,-16.9571883314291,-329.626101702312)) ;
#43498=CARTESIAN_POINT('Ctrl Pts',(7.29722734355125,-17.0725857512681,-329.629836868554)) ;
#43499=CARTESIAN_POINT('Ctrl Pts',(7.14247645797602,-17.137903636772,-329.632033082205)) ;
#43500=CARTESIAN_POINT('Ctrl Pts',(6.78299565728528,-17.283919907025,-329.63713695483)) ;
#43501=CARTESIAN_POINT('Ctrl Pts',(6.57767479668875,-17.3630962524391,-329.640053771993)) ;
#43502=CARTESIAN_POINT('Ctrl Pts',(5.88614552412401,-17.6157385971338,-329.649870233281)) ;
#43503=CARTESIAN_POINT('Ctrl Pts',(5.39411955705996,-17.7725751641341,-329.656848523493)) ;
#43504=CARTESIAN_POINT('Ctrl Pts',(4.57377480017317,-17.9968556303417,-329.668282517099)) ;
#43505=CARTESIAN_POINT('Ctrl Pts',(4.24902635027594,-18.0762829223292,-329.672756478773)) ;
#43506=CARTESIAN_POINT('Ctrl Pts',(3.81181733203114,-18.1707822396687,-329.678642341955)) ;
#43507=CARTESIAN_POINT('Ctrl Pts',(3.70110790283412,-18.1936549083765,-329.680120955029)) ;
#43508=CARTESIAN_POINT('Ctrl Pts',(3.52937242470506,-18.2275032014787,-329.682392797058)) ;
#43509=CARTESIAN_POINT('Ctrl Pts',(3.46848873676772,-18.2391866203068,-329.683193976596)) ;
#43510=CARTESIAN_POINT('Ctrl Pts',(3.34821219083737,-18.2616433530201,-329.684767572273)) ;
#43511=CARTESIAN_POINT('Ctrl Pts',(3.28882304493746,-18.2724324001376,-329.685540195379)) ;
#43512=CARTESIAN_POINT('Ctrl Pts',(3.15747565669814,-18.2956327784626,-329.687240277513)) ;
#43513=CARTESIAN_POINT('Ctrl Pts',(3.08549464887268,-18.3079096041915,-329.688166212846)) ;
#43514=CARTESIAN_POINT('Ctrl Pts',(2.90277885860415,-18.3379647786274,-329.690503960581)) ;
#43515=CARTESIAN_POINT('Ctrl Pts',(2.79195189252602,-18.3551649952279,-329.691910195381)) ;
#43516=CARTESIAN_POINT('Ctrl Pts',(1.79330179282447,-18.5009003548878,-329.70449959216)) ;
#43517=CARTESIAN_POINT('Ctrl Pts',(0.897414458449384,-18.5659340571168,
-329.715274424528)) ;
#43518=CARTESIAN_POINT('Ctrl Pts',(0.000329891259258086,-18.5659499970691,
-329.726459838768)) ;
#43519=CARTESIAN_POINT('Ctrl Pts',(0.000329891259327128,-18.5659499970691,
-329.726459838768)) ;
#43520=CARTESIAN_POINT('Ctrl Pts',(-0.136253520319998,-18.5659524239675,
-329.728162846592)) ;
#43521=CARTESIAN_POINT('Ctrl Pts',(-0.272822686892261,-18.5644478010107,
-329.729873348739)) ;
#43522=CARTESIAN_POINT('Ctrl Pts',(-0.52081802215839,-18.5589782610562,
-329.732996218987)) ;
#43523=CARTESIAN_POINT('Ctrl Pts',(-0.632238875283148,-18.5555166858021,
-329.734405427499)) ;
#43524=CARTESIAN_POINT('Ctrl Pts',(-0.859920157713469,-18.5463900473074,
-329.737298897399)) ;
#43525=CARTESIAN_POINT('Ctrl Pts',(-0.976172098714441,-18.5406346832325,
-329.738783663845)) ;
#43526=CARTESIAN_POINT('Ctrl Pts',(-1.21176310897569,-18.5267491937409,
-329.741808570231)) ;
#43527=CARTESIAN_POINT('Ctrl Pts',(-1.33109318480385,-18.5185581622254,
-329.743349036822)) ;
#43528=CARTESIAN_POINT('Ctrl Pts',(-1.61013486882489,-18.4966931552099,
-329.746971298007)) ;
#43529=CARTESIAN_POINT('Ctrl Pts',(-1.76976501935743,-18.4821027927569,
-329.749058885577)) ;
#43530=CARTESIAN_POINT('Ctrl Pts',(-2.34670282484013,-18.4218269524272,
-329.756659084622)) ;
#43531=CARTESIAN_POINT('Ctrl Pts',(-2.76261892917325,-18.3640588487467,
-329.76224575829)) ;
#43532=CARTESIAN_POINT('Ctrl Pts',(-3.65400732626134,-18.20928048276,-329.77438407974)) ;
#43533=CARTESIAN_POINT('Ctrl Pts',(-4.1283627564002,-18.1076305916397,-329.78094748189)) ;
#43534=CARTESIAN_POINT('Ctrl Pts',(-4.79406604446586,-17.9374553268578,
-329.790144827004)) ;
#43535=CARTESIAN_POINT('Ctrl Pts',(-4.98910851811562,-17.8841876875475,
-329.79283702122)) ;
#43536=CARTESIAN_POINT('Ctrl Pts',(-5.2876392560956,-17.7973928009225,-329.796935861391)) ;
#43537=CARTESIAN_POINT('Ctrl Pts',(-5.39176778905298,-17.7661239321431,
-329.798361396359)) ;
#43538=CARTESIAN_POINT('Ctrl Pts',(-5.5553925098561,-17.715417857826,-329.800591673918)) ;
#43539=CARTESIAN_POINT('Ctrl Pts',(-5.61507527316497,-17.6965913526919,
-329.801403113806)) ;
#43540=CARTESIAN_POINT('Ctrl Pts',(-5.73781484125675,-17.6571905905673,
-329.803066766056)) ;
#43541=CARTESIAN_POINT('Ctrl Pts',(-5.80085871142923,-17.636579512741,-329.803918334821)) ;
#43542=CARTESIAN_POINT('Ctrl Pts',(-5.95609198282375,-17.5849063459132,
-329.806008659625)) ;
#43543=CARTESIAN_POINT('Ctrl Pts',(-6.048150285661,-17.5534566699538,-329.807242784401)) ;
#43544=CARTESIAN_POINT('Ctrl Pts',(-6.44040665641951,-17.4159988661017,
-329.812485398895)) ;
#43545=CARTESIAN_POINT('Ctrl Pts',(-6.73809901036303,-17.3030019658653,
-329.816424924837)) ;
#43546=CARTESIAN_POINT('Ctrl Pts',(-7.10138855594153,-17.154307980473,-329.821252348044)) ;
#43547=CARTESIAN_POINT('Ctrl Pts',(-7.1698693614902,-17.1257985231261,-329.822163160209)) ;
#43548=CARTESIAN_POINT('Ctrl Pts',(-7.69652358319347,-16.9028328794199,
-329.829178972102)) ;
#43549=CARTESIAN_POINT('Ctrl Pts',(-8.14688135666589,-16.6904331514723,
-329.83524997844)) ;
#43550=CARTESIAN_POINT('Ctrl Pts',(-8.78016287223406,-16.360016525145,-329.844096547912)) ;
#43551=CARTESIAN_POINT('Ctrl Pts',(-8.97039921160087,-16.2564860456305,
-329.846794763054)) ;
#43552=CARTESIAN_POINT('Ctrl Pts',(-9.30758355962203,-16.0652622620885,
-329.851663636507)) ;
#43553=CARTESIAN_POINT('Ctrl Pts',(-9.45521297583125,-15.9788206926722,
-329.853825743391)) ;
#43554=CARTESIAN_POINT('Ctrl Pts',(-9.69586189517585,-15.8334103747961,
-329.85740420222)) ;
#43555=CARTESIAN_POINT('Ctrl Pts',(-9.78958880375593,-15.7756322537419,
-329.858811633972)) ;
#43556=CARTESIAN_POINT('Ctrl Pts',(-9.98833960575394,-15.6506586153321,
-329.861826285248)) ;
#43557=CARTESIAN_POINT('Ctrl Pts',(-10.0932118038639,-15.5832319691426,
-329.863435222272)) ;
#43558=CARTESIAN_POINT('Ctrl Pts',(-10.3500371588856,-15.4144281311376,
-329.867421173932)) ;
#43559=CARTESIAN_POINT('Ctrl Pts',(-10.5011884212268,-15.3118550601952,
-329.869807235057)) ;
#43560=CARTESIAN_POINT('Ctrl Pts',(-11.1579634310204,-14.8518597537046,
-329.880350628439)) ;
#43561=CARTESIAN_POINT('Ctrl Pts',(-11.6470370637305,-14.4715033306896,
-329.888680715013)) ;
#43562=CARTESIAN_POINT('Ctrl Pts',(-12.3644929425667,-13.8535629407165,
-329.901435332146)) ;
#43563=CARTESIAN_POINT('Ctrl Pts',(-12.6070916660311,-13.6331629472015,
-329.905846986957)) ;
#43564=CARTESIAN_POINT('Ctrl Pts',(-12.9428499074022,-13.3114979566371,
-329.91203586379)) ;
#43565=CARTESIAN_POINT('Ctrl Pts',(-13.0409140928282,-13.2154417738512,
-329.913853806637)) ;
#43566=CARTESIAN_POINT('Ctrl Pts',(-13.1420799039833,-13.1141248326584,
-329.915736193449)) ;
#43567=CARTESIAN_POINT('Ctrl Pts',(-13.1462537060571,-13.1099408017435,
-329.915813867578)) ;
#43568=CARTESIAN_POINT('Ctrl Pts',(-13.1541323861717,-13.1020352672882,
-329.915960512055)) ;
#43569=CARTESIAN_POINT('Ctrl Pts',(-13.1578376844421,-13.0983141834389,
-329.916029487675)) ;
#43570=CARTESIAN_POINT('Ctrl Pts',(-13.1648366365848,-13.0912794471348,
-329.916159793635)) ;
#43571=CARTESIAN_POINT('Ctrl Pts',(-13.168130619304,-13.087966122507,-329.91622112815)) ;
#43572=CARTESIAN_POINT('Ctrl Pts',(-13.1743569091214,-13.0816985426064,
-329.916337076405)) ;
#43573=CARTESIAN_POINT('Ctrl Pts',(-13.1772894740584,-13.0787445439314,
-329.916391693453)) ;
#43574=CARTESIAN_POINT('Ctrl Pts',(-13.1828364781382,-13.0731532379854,
-329.916495013334)) ;
#43575=CARTESIAN_POINT('Ctrl Pts',(-13.185451119886,-13.0705161320538,-329.91654371879)) ;
#43576=CARTESIAN_POINT('Ctrl Pts',(-13.1904002181376,-13.0655215163955,
-329.916635918766)) ;
#43577=CARTESIAN_POINT('Ctrl Pts',(-13.1927348342524,-13.0631641650537,
-329.91667941537)) ;
#43578=CARTESIAN_POINT('Ctrl Pts',(-13.19715693779,-13.0586966031236,-329.916761810844)) ;
#43579=CARTESIAN_POINT('Ctrl Pts',(-13.1992445512787,-13.0565865174873,
-329.916800711372)) ;
#43580=CARTESIAN_POINT('Ctrl Pts',(-13.2032014650222,-13.0525850906244,
-329.916874449564)) ;
#43581=CARTESIAN_POINT('Ctrl Pts',(-13.2050708651241,-13.0506938482598,
-329.916909288549)) ;
#43582=CARTESIAN_POINT('Ctrl Pts',(-13.2086164916422,-13.0471052525056,
-329.916975370551)) ;
#43583=CARTESIAN_POINT('Ctrl Pts',(-13.2102927973626,-13.045407977568,-329.917006614624)) ;
#43584=CARTESIAN_POINT('Ctrl Pts',(-13.2134741923686,-13.0421855438999,
-329.917065914791)) ;
#43585=CARTESIAN_POINT('Ctrl Pts',(-13.2149793448094,-13.0406604476216,
-329.917093971731)) ;
#43586=CARTESIAN_POINT('Ctrl Pts',(-13.2178376370418,-13.0377632789091,
-329.917147254611)) ;
#43587=CARTESIAN_POINT('Ctrl Pts',(-13.2191908273269,-13.036391256279,-329.91717248123)) ;
#43588=CARTESIAN_POINT('Ctrl Pts',(-13.2217620167917,-13.0337834715962,
-329.917220416279)) ;
#43589=CARTESIAN_POINT('Ctrl Pts',(-13.2229800563898,-13.0325477494406,
-329.917243125255)) ;
#43590=CARTESIAN_POINT('Ctrl Pts',(-13.2252957040405,-13.0301978261796,
-329.917286299576)) ;
#43591=CARTESIAN_POINT('Ctrl Pts',(-13.2263933445529,-13.0290836571056,
-329.91730676536)) ;
#43592=CARTESIAN_POINT('Ctrl Pts',(-13.2284811673707,-13.0269638595787,
-329.917345694697)) ;
#43593=CARTESIAN_POINT('Ctrl Pts',(-13.2294713758394,-13.0259582568844,
-329.917364158605)) ;
#43594=CARTESIAN_POINT('Ctrl Pts',(-13.2313557589736,-13.0240441417756,
-329.917399296822)) ;
#43595=CARTESIAN_POINT('Ctrl Pts',(-13.2322499546895,-13.0231356502212,
-329.917415971418)) ;
#43596=CARTESIAN_POINT('Ctrl Pts',(-13.2339523915323,-13.0214056395346,
-329.917447718652)) ;
#43597=CARTESIAN_POINT('Ctrl Pts',(-13.2347606497656,-13.0205841372061,
-329.917462791523)) ;
#43598=CARTESIAN_POINT('Ctrl Pts',(-13.236300120926,-13.0190191488729,-329.9174915012)) ;
#43599=CARTESIAN_POINT('Ctrl Pts',(-13.2370313477453,-13.018275676477,-329.917505138196)) ;
#43600=CARTESIAN_POINT('Ctrl Pts',(-13.2384246461423,-13.0168588062833,
-329.917531123067)) ;
#43601=CARTESIAN_POINT('Ctrl Pts',(-13.2390867289481,-13.016185419611,-329.917543471096)) ;
#43602=CARTESIAN_POINT('Ctrl Pts',(-13.240348739621,-13.0149016664813,-329.917567008425)) ;
#43603=CARTESIAN_POINT('Ctrl Pts',(-13.2409486766587,-13.0142913090591,
-329.917578197852)) ;
#43604=CARTESIAN_POINT('Ctrl Pts',(-13.2420926179423,-13.0131273375298,
-329.917599533895)) ;
#43605=CARTESIAN_POINT('Ctrl Pts',(-13.2426366297038,-13.0125737307635,
-329.917609680615)) ;
#43606=CARTESIAN_POINT('Ctrl Pts',(-13.2436742607209,-13.0115176660735,
-329.917629034472)) ;
#43607=CARTESIAN_POINT('Ctrl Pts',(-13.2441678861307,-13.011015214141,-329.917638241694)) ;
#43608=CARTESIAN_POINT('Ctrl Pts',(-13.2463371621554,-13.0088068978972,
-329.917678704169)) ;
#43609=CARTESIAN_POINT('Ctrl Pts',(-13.2480125118394,-13.007100737921,-329.917709955261)) ;
#43610=CARTESIAN_POINT('Ctrl Pts',(-13.2513002679626,-13.0037512245989,
-329.917771286414)) ;
#43611=CARTESIAN_POINT('Ctrl Pts',(-13.2529126984094,-13.0021078949263,
-329.917801366809)) ;
#43612=CARTESIAN_POINT('Ctrl Pts',(-13.2560781957448,-12.9988805361063,
-329.917860422972)) ;
#43613=CARTESIAN_POINT('Ctrl Pts',(-13.2576312844977,-12.9972965284314,
-329.917889399044)) ;
#43614=CARTESIAN_POINT('Ctrl Pts',(-13.2606814622409,-12.9941845121411,
-329.917946308983)) ;
#43615=CARTESIAN_POINT('Ctrl Pts',(-13.2621785711241,-12.9926565230596,
-329.917974243128)) ;
#43616=CARTESIAN_POINT('Ctrl Pts',(-13.2651199515759,-12.9896534339698,
-329.918029127914)) ;
#43617=CARTESIAN_POINT('Ctrl Pts',(-13.2665642412228,-12.9881783517878,
-329.918056078809)) ;
#43618=CARTESIAN_POINT('Ctrl Pts',(-13.2694029577258,-12.985278145785,-329.91810905233)) ;
#43619=CARTESIAN_POINT('Ctrl Pts',(-13.2707974011233,-12.9838530381487,
-329.918135075188)) ;
#43620=CARTESIAN_POINT('Ctrl Pts',(-13.2735392244,-12.9810500181953,-329.918186244628)) ;
#43621=CARTESIAN_POINT('Ctrl Pts',(-13.2748866193577,-12.9796721206575,
-329.918211391423)) ;
#43622=CARTESIAN_POINT('Ctrl Pts',(-13.2775369815361,-12.9769609147086,
-329.918260857706)) ;
#43623=CARTESIAN_POINT('Ctrl Pts',(-13.2788399625216,-12.9756276197984,
-329.91828517739)) ;
#43624=CARTESIAN_POINT('Ctrl Pts',(-13.2814039799834,-12.9730031596505,
-329.9183330356)) ;
#43625=CARTESIAN_POINT('Ctrl Pts',(-13.2826650290461,-12.9717120067467,
-329.918356574305)) ;
#43626=CARTESIAN_POINT('Ctrl Pts',(-13.2851475235741,-12.9691695083829,
-329.918402914072)) ;
#43627=CARTESIAN_POINT('Ctrl Pts',(-13.286368980566,-12.9679181741924,-329.918425715298)) ;
#43628=CARTESIAN_POINT('Ctrl Pts',(-13.2887744991332,-12.9654531193016,
-329.918470621163)) ;
#43629=CARTESIAN_POINT('Ctrl Pts',(-13.2899585712521,-12.9642394089288,
-329.918492725953)) ;
#43630=CARTESIAN_POINT('Ctrl Pts',(-13.2922914044472,-12.9618475276289,
-329.918536277709)) ;
#43631=CARTESIAN_POINT('Ctrl Pts',(-13.2934401751812,-12.9606693661677,
-329.918557724815)) ;
#43632=CARTESIAN_POINT('Ctrl Pts',(-13.2957043744873,-12.9583466207303,
-329.918599997825)) ;
#43633=CARTESIAN_POINT('Ctrl Pts',(-13.2968198119574,-12.9572020453913,
-329.918620823859)) ;
#43634=CARTESIAN_POINT('Ctrl Pts',(-13.2990192060026,-12.9549446148674,
-329.918661889354)) ;
#43635=CARTESIAN_POINT('Ctrl Pts',(-13.3001031707067,-12.9538317676457,
-329.918682128934)) ;
#43636=CARTESIAN_POINT('Ctrl Pts',(-13.3022413801625,-12.9516360337398,
-329.91872205429)) ;
#43637=CARTESIAN_POINT('Ctrl Pts',(-13.3032956323535,-12.9505531543938,
-329.918741740175)) ;
#43638=CARTESIAN_POINT('Ctrl Pts',(-13.3053760841499,-12.948415687916,-329.918780589174)) ;
#43639=CARTESIAN_POINT('Ctrl Pts',(-13.3064022906626,-12.9473611074531,
-329.918799752389)) ;
#43640=CARTESIAN_POINT('Ctrl Pts',(-13.3084282313942,-12.9452786554912,
-329.918837585468)) ;
#43641=CARTESIAN_POINT('Ctrl Pts',(-13.3094279719604,-12.9442507901264,
-329.918856255424)) ;
#43642=CARTESIAN_POINT('Ctrl Pts',(-13.3114024800716,-12.9422202643729,
-329.918893129899)) ;
#43643=CARTESIAN_POINT('Ctrl Pts',(-13.312377253389,-12.9412176096938,-329.918911334502)) ;
#43644=CARTESIAN_POINT('Ctrl Pts',(-13.314303250759,-12.9392360753006,-329.918947304783)) ;
#43645=CARTESIAN_POINT('Ctrl Pts',(-13.3152544801854,-12.9382572007762,
-329.91896507054)) ;
#43646=CARTESIAN_POINT('Ctrl Pts',(-13.3171347433885,-12.936321865463,-329.91900018834)) ;
#43647=CARTESIAN_POINT('Ctrl Pts',(-13.3180637820872,-12.9353654094764,
-329.919017540455)) ;
#43648=CARTESIAN_POINT('Ctrl Pts',(-13.3199009523127,-12.9334736139462,
-329.919051854973)) ;
#43649=CARTESIAN_POINT('Ctrl Pts',(-13.3208090883311,-12.9325382788646,
-329.919068817442)) ;
#43650=CARTESIAN_POINT('Ctrl Pts',(-13.3226056810972,-12.9306874873656,
-329.919102375543)) ;
#43651=CARTESIAN_POINT('Ctrl Pts',(-13.3234941420755,-12.9297720349585,
-329.919118971238)) ;
#43652=CARTESIAN_POINT('Ctrl Pts',(-13.3252525566396,-12.9279598261002,
-329.919151817627)) ;
#43653=CARTESIAN_POINT('Ctrl Pts',(-13.3261225140773,-12.9270630733858,
-329.919168068379)) ;
#43654=CARTESIAN_POINT('Ctrl Pts',(-13.3278450415625,-12.9252871322244,
-329.919200245755)) ;
#43655=CARTESIAN_POINT('Ctrl Pts',(-13.3286976151464,-12.9244079472267,
-329.919216172431)) ;
#43656=CARTESIAN_POINT('Ctrl Pts',(-13.3303864469596,-12.9226660570025,
-329.919247721637)) ;
#43657=CARTESIAN_POINT('Ctrl Pts',(-13.3312227084368,-12.9218033549558,
-329.919263344215)) ;
#43658=CARTESIAN_POINT('Ctrl Pts',(-13.3328799438208,-12.9200933896785,
-329.919294304383)) ;
#43659=CARTESIAN_POINT('Ctrl Pts',(-13.3337009207704,-12.9192461293142,
-329.919309642019)) ;
#43660=CARTESIAN_POINT('Ctrl Pts',(-13.3353285743212,-12.9175660463461,
-329.919340050708)) ;
#43661=CARTESIAN_POINT('Ctrl Pts',(-13.3361352536092,-12.9167332264882,
-329.919355121802)) ;
#43662=CARTESIAN_POINT('Ctrl Pts',(-13.3377352617355,-12.9150810601814,
-329.91938501512)) ;
#43663=CARTESIAN_POINT('Ctrl Pts',(-13.3385285931048,-12.9142617161851,
-329.919399837382)) ;
#43664=CARTESIAN_POINT('Ctrl Pts',(-13.3401028212343,-12.9126355707162,
-329.919429250116)) ;
#43665=CARTESIAN_POINT('Ctrl Pts',(-13.3408837203459,-12.9118287714575,
-329.919443840624)) ;
#43666=CARTESIAN_POINT('Ctrl Pts',(-13.3424339689639,-12.9102268148361,
-329.919472806354)) ;
#43667=CARTESIAN_POINT('Ctrl Pts',(-13.3432033205669,-12.9094316595537,
-329.919487181609)) ;
#43668=CARTESIAN_POINT('Ctrl Pts',(-13.3447313312106,-12.9078521176504,
-329.919515732822)) ;
#43669=CARTESIAN_POINT('Ctrl Pts',(-13.3454899922182,-12.9070677328714,
-329.919529908811)) ;
#43670=CARTESIAN_POINT('Ctrl Pts',(-13.3469974537501,-12.9055088831316,
-329.919558077014)) ;
#43671=CARTESIAN_POINT('Ctrl Pts',(-13.3477462559823,-12.9047344199293,
-329.919572069255)) ;
#43672=CARTESIAN_POINT('Ctrl Pts',(-13.3492348097786,-12.9031945861837,
-329.919599885074)) ;
#43673=CARTESIAN_POINT('Ctrl Pts',(-13.3499745629657,-12.902429217155,-329.919613708677)) ;
#43674=CARTESIAN_POINT('Ctrl Pts',(-13.3845269427947,-12.8666742201661,
-329.920259391737)) ;
#43675=CARTESIAN_POINT('Ctrl Pts',(-13.4182019741192,-12.8315518452594,
-329.920889147483)) ;
#43676=CARTESIAN_POINT('Ctrl Pts',(-13.4979550464683,-12.7477137287387,
-329.922381262118)) ;
#43677=CARTESIAN_POINT('Ctrl Pts',(-13.5439079100178,-12.6988800396488,
-329.923241371347)) ;
#43678=CARTESIAN_POINT('Ctrl Pts',(-13.6479130059014,-12.5871480495444,
-329.925189914056)) ;
#43679=CARTESIAN_POINT('Ctrl Pts',(-13.7057968945739,-12.5240950551092,
-329.926275792337)) ;
#43680=CARTESIAN_POINT('Ctrl Pts',(-13.9595612838452,-12.2438028896569,
-329.93104801048)) ;
#43681=CARTESIAN_POINT('Ctrl Pts',(-14.1507283567185,-12.0223520217235,
-329.934674815342)) ;
#43682=CARTESIAN_POINT('Ctrl Pts',(-14.7008339811295,-11.3537934882978,
-329.945337201584)) ;
#43683=CARTESIAN_POINT('Ctrl Pts',(-15.0443851190424,-10.8944767595447,
-329.952305808455)) ;
#43684=CARTESIAN_POINT('Ctrl Pts',(-15.4550558782701,-10.2888702007673,
-329.961353601538)) ;
#43685=CARTESIAN_POINT('Ctrl Pts',(-15.5422960980164,-10.1566054436673,
-329.963320739079)) ;
#43686=CARTESIAN_POINT('Ctrl Pts',(-15.7508580116747,-9.8314241099991,-329.968143145274)) ;
#43687=CARTESIAN_POINT('Ctrl Pts',(-15.8703412710499,-9.63735937916694,
-329.971009542133)) ;
#43688=CARTESIAN_POINT('Ctrl Pts',(-16.0548287586074,-9.3249758748697,-329.975615357569)) ;
#43689=CARTESIAN_POINT('Ctrl Pts',(-16.122167415691,-9.20806273281387,-329.977337287434)) ;
#43690=CARTESIAN_POINT('Ctrl Pts',(-16.2502161196128,-8.98003367331189,
-329.980693588445)) ;
#43691=CARTESIAN_POINT('Ctrl Pts',(-16.3110756363759,-8.86901010474918,
-329.982326729681)) ;
#43692=CARTESIAN_POINT('Ctrl Pts',(-16.4418118717734,-8.62461533990689,
-329.985920118333)) ;
#43693=CARTESIAN_POINT('Ctrl Pts',(-16.5112114197094,-8.49099904327274,
-329.987883680545)) ;
#43694=CARTESIAN_POINT('Ctrl Pts',(-16.7837122394884,-7.9503712518873,-329.995823471012)) ;
#43695=CARTESIAN_POINT('Ctrl Pts',(-16.9734496294718,-7.53680337919305,
-330.001890058656)) ;
#43696=CARTESIAN_POINT('Ctrl Pts',(-17.3290383100729,-6.68000499861943,
-330.014354572443)) ;
#43697=CARTESIAN_POINT('Ctrl Pts',(-17.4935232749659,-6.2365598488215,-330.020751702949)) ;
#43698=CARTESIAN_POINT('Ctrl Pts',(-17.6922594141145,-5.63077270183929,
-330.029268824819)) ;
#43699=CARTESIAN_POINT('Ctrl Pts',(-17.7415310120517,-5.47354746622276,
-330.031459075067)) ;
#43700=CARTESIAN_POINT('Ctrl Pts',(-17.8242658730452,-5.19667904602995,
-330.035269401811)) ;
#43701=CARTESIAN_POINT('Ctrl Pts',(-17.8586332119113,-5.07731689958857,
-330.036897023388)) ;
#43702=CARTESIAN_POINT('Ctrl Pts',(-17.9107216446587,-4.88933232942958,
-330.039432000762)) ;
#43703=CARTESIAN_POINT('Ctrl Pts',(-17.9292519857035,-4.820938053306,-330.040348430081)) ;
#43704=CARTESIAN_POINT('Ctrl Pts',(-17.96337531968,-4.69207269489941,-330.042062967361)) ;
#43705=CARTESIAN_POINT('Ctrl Pts',(-17.9790556422573,-4.63162577011559,
-330.04286220575)) ;
#43706=CARTESIAN_POINT('Ctrl Pts',(-18.0229290488223,-4.45891530031092,
-330.045132952961)) ;
#43707=CARTESIAN_POINT('Ctrl Pts',(-18.0503776788936,-4.34646556022606,
-330.046595961024)) ;
#43708=CARTESIAN_POINT('Ctrl Pts',(-18.1800605378239,-3.79276292687671,
-330.053738688009)) ;
#43709=CARTESIAN_POINT('Ctrl Pts',(-18.2671756163945,-3.34812618423389,
-330.0592880579)) ;
#43710=CARTESIAN_POINT('Ctrl Pts',(-18.4055755809194,-2.47318980316046,
-330.070138401297)) ;
#43711=CARTESIAN_POINT('Ctrl Pts',(-18.4582342332835,-2.0433964030528,-330.075436142913)) ;
#43712=CARTESIAN_POINT('Ctrl Pts',(-18.520702215416,-1.32671877871265,-330.084362257575)) ;
#43713=CARTESIAN_POINT('Ctrl Pts',(-18.5389709950648,-1.04074359066319,
-330.08794737285)) ;
#43714=CARTESIAN_POINT('Ctrl Pts',(-18.5564902974383,-0.609980587295372,
-330.093404559269)) ;
#43715=CARTESIAN_POINT('Ctrl Pts',(-18.5606782477298,-0.465436764969228,
-330.095245224115)) ;
#43716=CARTESIAN_POINT('Ctrl Pts',(-18.5653241829315,-0.196647865447113,
-330.09868757901)) ;
#43717=CARTESIAN_POINT('Ctrl Pts',(-18.5662243849018,-0.0724184965304549,
-330.100286310085)) ;
#43718=CARTESIAN_POINT('Ctrl Pts',(-18.5654349079548,0.210484620098622,
-330.103945340857)) ;
#43719=CARTESIAN_POINT('Ctrl Pts',(-18.5629579515323,0.369146422718707,
-330.106010586646)) ;
#43720=CARTESIAN_POINT('Ctrl Pts',(-18.548018142377,0.894501425156988,-330.112892034296)) ;
#43721=CARTESIAN_POINT('Ctrl Pts',(-18.5267199556095,1.2608554099375,-330.117761959716)) ;
#43722=CARTESIAN_POINT('Ctrl Pts',(-18.43265997682,2.33049874018311,-330.132134311281)) ;
#43723=CARTESIAN_POINT('Ctrl Pts',(-18.3305742706896,3.03054813755851,-330.141754210235)) ;
#43724=CARTESIAN_POINT('Ctrl Pts',(-18.1590066031488,3.86873181611012,-330.15307932388)) ;
#43725=CARTESIAN_POINT('Ctrl Pts',(-18.1274416699266,4.01403354532787,-330.155034373553)) ;
#43726=CARTESIAN_POINT('Ctrl Pts',(-18.0772217848843,4.23252317062873,-330.157954059474)) ;
#43727=CARTESIAN_POINT('Ctrl Pts',(-18.0598600987755,4.30600198360925,-330.158932502206)) ;
#43728=CARTESIAN_POINT('Ctrl Pts',(-18.0261927133768,4.44470418746964,-330.160771547352)) ;
#43729=CARTESIAN_POINT('Ctrl Pts',(-18.0099800383235,4.50994878727905,-330.161633168939)) ;
#43730=CARTESIAN_POINT('Ctrl Pts',(-17.9667452755004,4.67998666571188,-330.163871058409)) ;
#43731=CARTESIAN_POINT('Ctrl Pts',(-17.9391606473623,4.78463439632518,-330.165240821007)) ;
#43732=CARTESIAN_POINT('Ctrl Pts',(-17.7372999923676,5.5241378043481,-330.174884297477)) ;
#43733=CARTESIAN_POINT('Ctrl Pts',(-17.5302788647954,6.14957228770004,-330.182868660411)) ;
#43734=CARTESIAN_POINT('Ctrl Pts',(-17.1742018209146,7.05997079450781,-330.194869220699)) ;
#43735=CARTESIAN_POINT('Ctrl Pts',(-17.0502806158901,7.35420466829498,-330.198805602119)) ;
#43736=CARTESIAN_POINT('Ctrl Pts',(-16.8206005133454,7.86249384173043,-330.205759654458)) ;
#43737=CARTESIAN_POINT('Ctrl Pts',(-16.71818463764,8.07797704599655,-330.208757252731)) ;
#43738=CARTESIAN_POINT('Ctrl Pts',(-16.5505627479003,8.41380289599961,-330.213519254982)) ;
#43739=CARTESIAN_POINT('Ctrl Pts',(-16.488130174181,8.53550055577084,-330.215263894579)) ;
#43740=CARTESIAN_POINT('Ctrl Pts',(-16.3656770694023,8.76783630114897,-330.218632732258)) ;
#43741=CARTESIAN_POINT('Ctrl Pts',(-16.3058649255907,8.87857580464569,-330.220255336782)) ;
#43742=CARTESIAN_POINT('Ctrl Pts',(-16.1608172959327,9.14071484634711,-330.22413735203)) ;
#43743=CARTESIAN_POINT('Ctrl Pts',(-16.0745735575623,9.29154284178438,-330.226404045859)) ;
#43744=CARTESIAN_POINT('Ctrl Pts',(-15.5684391087905,10.1485560099807,-330.239472353046)) ;
#43745=CARTESIAN_POINT('Ctrl Pts',(-15.1041571454183,10.8274608739033,-330.250614457625)) ;
#43746=CARTESIAN_POINT('Ctrl Pts',(-14.4643211654238,11.6414613953628,-330.264507321033)) ;
#43747=CARTESIAN_POINT('Ctrl Pts',(-14.3293028673811,11.8072558088925,-330.267364092716)) ;
#43748=CARTESIAN_POINT('Ctrl Pts',(-14.145305022986,12.0253884570602,-330.27114166207)) ;
#43749=CARTESIAN_POINT('Ctrl Pts',(-14.0988428729793,12.0798282848755,-330.272086033692)) ;
#43750=CARTESIAN_POINT('Ctrl Pts',(-13.981638561609,12.2155595441264,-330.274443197448)) ;
#43751=CARTESIAN_POINT('Ctrl Pts',(-13.9105011979168,12.2965063460543,-330.275851344508)) ;
#43752=CARTESIAN_POINT('Ctrl Pts',(-13.7934508935331,12.4273815230122,-330.278128679977)) ;
#43753=CARTESIAN_POINT('Ctrl Pts',(-13.7479619785729,12.477685704791,-330.279004137428)) ;
#43754=CARTESIAN_POINT('Ctrl Pts',(-13.6509320763541,12.5838120293233,-330.280850419676)) ;
#43755=CARTESIAN_POINT('Ctrl Pts',(-13.5993220767821,12.6395692495885,-330.281820210794)) ;
#43756=CARTESIAN_POINT('Ctrl Pts',(-13.4438957033224,12.8054311976472,-330.284707014249)) ;
#43757=CARTESIAN_POINT('Ctrl Pts',(-13.3390738058178,12.914585164464,-330.286609457279)) ;
#43758=CARTESIAN_POINT('Ctrl Pts',(-12.7710775013925,13.4917620693357,-330.296718042306)) ;
#43759=CARTESIAN_POINT('Ctrl Pts',(-12.2845848681025,13.9361775345369,-330.30469415982)) ;
#43760=CARTESIAN_POINT('Ctrl Pts',(-11.5591430101337,14.531312247344,-330.316241653929)) ;
#43761=CARTESIAN_POINT('Ctrl Pts',(-11.3387881252921,14.7039010560922,-330.319704569893)) ;
#43762=CARTESIAN_POINT('Ctrl Pts',(-10.9394009754564,15.0023949674402,-330.325935682732)) ;
#43763=CARTESIAN_POINT('Ctrl Pts',(-10.7618850614671,15.1302405182814,-330.328689800325)) ;
#43764=CARTESIAN_POINT('Ctrl Pts',(-10.4726160288993,15.3309029260531,-330.333161913369)) ;
#43765=CARTESIAN_POINT('Ctrl Pts',(-10.3622651056525,15.4057045549696,-330.334864277859)) ;
#43766=CARTESIAN_POINT('Ctrl Pts',(-10.1460758427992,15.5488751184642,-330.338193616322)) ;
#43767=CARTESIAN_POINT('Ctrl Pts',(-10.0403281540684,15.6173679908819,-330.339819505918)) ;
#43768=CARTESIAN_POINT('Ctrl Pts',(-9.77912151819271,15.7828021601966,-330.343829718169)) ;
#43769=CARTESIAN_POINT('Ctrl Pts',(-9.62290924836227,15.8785288718491,-330.346223016252)) ;
#43770=CARTESIAN_POINT('Ctrl Pts',(-8.9415261233652,16.2823310855383,-330.356638513113)) ;
#43771=CARTESIAN_POINT('Ctrl Pts',(-8.40279578270078,16.5667804125906,-330.364826554985)) ;
#43772=CARTESIAN_POINT('Ctrl Pts',(-7.54849745567921,16.9654404918007,-330.377525684185)) ;
#43773=CARTESIAN_POINT('Ctrl Pts',(-7.24217209574838,17.0984481341291,-330.382021945385)) ;
#43774=CARTESIAN_POINT('Ctrl Pts',(-6.80380196922627,17.2748951637049,-330.388312954738)) ;
#43775=CARTESIAN_POINT('Ctrl Pts',(-6.67460098003471,17.3252251353954,-330.390149648642)) ;
#43776=CARTESIAN_POINT('Ctrl Pts',(-6.44220904980851,17.412767491037,-330.393415108041)) ;
#43777=CARTESIAN_POINT('Ctrl Pts',(-6.33922911760615,17.4505215792415,-330.394848843323)) ;
#43778=CARTESIAN_POINT('Ctrl Pts',(-6.17173349665641,17.5102498249634,-330.397155875418)) ;
#43779=CARTESIAN_POINT('Ctrl Pts',(-6.10742075147503,17.5327851492931,-330.39803575777)) ;
#43780=CARTESIAN_POINT('Ctrl Pts',(-5.97179533334822,17.5794717906068,-330.399877830968)) ;
#43781=CARTESIAN_POINT('Ctrl Pts',(-5.90045696742182,17.6035444026449,-330.400839121879)) ;
#43782=CARTESIAN_POINT('Ctrl Pts',(-5.68891678466876,17.6734967191664,-330.403669619952)) ;
#43783=CARTESIAN_POINT('Ctrl Pts',(-5.54831225292222,17.7181401882011,-330.405525074616)) ;
#43784=CARTESIAN_POINT('Ctrl Pts',(-5.25041902066515,17.8088308071335,-330.409414420272)) ;
#43785=CARTESIAN_POINT('Ctrl Pts',(-5.09302234233534,17.8544806179482,-330.41144512512)) ;
#43786=CARTESIAN_POINT('Ctrl Pts',(-4.35923786866158,18.0568076298321,-330.420834864404)) ;
#43787=CARTESIAN_POINT('Ctrl Pts',(-3.77610759536126,18.1876955589154,-330.428088034698)) ;
#43788=CARTESIAN_POINT('Ctrl Pts',(-2.95776386008898,18.3303191866483,-330.438355253695)) ;
#43789=CARTESIAN_POINT('Ctrl Pts',(-2.72710853489258,18.3660514901803,-330.441257084157)) ;
#43790=CARTESIAN_POINT('Ctrl Pts',(-2.30454491617452,18.4233775382452,-330.446605069067)) ;
#43791=CARTESIAN_POINT('Ctrl Pts',(-2.1128557045592,18.4463440222037,-330.449042903189)) ;
#43792=CARTESIAN_POINT('Ctrl Pts',(-1.79268696095943,18.4796475794912,-330.453139932179)) ;
#43793=CARTESIAN_POINT('Ctrl Pts',(-1.6643952672059,18.49164377605,-330.454788306525)) ;
#43794=CARTESIAN_POINT('Ctrl Pts',(-1.42056971561077,18.511885224267,-330.457934858882)) ;
#43795=CARTESIAN_POINT('Ctrl Pts',(-1.3050631783048,18.5203866842054,-330.459431292795)) ;
#43796=CARTESIAN_POINT('Ctrl Pts',(-0.998050736891243,18.540096875677,-330.463424609158)) ;
#43797=CARTESIAN_POINT('Ctrl Pts',(-0.806438011670655,18.5494192627321,
-330.465933369702)) ;
#43798=CARTESIAN_POINT('Ctrl Pts',(-0.265137891414773,18.5673514520463,
-330.473064661434)) ;
#43799=CARTESIAN_POINT('Ctrl Pts',(0.0846964548702557,18.5690512321255,
-330.477726569645)) ;
#43800=CARTESIAN_POINT('Ctrl Pts',(0.944716209138017,18.5489247062297,-330.489268022014)) ;
#43801=CARTESIAN_POINT('Ctrl Pts',(1.45435325300007,18.5159377958033,-330.496180897783)) ;
#43802=CARTESIAN_POINT('Ctrl Pts',(2.13144833796877,18.4439819671419,-330.505282965533)) ;
#43803=CARTESIAN_POINT('Ctrl Pts',(2.30065958393488,18.4236399343413,-330.507550052675)) ;
#43804=CARTESIAN_POINT('Ctrl Pts',(2.59566187134941,18.3840481175298,-330.511476914593)) ;
#43805=CARTESIAN_POINT('Ctrl Pts',(2.72157975272574,18.3658293977838,-330.51314484999)) ;
#43806=CARTESIAN_POINT('Ctrl Pts',(2.91790763442282,18.3353598241163,-330.515727535907)) ;
#43807=CARTESIAN_POINT('Ctrl Pts',(2.98845094562475,18.3239942645186,-330.516651901171)) ;
#43808=CARTESIAN_POINT('Ctrl Pts',(3.12012800451669,18.3019985444771,-330.518369393842)) ;
#43809=CARTESIAN_POINT('Ctrl Pts',(3.18127747027054,18.2914685892794,-330.519163759142)) ;
#43810=CARTESIAN_POINT('Ctrl Pts',(3.35400725115976,18.2608321006529,-330.521399854912)) ;
#43811=CARTESIAN_POINT('Ctrl Pts',(3.46545789937346,18.2400097383763,-330.522833492951)) ;
#43812=CARTESIAN_POINT('Ctrl Pts',(3.91002740191182,18.152728919914,-330.528526692099)) ;
#43813=CARTESIAN_POINT('Ctrl Pts',(4.24148600860538,18.0781547438008,-330.532715109503)) ;
#43814=CARTESIAN_POINT('Ctrl Pts',(4.66042007506674,17.9717431218927,-330.538020525971)) ;
#43815=CARTESIAN_POINT('Ctrl Pts',(4.74995628512105,17.948286308442,-330.539155018645)) ;
#43816=CARTESIAN_POINT('Ctrl Pts',(5.27296915614832,17.8070789640222,-330.54579214766)) ;
#43817=CARTESIAN_POINT('Ctrl Pts',(5.70223304603178,17.6742978052518,-330.551284558652)) ;
#43818=CARTESIAN_POINT('Ctrl Pts',(6.40224354314676,17.4296084892856,-330.560480792541)) ;
#43819=CARTESIAN_POINT('Ctrl Pts',(6.67591198718012,17.3266319028515,-330.564137295782)) ;
#43820=CARTESIAN_POINT('Ctrl Pts',(7.0819457151203,17.1628001430728,-330.569678279624)) ;
#43821=CARTESIAN_POINT('Ctrl Pts',(7.21621285815448,17.1067804033833,-330.571529771928)) ;
#43822=CARTESIAN_POINT('Ctrl Pts',(7.46381411742008,17.0000409174488,-330.574981784457)) ;
#43823=CARTESIAN_POINT('Ctrl Pts',(7.57732470549655,16.9497511082243,-330.57657920176)) ;
#43824=CARTESIAN_POINT('Ctrl Pts',(7.83362121755809,16.8331121763911,-330.580220594592)) ;
#43825=CARTESIAN_POINT('Ctrl Pts',(7.97608468603455,16.7660776540508,-330.582269327131)) ;
#43826=CARTESIAN_POINT('Ctrl Pts',(8.44374247239506,16.5387169922565,-330.58907612113)) ;
#43827=CARTESIAN_POINT('Ctrl Pts',(8.76509259141467,16.3706779779518,-330.593886625509)) ;
#43828=CARTESIAN_POINT('Ctrl Pts',(9.57457769856437,15.91671416956,-330.606304950867)) ;
#43829=CARTESIAN_POINT('Ctrl Pts',(10.0549420818349,15.6176972135123,-330.613970637585)) ;
#43830=CARTESIAN_POINT('Ctrl Pts',(10.6674054883339,15.1964658173426,-330.623914886536)) ;
#43831=CARTESIAN_POINT('Ctrl Pts',(10.8124493873061,15.0936096272304,-330.626282169136)) ;
#43832=CARTESIAN_POINT('Ctrl Pts',(11.0618242976338,14.9113288095529,-330.630360027915)) ;
#43833=CARTESIAN_POINT('Ctrl Pts',(11.1668329019886,14.8328529516374,-330.632079595866)) ;
#43834=CARTESIAN_POINT('Ctrl Pts',(11.3283788745497,14.7094372787573,-330.634723271198)) ;
#43835=CARTESIAN_POINT('Ctrl Pts',(11.3854999046103,14.6652686618184,-330.635657703338)) ;
#43836=CARTESIAN_POINT('Ctrl Pts',(11.4908750976571,14.5828009626417,-330.637379696597)) ;
#43837=CARTESIAN_POINT('Ctrl Pts',(11.5391990744827,14.5445927804325,-330.638168628663)) ;
#43838=CARTESIAN_POINT('Ctrl Pts',(11.6737859913536,14.4370863883866,-330.640365054213)) ;
#43839=CARTESIAN_POINT('Ctrl Pts',(11.7596209988422,14.3672564109107,-330.641764918546)) ;
#43840=CARTESIAN_POINT('Ctrl Pts',(12.3396772287036,13.8866781518124,-330.651236203986)) ;
#43841=CARTESIAN_POINT('Ctrl Pts',(12.8129095368567,13.4512757650125,-330.659035247609)) ;
#43842=CARTESIAN_POINT('Ctrl Pts',(13.5252414116801,12.7241185508863,-330.671527724634)) ;
#43843=CARTESIAN_POINT('Ctrl Pts',(13.7796804841054,12.448122477662,-330.676156981096)) ;
#43844=CARTESIAN_POINT('Ctrl Pts',(14.1654756076201,12.0033073898244,-330.683520318217)) ;
#43845=CARTESIAN_POINT('Ctrl Pts',(14.3025789224492,11.8396082462023,-330.68621010401)) ;
#43846=CARTESIAN_POINT('Ctrl Pts',(14.5200695499862,11.5706355311982,-330.690605657685)) ;
#43847=CARTESIAN_POINT('Ctrl Pts',(14.6022074586778,11.4668026757767,-330.692296822623)) ;
#43848=CARTESIAN_POINT('Ctrl Pts',(14.7606662782872,11.2620265454936,-330.695622348043)) ;
#43849=CARTESIAN_POINT('Ctrl Pts',(14.837079663646,11.1611638233146,-330.697255824766)) ;
#43850=CARTESIAN_POINT('Ctrl Pts',(15.0054393076973,10.93415089968,-330.70092278009)) ;
#43851=CARTESIAN_POINT('Ctrl Pts',(15.0968377294883,10.8076063577771,-330.702960441803)) ;
#43852=CARTESIAN_POINT('Ctrl Pts',(15.5928285095384,10.1023178330221,-330.714280342524)) ;
#43853=CARTESIAN_POINT('Ctrl Pts',(15.9657426802518,9.5020092214521,-330.723805345154)) ;
#43854=CARTESIAN_POINT('Ctrl Pts',(16.4398007717999,8.63183406651436,-330.737144509256)) ;
#43855=CARTESIAN_POINT('Ctrl Pts',(16.5702748949346,8.37863944746278,-330.740969656312)) ;
#43856=CARTESIAN_POINT('Ctrl Pts',(16.7732997251202,7.96134729735255,-330.747136047434)) ;
#43857=CARTESIAN_POINT('Ctrl Pts',(16.8493878936984,7.7990231606987,-330.749501435829)) ;
#43858=CARTESIAN_POINT('Ctrl Pts',(16.9562796271057,7.56211504431382,-330.752892970722)) ;
#43859=CARTESIAN_POINT('Ctrl Pts',(16.9889665435267,7.48839225356145,-330.753939942318)) ;
#43860=CARTESIAN_POINT('Ctrl Pts',(17.0476805726677,7.35360404775812,-330.755837214709)) ;
#43861=CARTESIAN_POINT('Ctrl Pts',(17.0738624229277,7.29260771989684,-330.756689363579)) ;
#43862=CARTESIAN_POINT('Ctrl Pts',(17.1377818994226,7.14146215730707,-330.758785892709)) ;
#43863=CARTESIAN_POINT('Ctrl Pts',(17.1751359140834,7.05115285248894,-330.760025569413)) ;
#43864=CARTESIAN_POINT('Ctrl Pts',(17.3324832943503,6.66207057259511,-330.765318662161)) ;
#43865=CARTESIAN_POINT('Ctrl Pts',(17.4454069882982,6.36049820391623,-330.769301620633)) ;
#43866=CARTESIAN_POINT('Ctrl Pts',(17.5813613865055,5.96650835964682,-330.774426246179)) ;
#43867=CARTESIAN_POINT('Ctrl Pts',(17.6116041530699,5.87663929233429,-330.775589856258)) ;
#43868=CARTESIAN_POINT('Ctrl Pts',(17.7504623036431,5.45330904603572,-330.781052110883)) ;
#43869=CARTESIAN_POINT('Ctrl Pts',(17.850303590099,5.11704536422929,-330.785337317924)) ;
#43870=CARTESIAN_POINT('Ctrl Pts',(18.0108946178227,4.51407365820172,-330.793020421365)) ;
#43871=CARTESIAN_POINT('Ctrl Pts',(18.0753888958531,4.248470532261,-330.796404094652)) ;
#43872=CARTESIAN_POINT('Ctrl Pts',(18.1801601453633,3.77128809313169,-330.802512228286)) ;
#43873=CARTESIAN_POINT('Ctrl Pts',(18.2226635623305,3.56024848195099,-330.805223510444)) ;
#43874=CARTESIAN_POINT('Ctrl Pts',(18.2854204969547,3.21799706598658,-330.809644639257)) ;
#43875=CARTESIAN_POINT('Ctrl Pts',(18.3079534214318,3.0872235624646,-330.811339542366)) ;
#43876=CARTESIAN_POINT('Ctrl Pts',(18.3492000632301,2.83148713834371,-330.814666222814)) ;
#43877=CARTESIAN_POINT('Ctrl Pts',(18.3680438894766,2.70655241874825,-330.816297048297)) ;
#43878=CARTESIAN_POINT('Ctrl Pts',(18.4114024266118,2.39774234540761,-330.82034251724)) ;
#43879=CARTESIAN_POINT('Ctrl Pts',(18.4344394283744,2.21367352296865,-330.822766516354)) ;
#43880=CARTESIAN_POINT('Ctrl Pts',(18.5072558371612,1.55146872798468,-330.831530158293)) ;
#43881=CARTESIAN_POINT('Ctrl Pts',(18.5412200923983,1.07178776105259,-330.837963614467)) ;
#43882=CARTESIAN_POINT('Ctrl Pts',(18.5722535928492,0.0979286306117823,
-330.851076039381)) ;
#43883=CARTESIAN_POINT('Ctrl Pts',(18.568291445729,-0.395901093677352,-330.857751613595)) ;
#43884=CARTESIAN_POINT('Ctrl Pts',(18.544654593739,-0.888979978073086,-330.86430516735)) ;
#43885=CARTESIAN_POINT('Origin',(0.,0.,-315.477129595899)) ;
#43886=CARTESIAN_POINT('',(18.5446545939399,-0.88897997388336,-332.65888667131)) ;
#43887=CARTESIAN_POINT('',(18.5446545937435,-0.888979977979341,-332.362654732516)) ;
#43888=CARTESIAN_POINT('',(18.544654593745,-0.888979977948782,-315.477129595899)) ;
#43889=CARTESIAN_POINT('Ctrl Pts',(18.5446545941347,-0.888979969817794,
-332.65888667131)) ;
#43890=CARTESIAN_POINT('Ctrl Pts',(18.549807122682,-0.781495138392689,-332.65744111959)) ;
#43891=CARTESIAN_POINT('Ctrl Pts',(18.5540254542741,-0.673959749677189,
-332.655998027345)) ;
#43892=CARTESIAN_POINT('Ctrl Pts',(18.5625531864199,-0.394553534468471,
-332.652260710908)) ;
#43893=CARTESIAN_POINT('Ctrl Pts',(18.5654107839571,-0.222656339114593,
-332.649973388167)) ;
#43894=CARTESIAN_POINT('Ctrl Pts',(18.5662305343021,0.0772676058847497,
-332.646015943345)) ;
#43895=CARTESIAN_POINT('Ctrl Pts',(18.5652564444396,0.205279736459089,-332.644337495356)) ;
#43896=CARTESIAN_POINT('Ctrl Pts',(18.5616731456678,0.404866537420916,-332.641742379208)) ;
#43897=CARTESIAN_POINT('Ctrl Pts',(18.5599735727799,0.476453434465815,-332.640815953297)) ;
#43898=CARTESIAN_POINT('Ctrl Pts',(18.5557735883991,0.618677214032688,-332.638985330595)) ;
#43899=CARTESIAN_POINT('Ctrl Pts',(18.553283867115,0.689313221327153,-332.638081040308)) ;
#43900=CARTESIAN_POINT('Ctrl Pts',(18.5453445207493,0.883117037619062,-332.635611442937)) ;
#43901=CARTESIAN_POINT('Ctrl Pts',(18.5390713076382,1.00624759371806,-332.634055158421)) ;
#43902=CARTESIAN_POINT('Ctrl Pts',(18.5186817551908,1.34083383255402,-332.629851165483)) ;
#43903=CARTESIAN_POINT('Ctrl Pts',(18.5021706053315,1.55212514206539,-332.62722334177)) ;
#43904=CARTESIAN_POINT('Ctrl Pts',(18.4258644882299,2.35202479411313,-332.617315128808)) ;
#43905=CARTESIAN_POINT('Ctrl Pts',(18.3415651534932,2.9379401085981,-332.610129238686)) ;
#43906=CARTESIAN_POINT('Ctrl Pts',(18.1989692959521,3.67666369827731,-332.60082916468)) ;
#43907=CARTESIAN_POINT('Ctrl Pts',(18.1664539358332,3.83409581363103,-332.598833986268)) ;
#43908=CARTESIAN_POINT('Ctrl Pts',(18.0824381810205,4.21578772559234,-332.59395653658)) ;
#43909=CARTESIAN_POINT('Ctrl Pts',(18.0288054755193,4.43955060391422,-332.591063081894)) ;
#43910=CARTESIAN_POINT('Ctrl Pts',(17.9370514416407,4.79322346820572,-332.586425045286)) ;
#43911=CARTESIAN_POINT('Ctrl Pts',(17.9016443649152,4.9238130146975,-332.584698412051)) ;
#43912=CARTESIAN_POINT('Ctrl Pts',(17.8303951398075,5.17566365698886,-332.581339738305)) ;
#43913=CARTESIAN_POINT('Ctrl Pts',(17.7947353896132,5.29696870781754,-332.579709005057)) ;
#43914=CARTESIAN_POINT('Ctrl Pts',(17.714149104945,5.56110025666202,-332.57612918988)) ;
#43915=CARTESIAN_POINT('Ctrl Pts',(17.6687283038838,5.70376670393188,-332.574176898779)) ;
#43916=CARTESIAN_POINT('Ctrl Pts',(17.3868838103935,6.55334922010558,-332.562439959055)) ;
#43917=CARTESIAN_POINT('Ctrl Pts',(17.1097877719656,7.24605184294243,-332.552376386737)) ;
#43918=CARTESIAN_POINT('Ctrl Pts',(16.6226325593421,8.27887961503089,-332.537010334729)) ;
#43919=CARTESIAN_POINT('Ctrl Pts',(16.4420112256915,8.63203503321068,-332.531694544842)) ;
#43920=CARTESIAN_POINT('Ctrl Pts',(16.2020137445322,9.06637661318281,-332.525183802754)) ;
#43921=CARTESIAN_POINT('Ctrl Pts',(16.1531062217308,9.1532285944377,-332.523883429686)) ;
#43922=CARTESIAN_POINT('Ctrl Pts',(16.0703500834186,9.29746121219674,-332.52172919014)) ;
#43923=CARTESIAN_POINT('Ctrl Pts',(16.0368877934428,9.35506102245181,-332.520870366894)) ;
#43924=CARTESIAN_POINT('Ctrl Pts',(15.9627790855007,9.48106079043604,-332.518995572742)) ;
#43925=CARTESIAN_POINT('Ctrl Pts',(15.9220015809274,9.54938194464102,-332.517981299589)) ;
#43926=CARTESIAN_POINT('Ctrl Pts',(15.7914525268394,9.76495093601675,-332.514785194037)) ;
#43927=CARTESIAN_POINT('Ctrl Pts',(15.7000678159441,9.91121135106646,-332.512622816313)) ;
#43928=CARTESIAN_POINT('Ctrl Pts',(15.1515977814083,10.7624079985534,-332.50001896546)) ;
#43929=CARTESIAN_POINT('Ctrl Pts',(14.649123808177,11.4369368134646,-332.489904354698)) ;
#43930=CARTESIAN_POINT('Ctrl Pts',(13.9354617321469,12.2704328666442,-332.476251252102)) ;
#43931=CARTESIAN_POINT('Ctrl Pts',(13.7641860659879,12.4622549320057,-332.473025864191)) ;
#43932=CARTESIAN_POINT('Ctrl Pts',(13.4936432589056,12.7528690346586,-332.467993299187)) ;
#43933=CARTESIAN_POINT('Ctrl Pts',(13.3971500553403,12.8541995992538,-332.466210113709)) ;
#43934=CARTESIAN_POINT('Ctrl Pts',(13.2123268252194,13.0439463078578,-332.462814949249)) ;
#43935=CARTESIAN_POINT('Ctrl Pts',(13.1242314196923,13.1325802875496,-332.461205136951)) ;
#43936=CARTESIAN_POINT('Ctrl Pts',(12.9187006471593,13.3352338531682,-332.457468131073)) ;
#43937=CARTESIAN_POINT('Ctrl Pts',(12.8006389329762,13.4486033149329,-332.455335270008)) ;
#43938=CARTESIAN_POINT('Ctrl Pts',(12.3502811365066,13.869758356576,-332.447251320563)) ;
#43939=CARTESIAN_POINT('Ctrl Pts',(12.0082596987081,14.1669099653063,-332.441212524246)) ;
#43940=CARTESIAN_POINT('Ctrl Pts',(11.6251546450346,14.4759048234444,-332.434600358558)) ;
#43941=CARTESIAN_POINT('Ctrl Pts',(11.5945153010191,14.5004570932174,-332.434072595585)) ;
#43942=CARTESIAN_POINT('Ctrl Pts',(11.1636381964721,14.8434936595125,-332.426666140075)) ;
#43943=CARTESIAN_POINT('Ctrl Pts',(10.7504837829534,15.1454026115569,-332.419743338692)) ;
#43944=CARTESIAN_POINT('Ctrl Pts',(10.1727890915306,15.5319856287705,-332.410502354599)) ;
#43945=CARTESIAN_POINT('Ctrl Pts',(10.018679129557,15.6318355985427,-332.408078385857)) ;
#43946=CARTESIAN_POINT('Ctrl Pts',(9.79422237962059,15.7725812536972,-332.404620432278)) ;
#43947=CARTESIAN_POINT('Ctrl Pts',(9.72504838303429,15.8153262817544,-332.403564522606)) ;
#43948=CARTESIAN_POINT('Ctrl Pts',(9.599006512591,15.8920723314215,-332.401659843577)) ;
#43949=CARTESIAN_POINT('Ctrl Pts',(9.54223336082573,15.9262259025619,-332.400809109733)) ;
#43950=CARTESIAN_POINT('Ctrl Pts',(9.40223221098179,16.0094303929321,-332.398728101208)) ;
#43951=CARTESIAN_POINT('Ctrl Pts',(9.31880185771756,16.0581370037351,-332.397502348841)) ;
#43952=CARTESIAN_POINT('Ctrl Pts',(8.99876857171655,16.2416382398168,-332.392848390569)) ;
#43953=CARTESIAN_POINT('Ctrl Pts',(8.75959023009571,16.3718730787138,-332.389469108606)) ;
#43954=CARTESIAN_POINT('Ctrl Pts',(7.99753636437719,16.7653370039253,-332.378898453835)) ;
#43955=CARTESIAN_POINT('Ctrl Pts',(7.46503062565287,17.0091279008574,-332.371786955298)) ;
#43956=CARTESIAN_POINT('Ctrl Pts',(6.70699416531564,17.3137046618252,-332.361687555079)) ;
#43957=CARTESIAN_POINT('Ctrl Pts',(6.49049194098694,17.3960240854922,-332.358807284647)) ;
#43958=CARTESIAN_POINT('Ctrl Pts',(6.09178352230214,17.539143141048,-332.353493805869)) ;
#43959=CARTESIAN_POINT('Ctrl Pts',(5.91006512688105,17.6012073060264,-332.351068725161)) ;
#43960=CARTESIAN_POINT('Ctrl Pts',(5.60501782098526,17.700136493211,-332.346986704977)) ;
#43961=CARTESIAN_POINT('Ctrl Pts',(5.48220940392533,17.7385579077676,-332.345340404376)) ;
#43962=CARTESIAN_POINT('Ctrl Pts',(5.2479779908468,17.8091739115513,-332.342193862824)) ;
#43963=CARTESIAN_POINT('Ctrl Pts',(5.1366332503701,17.8416071925664,-332.340695324067)) ;
#43964=CARTESIAN_POINT('Ctrl Pts',(4.8393466680386,17.9251893063669,-332.336686494892)) ;
#43965=CARTESIAN_POINT('Ctrl Pts',(4.65289962161678,17.9744878305147,-332.334164148901)) ;
#43966=CARTESIAN_POINT('Ctrl Pts',(4.12886536216532,18.104347778357,-332.327054360683)) ;
#43967=CARTESIAN_POINT('Ctrl Pts',(3.78973842521158,18.1783612973032,-332.322428693141)) ;
#43968=CARTESIAN_POINT('Ctrl Pts',(2.94666925870943,18.3377403420374,-332.310917710426)) ;
#43969=CARTESIAN_POINT('Ctrl Pts',(2.44089739739492,18.4118874597571,-332.303998350793)) ;
#43970=CARTESIAN_POINT('Ctrl Pts',(1.76315019111453,18.4828262822888,-332.294888972572)) ;
#43971=CARTESIAN_POINT('Ctrl Pts',(1.59335062937464,18.4982377506453,-332.292620963726)) ;
#43972=CARTESIAN_POINT('Ctrl Pts',(1.29647590031274,18.5210649023294,-332.288692707784)) ;
#43973=CARTESIAN_POINT('Ctrl Pts',(1.16949187160357,18.5295165538559,-332.287024292567)) ;
#43974=CARTESIAN_POINT('Ctrl Pts',(0.9710841898059,18.5406742419482,-332.284441039087)) ;
#43975=CARTESIAN_POINT('Ctrl Pts',(0.899714873390939,18.5442745615462,-332.28351657957)) ;
#43976=CARTESIAN_POINT('Ctrl Pts',(0.766343673871551,18.5502308963782,-332.28179904819)) ;
#43977=CARTESIAN_POINT('Ctrl Pts',(0.704347327440994,18.552688316967,-332.281004737179)) ;
#43978=CARTESIAN_POINT('Ctrl Pts',(0.529057906255504,18.5587565666582,-332.278769032386)) ;
#43979=CARTESIAN_POINT('Ctrl Pts',(0.415742335773235,18.5616407124527,-332.277335726447)) ;
#43980=CARTESIAN_POINT('Ctrl Pts',(0.0693115659325736,18.5672842219207,
-332.272981803393)) ;
#43981=CARTESIAN_POINT('Ctrl Pts',(-0.163835487773185,18.5666907591766,
-332.270090173147)) ;
#43982=CARTESIAN_POINT('Ctrl Pts',(-0.986102803364694,18.5491080095177,
-332.259950270748)) ;
#43983=CARTESIAN_POINT('Ctrl Pts',(-1.57436197876308,18.5084627287234,-332.252791425826)) ;
#43984=CARTESIAN_POINT('Ctrl Pts',(-2.31906779467445,18.4212424554523,-332.243522692214)) ;
#43985=CARTESIAN_POINT('Ctrl Pts',(-2.47819651328581,18.4005106180862,-332.24153092838)) ;
#43986=CARTESIAN_POINT('Ctrl Pts',(-2.86452019720768,18.345076665137,-332.23666016997)) ;
#43987=CARTESIAN_POINT('Ctrl Pts',(-3.09137803399052,18.3082138774632,-332.233769998456)) ;
#43988=CARTESIAN_POINT('Ctrl Pts',(-3.45056971924063,18.2429811602815,-332.229135871343)) ;
#43989=CARTESIAN_POINT('Ctrl Pts',(-3.58337856930062,18.2173596046806,-332.227409808361)) ;
#43990=CARTESIAN_POINT('Ctrl Pts',(-3.83979184654705,18.1649797373889,-332.224051428984)) ;
#43991=CARTESIAN_POINT('Ctrl Pts',(-3.96342630264408,18.1384051717356,-332.222420410533)) ;
#43992=CARTESIAN_POINT('Ctrl Pts',(-4.26037602091029,18.0713963451136,-332.218474134592)) ;
#43993=CARTESIAN_POINT('Ctrl Pts',(-4.43340010096782,18.02972914661,-332.216150919435)) ;
#43994=CARTESIAN_POINT('Ctrl Pts',(-5.00416456956719,17.8835661761346,-332.208409585335)) ;
#43995=CARTESIAN_POINT('Ctrl Pts',(-5.39903066813865,17.7683445645606,-332.20292582453)) ;
#43996=CARTESIAN_POINT('Ctrl Pts',(-6.25178648474601,17.4884575226222,-332.190872454635)) ;
#43997=CARTESIAN_POINT('Ctrl Pts',(-6.70769267480531,17.3187135609337,-332.184290612481)) ;
#43998=CARTESIAN_POINT('Ctrl Pts',(-7.3782482857547,17.0385959802947,-332.174580095819)) ;
#43999=CARTESIAN_POINT('Ctrl Pts',(-7.59826845615552,16.9416238186769,-332.171390033838)) ;
#44000=CARTESIAN_POINT('Ctrl Pts',(-7.89686119614982,16.8030343213242,-332.167083336066)) ;
#44001=CARTESIAN_POINT('Ctrl Pts',(-7.97710997844837,16.7650856120041,-332.165928187547)) ;
#44002=CARTESIAN_POINT('Ctrl Pts',(-8.11631926401209,16.698029345755,-332.16393035829)) ;
#44003=CARTESIAN_POINT('Ctrl Pts',(-8.1754028196708,16.6691814789894,-332.163084472881)) ;
#44004=CARTESIAN_POINT('Ctrl Pts',(-8.31123330013605,16.6019656179091,-332.161144487101)) ;
#44005=CARTESIAN_POINT('Ctrl Pts',(-8.38786982435409,16.5633783143841,-332.160053154124)) ;
#44006=CARTESIAN_POINT('Ctrl Pts',(-8.64060995370358,16.4339170254216,-332.156460633363)) ;
#44007=CARTESIAN_POINT('Ctrl Pts',(-8.81552630842516,16.3407547356567,-332.153984876491)) ;
#44008=CARTESIAN_POINT('Ctrl Pts',(-9.03816107448489,16.2175618127977,-332.150829232131)) ;
#44009=CARTESIAN_POINT('Ctrl Pts',(-9.08728011015319,16.1900897762684,-332.150132740655)) ;
#44010=CARTESIAN_POINT('Ctrl Pts',(-9.22120697819413,16.1143836382101,-332.148232133249)) ;
#44011=CARTESIAN_POINT('Ctrl Pts',(-9.30576073844549,16.0657036966129,-332.147030463072)) ;
#44012=CARTESIAN_POINT('Ctrl Pts',(-9.85890925570984,15.7414087704791,-332.139147988091)) ;
#44013=CARTESIAN_POINT('Ctrl Pts',(-10.3155886990881,15.445992107346,-332.132531119088)) ;
#44014=CARTESIAN_POINT('Ctrl Pts',(-10.9419331163267,15.000639239088,-332.123022636887)) ;
#44015=CARTESIAN_POINT('Ctrl Pts',(-11.1228370586685,14.8669961139795,-332.12022354312)) ;
#44016=CARTESIAN_POINT('Ctrl Pts',(-11.4504935675418,14.615610573834,-332.115040357684)) ;
#44017=CARTESIAN_POINT('Ctrl Pts',(-11.5979703829345,14.4988605835497,-332.112663686875)) ;
#44018=CARTESIAN_POINT('Ctrl Pts',(-11.8428089869817,14.298907853711,-332.108638495641)) ;
#44019=CARTESIAN_POINT('Ctrl Pts',(-11.9411299575785,14.216902116562,-332.106999932647)) ;
#44020=CARTESIAN_POINT('Ctrl Pts',(-12.139362567579,14.0480566872367,-332.103649814877)) ;
#44021=CARTESIAN_POINT('Ctrl Pts',(-12.2392095031714,13.9611522056943,-332.101937762266)) ;
#44022=CARTESIAN_POINT('Ctrl Pts',(-12.4975661940141,13.7313826984516,-332.097442367107)) ;
#44023=CARTESIAN_POINT('Ctrl Pts',(-12.6545571176853,13.5868397888012,-332.094644894841)) ;
#44024=CARTESIAN_POINT('Ctrl Pts',(-13.0736108157426,13.1874485506062,-332.087000375313)) ;
#44025=CARTESIAN_POINT('Ctrl Pts',(-13.3306951254719,12.9275158326647,-332.082114429343)) ;
#44026=CARTESIAN_POINT('Ctrl Pts',(-14.0278265935417,12.1797370741932,-332.06837410686)) ;
#44027=CARTESIAN_POINT('Ctrl Pts',(-14.4499043209779,11.6758802185596,-332.059457614808)) ;
#44028=CARTESIAN_POINT('Ctrl Pts',(-14.9095618170519,11.0639613116525,-332.049396399595)) ;
#44029=CARTESIAN_POINT('Ctrl Pts',(-14.9739702815395,10.9766337072438,-332.047978287905)) ;
#44030=CARTESIAN_POINT('Ctrl Pts',(-15.0770662924487,10.8342557420151,-332.045698096177)) ;
#44031=CARTESIAN_POINT('Ctrl Pts',(-15.1162266290251,10.7795509187291,-332.044829539051)) ;
#44032=CARTESIAN_POINT('Ctrl Pts',(-15.1986425315683,10.6630881759881,-332.042997316525)) ;
#44033=CARTESIAN_POINT('Ctrl Pts',(-15.241820923789,10.6012772437411,-332.042034684985)) ;
#44034=CARTESIAN_POINT('Ctrl Pts',(-15.3687001440728,10.4172689734459,-332.039195359237)) ;
#44035=CARTESIAN_POINT('Ctrl Pts',(-15.4513166261285,10.2943310430235,-332.037332544137)) ;
#44036=CARTESIAN_POINT('Ctrl Pts',(-15.6487065940519,9.99287336646802,-332.032832334635)) ;
#44037=CARTESIAN_POINT('Ctrl Pts',(-15.7619073672448,9.81334869196136,-332.030208875802)) ;
#44038=CARTESIAN_POINT('Ctrl Pts',(-16.1934971425816,9.10215161073052,-332.019971947279)) ;
#44039=CARTESIAN_POINT('Ctrl Pts',(-16.4882631041592,8.55661701258747,-332.012442079409)) ;
#44040=CARTESIAN_POINT('Ctrl Pts',(-16.8782807517906,7.73949515207647,-332.001206907818)) ;
#44041=CARTESIAN_POINT('Ctrl Pts',(-16.9953944594917,7.47881762195041,-331.997631340447)) ;
#44042=CARTESIAN_POINT('Ctrl Pts',(-17.1625964651567,7.08241884168303,-331.992185373938)) ;
#44043=CARTESIAN_POINT('Ctrl Pts',(-17.2171920751507,6.94864526685041,-331.990346172324)) ;
#44044=CARTESIAN_POINT('Ctrl Pts',(-17.3158209906011,6.69867739422563,-331.986905106338)) ;
#44045=CARTESIAN_POINT('Ctrl Pts',(-17.3602600745358,6.58265185952819,-331.985306181384)) ;
#44046=CARTESIAN_POINT('Ctrl Pts',(-17.4588547502433,6.31728759638807,-331.981644679739)) ;
#44047=CARTESIAN_POINT('Ctrl Pts',(-17.5122650125048,6.16768236795628,-331.979577130581)) ;
#44048=CARTESIAN_POINT('Ctrl Pts',(-17.6944191665561,5.63600684395028,-331.972218226346)) ;
#44049=CARTESIAN_POINT('Ctrl Pts',(-17.812631024771,5.25044924461633,-331.966859117515)) ;
#44050=CARTESIAN_POINT('Ctrl Pts',(-18.0880249195642,4.23538935364533,-331.952760877219)) ;
#44051=CARTESIAN_POINT('Ctrl Pts',(-18.224934926767,3.60096010385872,-331.943949095296)) ;
#44052=CARTESIAN_POINT('Ctrl Pts',(-18.354300904181,2.80010566932789,-331.933190710941)) ;
#44053=CARTESIAN_POINT('Ctrl Pts',(-18.3781268292017,2.63920591150181,-331.931048473519)) ;
#44054=CARTESIAN_POINT('Ctrl Pts',(-18.4102387373538,2.40076742977382,-331.927912089315)) ;
#44055=CARTESIAN_POINT('Ctrl Pts',(-18.4201554109191,2.32345632151092,-331.926901083589)) ;
#44056=CARTESIAN_POINT('Ctrl Pts',(-18.4376988707512,2.17950865988861,-331.925031166317)) ;
#44057=CARTESIAN_POINT('Ctrl Pts',(-18.445451957283,2.11288895321875,-331.924170888186)) ;
#44058=CARTESIAN_POINT('Ctrl Pts',(-18.4641932931997,1.94388000924365,-331.922000292302)) ;
#44059=CARTESIAN_POINT('Ctrl Pts',(-18.4746909976233,1.84143858090557,-331.920695530287)) ;
#44060=CARTESIAN_POINT('Ctrl Pts',(-18.4962502282,1.61226806216169,-331.917796287431)) ;
#44061=CARTESIAN_POINT('Ctrl Pts',(-18.5068626495285,1.48550184971682,-331.916205942429)) ;
#44062=CARTESIAN_POINT('Ctrl Pts',(-18.5370632018517,1.07391375680445,-331.911073602429)) ;
#44063=CARTESIAN_POINT('Ctrl Pts',(-18.5513849105104,0.788746615629087,
-331.907565632499)) ;
#44064=CARTESIAN_POINT('Ctrl Pts',(-18.5782190912367,-0.200637317172788,
-331.89543262566)) ;
#44065=CARTESIAN_POINT('Ctrl Pts',(-18.5572405141425,-0.905154107683385,
-331.886837573715)) ;
#44066=CARTESIAN_POINT('Ctrl Pts',(-18.482756003825,-1.76258047396206,-331.876009761189)) ;
#44067=CARTESIAN_POINT('Ctrl Pts',(-18.4672525632684,-1.91821325567096,
-331.874030727184)) ;
#44068=CARTESIAN_POINT('Ctrl Pts',(-18.4356442133644,-2.19944320287778,
-331.87042684652)) ;
#44069=CARTESIAN_POINT('Ctrl Pts',(-18.4202173037977,-2.32510696351003,
-331.86880645419)) ;
#44070=CARTESIAN_POINT('Ctrl Pts',(-18.3860454622188,-2.58173021350686,
-331.865475793732)) ;
#44071=CARTESIAN_POINT('Ctrl Pts',(-18.3671836865879,-2.71266695255667,
-331.863764847945)) ;
#44072=CARTESIAN_POINT('Ctrl Pts',(-18.314315537329,-3.05379766475358,-331.859276691535)) ;
#44073=CARTESIAN_POINT('Ctrl Pts',(-18.2780898313619,-3.26362768249181,
-331.856485439161)) ;
#44074=CARTESIAN_POINT('Ctrl Pts',(-18.1685694300383,-3.83880301681021,
-331.848754020709)) ;
#44075=CARTESIAN_POINT('Ctrl Pts',(-18.0878735331925,-4.20263652678464,
-331.843772455376)) ;
#44076=CARTESIAN_POINT('Ctrl Pts',(-17.8369727094456,-5.19200689056596,
-331.83005204173)) ;
#44077=CARTESIAN_POINT('Ctrl Pts',(-17.6448752355142,-5.81144634958503,
-331.821256627717)) ;
#44078=CARTESIAN_POINT('Ctrl Pts',(-17.3828153877897,-6.52259802301906,
-331.811290390954)) ;
#44079=CARTESIAN_POINT('Ctrl Pts',(-17.343935905551,-6.62528815485775,-331.809855037285)) ;
#44080=CARTESIAN_POINT('Ctrl Pts',(-17.2818738063739,-6.7849182387354,-331.80763302811)) ;
#44081=CARTESIAN_POINT('Ctrl Pts',(-17.2593154769174,-6.84209814715091,
-331.80683896384)) ;
#44082=CARTESIAN_POINT('Ctrl Pts',(-17.2095486636328,-6.96643266519715,
-331.805117228929)) ;
#44083=CARTESIAN_POINT('Ctrl Pts',(-17.1822301862727,-7.03354214666233,
-331.804191000133)) ;
#44084=CARTESIAN_POINT('Ctrl Pts',(-17.1038883530322,-7.22281309858469,
-331.801585299412)) ;
#44085=CARTESIAN_POINT('Ctrl Pts',(-17.0519501789276,-7.34459127760275,
-331.799916534015)) ;
#44086=CARTESIAN_POINT('Ctrl Pts',(-16.9262038767758,-7.63090009558715,
-331.796001182187)) ;
#44087=CARTESIAN_POINT('Ctrl Pts',(-16.8512923805617,-7.7949316355332,-331.793764295144)) ;
#44088=CARTESIAN_POINT('Ctrl Pts',(-16.522771143864,-8.48740750170448,-331.784304876384)) ;
#44089=CARTESIAN_POINT('Ctrl Pts',(-16.2466022108365,-9.00477488440505,
-331.777186250456)) ;
#44090=CARTESIAN_POINT('Ctrl Pts',(-15.7719329963083,-9.80085278874171,
-331.765741430216)) ;
#44091=CARTESIAN_POINT('Ctrl Pts',(-15.5894200194946,-10.0886356137815,
-331.761498829468)) ;
#44092=CARTESIAN_POINT('Ctrl Pts',(-15.3118355723882,-10.5007899538457,
-331.755226136013)) ;
#44093=CARTESIAN_POINT('Ctrl Pts',(-15.2229476208506,-10.6292409835721,
-331.753242599147)) ;
#44094=CARTESIAN_POINT('Ctrl Pts',(-15.060561513905,-10.8576876914856,-331.749660603606)) ;
#44095=CARTESIAN_POINT('Ctrl Pts',(-14.9876616231509,-10.9580971951812,
-331.748066943469)) ;
#44096=CARTESIAN_POINT('Ctrl Pts',(-14.8265571237866,-11.1753809992731,
-331.744575225948)) ;
#44097=CARTESIAN_POINT('Ctrl Pts',(-14.7379653691483,-11.291957904565,-331.742674122081)) ;
#44098=CARTESIAN_POINT('Ctrl Pts',(-14.4644798384884,-11.643132666103,-331.736862131884)) ;
#44099=CARTESIAN_POINT('Ctrl Pts',(-14.2752958122166,-11.8743271014631,
-331.732917557379)) ;
#44100=CARTESIAN_POINT('Ctrl Pts',(-13.7758045688742,-12.4555376226363,
-331.72271140743)) ;
#44101=CARTESIAN_POINT('Ctrl Pts',(-13.4576999457132,-12.7985749121859,
-331.716402170961)) ;
#44102=CARTESIAN_POINT('Ctrl Pts',(-13.0175413938636,-13.2386580457913,
-331.708021896245)) ;
#44103=CARTESIAN_POINT('Ctrl Pts',(-12.9067345198133,-13.3467095145243,
-331.705940395454)) ;
#44104=CARTESIAN_POINT('Ctrl Pts',(-12.585874295672,-13.6518581169642,-331.700005083862)) ;
#44105=CARTESIAN_POINT('Ctrl Pts',(-12.3725675824531,-13.8454697949743,
-331.696168941875)) ;
#44106=CARTESIAN_POINT('Ctrl Pts',(-12.0903131565385,-14.0899295538039,
-331.691276097674)) ;
#44107=CARTESIAN_POINT('Ctrl Pts',(-12.0253987302987,-14.1453728285473,
-331.690163031979)) ;
#44108=CARTESIAN_POINT('Ctrl Pts',(-11.9088513873796,-14.243533560263,-331.68818812439)) ;
#44109=CARTESIAN_POINT('Ctrl Pts',(-11.8573652216639,-14.2864229143945,
-331.687323798843)) ;
#44110=CARTESIAN_POINT('Ctrl Pts',(-11.7453469840887,-14.378714410044,-331.685461532607)) ;
#44111=CARTESIAN_POINT('Ctrl Pts',(-11.6847330806349,-14.4280149957899,
-331.684465030554)) ;
#44112=CARTESIAN_POINT('Ctrl Pts',(-11.496118967138,-14.5794569338287,-331.681395705522)) ;
#44113=CARTESIAN_POINT('Ctrl Pts',(-11.367077125032,-14.6802886069379,-331.679340252255)) ;
#44114=CARTESIAN_POINT('Ctrl Pts',(-10.8345928260364,-15.0851342673703,
-331.67100485757)) ;
#44115=CARTESIAN_POINT('Ctrl Pts',(-10.4201564032763,-15.3743299149691,
-331.664849149507)) ;
#44116=CARTESIAN_POINT('Ctrl Pts',(-9.55254222534979,-15.9285401780937,
-331.652227925905)) ;
#44117=CARTESIAN_POINT('Ctrl Pts',(-9.09888186648572,-16.1919672162433,
-331.645764047552)) ;
#44118=CARTESIAN_POINT('Ctrl Pts',(-8.50170607225066,-16.5056976929444,
-331.637266746582)) ;
#44119=CARTESIAN_POINT('Ctrl Pts',(-8.36788715208434,-16.5739412028438,
-331.635363940735)) ;
#44120=CARTESIAN_POINT('Ctrl Pts',(-8.11984223289753,-16.6966665136509,
-331.631836754783)) ;
#44121=CARTESIAN_POINT('Ctrl Pts',(-8.00585889708348,-16.7516188418197,
-331.63021586359)) ;
#44122=CARTESIAN_POINT('Ctrl Pts',(-7.76905820725154,-16.8628134880897,
-331.626847376093)) ;
#44123=CARTESIAN_POINT('Ctrl Pts',(-7.64617082176527,-16.9188893211251,
-331.625098706403)) ;
#44124=CARTESIAN_POINT('Ctrl Pts',(-7.31352357533365,-17.0663180829324,
-331.620363199763)) ;
#44125=CARTESIAN_POINT('Ctrl Pts',(-7.1026693458332,-17.1551428982102,-331.617359216536)) ;
#44126=CARTESIAN_POINT('Ctrl Pts',(-6.74222807817581,-17.2991983230211,
-331.6122239784)) ;
#44127=CARTESIAN_POINT('Ctrl Pts',(-6.593472910062,-17.3564402162134,-331.610104690238)) ;
#44128=CARTESIAN_POINT('Ctrl Pts',(-5.8994400066628,-17.6132980899344,-331.600225387217)) ;
#44129=CARTESIAN_POINT('Ctrl Pts',(-5.3457271956127,-17.7891781870182,-331.592356568875)) ;
#44130=CARTESIAN_POINT('Ctrl Pts',(-4.51125014092158,-18.0117519289392,
-331.580782584627)) ;
#44131=CARTESIAN_POINT('Ctrl Pts',(-4.236182275916,-18.0784221014574,-331.5770145252)) ;
#44132=CARTESIAN_POINT('Ctrl Pts',(-3.87623896552559,-18.1569977751432,
-331.572186867686)) ;
#44133=CARTESIAN_POINT('Ctrl Pts',(-3.79265524224161,-18.1746406557301,
-331.571073047531)) ;
#44134=CARTESIAN_POINT('Ctrl Pts',(-3.64328296360497,-18.2050949028238,
-331.569097235563)) ;
#44135=CARTESIAN_POINT('Ctrl Pts',(-3.57754117068616,-18.2181280702942,
-331.568232752751)) ;
#44136=CARTESIAN_POINT('Ctrl Pts',(-3.43504503767567,-18.2455765537329,
-331.566370786161)) ;
#44137=CARTESIAN_POINT('Ctrl Pts',(-3.35826753299521,-18.2598641119797,
-331.565374734357)) ;
#44138=CARTESIAN_POINT('Ctrl Pts',(-3.12043525453086,-18.3025716510351,
-331.562308562521)) ;
#44139=CARTESIAN_POINT('Ctrl Pts',(-2.95909324587885,-18.3293483937127,
-331.560255761816)) ;
#44140=CARTESIAN_POINT('Ctrl Pts',(-2.29837045352273,-18.4300522776387,
-331.551927054896)) ;
#44141=CARTESIAN_POINT('Ctrl Pts',(-1.79642693013304,-18.4857292583713,
-331.545775359711)) ;
#44142=CARTESIAN_POINT('Ctrl Pts',(-0.812797026515212,-18.5543909502474,
-331.533687473049)) ;
#44143=CARTESIAN_POINT('Ctrl Pts',(-0.331634497858101,-18.5692239972279,
-331.527759330114)) ;
#44144=CARTESIAN_POINT('Ctrl Pts',(0.335011049879787,-18.5638536358676,
-331.519388768985)) ;
#44145=CARTESIAN_POINT('Ctrl Pts',(0.520430378490183,-18.5595809834996,
-331.517044472027)) ;
#44146=CARTESIAN_POINT('Ctrl Pts',(0.832001976769622,-18.5477285307899,
-331.513073261548)) ;
#44147=CARTESIAN_POINT('Ctrl Pts',(0.958197217835081,-18.5416374406286,
-331.511456020372)) ;
#44148=CARTESIAN_POINT('Ctrl Pts',(1.2168000838953,-18.5265082493368,-331.50812288899)) ;
#44149=CARTESIAN_POINT('Ctrl Pts',(1.34919279268154,-18.5173375273755,-331.506406227867)) ;
#44150=CARTESIAN_POINT('Ctrl Pts',(1.69610351393776,-18.4895671278544,-331.50188069614)) ;
#44151=CARTESIAN_POINT('Ctrl Pts',(1.91041589647847,-18.4686537288215,-331.499057329471)) ;
#44152=CARTESIAN_POINT('Ctrl Pts',(2.39590829321267,-18.4127364592579,-331.492602293534)) ;
#44153=CARTESIAN_POINT('Ctrl Pts',(2.66677643416566,-18.3754603618096,-331.48895856669)) ;
#44154=CARTESIAN_POINT('Ctrl Pts',(3.28288049015549,-18.2767638210294,-331.480596404203)) ;
#44155=CARTESIAN_POINT('Ctrl Pts',(3.62739871416073,-18.2115177380719,-331.475866068262)) ;
#44156=CARTESIAN_POINT('Ctrl Pts',(4.06211988287781,-18.1163627901775,-331.469876197196)) ;
#44157=CARTESIAN_POINT('Ctrl Pts',(4.15422219233511,-18.095465085836,-331.468606048662)) ;
#44158=CARTESIAN_POINT('Ctrl Pts',(4.559525554593,-18.0002456461708,-331.463016086596)) ;
#44159=CARTESIAN_POINT('Ctrl Pts',(4.87092308454382,-17.9184883751614,-331.458718829005)) ;
#44160=CARTESIAN_POINT('Ctrl Pts',(5.2740535943237,-17.8013607134388,-331.453213303412)) ;
#44161=CARTESIAN_POINT('Ctrl Pts',(5.36785214476087,-17.7733015491847,-331.451936506685)) ;
#44162=CARTESIAN_POINT('Ctrl Pts',(5.52488445153144,-17.7249699538037,-331.449808603074)) ;
#44163=CARTESIAN_POINT('Ctrl Pts',(5.58823923867938,-17.7050978622671,-331.448952823472)) ;
#44164=CARTESIAN_POINT('Ctrl Pts',(5.72820564884005,-17.660369372822,-331.447068775207)) ;
#44165=CARTESIAN_POINT('Ctrl Pts',(5.80476473127387,-17.6353534917356,-331.446042377354)) ;
#44166=CARTESIAN_POINT('Ctrl Pts',(6.05057109729312,-17.5532615349998,-331.442756981622)) ;
#44167=CARTESIAN_POINT('Ctrl Pts',(6.21915853939948,-17.4942410060972,-331.440518976821)) ;
#44168=CARTESIAN_POINT('Ctrl Pts',(6.6527138797483,-17.3353989774364,-331.434776098598)) ;
#44169=CARTESIAN_POINT('Ctrl Pts',(6.91629713058768,-17.231932395471,-331.431296590616)) ;
#44170=CARTESIAN_POINT('Ctrl Pts',(7.8326643082319,-16.8478090348305,-331.419115265044)) ;
#44171=CARTESIAN_POINT('Ctrl Pts',(8.47161110839537,-16.5357523040289,-331.410445819442)) ;
#44172=CARTESIAN_POINT('Ctrl Pts',(9.22661848126712,-16.1117401110325,-331.399549676209)) ;
#44173=CARTESIAN_POINT('Ctrl Pts',(9.36117863113241,-16.0339325353331,-331.397582551302)) ;
#44174=CARTESIAN_POINT('Ctrl Pts',(9.60335744134876,-15.8898080428494,-331.393993254042)) ;
#44175=CARTESIAN_POINT('Ctrl Pts',(9.71130616221606,-15.8240641541709,-331.392375409092)) ;
#44176=CARTESIAN_POINT('Ctrl Pts',(9.93113454678339,-15.6870856100257,-331.389042781119)) ;
#44177=CARTESIAN_POINT('Ctrl Pts',(10.0429391620492,-15.6157440183855,-331.387327245373)) ;
#44178=CARTESIAN_POINT('Ctrl Pts',(10.3338336504723,-15.4257103199362,-331.382809072979)) ;
#44179=CARTESIAN_POINT('Ctrl Pts',(10.5116442313536,-15.3050969318215,-331.379992030126)) ;
#44180=CARTESIAN_POINT('Ctrl Pts',(10.9101489418954,-15.0245601684591,-331.373555269436)) ;
#44181=CARTESIAN_POINT('Ctrl Pts',(11.1294957261104,-14.8628087071858,-331.369923603706)) ;
#44182=CARTESIAN_POINT('Ctrl Pts',(11.6236155285815,-14.4813593904754,-331.361558434222)) ;
#44183=CARTESIAN_POINT('Ctrl Pts',(11.895864919779,-14.2585625232433,-331.356812603603)) ;
#44184=CARTESIAN_POINT('Ctrl Pts',(12.1713405341519,-14.0197408851476,-331.351905238972)) ;
#44185=CARTESIAN_POINT('Ctrl Pts',(12.1810516282365,-14.0113042260604,-331.351732106986)) ;
#44186=CARTESIAN_POINT('Ctrl Pts',(12.4691174520005,-13.7605168719309,-331.346592388863)) ;
#44187=CARTESIAN_POINT('Ctrl Pts',(12.7401933053267,-13.5099293110937,-331.341642916547)) ;
#44188=CARTESIAN_POINT('Ctrl Pts',(13.0860464946712,-13.1705437657862,-331.335263791768)) ;
#44189=CARTESIAN_POINT('Ctrl Pts',(13.1677166864622,-13.0888912164082,-331.333752638941)) ;
#44190=CARTESIAN_POINT('Ctrl Pts',(13.2923361147654,-12.9619517844708,-331.331443164222)) ;
#44191=CARTESIAN_POINT('Ctrl Pts',(13.33582765902,-12.9172014814219,-331.330636478535)) ;
#44192=CARTESIAN_POINT('Ctrl Pts',(13.4282651881927,-12.8211241103788,-331.328921334361)) ;
#44193=CARTESIAN_POINT('Ctrl Pts',(13.4771443639001,-12.7697341095066,-331.328014043487)) ;
#44194=CARTESIAN_POINT('Ctrl Pts',(13.6110335365427,-12.6273422848489,-331.32552585105)) ;
#44195=CARTESIAN_POINT('Ctrl Pts',(13.6954243430963,-12.5357632097247,-331.323954196127)) ;
#44196=CARTESIAN_POINT('Ctrl Pts',(13.8897140754676,-12.3206203347204,-331.320319419235)) ;
#44197=CARTESIAN_POINT('Ctrl Pts',(13.9988963246096,-12.1964234243719,-331.318264232337)) ;
#44198=CARTESIAN_POINT('Ctrl Pts',(14.416287535097,-11.7086432430554,-331.310327075914)) ;
#44199=CARTESIAN_POINT('Ctrl Pts',(14.7121100633971,-11.3347029741908,-331.304522422716)) ;
#44200=CARTESIAN_POINT('Ctrl Pts',(15.2590919205798,-10.5857376221815,-331.293132577096)) ;
#44201=CARTESIAN_POINT('Ctrl Pts',(15.511620235248,-10.2121184692607,-331.287556523951)) ;
#44202=CARTESIAN_POINT('Ctrl Pts',(15.8298309562162,-9.70224288055688,-331.279985662157)) ;
#44203=CARTESIAN_POINT('Ctrl Pts',(15.9078139956106,-9.57384556028879,-331.278082751899)) ;
#44204=CARTESIAN_POINT('Ctrl Pts',(16.0485996199982,-9.33557503486647,-331.274555440085)) ;
#44205=CARTESIAN_POINT('Ctrl Pts',(16.1118535889376,-9.22597880279746,-331.272934528528)) ;
#44206=CARTESIAN_POINT('Ctrl Pts',(16.2403002102788,-8.99807713892284,-331.269566072056)) ;
#44207=CARTESIAN_POINT('Ctrl Pts',(16.3053321333934,-8.87968958196487,-331.267817454528)) ;
#44208=CARTESIAN_POINT('Ctrl Pts',(16.4770092900949,-8.55891317545061,-331.263082291909)) ;
#44209=CARTESIAN_POINT('Ctrl Pts',(16.581215168311,-8.35524584512619,-331.260078605022)) ;
#44210=CARTESIAN_POINT('Ctrl Pts',(16.7515828989432,-8.00652016055762,-331.254943978081)) ;
#44211=CARTESIAN_POINT('Ctrl Pts',(16.8196886150558,-7.8624404297601,-331.252825003968)) ;
#44212=CARTESIAN_POINT('Ctrl Pts',(17.1272227276842,-7.1895543275475,-331.24294847965)) ;
#44213=CARTESIAN_POINT('Ctrl Pts',(17.3436213189177,-6.65058246789319,-331.235082189139)) ;
#44214=CARTESIAN_POINT('Ctrl Pts',(17.627519564387,-5.83483442152804,-331.223506895498)) ;
#44215=CARTESIAN_POINT('Ctrl Pts',(17.7144902594939,-5.56521105949688,-331.219735182345)) ;
#44216=CARTESIAN_POINT('Ctrl Pts',(17.8196119877708,-5.21183495058931,-331.214904127218)) ;
#44217=CARTESIAN_POINT('Ctrl Pts',(17.8434008144712,-5.129799445204,-331.213790445708)) ;
#44218=CARTESIAN_POINT('Ctrl Pts',(17.8848433319184,-4.98310845616582,-331.211814799966)) ;
#44219=CARTESIAN_POINT('Ctrl Pts',(17.9027146294807,-4.91851601892527,-331.210950346085)) ;
#44220=CARTESIAN_POINT('Ctrl Pts',(17.9406544522097,-4.77844295313092,-331.209088324576)) ;
#44221=CARTESIAN_POINT('Ctrl Pts',(17.9605971858126,-4.70292972316742,-331.208092190145)) ;
#44222=CARTESIAN_POINT('Ctrl Pts',(18.0208330490043,-4.46887394962515,-331.205025439859)) ;
#44223=CARTESIAN_POINT('Ctrl Pts',(18.0595078288074,-4.30992288747495,-331.202972152571)) ;
#44224=CARTESIAN_POINT('Ctrl Pts',(18.2089432480868,-3.65838523819651,-331.194642218824)) ;
#44225=CARTESIAN_POINT('Ctrl Pts',(18.3016899892517,-3.16188907643606,-331.188489787503)) ;
#44226=CARTESIAN_POINT('Ctrl Pts',(18.4430680056035,-2.18613150994227,-331.176402817181)) ;
#44227=CARTESIAN_POINT('Ctrl Pts',(18.4935194747455,-1.70753173741242,-331.170476360176)) ;
#44228=CARTESIAN_POINT('Ctrl Pts',(18.5327994065473,-1.1147295427976,-331.163016922969)) ;
#44229=CARTESIAN_POINT('Ctrl Pts',(18.539242482585,-1.00187985714273,-331.161591898881)) ;
#44230=CARTESIAN_POINT('Ctrl Pts',(18.5446545937584,-0.888979977668651,
-331.160160528407)) ;
#44231=CARTESIAN_POINT('Ctrl Pts',(18.544654593739,-0.888979978073095,-330.86430516735)) ;
#44232=CARTESIAN_POINT('Ctrl Pts',(18.5441097763335,-0.900345195346051,
-330.864456223428)) ;
#44233=CARTESIAN_POINT('Ctrl Pts',(18.5435545061637,-0.911710013754673,
-330.864607211556)) ;
#44234=CARTESIAN_POINT('Ctrl Pts',(18.5348507836707,-1.08655293568775,-330.866929103306)) ;
#44235=CARTESIAN_POINT('Ctrl Pts',(18.5245512397169,-1.24991694824044,-330.869085215214)) ;
#44236=CARTESIAN_POINT('Ctrl Pts',(18.5061469696207,-1.49101515632244,-330.872237563732)) ;
#44237=CARTESIAN_POINT('Ctrl Pts',(18.4997095493716,-1.56886853138097,-330.873250895538)) ;
#44238=CARTESIAN_POINT('Ctrl Pts',(18.4868372992938,-1.71342839907376,-330.875122446275)) ;
#44239=CARTESIAN_POINT('Ctrl Pts',(18.4805322972729,-1.78014499661427,-330.875982063671)) ;
#44240=CARTESIAN_POINT('Ctrl Pts',(18.4653723774058,-1.93179021210006,-330.877927551247)) ;
#44241=CARTESIAN_POINT('Ctrl Pts',(18.4562924851722,-2.01669486741578,-330.879010892966)) ;
#44242=CARTESIAN_POINT('Ctrl Pts',(18.4144730367111,-2.38377329764873,-330.883674247619)) ;
#44243=CARTESIAN_POINT('Ctrl Pts',(18.3758455132984,-2.66523820544436,-330.887198317088)) ;
#44244=CARTESIAN_POINT('Ctrl Pts',(18.2648938052935,-3.35567733726642,-330.89581417164)) ;
#44245=CARTESIAN_POINT('Ctrl Pts',(18.1852774394334,-3.76332314152292,-330.900877732374)) ;
#44246=CARTESIAN_POINT('Ctrl Pts',(18.0219310007999,-4.47236939637491,-330.909813241256)) ;
#44247=CARTESIAN_POINT('Ctrl Pts',(17.9441300679829,-4.77496394854851,-330.913667590865)) ;
#44248=CARTESIAN_POINT('Ctrl Pts',(17.7944207332213,-5.30173860754561,-330.920497826828)) ;
#44249=CARTESIAN_POINT('Ctrl Pts',(17.7258147158665,-5.52678331913014,-330.923454754092)) ;
#44250=CARTESIAN_POINT('Ctrl Pts',(17.6107652535368,-5.8799657432534,-330.928168356854)) ;
#44251=CARTESIAN_POINT('Ctrl Pts',(17.5671559334044,-6.00900010839035,-330.929905985652)) ;
#44252=CARTESIAN_POINT('Ctrl Pts',(17.4804553548932,-6.25652243519602,-330.933270674963)) ;
#44253=CARTESIAN_POINT('Ctrl Pts',(17.4375691811663,-6.3750743834906,-330.934896251667)) ;
#44254=CARTESIAN_POINT('Ctrl Pts',(17.3321846373426,-6.65737115925951,-330.938801366615)) ;
#44255=CARTESIAN_POINT('Ctrl Pts',(17.2685685885039,-6.8206857293893,-330.941088429854)) ;
#44256=CARTESIAN_POINT('Ctrl Pts',(16.9445284381231,-7.61895144320848,-330.952403088899)) ;
#44257=CARTESIAN_POINT('Ctrl Pts',(16.6513495227622,-8.24002530095249,-330.961654295319)) ;
#44258=CARTESIAN_POINT('Ctrl Pts',(16.1345251515381,-9.19405277906069,-330.97626331395)) ;
#44259=CARTESIAN_POINT('Ctrl Pts',(15.9333390915501,-9.53845976463505,-330.981619257573)) ;
#44260=CARTESIAN_POINT('Ctrl Pts',(15.6587906480133,-9.97549737373529,-330.988416315131)) ;
#44261=CARTESIAN_POINT('Ctrl Pts',(15.5954211016994,-10.0742797825858,-330.989952483218)) ;
#44262=CARTESIAN_POINT('Ctrl Pts',(15.4930181431378,-10.2306267590345,-330.99237947787)) ;
#44263=CARTESIAN_POINT('Ctrl Pts',(15.4545905330348,-10.288584283351,-330.993278182759)) ;
#44264=CARTESIAN_POINT('Ctrl Pts',(15.3804165740384,-10.3991021518454,-330.994988967119)) ;
#44265=CARTESIAN_POINT('Ctrl Pts',(15.3447241745437,-10.4516974494597,-330.995801905428)) ;
#44266=CARTESIAN_POINT('Ctrl Pts',(15.2396353103713,-10.6048547074545,-330.998167096647)) ;
#44267=CARTESIAN_POINT('Ctrl Pts',(15.1695153439629,-10.704916256608,-330.999709709479)) ;
#44268=CARTESIAN_POINT('Ctrl Pts',(14.9737474582542,-10.9784916136851,-331.003929616931)) ;
#44269=CARTESIAN_POINT('Ctrl Pts',(14.8460760999724,-11.1505343256369,-331.006586092132)) ;
#44270=CARTESIAN_POINT('Ctrl Pts',(14.3548839927377,-11.7890418912718,-331.016519408154)) ;
#44271=CARTESIAN_POINT('Ctrl Pts',(13.9721238991995,-12.2402597394375,-331.023702298116)) ;
#44272=CARTESIAN_POINT('Ctrl Pts',(13.4587842694715,-12.7898966129418,-331.032998896299)) ;
#44273=CARTESIAN_POINT('Ctrl Pts',(13.3475642182002,-12.9059233977497,-331.034993696942)) ;
#44274=CARTESIAN_POINT('Ctrl Pts',(13.0735143328098,-13.1844850527023,-331.039870406405)) ;
#44275=CARTESIAN_POINT('Ctrl Pts',(12.9091429360226,-13.3454655780042,-331.042763497922)) ;
#44276=CARTESIAN_POINT('Ctrl Pts',(12.6434200022662,-13.5962029582196,-331.047401101902)) ;
#44277=CARTESIAN_POINT('Ctrl Pts',(12.5440053229398,-13.6879777406398,-331.049127671882)) ;
#44278=CARTESIAN_POINT('Ctrl Pts',(12.3497617804306,-13.8634003642929,-331.052486312486)) ;
#44279=CARTESIAN_POINT('Ctrl Pts',(12.2550639238409,-13.9471822911523,-331.054117076876)) ;
#44280=CARTESIAN_POINT('Ctrl Pts',(12.0251287578649,-14.1464625951566,-331.05806146061)) ;
#44281=CARTESIAN_POINT('Ctrl Pts',(11.8890734092209,-14.2609978235547,-331.060383017681)) ;
#44282=CARTESIAN_POINT('Ctrl Pts',(11.2354921139579,-14.7953463681454,-331.0714750165)) ;
#44283=CARTESIAN_POINT('Ctrl Pts',(10.6972576826663,-15.1890496338167,-331.080453013357)) ;
#44284=CARTESIAN_POINT('Ctrl Pts',(9.79526015437213,-15.7770649091209,-331.094952856296)) ;
#44285=CARTESIAN_POINT('Ctrl Pts',(9.44415561414358,-15.9897099508716,-331.100468227632)) ;
#44286=CARTESIAN_POINT('Ctrl Pts',(8.98285514861447,-16.248596314188,-331.107436316812)) ;
#44287=CARTESIAN_POINT('Ctrl Pts',(8.8788626047792,-16.3056544706181,-331.108989249766)) ;
#44288=CARTESIAN_POINT('Ctrl Pts',(8.71283755442982,-16.3946890787099,-331.111435995875)) ;
#44289=CARTESIAN_POINT('Ctrl Pts',(8.65115926415511,-16.4273190647436,-331.112337903359)) ;
#44290=CARTESIAN_POINT('Ctrl Pts',(8.53315121297165,-16.4889005324727,-331.114049008568)) ;
#44291=CARTESIAN_POINT('Ctrl Pts',(8.47685443375419,-16.5179129830148,-331.114859118253)) ;
#44292=CARTESIAN_POINT('Ctrl Pts',(8.31268276261775,-16.6014582278814,-331.117205073238)) ;
#44293=CARTESIAN_POINT('Ctrl Pts',(8.20442230960213,-16.655226346107,-331.118731513974)) ;
#44294=CARTESIAN_POINT('Ctrl Pts',(7.90039294779327,-16.8025404115189,-331.122970471546)) ;
#44295=CARTESIAN_POINT('Ctrl Pts',(7.7034977824425,-16.8937176250662,-331.125661039915)) ;
#44296=CARTESIAN_POINT('Ctrl Pts',(6.96443610819583,-17.2203507106018,-331.135624246862)) ;
#44297=CARTESIAN_POINT('Ctrl Pts',(6.4127212551024,-17.4333260332723,-331.142803587748)) ;
#44298=CARTESIAN_POINT('Ctrl Pts',(5.69929878068553,-17.6702662954348,-331.152096073932)) ;
#44299=CARTESIAN_POINT('Ctrl Pts',(5.54615768729234,-17.7189292107757,-331.154090427393)) ;
#44300=CARTESIAN_POINT('Ctrl Pts',(5.1723034991462,-17.832405433101,-331.158966260683)) ;
#44301=CARTESIAN_POINT('Ctrl Pts',(4.95098045828004,-17.8951166311051,-331.161858922365)) ;
#44302=CARTESIAN_POINT('Ctrl Pts',(4.59772196794183,-17.9881559723658,-331.166496014513)) ;
#44303=CARTESIAN_POINT('Ctrl Pts',(4.46652158474351,-18.021181632986,-331.168222509841)) ;
#44304=CARTESIAN_POINT('Ctrl Pts',(4.21202743047192,-18.0822927554013,-331.171581111831)) ;
#44305=CARTESIAN_POINT('Ctrl Pts',(4.08878450538391,-18.1105584558184,-331.173211913479)) ;
#44306=CARTESIAN_POINT('Ctrl Pts',(3.79151063264642,-18.1755489379813,-331.177156575053)) ;
#44307=CARTESIAN_POINT('Ctrl Pts',(3.61722204271559,-18.2110361215927,-331.179478375634)) ;
#44308=CARTESIAN_POINT('Ctrl Pts',(2.78711546092656,-18.3676683775864,-331.190577515518)) ;
#44309=CARTESIAN_POINT('Ctrl Pts',(2.12559543858863,-18.4559229449141,-331.199562777584)) ;
#44310=CARTESIAN_POINT('Ctrl Pts',(1.15854057714928,-18.5322474007988,-331.212626014104)) ;
#44311=CARTESIAN_POINT('Ctrl Pts',(0.855773602491591,-18.5486943440046,
-331.216702170191)) ;
#44312=CARTESIAN_POINT('Ctrl Pts',(0.366577110325669,-18.5632650127573,
-331.223210402425)) ;
#44313=CARTESIAN_POINT('Ctrl Pts',(0.180341342491163,-18.5660082890026,
-331.225669690197)) ;
#44314=CARTESIAN_POINT('Ctrl Pts',(-0.0876156468409861,-18.5659230735206,
-331.22916757371)) ;
#44315=CARTESIAN_POINT('Ctrl Pts',(-0.169326398501262,-18.5653576536056,
-331.2302287745)) ;
#44316=CARTESIAN_POINT('Ctrl Pts',(-0.317213538112543,-18.5633578839317,
-331.232137936549)) ;
#44317=CARTESIAN_POINT('Ctrl Pts',(-0.38339085125449,-18.5621090344773,
-331.232987929659)) ;
#44318=CARTESIAN_POINT('Ctrl Pts',(-0.545502099660334,-18.5581824840665,
-331.235060209075)) ;
#44319=CARTESIAN_POINT('Ctrl Pts',(-0.641424653954942,-18.5551147693579,
-331.236278075621)) ;
#44320=CARTESIAN_POINT('Ctrl Pts',(-1.05959377305711,-18.5384946910379,
-331.241558517715)) ;
#44321=CARTESIAN_POINT('Ctrl Pts',(-1.38148069268011,-18.5172902016032,
-331.245549481872)) ;
#44322=CARTESIAN_POINT('Ctrl Pts',(-2.31060338030414,-18.4317213301951,
-331.257023430549)) ;
#44323=CARTESIAN_POINT('Ctrl Pts',(-2.91542254265853,-18.3457774854192,
-331.264446047105)) ;
#44324=CARTESIAN_POINT('Ctrl Pts',(-3.79144351382164,-18.1768746233684,
-331.275520600804)) ;
#44325=CARTESIAN_POINT('Ctrl Pts',(-4.06673109238057,-18.1172711174393,
-331.279045922301)) ;
#44326=CARTESIAN_POINT('Ctrl Pts',(-4.48041862951445,-18.0177978950799,
-331.2844327952)) ;
#44327=CARTESIAN_POINT('Ctrl Pts',(-4.61988588248379,-17.9825428246323,
-331.286264236867)) ;
#44328=CARTESIAN_POINT('Ctrl Pts',(-4.87794249438734,-17.9141099879679,
-331.289683369772)) ;
#44329=CARTESIAN_POINT('Ctrl Pts',(-4.99663878565135,-17.8813662910714,
-331.291268074259)) ;
#44330=CARTESIAN_POINT('Ctrl Pts',(-5.26793522173483,-17.8036139041292,
-331.29491844428)) ;
#44331=CARTESIAN_POINT('Ctrl Pts',(-5.42030009698362,-17.7578195818207,
-331.296989266319)) ;
#44332=CARTESIAN_POINT('Ctrl Pts',(-5.9591785416877,-17.5882741672656,-331.304386606565)) ;
#44333=CARTESIAN_POINT('Ctrl Pts',(-6.34220099019749,-17.453815690401,-331.309781902109)) ;
#44334=CARTESIAN_POINT('Ctrl Pts',(-7.10537514608677,-17.1574648868725,
-331.320757430125)) ;
#44335=CARTESIAN_POINT('Ctrl Pts',(-7.48515017746701,-16.9952194358773,
-331.326336177218)) ;
#44336=CARTESIAN_POINT('Ctrl Pts',(-8.17091560180506,-16.6748018809099,
-331.336507069752)) ;
#44337=CARTESIAN_POINT('Ctrl Pts',(-8.47852385226896,-16.5205179601351,
-331.341106013271)) ;
#44338=CARTESIAN_POINT('Ctrl Pts',(-8.86846276489182,-16.3111793646129,
-331.346911105294)) ;
#44339=CARTESIAN_POINT('Ctrl Pts',(-8.95488619290344,-16.2638930576343,
-331.348196006464)) ;
#44340=CARTESIAN_POINT('Ctrl Pts',(-9.0989852571619,-16.1835529131439,-331.350332932471)) ;
#44341=CARTESIAN_POINT('Ctrl Pts',(-9.15686703757934,-16.1508731557966,
-331.351189727604)) ;
#44342=CARTESIAN_POINT('Ctrl Pts',(-9.28419381412733,-16.0780806075834,
-331.35307044433)) ;
#44343=CARTESIAN_POINT('Ctrl Pts',(-9.35355679167832,-16.0378273519455,
-331.354092555978)) ;
#44344=CARTESIAN_POINT('Ctrl Pts',(-9.57466023518528,-15.9075925907088,
-331.357346113269)) ;
#44345=CARTESIAN_POINT('Ctrl Pts',(-9.72538006394519,-15.8158971751446,
-331.359557121069)) ;
#44346=CARTESIAN_POINT('Ctrl Pts',(-10.1098017594987,-15.5744482735364,
-331.365204760896)) ;
#44347=CARTESIAN_POINT('Ctrl Pts',(-10.3414937842337,-15.421577005722,-331.368617015808)) ;
#44348=CARTESIAN_POINT('Ctrl Pts',(-10.7804742594848,-15.117593091634,-331.375164255486)) ;
#44349=CARTESIAN_POINT('Ctrl Pts',(-10.9882302316875,-14.9672656998948,
-331.378299816587)) ;
#44350=CARTESIAN_POINT('Ctrl Pts',(-11.5704488233802,-14.5273278901423,
-331.387255314615)) ;
#44351=CARTESIAN_POINT('Ctrl Pts',(-11.9370405010022,-14.2276352316939,
-331.393102684929)) ;
#44352=CARTESIAN_POINT('Ctrl Pts',(-12.4053085549168,-13.8139699922844,
-331.400971149525)) ;
#44353=CARTESIAN_POINT('Ctrl Pts',(-12.5176076779195,-13.712291756874,-331.402889671316)) ;
#44354=CARTESIAN_POINT('Ctrl Pts',(-12.7206782089786,-13.5238532698427,
-331.406419877833)) ;
#44355=CARTESIAN_POINT('Ctrl Pts',(-12.8118379976024,-13.4375246392885,
-331.40802774849)) ;
#44356=CARTESIAN_POINT('Ctrl Pts',(-12.9985854536365,-13.2570462143434,
-331.411370867122)) ;
#44357=CARTESIAN_POINT('Ctrl Pts',(-13.0940423455259,-13.1627714830096,
-331.413107192211)) ;
#44358=CARTESIAN_POINT('Ctrl Pts',(-13.3458267635657,-12.9086556634847,
-331.417761492747)) ;
#44359=CARTESIAN_POINT('Ctrl Pts',(-13.500302809021,-12.747011682148,-331.420695569395)) ;
#44360=CARTESIAN_POINT('Ctrl Pts',(-13.7561735302441,-12.469398426364,-331.42568731787)) ;
#44361=CARTESIAN_POINT('Ctrl Pts',(-13.8591128683516,-12.3548855816682,
-331.427733222945)) ;
#44362=CARTESIAN_POINT('Ctrl Pts',(-14.3167461561979,-11.8328831840082,
-331.436993826502)) ;
#44363=CARTESIAN_POINT('Ctrl Pts',(-14.6549763772027,-11.4113106375806,
-331.444303884208)) ;
#44364=CARTESIAN_POINT('Ctrl Pts',(-15.1700617287894,-10.7085637566994,
-331.456006102515)) ;
#44365=CARTESIAN_POINT('Ctrl Pts',(-15.3586058313691,-10.4363469801212,
-331.460427998719)) ;
#44366=CARTESIAN_POINT('Ctrl Pts',(-15.5933070923309,-10.0773431855292,
-331.466052962013)) ;
#44367=CARTESIAN_POINT('Ctrl Pts',(-15.6461958840107,-9.99503007270438,
-331.467328887012)) ;
#44368=CARTESIAN_POINT('Ctrl Pts',(-15.7338771291969,-9.85616647304519,
-331.469455822043)) ;
#44369=CARTESIAN_POINT('Ctrl Pts',(-15.7690212956443,-9.7998405330711,-331.4703114943)) ;
#44370=CARTESIAN_POINT('Ctrl Pts',(-15.8461503563063,-9.67473572291543,
-331.472195910214)) ;
#44371=CARTESIAN_POINT('Ctrl Pts',(-15.8879910467882,-9.60586971305204,
-331.473222776428)) ;
#44372=CARTESIAN_POINT('Ctrl Pts',(-16.0212528030751,-9.38328013874559,
-331.476511670561)) ;
#44373=CARTESIAN_POINT('Ctrl Pts',(-16.1109014472047,-9.22850704607624,
-331.478752643936)) ;
#44374=CARTESIAN_POINT('Ctrl Pts',(-16.3369549921495,-8.82490294762817,
-331.484506056995)) ;
#44375=CARTESIAN_POINT('Ctrl Pts',(-16.4699168260395,-8.57419679058869,
-331.487993020809)) ;
#44376=CARTESIAN_POINT('Ctrl Pts',(-16.9147867202385,-7.68680969129279,
-331.500162302095)) ;
#44377=CARTESIAN_POINT('Ctrl Pts',(-17.1959353729,-7.03540043254521,-331.508812879716)) ;
#44378=CARTESIAN_POINT('Ctrl Pts',(-17.4925489170177,-6.22329999630359,
-331.519691540344)) ;
#44379=CARTESIAN_POINT('Ctrl Pts',(-17.5441120608831,-6.07641854716277,
-331.521661534681)) ;
#44380=CARTESIAN_POINT('Ctrl Pts',(-17.6342000371274,-5.80908562643832,
-331.525254342114)) ;
#44381=CARTESIAN_POINT('Ctrl Pts',(-17.673353004309,-5.68885579852728,-331.526872797266)) ;
#44382=CARTESIAN_POINT('Ctrl Pts',(-17.7510257764981,-5.44179659955389,
-331.530204930518)) ;
#44383=CARTESIAN_POINT('Ctrl Pts',(-17.7894216919508,-5.31493576185626,
-331.531919343106)) ;
#44384=CARTESIAN_POINT('Ctrl Pts',(-17.8863554478203,-4.9818413814567,-331.53643017183)) ;
#44385=CARTESIAN_POINT('Ctrl Pts',(-17.9426854311605,-4.77498628527236,
-331.539240904705)) ;
#44386=CARTESIAN_POINT('Ctrl Pts',(-18.1639374705924,-3.9032221108315,-331.551119309564)) ;
#44387=CARTESIAN_POINT('Ctrl Pts',(-18.2955763650669,-3.23042511831326,
-331.560387604609)) ;
#44388=CARTESIAN_POINT('Ctrl Pts',(-18.4381439038572,-2.20304207254931,
-331.574329804321)) ;
#44389=CARTESIAN_POINT('Ctrl Pts',(-18.4766175319275,-1.85287626235518,
-331.57904062491)) ;
#44390=CARTESIAN_POINT('Ctrl Pts',(-18.5132166667941,-1.40191192968094,
-331.584977635847)) ;
#44391=CARTESIAN_POINT('Ctrl Pts',(-18.520516264185,-1.30193155020809,-331.586285614674)) ;
#44392=CARTESIAN_POINT('Ctrl Pts',(-18.5313229321195,-1.13534887234126,
-331.588448405205)) ;
#44393=CARTESIAN_POINT('Ctrl Pts',(-18.5352814976047,-1.06877804941513,
-331.58930826546)) ;
#44394=CARTESIAN_POINT('Ctrl Pts',(-18.5431600794371,-0.923036708281147,
-331.591180345956)) ;
#44395=CARTESIAN_POINT('Ctrl Pts',(-18.5469319141503,-0.843859639608341,
-331.592190921782)) ;
#44396=CARTESIAN_POINT('Ctrl Pts',(-18.55722350396,-0.594192050500668,-331.595360264501)) ;
#44397=CARTESIAN_POINT('Ctrl Pts',(-18.5619002946768,-0.423634270060247,
-331.597500026508)) ;
#44398=CARTESIAN_POINT('Ctrl Pts',(-18.5678128423706,0.0101452110234948,
-331.602901064301)) ;
#44399=CARTESIAN_POINT('Ctrl Pts',(-18.5658030798211,0.273373418284622,
-331.60614043762)) ;
#44400=CARTESIAN_POINT('Ctrl Pts',(-18.5362661362121,1.2951500308187,-331.618681193349)) ;
#44401=CARTESIAN_POINT('Ctrl Pts',(-18.4678316157956,2.05177281078287,-331.627926452439)) ;
#44402=CARTESIAN_POINT('Ctrl Pts',(-18.3285550607503,2.96401847065086,-331.639553227547)) ;
#44403=CARTESIAN_POINT('Ctrl Pts',(-18.3016883016166,3.12562654674809,-331.641629943042)) ;
#44404=CARTESIAN_POINT('Ctrl Pts',(-18.2505600686712,3.40986463996013,-331.645315617827)) ;
#44405=CARTESIAN_POINT('Ctrl Pts',(-18.2271923110643,3.53264491375653,-331.64691863487)) ;
#44406=CARTESIAN_POINT('Ctrl Pts',(-18.1750547849223,3.79228681864865,-331.650332617048)) ;
#44407=CARTESIAN_POINT('Ctrl Pts',(-18.14597474636,3.92907828651783,-331.652145540222)) ;
#44408=CARTESIAN_POINT('Ctrl Pts',(-18.059146120464,4.31597295924445,-331.65731397514)) ;
#44409=CARTESIAN_POINT('Ctrl Pts',(-17.9977526962845,4.56522492894707,-331.660692662125)) ;
#44410=CARTESIAN_POINT('Ctrl Pts',(-17.8382533704448,5.15943702951864,-331.668856110161)) ;
#44411=CARTESIAN_POINT('Ctrl Pts',(-17.7352822109154,5.5029844533492,-331.673665711063)) ;
#44412=CARTESIAN_POINT('Ctrl Pts',(-17.4371298653266,6.40215753372959,-331.686416412542)) ;
#44413=CARTESIAN_POINT('Ctrl Pts',(-17.2253557058779,6.95185158931128,-331.694385868993)) ;
#44414=CARTESIAN_POINT('Ctrl Pts',(-16.9441938947519,7.58949843422687,-331.703546542479)) ;
#44415=CARTESIAN_POINT('Ctrl Pts',(-16.8997012346149,7.68806161913078,-331.704959715081)) ;
#44416=CARTESIAN_POINT('Ctrl Pts',(-16.8261613680886,7.84724861457569,-331.707234191653)) ;
#44417=CARTESIAN_POINT('Ctrl Pts',(-16.7976415635973,7.90811324806361,-331.708101911654)) ;
#44418=CARTESIAN_POINT('Ctrl Pts',(-16.7363726172915,8.03704149195143,-331.709934970161)) ;
#44419=CARTESIAN_POINT('Ctrl Pts',(-16.7035374133237,8.1050627530071,-331.710899249294)) ;
#44420=CARTESIAN_POINT('Ctrl Pts',(-16.6047632936052,8.30653306224311,-331.71374945145)) ;
#44421=CARTESIAN_POINT('Ctrl Pts',(-16.5376335534004,8.43939169173527,-331.715621338628)) ;
#44422=CARTESIAN_POINT('Ctrl Pts',(-16.370215984556,8.76106331629915,-331.720149750636)) ;
#44423=CARTESIAN_POINT('Ctrl Pts',(-16.2682504626407,8.94897921107539,-331.722792116712)) ;
#44424=CARTESIAN_POINT('Ctrl Pts',(-15.7588434336498,9.85029222155326,-331.735530399111)) ;
#44425=CARTESIAN_POINT('Ctrl Pts',(-15.3076006685487,10.5378730508359,-331.745490731296)) ;
#44426=CARTESIAN_POINT('Ctrl Pts',(-14.7075415985295,11.3319422662572,-331.758011912124)) ;
#44427=CARTESIAN_POINT('Ctrl Pts',(-14.6008356007635,11.46910175331,-331.760212097871)) ;
#44428=CARTESIAN_POINT('Ctrl Pts',(-14.413549669923,11.7029879271909,-331.764032896281)) ;
#44429=CARTESIAN_POINT('Ctrl Pts',(-14.3338823905267,11.8004303342313,-331.765645936428)) ;
#44430=CARTESIAN_POINT('Ctrl Pts',(-14.1655944190609,12.0020472255589,-331.769029003547)) ;
#44431=CARTESIAN_POINT('Ctrl Pts',(-14.0768009770804,12.1060677775006,-331.770800431064)) ;
#44432=CARTESIAN_POINT('Ctrl Pts',(-13.8300367499831,12.3887633853556,-331.775686959527)) ;
#44433=CARTESIAN_POINT('Ctrl Pts',(-13.6697600891816,12.5653903039335,-331.778821220587)) ;
#44434=CARTESIAN_POINT('Ctrl Pts',(-13.2872091435448,12.9709817724761,-331.786205178204)) ;
#44435=CARTESIAN_POINT('Ctrl Pts',(-13.0623464112431,13.1974012823016,-331.790473241135)) ;
#44436=CARTESIAN_POINT('Ctrl Pts',(-12.5310896485368,13.7054504773766,-331.800352556521)) ;
#44437=CARTESIAN_POINT('Ctrl Pts',(-12.220838141711,13.9827999893821,-331.805976160708)) ;
#44438=CARTESIAN_POINT('Ctrl Pts',(-11.7253475713879,14.3966461032938,-331.814622879287)) ;
#44439=CARTESIAN_POINT('Ctrl Pts',(-11.5464485919751,14.5405199324681,-331.817680380057)) ;
#44440=CARTESIAN_POINT('Ctrl Pts',(-11.2740033495633,14.7514260114405,-331.822215745074)) ;
#44441=CARTESIAN_POINT('Ctrl Pts',(-11.1824270203272,14.8209664628872,-331.823720236991)) ;
#44442=CARTESIAN_POINT('Ctrl Pts',(-11.040232292008,14.9268768961609,-331.826021999575)) ;
#44443=CARTESIAN_POINT('Ctrl Pts',(-10.9900669219232,14.963850172938,-331.826827548958)) ;
#44444=CARTESIAN_POINT('Ctrl Pts',(-10.8823156573827,15.0424317369025,-331.82854307448)) ;
#44445=CARTESIAN_POINT('Ctrl Pts',(-10.8246751445475,15.0839634929808,-331.829451860772)) ;
#44446=CARTESIAN_POINT('Ctrl Pts',(-10.6648438465556,15.197738874673,-331.83194929016)) ;
#44447=CARTESIAN_POINT('Ctrl Pts',(-10.5621587225438,15.2692817241382,-331.833528574788)) ;
#44448=CARTESIAN_POINT('Ctrl Pts',(-10.3211816787165,15.4335813705844,-331.837185126018)) ;
#44449=CARTESIAN_POINT('Ctrl Pts',(-10.1823495050015,15.5255268461562,-331.839254326873)) ;
#44450=CARTESIAN_POINT('Ctrl Pts',(-9.63513571133012,15.8774369437671,-331.847296862428)) ;
#44451=CARTESIAN_POINT('Ctrl Pts',(-9.21788657678393,16.1232568767848,-331.853191078634)) ;
#44452=CARTESIAN_POINT('Ctrl Pts',(-8.42548722669793,16.5492706422417,-331.8642430431)) ;
#44453=CARTESIAN_POINT('Ctrl Pts',(-8.05296334221619,16.7337077234566,-331.869382937618)) ;
#44454=CARTESIAN_POINT('Ctrl Pts',(-7.51311146723126,16.9787836771746,-331.876836955329)) ;
#44455=CARTESIAN_POINT('Ctrl Pts',(-7.35061568420548,17.0497621098074,-331.879080823854)) ;
#44456=CARTESIAN_POINT('Ctrl Pts',(-7.07061997982843,17.1673177713276,-331.882951686474)) ;
#44457=CARTESIAN_POINT('Ctrl Pts',(-6.95361536788679,17.2150428295426,-331.884570531106)) ;
#44458=CARTESIAN_POINT('Ctrl Pts',(-6.71017734321866,17.3114520607135,-331.887942293788)) ;
#44459=CARTESIAN_POINT('Ctrl Pts',(-6.58367982288382,17.3599542727317,-331.889696364602)) ;
#44460=CARTESIAN_POINT('Ctrl Pts',(-6.24001542907438,17.4874269292189,-331.894467540683)) ;
#44461=CARTESIAN_POINT('Ctrl Pts',(-6.0218869607842,17.5637345198057,-331.897502259535)) ;
#44462=CARTESIAN_POINT('Ctrl Pts',(-5.64870356937853,17.686515319265,-331.902701027425)) ;
#44463=CARTESIAN_POINT('Ctrl Pts',(-5.49436144900012,17.7350688844233,-331.904853028325)) ;
#44464=CARTESIAN_POINT('Ctrl Pts',(-4.76454484726649,17.9542160009468,-331.91502880749)) ;
#44465=CARTESIAN_POINT('Ctrl Pts',(-4.18165407044763,18.0988542924827,-331.923168279854)) ;
#44466=CARTESIAN_POINT('Ctrl Pts',(-3.45341113900785,18.242495213728,-331.933103108547)) ;
#44467=CARTESIAN_POINT('Ctrl Pts',(-3.31372652463599,18.2683851696051,-331.934997497831)) ;
#44468=CARTESIAN_POINT('Ctrl Pts',(-3.03179040997574,18.3173007821852,-331.938790579861)) ;
#44469=CARTESIAN_POINT('Ctrl Pts',(-2.88954021443678,18.3402785826744,-331.940688819553)) ;
#44470=CARTESIAN_POINT('Ctrl Pts',(-2.66534431492158,18.3738200199791,-331.943648910296)) ;
#44471=CARTESIAN_POINT('Ctrl Pts',(-2.58357105750912,18.3854965410316,-331.944721963404)) ;
#44472=CARTESIAN_POINT('Ctrl Pts',(-2.43626337686835,18.4055286341393,-331.946641408023)) ;
#44473=CARTESIAN_POINT('Ctrl Pts',(-2.37075732425834,18.4140808419076,-331.94748998443)) ;
#44474=CARTESIAN_POINT('Ctrl Pts',(-2.21132165961733,18.4340312566281,-331.949543845586)) ;
#44475=CARTESIAN_POINT('Ctrl Pts',(-2.11734790080118,18.4450613920446,-331.950744928739)) ;
#44476=CARTESIAN_POINT('Ctrl Pts',(-1.72167342631557,18.4884398566989,-331.955769106123)) ;
#44477=CARTESIAN_POINT('Ctrl Pts',(-1.41928694166473,18.5141079477051,-331.959528927246)) ;
#44478=CARTESIAN_POINT('Ctrl Pts',(-0.280721623934055,18.5826962338751,
-331.97356903952)) ;
#44479=CARTESIAN_POINT('Ctrl Pts',(0.557410764232457,18.576455562283,-331.983713292041)) ;
#44480=CARTESIAN_POINT('Ctrl Pts',(1.5460708546203,18.5021068267284,-331.99619191967)) ;
#44481=CARTESIAN_POINT('Ctrl Pts',(1.69973510802066,18.4886233285991,-331.998144487635)) ;
#44482=CARTESIAN_POINT('Ctrl Pts',(1.97871519221223,18.4606363602097,-332.001716011425)) ;
#44483=CARTESIAN_POINT('Ctrl Pts',(2.10408538715813,18.4467675560337,-332.003330794352)) ;
#44484=CARTESIAN_POINT('Ctrl Pts',(2.36139797415323,18.4156456030462,-332.00666613251)) ;
#44485=CARTESIAN_POINT('Ctrl Pts',(2.49331584615126,18.3982493568772,-332.008387534452)) ;
#44486=CARTESIAN_POINT('Ctrl Pts',(2.84015425265685,18.3487123095595,-332.012944074571)) ;
#44487=CARTESIAN_POINT('Ctrl Pts',(3.05471698134277,18.3142137014464,-332.015794089639)) ;
#44488=CARTESIAN_POINT('Ctrl Pts',(3.41391851047208,18.2499711086659,-332.020615073385)) ;
#44489=CARTESIAN_POINT('Ctrl Pts',(3.55889755013297,18.2222537909799,-332.022574541392)) ;
#44490=CARTESIAN_POINT('Ctrl Pts',(4.19104212886648,18.0935674224194,-332.031172393643)) ;
#44491=CARTESIAN_POINT('Ctrl Pts',(4.67436711268179,17.9747686139255,-332.037892972326)) ;
#44492=CARTESIAN_POINT('Ctrl Pts',(5.22665637259435,17.8152335712315,-332.045626956807)) ;
#44493=CARTESIAN_POINT('Ctrl Pts',(5.30084326235868,17.7933005580051,-332.046666834219)) ;
#44494=CARTESIAN_POINT('Ctrl Pts',(5.67741552285269,17.6794045647664,-332.051947576863)) ;
#44495=CARTESIAN_POINT('Ctrl Pts',(5.9775549568405,17.5801942605611,-332.056165041427)) ;
#44496=CARTESIAN_POINT('Ctrl Pts',(6.36632838708065,17.4405784202165,-332.061581276427)) ;
#44497=CARTESIAN_POINT('Ctrl Pts',(6.45738288298993,17.4070709513657,-332.062846334359)) ;
#44498=CARTESIAN_POINT('Ctrl Pts',(6.61020879545238,17.3494678478016,-332.064961230441)) ;
#44499=CARTESIAN_POINT('Ctrl Pts',(6.67212127391179,17.3257522971288,-332.065815600062)) ;
#44500=CARTESIAN_POINT('Ctrl Pts',(6.80944650943599,17.2723046659681,-332.067704770073)) ;
#44501=CARTESIAN_POINT('Ctrl Pts',(6.88479410764785,17.242409354803,-332.06873760878)) ;
#44502=CARTESIAN_POINT('Ctrl Pts',(7.12863509967626,17.143808528611,-332.072071437282)) ;
#44503=CARTESIAN_POINT('Ctrl Pts',(7.29631500291615,17.0731191302671,-332.07435057508)) ;
#44504=CARTESIAN_POINT('Ctrl Pts',(7.73010947118155,16.8826849081625,-332.080240549846)) ;
#44505=CARTESIAN_POINT('Ctrl Pts',(7.99448821531071,16.7591109774453,-332.083824459769)) ;
#44506=CARTESIAN_POINT('Ctrl Pts',(8.87348924595585,16.3227203352077,-332.095852635572)) ;
#44507=CARTESIAN_POINT('Ctrl Pts',(9.47357100943901,15.981910468644,-332.104272765041)) ;
#44508=CARTESIAN_POINT('Ctrl Pts',(10.2009303023555,15.5134250575098,-332.115153500138)) ;
#44509=CARTESIAN_POINT('Ctrl Pts',(10.3472047410798,15.4162475966418,-332.117376298661)) ;
#44510=CARTESIAN_POINT('Ctrl Pts',(10.5961247282556,15.2457385971344,-332.121222959738)) ;
#44511=CARTESIAN_POINT('Ctrl Pts',(10.6994420508467,15.1734091217618,-332.122838952109)) ;
#44512=CARTESIAN_POINT('Ctrl Pts',(10.9126864268451,15.0208618490027,-332.126215857696)) ;
#44513=CARTESIAN_POINT('Ctrl Pts',(11.0224846925921,14.9404767953348,-332.127978040791)) ;
#44514=CARTESIAN_POINT('Ctrl Pts',(11.3190867362795,14.7182803635872,-332.132802981054)) ;
#44515=CARTESIAN_POINT('Ctrl Pts',(11.5041027549559,14.574125046996,-332.135884065854)) ;
#44516=CARTESIAN_POINT('Ctrl Pts',(11.9279271975545,14.2308016947911,-332.143104590161)) ;
#44517=CARTESIAN_POINT('Ctrl Pts',(12.1645621819109,14.0290623518186,-332.147261178875)) ;
#44518=CARTESIAN_POINT('Ctrl Pts',(12.8918232658396,13.3768062620202,-332.160385108515)) ;
#44519=CARTESIAN_POINT('Ctrl Pts',(13.3633411116242,12.9057803530218,-332.169430712286)) ;
#44520=CARTESIAN_POINT('Ctrl Pts',(13.8835154218664,12.3270062604297,-332.17966858666)) ;
#44521=CARTESIAN_POINT('Ctrl Pts',(13.9577448622368,12.2428935400364,-332.181135664912)) ;
#44522=CARTESIAN_POINT('Ctrl Pts',(14.0717118413588,12.1113686636672,-332.183394194914)) ;
#44523=CARTESIAN_POINT('Ctrl Pts',(14.1119823935993,12.0644219916771,-332.184193451988)) ;
#44524=CARTESIAN_POINT('Ctrl Pts',(14.1984744379758,11.9625655436357,-332.185911817685)) ;
#44525=CARTESIAN_POINT('Ctrl Pts',(14.2446136457105,11.9075871969891,-332.186829605341)) ;
#44526=CARTESIAN_POINT('Ctrl Pts',(14.3726990777383,11.7531539064573,-332.189382675768)) ;
#44527=CARTESIAN_POINT('Ctrl Pts',(14.4539304202055,11.6531112162949,-332.191007916671)) ;
#44528=CARTESIAN_POINT('Ctrl Pts',(14.6420919725536,11.4163810613987,-332.194796582731)) ;
#44529=CARTESIAN_POINT('Ctrl Pts',(14.7481603794183,11.2790238687871,-332.196951126732)) ;
#44530=CARTESIAN_POINT('Ctrl Pts',(15.1719887096987,10.7139693471667,-332.205675302701)) ;
#44531=CARTESIAN_POINT('Ctrl Pts',(15.4731939097454,10.2741740416133,-332.21215398903)) ;
#44532=CARTESIAN_POINT('Ctrl Pts',(15.8754760600177,9.6288920249461,-332.221516070776)) ;
#44533=CARTESIAN_POINT('Ctrl Pts',(15.9923231607515,9.43355190260966,-332.224331099906)) ;
#44534=CARTESIAN_POINT('Ctrl Pts',(16.2258969649451,9.0262556394395,-332.230182629515)) ;
#44535=CARTESIAN_POINT('Ctrl Pts',(16.3421313944118,8.81406627810662,-332.233221411081)) ;
#44536=CARTESIAN_POINT('Ctrl Pts',(16.5178063467136,8.47793832322024,-332.238032400112)) ;
#44537=CARTESIAN_POINT('Ctrl Pts',(16.580073918033,8.35550797528294,-332.239784105139)) ;
#44538=CARTESIAN_POINT('Ctrl Pts',(16.6966971540801,8.11976565726892,-332.24315734619)) ;
#44539=CARTESIAN_POINT('Ctrl Pts',(16.7512721435412,8.00657053325846,-332.244777180012)) ;
#44540=CARTESIAN_POINT('Ctrl Pts',(16.87793405211,7.73689355733387,-332.248637180834)) ;
#44541=CARTESIAN_POINT('Ctrl Pts',(16.9490002600113,7.57994523975932,-332.250884400886)) ;
#44542=CARTESIAN_POINT('Ctrl Pts',(17.24932435737,6.89133627237522,-332.260745764029)) ;
#44543=CARTESIAN_POINT('Ctrl Pts',(17.4558253886552,6.35010725633239,-332.268512042367)) ;
#44544=CARTESIAN_POINT('Ctrl Pts',(17.8004348630631,5.30223669175835,-332.283369264019)) ;
#44545=CARTESIAN_POINT('Ctrl Pts',(17.9430154746527,4.79764441870485,-332.290445425046)) ;
#44546=CARTESIAN_POINT('Ctrl Pts',(18.089801287868,4.17923622088749,-332.29880618908)) ;
#44547=CARTESIAN_POINT('Ctrl Pts',(18.11456839653,4.07054515869485,-332.300263857364)) ;
#44548=CARTESIAN_POINT('Ctrl Pts',(18.1515286734727,3.90132255242415,-332.302511540022)) ;
#44549=CARTESIAN_POINT('Ctrl Pts',(18.1644012889704,3.84094215962314,-332.303309241649)) ;
#44550=CARTESIAN_POINT('Ctrl Pts',(18.1916272130505,3.71003750282837,-332.305028508422)) ;
#44551=CARTESIAN_POINT('Ctrl Pts',(18.2058721028726,3.63949171214811,-332.305948717724)) ;
#44552=CARTESIAN_POINT('Ctrl Pts',(18.2446711724638,3.44141537883529,-332.308516838372)) ;
#44553=CARTESIAN_POINT('Ctrl Pts',(18.2682979473849,3.31370731835557,-332.310154519616)) ;
#44554=CARTESIAN_POINT('Ctrl Pts',(18.3206904642593,3.01290338390637,-332.313979237911)) ;
#44555=CARTESIAN_POINT('Ctrl Pts',(18.3483461492828,2.83962666834625,-332.316157164572)) ;
#44556=CARTESIAN_POINT('Ctrl Pts',(18.4521236564401,2.12440841226223,-332.325081521149)) ;
#44557=CARTESIAN_POINT('Ctrl Pts',(18.5067223202752,1.57962305695096,-332.331733489889)) ;
#44558=CARTESIAN_POINT('Ctrl Pts',(18.5408754758118,0.966877152202078,-332.339294922937)) ;
#44559=CARTESIAN_POINT('Ctrl Pts',(18.544217236243,0.900512036507376,-332.340114796803)) ;
#44560=CARTESIAN_POINT('Ctrl Pts',(18.554037632943,0.68215183631762,-332.342816323201)) ;
#44561=CARTESIAN_POINT('Ctrl Pts',(18.5590043576457,0.530095088599722,-332.344703822096)) ;
#44562=CARTESIAN_POINT('Ctrl Pts',(18.5669195460512,0.141405603914571,-332.349551882388)) ;
#44563=CARTESIAN_POINT('Ctrl Pts',(18.5672136693237,-0.0952535122605108,
-332.352525865488)) ;
#44564=CARTESIAN_POINT('Ctrl Pts',(18.5605451549998,-0.468272513056562,
-332.357259767486)) ;
#44565=CARTESIAN_POINT('Ctrl Pts',(18.5566026237942,-0.604660726114443,
-332.359000340067)) ;
#44566=CARTESIAN_POINT('Ctrl Pts',(18.5491863659681,-0.790330730519442,
-332.361384090202)) ;
#44567=CARTESIAN_POINT('Ctrl Pts',(18.5470188521273,-0.839660132558339,
-332.362018778973)) ;
#44568=CARTESIAN_POINT('Ctrl Pts',(18.544654593742,-0.888979978009869,-332.362654732516)) ;
#44569=CARTESIAN_POINT('Origin',(0.,0.,-315.477129595899)) ;
#44570=CARTESIAN_POINT('',(18.5446545951453,-0.888979948736908,-334.159397110263)) ;
#44571=CARTESIAN_POINT('',(18.5446545936727,-0.888979979456325,-333.864249094225)) ;
#44572=CARTESIAN_POINT('',(18.544654593745,-0.888979977948782,-315.477129595899)) ;
#44573=CARTESIAN_POINT('Ctrl Pts',(18.5446545951453,-0.888979948736927,
-334.159397110264)) ;
#44574=CARTESIAN_POINT('Ctrl Pts',(18.5692830990318,-0.37521459506579,-334.153090696754)) ;
#44575=CARTESIAN_POINT('Ctrl Pts',(18.5725507246078,0.139351443153365,-334.14674863002)) ;
#44576=CARTESIAN_POINT('Ctrl Pts',(18.5498213412484,0.784805709244924,-334.138615311045)) ;
#44577=CARTESIAN_POINT('Ctrl Pts',(18.5437973724742,0.916171788360239,-334.136951158575)) ;
#44578=CARTESIAN_POINT('Ctrl Pts',(18.5298187220353,1.16354438066611,-334.133798953664)) ;
#44579=CARTESIAN_POINT('Ctrl Pts',(18.5221688495189,1.27956182573606,-334.132312908977)) ;
#44580=CARTESIAN_POINT('Ctrl Pts',(18.5039344669633,1.52146869963332,-334.129197490693)) ;
#44581=CARTESIAN_POINT('Ctrl Pts',(18.4931537900458,1.64733742915553,-334.127566917763)) ;
#44582=CARTESIAN_POINT('Ctrl Pts',(18.4633853879098,1.95761704116994,-334.123523240871)) ;
#44583=CARTESIAN_POINT('Ctrl Pts',(18.4429186453917,2.14187211037741,-334.121100800655)) ;
#44584=CARTESIAN_POINT('Ctrl Pts',(18.3594588929034,2.802853369882,-334.112336877021)) ;
#44585=CARTESIAN_POINT('Ctrl Pts',(18.2807109584137,3.27739567166514,-334.105901468451)) ;
#44586=CARTESIAN_POINT('Ctrl Pts',(18.0625214680297,4.33585721756017,-334.091357686981)) ;
#44587=CARTESIAN_POINT('Ctrl Pts',(17.9130095474824,4.91715660980554,-334.083234044209)) ;
#44588=CARTESIAN_POINT('Ctrl Pts',(17.7080335944691,5.57931436451973,-334.074123382003)) ;
#44589=CARTESIAN_POINT('Ctrl Pts',(17.6797749559515,5.66822371659494,-334.072903407742)) ;
#44590=CARTESIAN_POINT('Ctrl Pts',(17.6341251077477,5.80818727544336,-334.070990223011)) ;
#44591=CARTESIAN_POINT('Ctrl Pts',(17.6171795104917,5.85938510809401,-334.070291949485)) ;
#44592=CARTESIAN_POINT('Ctrl Pts',(17.5786718350788,5.97405130371369,-334.068732139851)) ;
#44593=CARTESIAN_POINT('Ctrl Pts',(17.5569886692368,6.03747805985553,-334.067872322134)) ;
#44594=CARTESIAN_POINT('Ctrl Pts',(17.5068765580993,6.18151097362589,-334.065925587167)) ;
#44595=CARTESIAN_POINT('Ctrl Pts',(17.4782334987114,6.26204108329537,-334.064841209301)) ;
#44596=CARTESIAN_POINT('Ctrl Pts',(17.3497200452353,6.61560537919624,-334.060092859409)) ;
#44597=CARTESIAN_POINT('Ctrl Pts',(17.244000317387,6.88647035464091,-334.05648769146)) ;
#44598=CARTESIAN_POINT('Ctrl Pts',(17.0806633808841,7.27757918171694,-334.051267392867)) ;
#44599=CARTESIAN_POINT('Ctrl Pts',(17.0280434709812,7.39986188069287,-334.049633203596)) ;
#44600=CARTESIAN_POINT('Ctrl Pts',(16.7795470644528,7.96065000708573,-334.042113015239)) ;
#44601=CARTESIAN_POINT('Ctrl Pts',(16.5680172306455,8.39201722617697,-334.036250076017)) ;
#44602=CARTESIAN_POINT('Ctrl Pts',(16.2388160084323,9.00226497050727,-334.027658724401)) ;
#44603=CARTESIAN_POINT('Ctrl Pts',(16.1344088880154,9.18807757900674,-334.025002270858)) ;
#44604=CARTESIAN_POINT('Ctrl Pts',(15.9412332871798,9.51842060476988,-334.020194004397)) ;
#44605=CARTESIAN_POINT('Ctrl Pts',(15.8536394513711,9.66361037874798,-334.018050305824)) ;
#44606=CARTESIAN_POINT('Ctrl Pts',(15.7070164604246,9.89928268928725,-334.01451689974)) ;
#44607=CARTESIAN_POINT('Ctrl Pts',(15.6491646340442,9.99048597786419,-334.013136086918)) ;
#44608=CARTESIAN_POINT('Ctrl Pts',(15.5219760540935,10.1871828227723,-334.010128137392)) ;
#44609=CARTESIAN_POINT('Ctrl Pts',(15.4523524836459,10.2924844986942,-334.008498839566)) ;
#44610=CARTESIAN_POINT('Ctrl Pts',(15.2950159774999,10.5252517325553,-334.004854276294)) ;
#44611=CARTESIAN_POINT('Ctrl Pts',(15.2067725995651,10.6523473842412,-334.002835003797)) ;
#44612=CARTESIAN_POINT('Ctrl Pts',(14.7012089519089,11.361416823867,-333.991404950764)) ;
#44613=CARTESIAN_POINT('Ctrl Pts',(14.2520796862702,11.9199644773943,-333.981742644226)) ;
#44614=CARTESIAN_POINT('Ctrl Pts',(13.5835439141688,12.6594093651944,-333.968325100605)) ;
#44615=CARTESIAN_POINT('Ctrl Pts',(13.3905720599802,12.8633545765292,-333.964555456458)) ;
#44616=CARTESIAN_POINT('Ctrl Pts',(13.0680413219491,13.1891001504586,-333.95846528223)) ;
#44617=CARTESIAN_POINT('Ctrl Pts',(12.9412266317032,13.3135540044423,-333.956121271594)) ;
#44618=CARTESIAN_POINT('Ctrl Pts',(12.7544635830763,13.4916500616955,-333.952754032292)) ;
#44619=CARTESIAN_POINT('Ctrl Pts',(12.6959223057353,13.5467530984379,-333.951710373808)) ;
#44620=CARTESIAN_POINT('Ctrl Pts',(12.5883596461338,13.6466887370341,-333.94981579123)) ;
#44621=CARTESIAN_POINT('Ctrl Pts',(12.5394521574716,13.6916416711179,-333.948963062504)) ;
#44622=CARTESIAN_POINT('Ctrl Pts',(12.4176786583323,13.8023690588317,-333.946860518498)) ;
#44623=CARTESIAN_POINT('Ctrl Pts',(12.3445302483214,13.8678299631384,-333.945615476673)) ;
#44624=CARTESIAN_POINT('Ctrl Pts',(12.0012220180292,14.1701896620871,-333.939846560031)) ;
#44625=CARTESIAN_POINT('Ctrl Pts',(11.7247399425815,14.3997944263043,-333.935411730716)) ;
#44626=CARTESIAN_POINT('Ctrl Pts',(10.9086096140476,15.0384529981051,-333.922687356617)) ;
#44627=CARTESIAN_POINT('Ctrl Pts',(10.3530271884397,15.4262004709477,-333.914449845671)) ;
#44628=CARTESIAN_POINT('Ctrl Pts',(9.59285037226465,15.8971352391819,-333.903272452604)) ;
#44629=CARTESIAN_POINT('Ctrl Pts',(9.40619431640646,16.008285208616,-333.900536990305)) ;
#44630=CARTESIAN_POINT('Ctrl Pts',(9.1021433642462,16.1821873071397,-333.8960870842)) ;
#44631=CARTESIAN_POINT('Ctrl Pts',(8.98594903340544,16.2469972540788,-333.894387970544)) ;
#44632=CARTESIAN_POINT('Ctrl Pts',(8.75825228644693,16.3708102256992,-333.891059844996)) ;
#44633=CARTESIAN_POINT('Ctrl Pts',(8.64682519713828,16.4299368384491,-333.889431860268)) ;
#44634=CARTESIAN_POINT('Ctrl Pts',(8.39778883853749,16.5588479544717,-333.885794395821)) ;
#44635=CARTESIAN_POINT('Ctrl Pts',(8.25989474318021,16.6280618741974,-333.883780964798)) ;
#44636=CARTESIAN_POINT('Ctrl Pts',(7.47187998009878,17.0113729819262,-333.872280354112)) ;
#44637=CARTESIAN_POINT('Ctrl Pts',(6.80473730189455,17.2890526868623,-333.862536633007)) ;
#44638=CARTESIAN_POINT('Ctrl Pts',(5.86093735137052,17.6187697192086,-333.849081427472)) ;
#44639=CARTESIAN_POINT('Ctrl Pts',(5.5967244496135,17.704471435148,-333.845352811526)) ;
#44640=CARTESIAN_POINT('Ctrl Pts',(5.16163428212565,17.8348865430217,-333.839319127925)) ;
#44641=CARTESIAN_POINT('Ctrl Pts',(4.99186582908364,17.8831463170608,-333.836991066754)) ;
#44642=CARTESIAN_POINT('Ctrl Pts',(4.74397920997699,17.9498076288454,-333.833641974073)) ;
#44643=CARTESIAN_POINT('Ctrl Pts',(4.66638920507221,17.9701347927033,-333.832600805548)) ;
#44644=CARTESIAN_POINT('Ctrl Pts',(4.52426470362131,18.0063862611952,-333.830708224011)) ;
#44645=CARTESIAN_POINT('Ctrl Pts',(4.45977193103318,18.0224679667486,-333.829855039123)) ;
#44646=CARTESIAN_POINT('Ctrl Pts',(4.29950209943545,18.0615193633396,-333.82774787789)) ;
#44647=CARTESIAN_POINT('Ctrl Pts',(4.20362595769419,18.0840739011969,-333.826498728546)) ;
#44648=CARTESIAN_POINT('Ctrl Pts',(3.77175816303019,18.1820492988108,-333.820914791877)) ;
#44649=CARTESIAN_POINT('Ctrl Pts',(3.43388608153248,18.2488767828614,-333.816661098102)) ;
#44650=CARTESIAN_POINT('Ctrl Pts',(2.68726277554283,18.3750802405742,-333.807359209547)) ;
#44651=CARTESIAN_POINT('Ctrl Pts',(2.27799271379392,18.4302931196425,-333.802322862565)) ;
#44652=CARTESIAN_POINT('Ctrl Pts',(1.46364213842278,18.5126117262138,-333.792248250432)) ;
#44653=CARTESIAN_POINT('Ctrl Pts',(1.05883351414502,18.5401702184589,-333.787214228111)) ;
#44654=CARTESIAN_POINT('Ctrl Pts',(0.494473051735657,18.5600458076499,-333.78009006683)) ;
#44655=CARTESIAN_POINT('Ctrl Pts',(0.335432275881041,18.5636011880126,-333.778071112791)) ;
#44656=CARTESIAN_POINT('Ctrl Pts',(0.0521132528771823,18.5662926741285,
-333.774451608744)) ;
#44657=CARTESIAN_POINT('Ctrl Pts',(-0.0721477423311649,18.5662256289417,
-333.772856305163)) ;
#44658=CARTESIAN_POINT('Ctrl Pts',(-0.34071551233004,18.5633844449062,-333.769390625146)) ;
#44659=CARTESIAN_POINT('Ctrl Pts',(-0.485009577318701,18.560174965229,-333.767517538534)) ;
#44660=CARTESIAN_POINT('Ctrl Pts',(-0.913808476523894,18.5456334302443,
-333.761918219622)) ;
#44661=CARTESIAN_POINT('Ctrl Pts',(-1.19810533775556,18.5294389634879,-333.75816198962)) ;
#44662=CARTESIAN_POINT('Ctrl Pts',(-2.10139076772849,18.4571087950124,-333.746107531459)) ;
#44663=CARTESIAN_POINT('Ctrl Pts',(-2.71798323154306,18.3764325132396,-333.737686877406)) ;
#44664=CARTESIAN_POINT('Ctrl Pts',(-3.53802108650753,18.2269550613262,-333.726503384322)) ;
#44665=CARTESIAN_POINT('Ctrl Pts',(-3.74601189793647,18.1853479229615,-333.723669825537)) ;
#44666=CARTESIAN_POINT('Ctrl Pts',(-4.09790431537208,18.1086609116143,-333.718902910338)) ;
#44667=CARTESIAN_POINT('Ctrl Pts',(-4.24218232867045,18.075406191845,-333.716956297397)) ;
#44668=CARTESIAN_POINT('Ctrl Pts',(-4.45930081313688,18.0226196465507,-333.714046435685)) ;
#44669=CARTESIAN_POINT('Ctrl Pts',(-4.5324452648662,18.0043639878663,-333.713069512077)) ;
#44670=CARTESIAN_POINT('Ctrl Pts',(-4.67065480223079,17.9689735342331,-333.711231325064)) ;
#44671=CARTESIAN_POINT('Ctrl Pts',(-4.73574178028643,17.9519295881244,-333.710369064216)) ;
#44672=CARTESIAN_POINT('Ctrl Pts',(-4.9055812912154,17.9064667671088,-333.708126543744)) ;
#44673=CARTESIAN_POINT('Ctrl Pts',(-5.01017991395002,17.87748240578,-333.706752842434)) ;
#44674=CARTESIAN_POINT('Ctrl Pts',(-5.34894532859809,17.7804036015817,-333.702319879708)) ;
#44675=CARTESIAN_POINT('Ctrl Pts',(-5.58202630834632,17.7086123413543,-333.699294652362)) ;
#44676=CARTESIAN_POINT('Ctrl Pts',(-6.37225276910644,17.448062459815,-333.689037002683)) ;
#44677=CARTESIAN_POINT('Ctrl Pts',(-6.92181120246833,17.237430787031,-333.681891415801)) ;
#44678=CARTESIAN_POINT('Ctrl Pts',(-7.60725702771698,16.9366420850312,-333.672638052061)) ;
#44679=CARTESIAN_POINT('Ctrl Pts',(-7.75323090664983,16.8703175736685,-333.67064796991)) ;
#44680=CARTESIAN_POINT('Ctrl Pts',(-8.10618869083638,16.7043993664949,-333.665780508128)) ;
#44681=CARTESIAN_POINT('Ctrl Pts',(-8.31221868165109,16.6028393233701,-333.662891954769)) ;
#44682=CARTESIAN_POINT('Ctrl Pts',(-8.63647546490246,16.435451874502,-333.658259754524)) ;
#44683=CARTESIAN_POINT('Ctrl Pts',(-8.7559585196429,16.372109733101,-333.656533972646)) ;
#44684=CARTESIAN_POINT('Ctrl Pts',(-8.98581988854134,16.2470161496915,-333.653175737703)) ;
#44685=CARTESIAN_POINT('Ctrl Pts',(-9.09628033315285,16.1854310070601,-333.651544577984)) ;
#44686=CARTESIAN_POINT('Ctrl Pts',(-9.33624777553899,16.0484091735632,-333.647962346435)) ;
#44687=CARTESIAN_POINT('Ctrl Pts',(-9.46548800247803,15.9725231668492,-333.646008046625)) ;
#44688=CARTESIAN_POINT('Ctrl Pts',(-9.99026865752007,15.6557812670232,-333.637970515521)) ;
#44689=CARTESIAN_POINT('Ctrl Pts',(-10.3776488787435,15.4017322558545,-333.631792861434)) ;
#44690=CARTESIAN_POINT('Ctrl Pts',(-11.1365818345413,14.862370214123,-333.61928034052)) ;
#44691=CARTESIAN_POINT('Ctrl Pts',(-11.5076536681429,14.5769479049027,-333.612949141621)) ;
#44692=CARTESIAN_POINT('Ctrl Pts',(-11.9936612400819,14.1729842911952,-333.60450731056)) ;
#44693=CARTESIAN_POINT('Ctrl Pts',(-12.1183841170804,14.066490684263,-333.602327403826)) ;
#44694=CARTESIAN_POINT('Ctrl Pts',(-12.3347543696887,13.8767308829797,-333.598532814423)) ;
#44695=CARTESIAN_POINT('Ctrl Pts',(-12.4270102791998,13.7941741672047,-333.596910668063)) ;
#44696=CARTESIAN_POINT('Ctrl Pts',(-12.5707030980533,13.6629767147845,-333.594382168563)) ;
#44697=CARTESIAN_POINT('Ctrl Pts',(-12.6226992443621,13.6149540174045,-333.593466814658)) ;
#44698=CARTESIAN_POINT('Ctrl Pts',(-12.7200937472086,13.5239647056672,-333.591752626714)) ;
#44699=CARTESIAN_POINT('Ctrl Pts',(-12.7655521980344,13.4810638819443,-333.590952677344)) ;
#44700=CARTESIAN_POINT('Ctrl Pts',(-12.8948185414723,13.3578303287826,-333.588676933265)) ;
#44701=CARTESIAN_POINT('Ctrl Pts',(-12.9780908578955,13.2769399357469,-333.587209698565)) ;
#44702=CARTESIAN_POINT('Ctrl Pts',(-13.331639652637,12.9269995596112,-333.580962157566)) ;
#44703=CARTESIAN_POINT('Ctrl Pts',(-13.5943507165442,12.650437279709,-333.576271993925)) ;
#44704=CARTESIAN_POINT('Ctrl Pts',(-14.1678844608095,12.0081509177686,-333.565714991819)) ;
#44705=CARTESIAN_POINT('Ctrl Pts',(-14.4734218025395,11.6380711347027,-333.559858378116)) ;
#44706=CARTESIAN_POINT('Ctrl Pts',(-14.8520357558492,11.1414757484322,-333.552120820938)) ;
#44707=CARTESIAN_POINT('Ctrl Pts',(-14.9384405700915,11.0253544714751,-333.550320186945)) ;
#44708=CARTESIAN_POINT('Ctrl Pts',(-15.1494712252881,10.7347103304112,-333.545829066294)) ;
#44709=CARTESIAN_POINT('Ctrl Pts',(-15.2724477531899,10.5590162268466,-333.543127874812)) ;
#44710=CARTESIAN_POINT('Ctrl Pts',(-15.4664702909421,10.2713371235415,-333.538718752159)) ;
#44711=CARTESIAN_POINT('Ctrl Pts',(-15.5394085003944,10.1606521918083,-333.537025604286)) ;
#44712=CARTESIAN_POINT('Ctrl Pts',(-15.6795898404427,9.94288425436778,-333.533699481161)) ;
#44713=CARTESIAN_POINT('Ctrl Pts',(-15.7469367700883,9.83587653262878,-333.532067425934)) ;
#44714=CARTESIAN_POINT('Ctrl Pts',(-15.9106771142496,9.5697163749156,-333.528013256429)) ;
#44715=CARTESIAN_POINT('Ctrl Pts',(-16.0057810010364,9.40978703854107,-333.52558169223)) ;
#44716=CARTESIAN_POINT('Ctrl Pts',(-16.4164959449692,8.6948698192667,-333.514734724878)) ;
#44717=CARTESIAN_POINT('Ctrl Pts',(-16.7057598459684,8.125249703337,-333.506135488341)) ;
#44718=CARTESIAN_POINT('Ctrl Pts',(-17.090972395195,7.25873065620679,-333.493364243733)) ;
#44719=CARTESIAN_POINT('Ctrl Pts',(-17.2097332866985,6.97248798422702,-333.4891967115)) ;
#44720=CARTESIAN_POINT('Ctrl Pts',(-17.3892050262139,6.50735408952412,-333.482565162445)) ;
#44721=CARTESIAN_POINT('Ctrl Pts',(-17.4544472120541,6.33027498883063,-333.48007279)) ;
#44722=CARTESIAN_POINT('Ctrl Pts',(-17.5441772127584,6.0747907152436,-333.476537569209)) ;
#44723=CARTESIAN_POINT('Ctrl Pts',(-17.5708619455238,5.99716990116247,-333.475471481229)) ;
#44724=CARTESIAN_POINT('Ctrl Pts',(-17.6181163218021,5.85669277619681,-333.473558119492)) ;
#44725=CARTESIAN_POINT('Ctrl Pts',(-17.6388664331624,5.79389885605945,-333.472708749965)) ;
#44726=CARTESIAN_POINT('Ctrl Pts',(-17.6887291968813,5.64025354774623,-333.470644250884)) ;
#44727=CARTESIAN_POINT('Ctrl Pts',(-17.7174779456772,5.54928607709174,-333.469433449243)) ;
#44728=CARTESIAN_POINT('Ctrl Pts',(-17.8342297195443,5.16969957900751,-333.464421803735)) ;
#44729=CARTESIAN_POINT('Ctrl Pts',(-17.915891486114,4.87917784760495,-333.460683097522)) ;
#44730=CARTESIAN_POINT('Ctrl Pts',(-18.1301344319383,4.03886902972851,-333.45000879692)) ;
#44731=CARTESIAN_POINT('Ctrl Pts',(-18.2447273919423,3.48484733495916,-333.443132978278)) ;
#44732=CARTESIAN_POINT('Ctrl Pts',(-18.36987529007,2.70081382021052,-333.433314142055)) ;
#44733=CARTESIAN_POINT('Ctrl Pts',(-18.4017243567966,2.4745209508225,-333.430471384381)) ;
#44734=CARTESIAN_POINT('Ctrl Pts',(-18.4524154644303,2.05889304739787,-333.425218042883)) ;
#44735=CARTESIAN_POINT('Ctrl Pts',(-18.4725398633097,1.86974540628183,-333.422815256417)) ;
#44736=CARTESIAN_POINT('Ctrl Pts',(-18.5013730181646,1.5524741441585,-333.418759437293)) ;
#44737=CARTESIAN_POINT('Ctrl Pts',(-18.5116653282435,1.42450912418015,-333.417116728114)) ;
#44738=CARTESIAN_POINT('Ctrl Pts',(-18.5298379766709,1.16490060248909,-333.41376909457)) ;
#44739=CARTESIAN_POINT('Ctrl Pts',(-18.5376445174144,1.0332591834301,-333.412063787439)) ;
#44740=CARTESIAN_POINT('Ctrl Pts',(-18.5542722681086,0.691240208612273,
-333.407612518334)) ;
#44741=CARTESIAN_POINT('Ctrl Pts',(-18.560918255816,0.480776131755427,-333.404852958042)) ;
#44742=CARTESIAN_POINT('Ctrl Pts',(-18.5683727225125,-0.0312949001774819,
-333.398092566935)) ;
#44743=CARTESIAN_POINT('Ctrl Pts',(-18.5654147377214,-0.332896377994954,
-333.394071376608)) ;
#44744=CARTESIAN_POINT('Ctrl Pts',(-18.53738235311,-1.15293620149796,-333.38306718218)) ;
#44745=CARTESIAN_POINT('Ctrl Pts',(-18.4979153065857,-1.67060915684535,
-333.376038559188)) ;
#44746=CARTESIAN_POINT('Ctrl Pts',(-18.4166079898426,-2.3563751073202,-333.36680614447)) ;
#44747=CARTESIAN_POINT('Ctrl Pts',(-18.3940391067207,-2.52651518302799,
-333.364522764008)) ;
#44748=CARTESIAN_POINT('Ctrl Pts',(-18.3505456388797,-2.82282166304914,
-333.360571273815)) ;
#44749=CARTESIAN_POINT('Ctrl Pts',(-18.3306704145828,-2.9491303158564,-333.358894870481)) ;
#44750=CARTESIAN_POINT('Ctrl Pts',(-18.2976362631068,-3.14581146565148,
-333.356302171456)) ;
#44751=CARTESIAN_POINT('Ctrl Pts',(-18.2853723783848,-3.21633014411529,
-333.35537614589)) ;
#44752=CARTESIAN_POINT('Ctrl Pts',(-18.2617300550024,-3.34776869689039,
-333.353657964594)) ;
#44753=CARTESIAN_POINT('Ctrl Pts',(-18.2504537970105,-3.4087059216986,-333.352864548875)) ;
#44754=CARTESIAN_POINT('Ctrl Pts',(-18.2177727128358,-3.58050342308387,
-333.350635298725)) ;
#44755=CARTESIAN_POINT('Ctrl Pts',(-18.1956613899698,-3.69122662803234,
-333.349207476479)) ;
#44756=CARTESIAN_POINT('Ctrl Pts',(-18.1047247376207,-4.12590903588858,
-333.34362636548)) ;
#44757=CARTESIAN_POINT('Ctrl Pts',(-18.0282461089619,-4.44820484537856,
-333.33954052548)) ;
#44758=CARTESIAN_POINT('Ctrl Pts',(-17.9267926501359,-4.82997719464514,
-333.334690492664)) ;
#44759=CARTESIAN_POINT('Ctrl Pts',(-17.9100796345253,-4.89158684975666,
-333.333907524337)) ;
#44760=CARTESIAN_POINT('Ctrl Pts',(-17.8849184428461,-4.98248136324957,
-333.3327514136)) ;
#44761=CARTESIAN_POINT('Ctrl Pts',(-17.8767153708889,-5.01183357572234,
-333.332377924923)) ;
#44762=CARTESIAN_POINT('Ctrl Pts',(-17.8622613012014,-5.06306610916138,
-333.331725690591)) ;
#44763=CARTESIAN_POINT('Ctrl Pts',(-17.8560422817328,-5.0849553833973,-333.331446915185)) ;
#44764=CARTESIAN_POINT('Ctrl Pts',(-17.7289416419351,-5.52920699078976,
-333.325786573104)) ;
#44765=CARTESIAN_POINT('Ctrl Pts',(-17.5931466062252,-5.94715846502317,
-333.320411877526)) ;
#44766=CARTESIAN_POINT('Ctrl Pts',(-17.3726313318442,-6.55194358233835,
-333.312426210817)) ;
#44767=CARTESIAN_POINT('Ctrl Pts',(-17.2994413886565,-6.7428192594266,-333.309875342685)) ;
#44768=CARTESIAN_POINT('Ctrl Pts',(-17.1574812137254,-7.09550804337873,
-333.305094131393)) ;
#44769=CARTESIAN_POINT('Ctrl Pts',(-17.0895355599389,-7.25762841460121,
-333.30286922916)) ;
#44770=CARTESIAN_POINT('Ctrl Pts',(-16.968893916478,-7.53439114756365,-333.299020155823)) ;
#44771=CARTESIAN_POINT('Ctrl Pts',(-16.9173125995371,-7.64950619776049,
-333.297403882696)) ;
#44772=CARTESIAN_POINT('Ctrl Pts',(-16.8076829591078,-7.88763542036514,
-333.294027515067)) ;
#44773=CARTESIAN_POINT('Ctrl Pts',(-16.7494477877459,-8.01055539379359,
-333.29226616257)) ;
#44774=CARTESIAN_POINT('Ctrl Pts',(-16.5872887736351,-8.34333184907166,
-333.287446739549)) ;
#44775=CARTESIAN_POINT('Ctrl Pts',(-16.4807369767188,-8.55187953532895,
-333.284370415212)) ;
#44776=CARTESIAN_POINT('Ctrl Pts',(-16.2545256582397,-8.97469180329129,
-333.2780226828)) ;
#44777=CARTESIAN_POINT('Ctrl Pts',(-16.1345054089778,-9.18871222005039,
-333.274749568037)) ;
#44778=CARTESIAN_POINT('Ctrl Pts',(-15.7422714225201,-9.85675279015021,
-333.264365137266)) ;
#44779=CARTESIAN_POINT('Ctrl Pts',(-15.4548658599776,-10.3015438385861,
-333.257194560458)) ;
#44780=CARTESIAN_POINT('Ctrl Pts',(-15.0487989196275,-10.8746540419668,
-333.247802727714)) ;
#44781=CARTESIAN_POINT('Ctrl Pts',(-14.9467784414668,-11.0144570366248,
-333.245499818777)) ;
#44782=CARTESIAN_POINT('Ctrl Pts',(-14.7655569543291,-11.2556372227482,
-333.241518848225)) ;
#44783=CARTESIAN_POINT('Ctrl Pts',(-14.68722915737,-11.3576556218177,-333.239832332498)) ;
#44784=CARTESIAN_POINT('Ctrl Pts',(-14.5635794938802,-11.5152853247837,
-333.237227681259)) ;
#44785=CARTESIAN_POINT('Ctrl Pts',(-14.5189847332259,-11.5714617106029,
-333.236299677707)) ;
#44786=CARTESIAN_POINT('Ctrl Pts',(-14.4353110320079,-11.6756209287948,
-333.23458064765)) ;
#44787=CARTESIAN_POINT('Ctrl Pts',(-14.3963155664725,-11.723669510049,-333.233788334913)) ;
#44788=CARTESIAN_POINT('Ctrl Pts',(-14.2858413079411,-11.8584089090477,
-333.231567079246)) ;
#44789=CARTESIAN_POINT('Ctrl Pts',(-14.2138146635012,-11.9446471902443,
-333.230146054956)) ;
#44790=CARTESIAN_POINT('Ctrl Pts',(-13.98853429261,-12.2094544990122,-333.22577622842)) ;
#44791=CARTESIAN_POINT('Ctrl Pts',(-13.8326651170548,-12.3857679185673,
-333.222857415561)) ;
#44792=CARTESIAN_POINT('Ctrl Pts',(-13.2749867479253,-12.9929312737018,
-333.212693575408)) ;
#44793=CARTESIAN_POINT('Ctrl Pts',(-12.8560631429616,-13.4075791339206,
-333.205537449396)) ;
#44794=CARTESIAN_POINT('Ctrl Pts',(-12.2988693475015,-13.9089198972071,
-333.196271867447)) ;
#44795=CARTESIAN_POINT('Ctrl Pts',(-12.1782161773896,-14.0146812520494,
-333.194280448067)) ;
#44796=CARTESIAN_POINT('Ctrl Pts',(-11.8814612471979,-14.2680825636807,
-333.189410364834)) ;
#44797=CARTESIAN_POINT('Ctrl Pts',(-11.7039600957701,-14.4140424313026,
-333.186520524698)) ;
#44798=CARTESIAN_POINT('Ctrl Pts',(-11.4177533764113,-14.6406181413896,
-333.181886792184)) ;
#44799=CARTESIAN_POINT('Ctrl Pts',(-11.3107969897057,-14.7234052827344,
-333.180160786767)) ;
#44800=CARTESIAN_POINT('Ctrl Pts',(-11.1021051831103,-14.8813222298902,
-333.176802437003)) ;
#44801=CARTESIAN_POINT('Ctrl Pts',(-11.000487798258,-14.9565958343809,-333.175171389659)) ;
#44802=CARTESIAN_POINT('Ctrl Pts',(-10.7768104118294,-15.1187732650137,
-333.171589794287)) ;
#44803=CARTESIAN_POINT('Ctrl Pts',(-10.6544513640579,-15.2052495452927,
-333.16963602323)) ;
#44804=CARTESIAN_POINT('Ctrl Pts',(-9.91982750880368,-15.7112173847607,
-333.157939549185)) ;
#44805=CARTESIAN_POINT('Ctrl Pts',(-9.283904202491,-16.0951683027597,-333.1479207311)) ;
#44806=CARTESIAN_POINT('Ctrl Pts',(-8.27316496431097,-16.625542304717,-333.132560644341)) ;
#44807=CARTESIAN_POINT('Ctrl Pts',(-7.91372136979153,-16.7996110258989,
-333.127207769158)) ;
#44808=CARTESIAN_POINT('Ctrl Pts',(-7.45779720944002,-17.002520805654,-333.120660130185)) ;
#44809=CARTESIAN_POINT('Ctrl Pts',(-7.36632342917403,-17.0423511330805,
-333.1193585085)) ;
#44810=CARTESIAN_POINT('Ctrl Pts',(-7.21323448595236,-17.1075476515262,
-333.117202866894)) ;
#44811=CARTESIAN_POINT('Ctrl Pts',(-7.15179588484512,-17.1333229134784,
-333.116343875141)) ;
#44812=CARTESIAN_POINT('Ctrl Pts',(-7.01673177460878,-17.1891331129643,
-333.11446953512)) ;
#44813=CARTESIAN_POINT('Ctrl Pts',(-6.94304950495508,-17.2190268472688,
-333.113455875768)) ;
#44814=CARTESIAN_POINT('Ctrl Pts',(-6.70924650779701,-17.3121386693541,
-333.110264227876)) ;
#44815=CARTESIAN_POINT('Ctrl Pts',(-6.54843721916864,-17.3736036611754,
-333.108105618731)) ;
#44816=CARTESIAN_POINT('Ctrl Pts',(-5.59749910868084,-17.7219951867835,
-333.095499404855)) ;
#44817=CARTESIAN_POINT('Ctrl Pts',(-4.7894729398757,-17.9572288907603,-333.085379532532)) ;
#44818=CARTESIAN_POINT('Ctrl Pts',(-3.71710613448742,-18.1918590541924,
-333.071720796045)) ;
#44819=CARTESIAN_POINT('Ctrl Pts',(-3.46480671498847,-18.2415933491819,
-333.068495469153)) ;
#44820=CARTESIAN_POINT('Ctrl Pts',(-3.07374632681347,-18.3102747194317,
-333.063462976479)) ;
#44821=CARTESIAN_POINT('Ctrl Pts',(-2.93566733276767,-18.3329194080751,
-333.061679801131)) ;
#44822=CARTESIAN_POINT('Ctrl Pts',(-2.67380805737983,-18.3728295571781,
-333.058284644254)) ;
#44823=CARTESIAN_POINT('Ctrl Pts',(-2.55008357236757,-18.3904102506348,
-333.056674829264)) ;
#44824=CARTESIAN_POINT('Ctrl Pts',(-2.26391990133328,-18.4281294636121,
-333.052937799777)) ;
#44825=CARTESIAN_POINT('Ctrl Pts',(-2.10137310712073,-18.4473716230041,
-333.050804917556)) ;
#44826=CARTESIAN_POINT('Ctrl Pts',(-1.48812799914729,-18.5117565419224,
-333.042720739618)) ;
#44827=CARTESIAN_POINT('Ctrl Pts',(-1.03608411202386,-18.5425506028167,
-333.036681729249)) ;
#44828=CARTESIAN_POINT('Ctrl Pts',(-0.544158216969694,-18.5580152554972,
-333.030069792708)) ;
#44829=CARTESIAN_POINT('Ctrl Pts',(-0.504943872655379,-18.5591236343007,
-333.029542473251)) ;
#44830=CARTESIAN_POINT('Ctrl Pts',(0.0372160390379098,-18.5727279808557,
-333.022249287284)) ;
#44831=CARTESIAN_POINT('Ctrl Pts',(0.540463392778109,-18.5648999197735,
-333.015440918262)) ;
#44832=CARTESIAN_POINT('Ctrl Pts',(1.23205076363308,-18.5259950052167,-333.006226404174)) ;
#44833=CARTESIAN_POINT('Ctrl Pts',(1.42115774437797,-18.5124485389726,-333.003722245486)) ;
#44834=CARTESIAN_POINT('Ctrl Pts',(1.69192281180645,-18.4888792196527,-333.000173742365)) ;
#44835=CARTESIAN_POINT('Ctrl Pts',(1.7737732018656,-18.4812062986659,-332.999105928424)) ;
#44836=CARTESIAN_POINT('Ctrl Pts',(1.92135361262873,-18.4663821807441,-332.997191069649)) ;
#44837=CARTESIAN_POINT('Ctrl Pts',(1.98710131570599,-18.4594230383671,-332.996341906909)) ;
#44838=CARTESIAN_POINT('Ctrl Pts',(2.1474303671283,-18.4415863182516,-332.994280091972)) ;
#44839=CARTESIAN_POINT('Ctrl Pts',(2.24196789579737,-18.4303321485726,-332.9930717359)) ;
#44840=CARTESIAN_POINT('Ctrl Pts',(2.6310336042233,-18.3809781729037,-332.98812232515)) ;
#44841=CARTESIAN_POINT('Ctrl Pts',(2.92471402419203,-18.3365412509288,-332.984441352276)) ;
#44842=CARTESIAN_POINT('Ctrl Pts',(3.35323236843257,-18.2611447917583,-332.979084366988)) ;
#44843=CARTESIAN_POINT('Ctrl Pts',(3.48899117366929,-18.2356934894022,-332.977389420714)) ;
#44844=CARTESIAN_POINT('Ctrl Pts',(3.6503414371363,-18.2035766689314,-332.975372888862)) ;
#44845=CARTESIAN_POINT('Ctrl Pts',(3.67621850707237,-18.1983684333975,-332.975049418475)) ;
#44846=CARTESIAN_POINT('Ctrl Pts',(4.14721753276944,-18.102525632827,-332.969160193723)) ;
#44847=CARTESIAN_POINT('Ctrl Pts',(4.5888763651798,-17.9956400538634,-332.96360726497)) ;
#44848=CARTESIAN_POINT('Ctrl Pts',(5.1613354044454,-17.8346525368428,-332.956233668114)) ;
#44849=CARTESIAN_POINT('Ctrl Pts',(5.29606622703783,-17.7951087867409,-332.954485658933)) ;
#44850=CARTESIAN_POINT('Ctrl Pts',(5.63121336889924,-17.6925990857405,-332.950100840433)) ;
#44851=CARTESIAN_POINT('Ctrl Pts',(5.83103379149865,-17.6277528663971,-332.94745349345)) ;
#44852=CARTESIAN_POINT('Ctrl Pts',(6.15434988998392,-17.5167303917779,-332.943108402183)) ;
#44853=CARTESIAN_POINT('Ctrl Pts',(6.27852995990068,-17.4726050624739,-332.941424597006)) ;
#44854=CARTESIAN_POINT('Ctrl Pts',(6.52138634063726,-17.3833867285,-332.938100962584)) ;
#44855=CARTESIAN_POINT('Ctrl Pts',(6.64009087741226,-17.3383911318642,-332.936461879296)) ;
#44856=CARTESIAN_POINT('Ctrl Pts',(6.9345918049107,-17.2232909747025,-332.932358509805)) ;
#44857=CARTESIAN_POINT('Ctrl Pts',(7.10979519491607,-17.1517091746467,-332.929884237081)) ;
#44858=CARTESIAN_POINT('Ctrl Pts',(7.61203546791065,-16.9374938158835,-332.922697475816)) ;
#44859=CARTESIAN_POINT('Ctrl Pts',(7.93609426646273,-16.7880966034519,-332.917942614331)) ;
#44860=CARTESIAN_POINT('Ctrl Pts',(8.33557230198092,-16.5897768638928,-332.911958661224)) ;
#44861=CARTESIAN_POINT('Ctrl Pts',(8.41521118746939,-16.5495221277923,-332.910759603925)) ;
#44862=CARTESIAN_POINT('Ctrl Pts',(8.70344943512226,-16.40120900095,-332.906399509063)) ;
#44863=CARTESIAN_POINT('Ctrl Pts',(8.91028319052653,-16.2897680215416,-332.903231597078)) ;
#44864=CARTESIAN_POINT('Ctrl Pts',(9.35693018908766,-16.0380643855839,-332.896331454507)) ;
#44865=CARTESIAN_POINT('Ctrl Pts',(9.59582367187074,-15.8962832185917,-332.892602377735)) ;
#44866=CARTESIAN_POINT('Ctrl Pts',(9.98116717012184,-15.6557322764152,-332.886568058921)) ;
#44867=CARTESIAN_POINT('Ctrl Pts',(10.1295480204247,-15.5601384402183,-332.884239817908)) ;
#44868=CARTESIAN_POINT('Ctrl Pts',(10.34334515574,-15.418046049537,-332.880890520515)) ;
#44869=CARTESIAN_POINT('Ctrl Pts',(10.409858547089,-15.373216255875,-332.879849323828)) ;
#44870=CARTESIAN_POINT('Ctrl Pts',(10.530954039724,-15.2904520616228,-332.87795671976)) ;
#44871=CARTESIAN_POINT('Ctrl Pts',(10.5856267773618,-15.2526529810222,-332.877103540131)) ;
#44872=CARTESIAN_POINT('Ctrl Pts',(10.7208050231096,-15.1581179217008,-332.874996431596)) ;
#44873=CARTESIAN_POINT('Ctrl Pts',(10.8010643091807,-15.1010333785959,-332.87374732908)) ;
#44874=CARTESIAN_POINT('Ctrl Pts',(11.1599329203825,-14.8414628188532,-332.868162609989)) ;
#44875=CARTESIAN_POINT('Ctrl Pts',(11.4333301451273,-14.6318858762706,-332.863908122262)) ;
#44876=CARTESIAN_POINT('Ctrl Pts',(12.0212907954074,-14.1546290028262,-332.854605456179)) ;
#44877=CARTESIAN_POINT('Ctrl Pts',(12.3330734993834,-13.8838126197973,-332.849569113175)) ;
#44878=CARTESIAN_POINT('Ctrl Pts',(12.8389638225102,-13.4138947703999,-332.841070371004)) ;
#44879=CARTESIAN_POINT('Ctrl Pts',(13.0380963319374,-13.2204239209766,-332.837634644567)) ;
#44880=CARTESIAN_POINT('Ctrl Pts',(13.3854128889989,-12.867499803572,-332.8314456633)) ;
#44881=CARTESIAN_POINT('Ctrl Pts',(13.5352728976098,-12.7097685561562,-332.828706175293)) ;
#44882=CARTESIAN_POINT('Ctrl Pts',(13.7722939630875,-12.4513506979463,-332.82425147736)) ;
#44883=CARTESIAN_POINT('Ctrl Pts',(13.8612043676685,-12.3522964919465,-332.822551662309)) ;
#44884=CARTESIAN_POINT('Ctrl Pts',(14.0322636603256,-12.1575482219666,-332.819223282005)) ;
#44885=CARTESIAN_POINT('Ctrl Pts',(14.1145178856588,-12.0619561848061,-332.817595756327)) ;
#44886=CARTESIAN_POINT('Ctrl Pts',(14.2951272822193,-11.8476829683592,-332.813960781191)) ;
#44887=CARTESIAN_POINT('Ctrl Pts',(14.3929912802687,-11.7285999865457,-332.811949399969)) ;
#44888=CARTESIAN_POINT('Ctrl Pts',(14.9427819225857,-11.0423576764162,-332.800409483092)) ;
#44889=CARTESIAN_POINT('Ctrl Pts',(15.3626527370053,-10.4503247213044,-332.790621728403)) ;
#44890=CARTESIAN_POINT('Ctrl Pts',(15.8930124970672,-9.60118825909509,-332.777148086387)) ;
#44891=CARTESIAN_POINT('Ctrl Pts',(16.03397298161,-9.36388663691548,-332.773443414459)) ;
#44892=CARTESIAN_POINT('Ctrl Pts',(16.2559757189144,-8.97043222789427,-332.767442758364)) ;
#44893=CARTESIAN_POINT('Ctrl Pts',(16.3401816093379,-8.81611400160364,-332.765124063464)) ;
#44894=CARTESIAN_POINT('Ctrl Pts',(16.459547058751,-8.58977447864423,-332.761785635381)) ;
#44895=CARTESIAN_POINT('Ctrl Pts',(16.4964518984026,-8.51868474359152,-332.76074593629)) ;
#44896=CARTESIAN_POINT('Ctrl Pts',(16.5631485078854,-8.38814830453622,-332.758854527169)) ;
#44897=CARTESIAN_POINT('Ctrl Pts',(16.5930830832363,-8.3287762762166,-332.758001064639)) ;
#44898=CARTESIAN_POINT('Ctrl Pts',(16.6666543092695,-8.18088462090552,-332.755891138458)) ;
#44899=CARTESIAN_POINT('Ctrl Pts',(16.7099053305672,-8.09217541392718,-332.75463953383)) ;
#44900=CARTESIAN_POINT('Ctrl Pts',(16.9002205556867,-7.69380033799361,-332.7490727928)) ;
#44901=CARTESIAN_POINT('Ctrl Pts',(17.0393988278243,-7.38044085099692,-332.74483786168)) ;
#44902=CARTESIAN_POINT('Ctrl Pts',(17.3716548903147,-6.57278856447777,-332.734109208009)) ;
#44903=CARTESIAN_POINT('Ctrl Pts',(17.5523666019045,-6.0737443320153,-332.72764827758)) ;
#44904=CARTESIAN_POINT('Ctrl Pts',(17.7782196889635,-5.35527436640358,-332.718327791977)) ;
#44905=CARTESIAN_POINT('Ctrl Pts',(17.841154658909,-5.14171752177126,-332.715556268902)) ;
#44906=CARTESIAN_POINT('Ctrl Pts',(17.9497913517044,-4.74703713211614,-332.710417468934)) ;
#44907=CARTESIAN_POINT('Ctrl Pts',(17.9966295609324,-4.56625616796636,-332.708057379554)) ;
#44908=CARTESIAN_POINT('Ctrl Pts',(18.0709180036974,-4.26060527506791,-332.704051595018)) ;
#44909=CARTESIAN_POINT('Ctrl Pts',(18.0998201592889,-4.13610262839098,-332.702415626751)) ;
#44910=CARTESIAN_POINT('Ctrl Pts',(18.1561050314027,-3.88174683897472,-332.699063668517)) ;
#44911=CARTESIAN_POINT('Ctrl Pts',(18.1833857054804,-3.75187855035543,-332.697347105609)) ;
#44912=CARTESIAN_POINT('Ctrl Pts',(18.2512659101287,-3.41059154049628,-332.692822216165)) ;
#44913=CARTESIAN_POINT('Ctrl Pts',(18.2895845965861,-3.19873990971338,-332.689999401413)) ;
#44914=CARTESIAN_POINT('Ctrl Pts',(18.3708577754708,-2.70003526168335,-332.683325378463)) ;
#44915=CARTESIAN_POINT('Ctrl Pts',(18.41079185662,-2.41274709572377,-332.679457954179)) ;
#44916=CARTESIAN_POINT('Ctrl Pts',(18.491288153212,-1.71396019208233,-332.670025252939)) ;
#44917=CARTESIAN_POINT('Ctrl Pts',(18.5248630693649,-1.30184302996486,-332.664439221364)) ;
#44918=CARTESIAN_POINT('Ctrl Pts',(18.5446545941347,-0.888979969817808,
-332.65888667131)) ;
#44919=CARTESIAN_POINT('',(-0.00018199629320621,-18.565949999108,-332.726272944078)) ;
#44920=CARTESIAN_POINT('Ctrl Pts',(18.544654593742,-0.888979978009869,-332.362654732516)) ;
#44921=CARTESIAN_POINT('Ctrl Pts',(18.5409868706898,-0.965490876829128,
-332.363641300434)) ;
#44922=CARTESIAN_POINT('Ctrl Pts',(18.5368456630169,-1.0419787767752,-332.364630914379)) ;
#44923=CARTESIAN_POINT('Ctrl Pts',(18.5217124712218,-1.2927315997512,-332.367886299804)) ;
#44924=CARTESIAN_POINT('Ctrl Pts',(18.5087355062214,-1.46686661895616,-332.370164677092)) ;
#44925=CARTESIAN_POINT('Ctrl Pts',(18.4754067491204,-1.84251367258044,-332.375116982855)) ;
#44926=CARTESIAN_POINT('Ctrl Pts',(18.4542100364302,-2.04392830592316,-332.37779565012)) ;
#44927=CARTESIAN_POINT('Ctrl Pts',(18.3776161067625,-2.67271798459491,-332.386222756599)) ;
#44928=CARTESIAN_POINT('Ctrl Pts',(18.3106326642475,-3.09853602029094,-332.392026252816)) ;
#44929=CARTESIAN_POINT('Ctrl Pts',(18.1424767781622,-3.96895420045448,-332.403967813284)) ;
#44930=CARTESIAN_POINT('Ctrl Pts',(18.0396235006283,-4.41294075369034,-332.410102143892)) ;
#44931=CARTESIAN_POINT('Ctrl Pts',(17.8902346562831,-4.96461976450407,-332.417627154172)) ;
#44932=CARTESIAN_POINT('Ctrl Pts',(17.8588782837582,-5.07625964389746,-332.419144621208)) ;
#44933=CARTESIAN_POINT('Ctrl Pts',(17.8090195386367,-5.24759245222634,-332.421461410201)) ;
#44934=CARTESIAN_POINT('Ctrl Pts',(17.791258235538,-5.30749789265439,-332.422269176853)) ;
#44935=CARTESIAN_POINT('Ctrl Pts',(17.7527239993247,-5.43509927222149,-332.423983995539)) ;
#44936=CARTESIAN_POINT('Ctrl Pts',(17.7318654957402,-5.50276835324022,-332.424889900873)) ;
#44937=CARTESIAN_POINT('Ctrl Pts',(17.6734297404255,-5.68856272965468,-332.427369518159)) ;
#44938=CARTESIAN_POINT('Ctrl Pts',(17.6350557814675,-5.80643370570242,-332.428934086973)) ;
#44939=CARTESIAN_POINT('Ctrl Pts',(17.5430835655907,-6.07961426783794,-332.432548681069)) ;
#44940=CARTESIAN_POINT('Ctrl Pts',(17.4885983982314,-6.2346144084199,-332.434590891464)) ;
#44941=CARTESIAN_POINT('Ctrl Pts',(17.2703839569688,-6.83001348206777,-332.442431959297)) ;
#44942=CARTESIAN_POINT('Ctrl Pts',(17.0920173096295,-7.26486005268108,-332.448155136249)) ;
#44943=CARTESIAN_POINT('Ctrl Pts',(16.7063296984482,-8.11206469713462,-332.459584149927)) ;
#44944=CARTESIAN_POINT('Ctrl Pts',(16.4997489320953,-8.52439613518244,-332.465284461519)) ;
#44945=CARTESIAN_POINT('Ctrl Pts',(16.2060261536226,-9.05989162087997,-332.47297873807)) ;
#44946=CARTESIAN_POINT('Ctrl Pts',(16.1324313039198,-9.19029814611917,-332.474875686368)) ;
#44947=CARTESIAN_POINT('Ctrl Pts',(15.9937972000412,-9.42915357596829,-332.478395817969)) ;
#44948=CARTESIAN_POINT('Ctrl Pts',(15.9292119177615,-9.53785582092768,-332.480015573261)) ;
#44949=CARTESIAN_POINT('Ctrl Pts',(15.7932306403496,-9.76148909423286,-332.483385838611)) ;
#44950=CARTESIAN_POINT('Ctrl Pts',(15.7216785042645,-9.87631653698226,-332.485137465665)) ;
#44951=CARTESIAN_POINT('Ctrl Pts',(15.5250964041906,-10.1842425639224,-332.489892491676)) ;
#44952=CARTESIAN_POINT('Ctrl Pts',(15.3977224475582,-10.3758160200987,-332.492913292005)) ;
#44953=CARTESIAN_POINT('Ctrl Pts',(15.1753762556539,-10.6971154466316,-332.498083256662)) ;
#44954=CARTESIAN_POINT('Ctrl Pts',(15.0822189537513,-10.8280651423035,-332.500220409201)) ;
#44955=CARTESIAN_POINT('Ctrl Pts',(14.6384377756168,-11.4350410914577,-332.51025984871)) ;
#44956=CARTESIAN_POINT('Ctrl Pts',(14.2669060409798,-11.8953526650251,-332.518274623767)) ;
#44957=CARTESIAN_POINT('Ctrl Pts',(13.7307723517689,-12.4982750308487,-332.529079789098)) ;
#44958=CARTESIAN_POINT('Ctrl Pts',(13.584700872033,-12.6568910316472,-332.531952136263)) ;
#44959=CARTESIAN_POINT('Ctrl Pts',(13.35203643845,-12.9008677614489,-332.536395435434)) ;
#44960=CARTESIAN_POINT('Ctrl Pts',(13.2673116211508,-12.9879832334004,-332.537987133545)) ;
#44961=CARTESIAN_POINT('Ctrl Pts',(13.1370589384309,-13.1193066572941,-332.540390125203)) ;
#44962=CARTESIAN_POINT('Ctrl Pts',(13.0921496439651,-13.164123306637,-332.541210833072)) ;
#44963=CARTESIAN_POINT('Ctrl Pts',(13.01356401674,-13.2417469099432,-332.542632689696)) ;
#44964=CARTESIAN_POINT('Ctrl Pts',(12.9799911976487,-13.2746577414469,-332.543235613906)) ;
#44965=CARTESIAN_POINT('Ctrl Pts',(12.8997183716975,-13.3527520653254,-332.544666976938)) ;
#44966=CARTESIAN_POINT('Ctrl Pts',(12.852905411894,-13.3978186385798,-332.545493540795)) ;
#44967=CARTESIAN_POINT('Ctrl Pts',(12.8048044867707,-13.4436410086833,-332.54633508729)) ;
#44968=CARTESIAN_POINT('Ctrl Pts',(12.8037520618402,-13.4446433442356,-332.546353496141)) ;
#44969=CARTESIAN_POINT('Ctrl Pts',(12.8015299140816,-13.446759232976,-332.546392357637)) ;
#44970=CARTESIAN_POINT('Ctrl Pts',(12.8003601636317,-13.4478727571338,-332.54641280988)) ;
#44971=CARTESIAN_POINT('Ctrl Pts',(12.7978893088446,-13.4502242310845,-332.546456001175)) ;
#44972=CARTESIAN_POINT('Ctrl Pts',(12.7965881701203,-13.4514621447718,-332.54647873973)) ;
#44973=CARTESIAN_POINT('Ctrl Pts',(12.7938386573008,-13.4540772930743,-332.546526777789)) ;
#44974=CARTESIAN_POINT('Ctrl Pts',(12.7923902403966,-13.4554544826427,-332.546552076675)) ;
#44975=CARTESIAN_POINT('Ctrl Pts',(12.7893282179307,-13.4583649858114,-332.54660554475)) ;
#44976=CARTESIAN_POINT('Ctrl Pts',(12.7877145589167,-13.4598982431868,-332.54663371317)) ;
#44977=CARTESIAN_POINT('Ctrl Pts',(12.7843017506741,-13.463139838298,-332.546693269437)) ;
#44978=CARTESIAN_POINT('Ctrl Pts',(12.7825025346857,-13.4648481056643,-332.546724656326)) ;
#44979=CARTESIAN_POINT('Ctrl Pts',(12.7786956554764,-13.468461100137,-332.546791043452)) ;
#44980=CARTESIAN_POINT('Ctrl Pts',(12.7766879086751,-13.4703657391146,-332.546826042496)) ;
#44981=CARTESIAN_POINT('Ctrl Pts',(12.7724380161347,-13.4743955734633,-332.546900098139)) ;
#44982=CARTESIAN_POINT('Ctrl Pts',(12.7701957656623,-13.476520658272,-332.546939153251)) ;
#44983=CARTESIAN_POINT('Ctrl Pts',(12.7654475493937,-13.4810185140472,-332.547021821446)) ;
#44984=CARTESIAN_POINT('Ctrl Pts',(12.7629414521835,-13.4833911461674,-332.547065432674)) ;
#44985=CARTESIAN_POINT('Ctrl Pts',(12.75763246256,-13.4884145931151,-332.547157776002)) ;
#44986=CARTESIAN_POINT('Ctrl Pts',(12.754829405148,-13.491065233372,-332.547206505789)) ;
#44987=CARTESIAN_POINT('Ctrl Pts',(12.7488892289613,-13.4966789045023,-332.54730971815)) ;
#44988=CARTESIAN_POINT('Ctrl Pts',(12.7457519028935,-13.4996417157439,-332.547364197842)) ;
#44989=CARTESIAN_POINT('Ctrl Pts',(12.7391012973305,-13.5059179940145,-332.547479617562)) ;
#44990=CARTESIAN_POINT('Ctrl Pts',(12.7355877573517,-13.5092311846192,-332.547540554)) ;
#44991=CARTESIAN_POINT('Ctrl Pts',(12.7281377605599,-13.5162508775382,-332.547669676858)) ;
#44992=CARTESIAN_POINT('Ctrl Pts',(12.7242009764884,-13.5199570319687,-332.547737858814)) ;
#44993=CARTESIAN_POINT('Ctrl Pts',(12.7158520214465,-13.5278100014189,-332.547882350458)) ;
#44994=CARTESIAN_POINT('Ctrl Pts',(12.7114394396194,-13.5319563788357,-332.547958654604)) ;
#44995=CARTESIAN_POINT('Ctrl Pts',(12.7050382142322,-13.5379655340834,-332.548069257284)) ;
#44996=CARTESIAN_POINT('Ctrl Pts',(12.7030511879628,-13.5398300337608,-332.548103577291)) ;
#44997=CARTESIAN_POINT('Ctrl Pts',(12.6983451597256,-13.5442439249794,-332.548184830406)) ;
#44998=CARTESIAN_POINT('Ctrl Pts',(12.6956258004738,-13.5467929352011,-332.548231758789)) ;
#44999=CARTESIAN_POINT('Ctrl Pts',(12.6891931047241,-13.5528190289879,-332.548342713677)) ;
#45000=CARTESIAN_POINT('Ctrl Pts',(12.6854791063044,-13.5562954056407,-332.548406731505)) ;
#45001=CARTESIAN_POINT('Ctrl Pts',(12.676709544919,-13.5644971305199,-332.548557789804)) ;
#45002=CARTESIAN_POINT('Ctrl Pts',(12.6716527677834,-13.5692211796721,-332.548644814534)) ;
#45003=CARTESIAN_POINT('Ctrl Pts',(12.6597452500862,-13.5803327403396,-332.548849551092)) ;
#45004=CARTESIAN_POINT('Ctrl Pts',(12.6528923143566,-13.5867178971502,-332.548967234885)) ;
#45005=CARTESIAN_POINT('Ctrl Pts',(12.6368208738301,-13.6016696023582,-332.549242890204)) ;
#45006=CARTESIAN_POINT('Ctrl Pts',(12.6275984849127,-13.6102319698409,-332.549400813138)) ;
#45007=CARTESIAN_POINT('Ctrl Pts',(12.4983428206846,-13.7299926874607,-332.551610607558)) ;
#45008=CARTESIAN_POINT('Ctrl Pts',(12.3768532024904,-13.8396090040588,-332.55364472926)) ;
#45009=CARTESIAN_POINT('Ctrl Pts',(11.904103637039,-14.2549520122255,-332.561426604256)) ;
#45010=CARTESIAN_POINT('Ctrl Pts',(11.5428373024626,-14.5490291213305,-332.567099681078)) ;
#45011=CARTESIAN_POINT('Ctrl Pts',(10.7989595345716,-15.1093948371796,-332.578532570543)) ;
#45012=CARTESIAN_POINT('Ctrl Pts',(10.4166128295706,-15.3754842252688,-332.584288652172)) ;
#45013=CARTESIAN_POINT('Ctrl Pts',(9.8871001486967,-15.7151666607572,-332.592213475305)) ;
#45014=CARTESIAN_POINT('Ctrl Pts',(9.74837264789605,-15.8015962210896,-332.594284999122)) ;
#45015=CARTESIAN_POINT('Ctrl Pts',(9.51904113291167,-15.9403039899409,-332.597704701943)) ;
#45016=CARTESIAN_POINT('Ctrl Pts',(9.4291044502902,-15.9936682664424,-332.599044607796)) ;
#45017=CARTESIAN_POINT('Ctrl Pts',(9.22697557530512,-16.1113046610739,-332.602053913314)) ;
#45018=CARTESIAN_POINT('Ctrl Pts',(9.11455317023766,-16.1751703730894,-332.603726262867)) ;
#45019=CARTESIAN_POINT('Ctrl Pts',(8.88289600347169,-16.3035897687109,-332.607169767099)) ;
#45020=CARTESIAN_POINT('Ctrl Pts',(8.76360270731259,-16.3680221248359,-332.608941672812)) ;
#45021=CARTESIAN_POINT('Ctrl Pts',(8.14939385975142,-16.6911271470905,-332.618056551196)) ;
#45022=CARTESIAN_POINT('Ctrl Pts',(7.64369650447566,-16.9286811569303,-332.625544074346)) ;
#45023=CARTESIAN_POINT('Ctrl Pts',(6.63009557290528,-17.3501347971755,-332.64032768909)) ;
#45024=CARTESIAN_POINT('Ctrl Pts',(6.12334035574825,-17.5353941693649,-332.647613201731)) ;
#45025=CARTESIAN_POINT('Ctrl Pts',(5.50403285938207,-17.7316751127372,-332.656157204252)) ;
#45026=CARTESIAN_POINT('Ctrl Pts',(5.39852924709108,-17.7640806698403,-332.657600083318)) ;
#45027=CARTESIAN_POINT('Ctrl Pts',(5.23373904423387,-17.8130925005906,-332.659830742326)) ;
#45028=CARTESIAN_POINT('Ctrl Pts',(5.17464822546492,-17.8303478536104,-332.66062602472)) ;
#45029=CARTESIAN_POINT('Ctrl Pts',(5.05733082060934,-17.8639738736241,-332.662195094564)) ;
#45030=CARTESIAN_POINT('Ctrl Pts',(4.99910790565926,-17.8803545195542,-332.66296904373)) ;
#45031=CARTESIAN_POINT('Ctrl Pts',(4.86967388166753,-17.9160883316886,-332.664680029477)) ;
#45032=CARTESIAN_POINT('Ctrl Pts',(4.79842530900951,-17.9353020435515,-332.665615460567)) ;
#45033=CARTESIAN_POINT('Ctrl Pts',(4.45985225517868,-18.024443652093,-332.670033992866)) ;
#45034=CARTESIAN_POINT('Ctrl Pts',(4.191102559177,-18.0888228212409,-332.673463197062)) ;
#45035=CARTESIAN_POINT('Ctrl Pts',(3.31931893444489,-18.2771869378127,-332.684455730257)) ;
#45036=CARTESIAN_POINT('Ctrl Pts',(2.71152845299985,-18.3771884593749,-332.69193046579)) ;
#45037=CARTESIAN_POINT('Ctrl Pts',(1.79635042048582,-18.4813678616395,-332.703336185325)) ;
#45038=CARTESIAN_POINT('Ctrl Pts',(1.49199948812602,-18.5084242934456,-332.707151221583)) ;
#45039=CARTESIAN_POINT('Ctrl Pts',(1.04052901559977,-18.5373508354029,-332.712870389489)) ;
#45040=CARTESIAN_POINT('Ctrl Pts',(0.893831572952765,-18.5450031454643,
-332.714737914278)) ;
#45041=CARTESIAN_POINT('Ctrl Pts',(0.633226507880376,-18.5554979029746,
-332.718073822772)) ;
#45042=CARTESIAN_POINT('Ctrl Pts',(0.519354396397132,-18.559034166926,-332.719537637324)) ;
#45043=CARTESIAN_POINT('Ctrl Pts',(0.270264067520439,-18.5644752847932,
-332.722753767207)) ;
#45044=CARTESIAN_POINT('Ctrl Pts',(0.135042993128688,-18.5659513246769,
-332.724508765686)) ;
#45045=CARTESIAN_POINT('Ctrl Pts',(-0.000181996293217197,-18.565949999108,
-332.726272944078)) ;
#45046=CARTESIAN_POINT('Ctrl Pts',(-0.000181996293162345,-18.565949999108,
-332.726272944078)) ;
#45047=CARTESIAN_POINT('Ctrl Pts',(-0.176929924793901,-18.5659482665024,
-332.728578840921)) ;
#45048=CARTESIAN_POINT('Ctrl Pts',(-0.353668593251895,-18.5634225729408,
-332.730900257364)) ;
#45049=CARTESIAN_POINT('Ctrl Pts',(-1.23228127524413,-18.5383143938595,
-332.742513137644)) ;
#45050=CARTESIAN_POINT('Ctrl Pts',(-1.93251401323006,-18.4784469184749,
-332.752022876382)) ;
#45051=CARTESIAN_POINT('Ctrl Pts',(-2.85588299120307,-18.3464323542094,
-332.764551949736)) ;
#45052=CARTESIAN_POINT('Ctrl Pts',(-3.08347441316332,-18.3095557992409,
-332.76763672847)) ;
#45053=CARTESIAN_POINT('Ctrl Pts',(-3.42092087897222,-18.2484090793984,
-332.772181144825)) ;
#45054=CARTESIAN_POINT('Ctrl Pts',(-3.53133749106253,-18.2273637469237,
-332.773663379807)) ;
#45055=CARTESIAN_POINT('Ctrl Pts',(-3.71324816206135,-18.1909766879873,
-332.776093915746)) ;
#45056=CARTESIAN_POINT('Ctrl Pts',(-3.78485478925804,-18.1762129998792,
-332.777047722042)) ;
#45057=CARTESIAN_POINT('Ctrl Pts',(-3.91543010248418,-18.1484862066509,
-332.778780460323)) ;
#45058=CARTESIAN_POINT('Ctrl Pts',(-3.97442633978652,-18.1356576875728,
-332.779560897449)) ;
#45059=CARTESIAN_POINT('Ctrl Pts',(-4.09381883038044,-18.1090856544887,
-332.781134577953)) ;
#45060=CARTESIAN_POINT('Ctrl Pts',(-4.15421098431024,-18.0953272134762,
-332.781927600122)) ;
#45061=CARTESIAN_POINT('Ctrl Pts',(-4.3243022977065,-18.0556809048547,-332.784154003867)) ;
#45062=CARTESIAN_POINT('Ctrl Pts',(-4.43383628045254,-18.0290959062432,
-332.78557940658)) ;
#45063=CARTESIAN_POINT('Ctrl Pts',(-5.03576689168719,-17.8771840324648,
-332.793381650613)) ;
#45064=CARTESIAN_POINT('Ctrl Pts',(-5.52310234356574,-17.7326817118893,
-332.799590249782)) ;
#45065=CARTESIAN_POINT('Ctrl Pts',(-6.55537570103544,-17.379907846883,-332.812951873021)) ;
#45066=CARTESIAN_POINT('Ctrl Pts',(-7.0976741910527,-17.1655808796899,-332.820105890676)) ;
#45067=CARTESIAN_POINT('Ctrl Pts',(-7.75311857595609,-16.8701567734299,
-332.829146257708)) ;
#45068=CARTESIAN_POINT('Ctrl Pts',(-7.87662706486075,-16.8128457803031,
-332.830866921865)) ;
#45069=CARTESIAN_POINT('Ctrl Pts',(-8.1100755980492,-16.7013828533122,-332.834154145294)) ;
#45070=CARTESIAN_POINT('Ctrl Pts',(-8.22013179967204,-16.6474907588765,
-332.835718824259)) ;
#45071=CARTESIAN_POINT('Ctrl Pts',(-8.44020691714935,-16.537010334569,-332.838878912442)) ;
#45072=CARTESIAN_POINT('Ctrl Pts',(-8.55020991456653,-16.4804039385023,
-332.840474393702)) ;
#45073=CARTESIAN_POINT('Ctrl Pts',(-8.81054845943651,-16.3431282502931,
-332.844288980448)) ;
#45074=CARTESIAN_POINT('Ctrl Pts',(-8.96035389264517,-16.2614778895082,
-332.84651508752)) ;
#45075=CARTESIAN_POINT('Ctrl Pts',(-9.79018821526244,-15.7942336964093,
-332.859019194102)) ;
#45076=CARTESIAN_POINT('Ctrl Pts',(-10.4464584434506,-15.3680544684858,
-332.869601025997)) ;
#45077=CARTESIAN_POINT('Ctrl Pts',(-11.2642053296691,-14.7603655938016,
-332.883290971973)) ;
#45078=CARTESIAN_POINT('Ctrl Pts',(-11.4517824153023,-14.6153136788311,
-332.886465129517)) ;
#45079=CARTESIAN_POINT('Ctrl Pts',(-11.7255762648179,-14.3950831937948,
-332.891123080878)) ;
#45080=CARTESIAN_POINT('Ctrl Pts',(-11.8139594273255,-14.3226366846006,
-332.892630609544)) ;
#45081=CARTESIAN_POINT('Ctrl Pts',(-11.9583122307089,-14.2020672763326,
-332.8950955234)) ;
#45082=CARTESIAN_POINT('Ctrl Pts',(-12.0146737414955,-14.1544184349344,
-332.896058623406)) ;
#45083=CARTESIAN_POINT('Ctrl Pts',(-12.1067113572339,-14.0756626728235,
-332.897631423471)) ;
#45084=CARTESIAN_POINT('Ctrl Pts',(-12.1425552574274,-14.044753162371,-332.898243964958)) ;
#45085=CARTESIAN_POINT('Ctrl Pts',(-12.2288590228466,-13.9697529159751,
-332.89971843141)) ;
#45086=CARTESIAN_POINT('Ctrl Pts',(-12.2791990428529,-13.9255254978142,
-332.900577988846)) ;
#45087=CARTESIAN_POINT('Ctrl Pts',(-12.3931207798733,-13.8243388091023,
-332.90252310191)) ;
#45088=CARTESIAN_POINT('Ctrl Pts',(-12.4565513528077,-13.7672115766006,
-332.90360613236)) ;
#45089=CARTESIAN_POINT('Ctrl Pts',(-12.730181348142,-13.5173339745886,-332.908283453334)) ;
#45090=CARTESIAN_POINT('Ctrl Pts',(-12.9363182381565,-13.3201916672341,
-332.911821302352)) ;
#45091=CARTESIAN_POINT('Ctrl Pts',(-13.5470356076894,-12.7085686694285,
-332.922469851462)) ;
#45092=CARTESIAN_POINT('Ctrl Pts',(-13.9368401105088,-12.2798363346107,
-332.92950785098)) ;
#45093=CARTESIAN_POINT('Ctrl Pts',(-14.4074314911705,-11.7109247399394,
-332.938636336359)) ;
#45094=CARTESIAN_POINT('Ctrl Pts',(-14.5073134754075,-11.5869623323296,
-332.940612580873)) ;
#45095=CARTESIAN_POINT('Ctrl Pts',(-14.7467130345622,-11.281897454798,-332.945452887256)) ;
#45096=CARTESIAN_POINT('Ctrl Pts',(-14.8845036534993,-11.0994732406175,
-332.948328095774)) ;
#45097=CARTESIAN_POINT('Ctrl Pts',(-15.0982780968702,-10.8053104507544,
-332.952944404618)) ;
#45098=CARTESIAN_POINT('Ctrl Pts',(-15.1764716033163,-10.6952066383531,
-332.954667866966)) ;
#45099=CARTESIAN_POINT('Ctrl Pts',(-15.325601580407,-10.4802886616336,-332.958024926894)) ;
#45100=CARTESIAN_POINT('Ctrl Pts',(-15.3966812991223,-10.3755828343112,
-332.95965726923)) ;
#45101=CARTESIAN_POINT('Ctrl Pts',(-15.549816115602,-10.1449643941507,-332.963246173694)) ;
#45102=CARTESIAN_POINT('Ctrl Pts',(-15.6314241046803,-10.0187656005502,
-332.965206015731)) ;
#45103=CARTESIAN_POINT('Ctrl Pts',(-15.9520549379486,-9.50948566049929,
-332.973097945853)) ;
#45104=CARTESIAN_POINT('Ctrl Pts',(-16.1785990612862,-9.11873371953784,
-332.979118948172)) ;
#45105=CARTESIAN_POINT('Ctrl Pts',(-16.6142149381398,-8.29993282078138,
-332.991579490287)) ;
#45106=CARTESIAN_POINT('Ctrl Pts',(-16.8215181447942,-7.87131182849796,
-332.998019712317)) ;
#45107=CARTESIAN_POINT('Ctrl Pts',(-17.0783009664027,-7.28377947165542,
-333.006585977831)) ;
#45108=CARTESIAN_POINT('Ctrl Pts',(-17.1424553603454,-7.13148172756422,
-333.008782922735)) ;
#45109=CARTESIAN_POINT('Ctrl Pts',(-17.2513534187016,-6.86300212038146,
-333.012603428887)) ;
#45110=CARTESIAN_POINT('Ctrl Pts',(-17.296977672553,-6.74718877406822,-333.014234588078)) ;
#45111=CARTESIAN_POINT('Ctrl Pts',(-17.3667602501668,-6.56469087141144,
-333.016773751578)) ;
#45112=CARTESIAN_POINT('Ctrl Pts',(-17.3917069630018,-6.4983118390143,-333.017690876499)) ;
#45113=CARTESIAN_POINT('Ctrl Pts',(-17.4378935300134,-6.37324592913827,
-333.019405647015)) ;
#45114=CARTESIAN_POINT('Ctrl Pts',(-17.4592189398208,-6.31459170973239,
-333.02020443272)) ;
#45115=CARTESIAN_POINT('Ctrl Pts',(-17.5191764854918,-6.14705636966585,
-333.022471991032)) ;
#45116=CARTESIAN_POINT('Ctrl Pts',(-17.557088652206,-6.03792057438868,-333.023932300637)) ;
#45117=CARTESIAN_POINT('Ctrl Pts',(-17.7367135743688,-5.50484301195917,
-333.030997981614)) ;
#45118=CARTESIAN_POINT('Ctrl Pts',(-17.8641034620573,-5.0762303525688,-333.036476400351)) ;
#45119=CARTESIAN_POINT('Ctrl Pts',(-17.979978128308,-4.62765078362187,-333.042151636226)) ;
#45120=CARTESIAN_POINT('Ctrl Pts',(-17.9840353998729,-4.61185819444987,
-333.042351358)) ;
#45121=CARTESIAN_POINT('Ctrl Pts',(-18.0936516372944,-4.18284189887237,
-333.047774940359)) ;
#45122=CARTESIAN_POINT('Ctrl Pts',(-18.1849614602823,-3.76610836205566,
-333.052996460066)) ;
#45123=CARTESIAN_POINT('Ctrl Pts',(-18.3130614144305,-3.06708856862826,
-333.061816050813)) ;
#45124=CARTESIAN_POINT('Ctrl Pts',(-18.3578598786626,-2.7864369451825,-333.065372402138)) ;
#45125=CARTESIAN_POINT('Ctrl Pts',(-18.415659413607,-2.36194687002244,-333.070795778185)) ;
#45126=CARTESIAN_POINT('Ctrl Pts',(-18.4334536911952,-2.21880363980699,
-333.072632023555)) ;
#45127=CARTESIAN_POINT('Ctrl Pts',(-18.4634698061982,-1.95197961470612,
-333.076070496639)) ;
#45128=CARTESIAN_POINT('Ctrl Pts',(-18.476121313219,-1.82835523589385,-333.077669824517)) ;
#45129=CARTESIAN_POINT('Ctrl Pts',(-18.502147401213,-1.54608704770923,-333.08133637996)) ;
#45130=CARTESIAN_POINT('Ctrl Pts',(-18.5147244500455,-1.3873795616715,-333.083408633878)) ;
#45131=CARTESIAN_POINT('Ctrl Pts',(-18.5498716322094,-0.857387975054706,
-333.090363986786)) ;
#45132=CARTESIAN_POINT('Ctrl Pts',(-18.5633254564996,-0.485590909472479,
-333.095302554508)) ;
#45133=CARTESIAN_POINT('Ctrl Pts',(-18.5689934955609,0.440391615893321,
-333.107700349429)) ;
#45134=CARTESIAN_POINT('Ctrl Pts',(-18.5475829596294,0.994298371991139,
-333.115208955269)) ;
#45135=CARTESIAN_POINT('Ctrl Pts',(-18.4908309556074,1.67328353686872,-333.124322660921)) ;
#45136=CARTESIAN_POINT('Ctrl Pts',(-18.4789222552042,1.80003876600416,-333.126019659971)) ;
#45137=CARTESIAN_POINT('Ctrl Pts',(-18.4490094526925,2.08673217205175,-333.129841518427)) ;
#45138=CARTESIAN_POINT('Ctrl Pts',(-18.4302274354707,2.24657912593199,-333.131960848237)) ;
#45139=CARTESIAN_POINT('Ctrl Pts',(-18.3993055249026,2.48316042006527,-333.135070844765)) ;
#45140=CARTESIAN_POINT('Ctrl Pts',(-18.3887585787039,2.56009519873291,-333.136077983377)) ;
#45141=CARTESIAN_POINT('Ctrl Pts',(-18.3682984900442,2.70268732811283,-333.137935355076)) ;
#45142=CARTESIAN_POINT('Ctrl Pts',(-18.3585152092227,2.76836188310839,-333.13878700645)) ;
#45143=CARTESIAN_POINT('Ctrl Pts',(-18.3353135440008,2.9185790970442,-333.140727267773)) ;
#45144=CARTESIAN_POINT('Ctrl Pts',(-18.3216623492075,3.00308432966621,-333.141813237655)) ;
#45145=CARTESIAN_POINT('Ctrl Pts',(-18.2587679154238,3.37601977232114,-333.146586721839)) ;
#45146=CARTESIAN_POINT('Ctrl Pts',(-18.2032944417357,3.66335740573778,-333.150214663096)) ;
#45147=CARTESIAN_POINT('Ctrl Pts',(-18.019125931765,4.50934051785376,-333.160877124651)) ;
#45148=CARTESIAN_POINT('Ctrl Pts',(-17.8713268841018,5.0634699376241,-333.167844748277)) ;
#45149=CARTESIAN_POINT('Ctrl Pts',(-17.6502601443748,5.76089538616308,-333.176891397168)) ;
#45150=CARTESIAN_POINT('Ctrl Pts',(-17.6004586124387,5.91129895829353,-333.178858404637)) ;
#45151=CARTESIAN_POINT('Ctrl Pts',(-17.4743482121151,6.27643035666174,-333.183680555006)) ;
#45152=CARTESIAN_POINT('Ctrl Pts',(-17.3959993431832,6.49042602919687,-333.186546825843)) ;
#45153=CARTESIAN_POINT('Ctrl Pts',(-17.2650232031959,6.82873889115415,-333.191152491203)) ;
#45154=CARTESIAN_POINT('Ctrl Pts',(-17.2149450666118,6.95401807158209,-333.192874399146)) ;
#45155=CARTESIAN_POINT('Ctrl Pts',(-17.1152335539942,7.19578413442279,-333.196230689402)) ;
#45156=CARTESIAN_POINT('Ctrl Pts',(-17.0657652073416,7.3123311433941,-333.197863842168)) ;
#45157=CARTESIAN_POINT('Ctrl Pts',(-16.9548674376392,7.56634910408699,-333.201457295405)) ;
#45158=CARTESIAN_POINT('Ctrl Pts',(-16.8929499640735,7.70359721267887,-333.203420911174)) ;
#45159=CARTESIAN_POINT('Ctrl Pts',(-16.6372681660222,8.2524392288631,-333.211361418898)) ;
#45160=CARTESIAN_POINT('Ctrl Pts',(-16.4300759095894,8.65760063636187,-333.21742869212)) ;
#45161=CARTESIAN_POINT('Ctrl Pts',(-15.9776498207253,9.46745464102918,-333.229893271224)) ;
#45162=CARTESIAN_POINT('Ctrl Pts',(-15.7314075543493,9.87121103609941,-333.236289759675)) ;
#45163=CARTESIAN_POINT('Ctrl Pts',(-15.378933915341,10.4024051829712,-333.244806148928)) ;
#45164=CARTESIAN_POINT('Ctrl Pts',(-15.2860201891735,10.5384642552784,-333.246996299036)) ;
#45165=CARTESIAN_POINT('Ctrl Pts',(-15.1199049341371,10.7748967892186,-333.250806473477)) ;
#45166=CARTESIAN_POINT('Ctrl Pts',(-15.0474839179221,10.8758058943466,-333.2524340421)) ;
#45167=CARTESIAN_POINT('Ctrl Pts',(-14.932164897378,11.0331306448998,-333.254968956818)) ;
#45168=CARTESIAN_POINT('Ctrl Pts',(-14.8899471862556,11.0900402686853,-333.255885375728)) ;
#45169=CARTESIAN_POINT('Ctrl Pts',(-14.8099120409585,11.1966470185692,-333.257599909561)) ;
#45170=CARTESIAN_POINT('Ctrl Pts',(-14.7721676515203,11.2463977346799,-333.258399154765)) ;
#45171=CARTESIAN_POINT('Ctrl Pts',(-14.6637467701677,11.3878193072035,-333.260669949941)) ;
#45172=CARTESIAN_POINT('Ctrl Pts',(-14.5924629520732,11.4790209934549,-333.262132998586)) ;
#45173=CARTESIAN_POINT('Ctrl Pts',(-14.3783186347003,11.7477822063117,-333.266449164744)) ;
#45174=CARTESIAN_POINT('Ctrl Pts',(-14.2330366047752,11.9233847062325,-333.269275648092)) ;
#45175=CARTESIAN_POINT('Ctrl Pts',(-13.7002330261233,12.5437663859952,-333.279358226079)) ;
#45176=CARTESIAN_POINT('Ctrl Pts',(-13.294798738075,12.9726939444986,-333.286523635674)) ;
#45177=CARTESIAN_POINT('Ctrl Pts',(-12.753927095584,13.4928727350859,-333.295799978066)) ;
#45178=CARTESIAN_POINT('Ctrl Pts',(-12.6367812814632,13.6026478957221,-333.297792572643)) ;
#45179=CARTESIAN_POINT('Ctrl Pts',(-12.3484618773211,13.865887384913,-333.302664959189)) ;
#45180=CARTESIAN_POINT('Ctrl Pts',(-12.1758333134102,14.0177183076487,-333.305555929677)) ;
#45181=CARTESIAN_POINT('Ctrl Pts',(-11.8972193203939,14.2537352478201,-333.310191008007)) ;
#45182=CARTESIAN_POINT('Ctrl Pts',(-11.7930561523791,14.3400356552821,-333.311917209591)) ;
#45183=CARTESIAN_POINT('Ctrl Pts',(-11.5897113876162,14.5047950338148,-333.315275659948)) ;
#45184=CARTESIAN_POINT('Ctrl Pts',(-11.4906528442039,14.583394192752,-333.316906608506)) ;
#45185=CARTESIAN_POINT('Ctrl Pts',(-11.2502951582311,14.7701393510807,-333.320852365073)) ;
#45186=CARTESIAN_POINT('Ctrl Pts',(-11.1082293152159,14.8772779409375,-333.323175125279)) ;
#45187=CARTESIAN_POINT('Ctrl Pts',(-10.42546366122,15.3769511933369,-333.334291737183)) ;
#45188=CARTESIAN_POINT('Ctrl Pts',(-9.86537549259348,15.7421498024099,-333.343294375837)) ;
#45189=CARTESIAN_POINT('Ctrl Pts',(-9.02511469636042,16.2275430629978,-333.356361744373)) ;
#45190=CARTESIAN_POINT('Ctrl Pts',(-8.75974936913429,16.3723132289215,-333.360425239304)) ;
#45191=CARTESIAN_POINT('Ctrl Pts',(-8.32564814620522,16.5955608989263,-333.366916336885)) ;
#45192=CARTESIAN_POINT('Ctrl Pts',(-8.15906000204271,16.6780933772944,-333.369370995283)) ;
#45193=CARTESIAN_POINT('Ctrl Pts',(-7.91755207820026,16.7932586717237,-333.372863653351)) ;
#45194=CARTESIAN_POINT('Ctrl Pts',(-7.84361264475933,16.8279205022621,-333.373924163669)) ;
#45195=CARTESIAN_POINT('Ctrl Pts',(-7.70932501505491,16.8897954177682,-333.375832735668)) ;
#45196=CARTESIAN_POINT('Ctrl Pts',(-7.649055555295,16.9171756079629,-333.376682821338)) ;
#45197=CARTESIAN_POINT('Ctrl Pts',(-7.50097916736094,16.9834930700749,-333.378756219468)) ;
#45198=CARTESIAN_POINT('Ctrl Pts',(-7.41301404435475,17.0220723810835,-333.379975098996)) ;
#45199=CARTESIAN_POINT('Ctrl Pts',(-7.04182369300143,17.1814441864609,-333.385071949227)) ;
#45200=CARTESIAN_POINT('Ctrl Pts',(-6.75591510037491,17.2958641657077,-333.388885258305)) ;
#45201=CARTESIAN_POINT('Ctrl Pts',(-6.35051256678759,17.4465185807303,-333.39420697231)) ;
#45202=CARTESIAN_POINT('Ctrl Pts',(-6.23329813465139,17.4887396581955,-333.395735679651)) ;
#45203=CARTESIAN_POINT('Ctrl Pts',(-5.66970197980063,17.685363186401,-333.403052330168)) ;
#45204=CARTESIAN_POINT('Ctrl Pts',(-5.21796143599458,17.8238735920603,-333.408820737122)) ;
#45205=CARTESIAN_POINT('Ctrl Pts',(-4.62272552435464,17.9818103159411,-333.416452869909)) ;
#45206=CARTESIAN_POINT('Ctrl Pts',(-4.48359671517524,18.0170045776417,-333.41823855001)) ;
#45207=CARTESIAN_POINT('Ctrl Pts',(-4.13678870436674,18.1004677943033,-333.422699542089)) ;
#45208=CARTESIAN_POINT('Ctrl Pts',(-3.92865980879362,18.146778971393,-333.42538551301)) ;
#45209=CARTESIAN_POINT('Ctrl Pts',(-3.59012837434456,18.2160091717535,-333.429776528879)) ;
#45210=CARTESIAN_POINT('Ctrl Pts',(-3.46019727490057,18.2411361117591,-333.431467031026)) ;
#45211=CARTESIAN_POINT('Ctrl Pts',(-3.20548983433008,18.2875737776433,-333.43479236479)) ;
#45212=CARTESIAN_POINT('Ctrl Pts',(-3.08074211150248,18.3090018225732,-333.43642632485)) ;
#45213=CARTESIAN_POINT('Ctrl Pts',(-2.80152664549176,18.354028504838,-333.440095851601)) ;
#45214=CARTESIAN_POINT('Ctrl Pts',(-2.64696042991937,18.3769560669108,-333.442135621647)) ;
#45215=CARTESIAN_POINT('Ctrl Pts',(-1.79334964999277,18.4925833918664,-333.45344505984)) ;
#45216=CARTESIAN_POINT('Ctrl Pts',(-1.08975279150549,18.547349525349,-333.462956628382)) ;
#45217=CARTESIAN_POINT('Ctrl Pts',(-0.0996556950809554,18.5678723710647,
-333.476287607101)) ;
#45218=CARTESIAN_POINT('Ctrl Pts',(0.18554171743911,18.5672127750281,-333.480117712307)) ;
#45219=CARTESIAN_POINT('Ctrl Pts',(0.649956807699827,18.5554369731698,-333.486290900692)) ;
#45220=CARTESIAN_POINT('Ctrl Pts',(0.829227908166867,18.5482901203723,-333.488658187769)) ;
#45221=CARTESIAN_POINT('Ctrl Pts',(1.08891360215054,18.5341650324675,-333.492051879007)) ;
#45222=CARTESIAN_POINT('Ctrl Pts',(1.16943045096206,18.5292589902646,-333.493099143531)) ;
#45223=CARTESIAN_POINT('Ctrl Pts',(1.31613560772452,18.5193599211075,-333.494996655237)) ;
#45224=CARTESIAN_POINT('Ctrl Pts',(1.38233380571354,18.5145363989898,-333.495848754326)) ;
#45225=CARTESIAN_POINT('Ctrl Pts',(1.54589729654637,18.5017362520058,-333.497944758691)) ;
#45226=CARTESIAN_POINT('Ctrl Pts',(1.64322822103561,18.4933459342484,-333.499183966519)) ;
#45227=CARTESIAN_POINT('Ctrl Pts',(2.06733839139269,18.4534113225673,-333.504556464405)) ;
#45228=CARTESIAN_POINT('Ctrl Pts',(2.39331533652417,18.4139707869471,-333.508616222852)) ;
#45229=CARTESIAN_POINT('Ctrl Pts',(2.77327452358049,18.3577384641806,-333.513337736712)) ;
#45230=CARTESIAN_POINT('Ctrl Pts',(2.82843672518767,18.3493203905691,-333.514022911433)) ;
#45231=CARTESIAN_POINT('Ctrl Pts',(2.89902717831782,18.3382219957264,-333.514899683102)) ;
#45232=CARTESIAN_POINT('Ctrl Pts',(2.91449113222997,18.3357706678868,-333.515091751334)) ;
#45233=CARTESIAN_POINT('Ctrl Pts',(3.41593761832023,18.2556315693196,-333.521320011182)) ;
#45234=CARTESIAN_POINT('Ctrl Pts',(3.89864304961073,18.1586699990293,-333.527324615667)) ;
#45235=CARTESIAN_POINT('Ctrl Pts',(4.58633430475311,17.991844554022,-333.536089917377)) ;
#45236=CARTESIAN_POINT('Ctrl Pts',(4.79484418843973,17.937402315364,-333.538775009016)) ;
#45237=CARTESIAN_POINT('Ctrl Pts',(5.17809607999879,17.8301744667059,-333.543774234244)) ;
#45238=CARTESIAN_POINT('Ctrl Pts',(5.35309862543383,17.7784176878733,-333.546081889967)) ;
#45239=CARTESIAN_POINT('Ctrl Pts',(5.64868210456148,17.686239109797,-333.550026540283)) ;
#45240=CARTESIAN_POINT('Ctrl Pts',(5.76966260925521,17.6471430177341,-333.551654527742)) ;
#45241=CARTESIAN_POINT('Ctrl Pts',(6.00180500329098,17.5694814350065,-333.554805330464)) ;
#45242=CARTESIAN_POINT('Ctrl Pts',(6.11302070434476,17.5310957734354,-333.556326854624)) ;
#45243=CARTESIAN_POINT('Ctrl Pts',(6.4157881906657,17.4233653402193,-333.560502253498)) ;
#45244=CARTESIAN_POINT('Ctrl Pts',(6.60657519515343,17.3519209847571,-333.563170138087)) ;
#45245=CARTESIAN_POINT('Ctrl Pts',(7.09273641182047,17.1606866200038,-333.570060297574)) ;
#45246=CARTESIAN_POINT('Ctrl Pts',(7.38627148474827,17.0364041972363,-333.574309370653)) ;
#45247=CARTESIAN_POINT('Ctrl Pts',(8.14620853083603,16.6913136563169,-333.585504218126)) ;
#45248=CARTESIAN_POINT('Ctrl Pts',(8.60685984457301,16.4585123238381,-333.592491315004)) ;
#45249=CARTESIAN_POINT('Ctrl Pts',(9.20665712865618,16.1233145266273,-333.601677003311)) ;
#45250=CARTESIAN_POINT('Ctrl Pts',(9.35493598143648,16.0377361159052,-333.603954576904)) ;
#45251=CARTESIAN_POINT('Ctrl Pts',(9.61166097353728,15.8847966016328,-333.607897292968)) ;
#45252=CARTESIAN_POINT('Ctrl Pts',(9.72063542347296,15.8183449447465,-333.609570681551)) ;
#45253=CARTESIAN_POINT('Ctrl Pts',(9.88960188788093,15.7129052302107,-333.612159816118)) ;
#45254=CARTESIAN_POINT('Ctrl Pts',(9.9500683670251,15.6746851892984,-333.61308525093)) ;
#45255=CARTESIAN_POINT('Ctrl Pts',(10.0625274449029,15.6026883796109,-333.614803184514)) ;
#45256=CARTESIAN_POINT('Ctrl Pts',(10.114574648318,15.568998777777,-333.61559693542)) ;
#45257=CARTESIAN_POINT('Ctrl Pts',(10.2610659579705,15.4731318847202,-333.617828606163)) ;
#45258=CARTESIAN_POINT('Ctrl Pts',(10.3551122665437,15.4103515508876,-333.619258485455)) ;
#45259=CARTESIAN_POINT('Ctrl Pts',(10.7253450185761,15.1582841852052,-333.624887190084)) ;
#45260=CARTESIAN_POINT('Ctrl Pts',(10.9969634426094,14.9623995799628,-333.629016977603)) ;
#45261=CARTESIAN_POINT('Ctrl Pts',(11.740756916482,14.3947940503471,-333.640503094221)) ;
#45262=CARTESIAN_POINT('Ctrl Pts',(12.2004042197325,14.0073411442073,-333.647819213943)) ;
#45263=CARTESIAN_POINT('Ctrl Pts',(12.8294321369826,13.4226205212189,-333.658504264199)) ;
#45264=CARTESIAN_POINT('Ctrl Pts',(13.0147269504874,13.2430341176597,-333.661740457688)) ;
#45265=CARTESIAN_POINT('Ctrl Pts',(13.2947435777149,12.9600891630984,-333.666785829568)) ;
#45266=CARTESIAN_POINT('Ctrl Pts',(13.3921388852559,12.8594219900997,-333.668570806938)) ;
#45267=CARTESIAN_POINT('Ctrl Pts',(13.5742329689178,12.6668980673108,-333.671967317222)) ;
#45268=CARTESIAN_POINT('Ctrl Pts',(13.6591618763326,12.5752695448711,-333.673576657815)) ;
#45269=CARTESIAN_POINT('Ctrl Pts',(13.8530178108667,12.3618402697478,-333.677309511865)) ;
#45270=CARTESIAN_POINT('Ctrl Pts',(13.9612745899325,12.2394448008588,-333.679438650682)) ;
#45271=CARTESIAN_POINT('Ctrl Pts',(14.3617278444615,11.7744641154123,-333.687483559095)) ;
#45272=CARTESIAN_POINT('Ctrl Pts',(14.6430450139477,11.4227169523423,-333.693485899691)) ;
#45273=CARTESIAN_POINT('Ctrl Pts',(15.1972894421022,10.6755482321547,-333.70598251633)) ;
#45274=CARTESIAN_POINT('Ctrl Pts',(15.4682228352271,10.279057275902,-333.71247876251)) ;
#45275=CARTESIAN_POINT('Ctrl Pts',(15.8505502133089,9.67014254485675,-333.722085091886)) ;
#45276=CARTESIAN_POINT('Ctrl Pts',(15.9736968933091,9.4653371232579,-333.725255353887)) ;
#45277=CARTESIAN_POINT('Ctrl Pts',(16.1370398842255,9.18141023135086,-333.729540547771)) ;
#45278=CARTESIAN_POINT('Ctrl Pts',(16.180673367045,9.10429346415845,-333.730693512643)) ;
#45279=CARTESIAN_POINT('Ctrl Pts',(16.2557201555781,8.96941382747543,-333.732689129548)) ;
#45280=CARTESIAN_POINT('Ctrl Pts',(16.2873816434602,8.91179114438341,-333.733534959612)) ;
#45281=CARTESIAN_POINT('Ctrl Pts',(16.3597272152027,8.77845161932615,-333.735476796217)) ;
#45282=CARTESIAN_POINT('Ctrl Pts',(16.4001928227195,8.70261815746615,-333.736570010765)) ;
#45283=CARTESIAN_POINT('Ctrl Pts',(16.5382760413192,8.43946340826532,-333.74032952922)) ;
#45284=CARTESIAN_POINT('Ctrl Pts',(16.6332226873881,8.25075877571256,-333.742966198425)) ;
#45285=CARTESIAN_POINT('Ctrl Pts',(16.7425142792203,8.02398627156324,-333.746085120462)) ;
#45286=CARTESIAN_POINT('Ctrl Pts',(16.7599803184982,7.98744012816727,-333.746586233416)) ;
#45287=CARTESIAN_POINT('Ctrl Pts',(17.0420250203897,7.3922881940109,-333.754723873783)) ;
#45288=CARTESIAN_POINT('Ctrl Pts',(17.2786657371352,6.82086902301961,-333.762223247522)) ;
#45289=CARTESIAN_POINT('Ctrl Pts',(17.5657830324307,6.01611366258911,-333.772780686972)) ;
#45290=CARTESIAN_POINT('Ctrl Pts',(17.6409432985255,5.79201833904203,-333.775718272788)) ;
#45291=CARTESIAN_POINT('Ctrl Pts',(17.7701980291416,5.38075198599374,-333.781123390985)) ;
#45292=CARTESIAN_POINT('Ctrl Pts',(17.8256641395329,5.19404733675151,-333.783582278872)) ;
#45293=CARTESIAN_POINT('Ctrl Pts',(17.9130052370937,4.88215308761592,-333.787704115441)) ;
#45294=CARTESIAN_POINT('Ctrl Pts',(17.9465296318657,4.75744148791338,-333.789355941754)) ;
#45295=CARTESIAN_POINT('Ctrl Pts',(18.0075871354738,4.52047147742886,-333.792502684003)) ;
#45296=CARTESIAN_POINT('Ctrl Pts',(18.0353783713527,4.40828580979545,-333.793995787677)) ;
#45297=CARTESIAN_POINT('Ctrl Pts',(18.1061322251825,4.11079749109798,-333.797964428802)) ;
#45298=CARTESIAN_POINT('Ctrl Pts',(18.1472976861948,3.92508174182237,-333.800451563522)) ;
#45299=CARTESIAN_POINT('Ctrl Pts',(18.2569187187187,3.39187795202367,-333.807617486295)) ;
#45300=CARTESIAN_POINT('Ctrl Pts',(18.3182952743577,3.04302061328379,-333.812337517632)) ;
#45301=CARTESIAN_POINT('Ctrl Pts',(18.3826886844754,2.60371476109412,-333.818294559685)) ;
#45302=CARTESIAN_POINT('Ctrl Pts',(18.3950751401083,2.51471358404458,-333.819502000797)) ;
#45303=CARTESIAN_POINT('Ctrl Pts',(18.4374616456409,2.19306442715255,-333.823865764763)) ;
#45304=CARTESIAN_POINT('Ctrl Pts',(18.4636980920934,1.95994291975142,-333.827028918595)) ;
#45305=CARTESIAN_POINT('Ctrl Pts',(18.5113566890086,1.44963241527223,-333.833926997681)) ;
#45306=CARTESIAN_POINT('Ctrl Pts',(18.5309848337237,1.17233186742342,-333.837658748359)) ;
#45307=CARTESIAN_POINT('Ctrl Pts',(18.5528889688586,0.718324094432647,-333.843696752568)) ;
#45308=CARTESIAN_POINT('Ctrl Pts',(18.5588816463034,0.541840218410327,-333.846026036718)) ;
#45309=CARTESIAN_POINT('Ctrl Pts',(18.5639343351448,0.285091147960057,-333.84937652137)) ;
#45310=CARTESIAN_POINT('Ctrl Pts',(18.5649928927966,0.204875270651735,-333.850417881275)) ;
#45311=CARTESIAN_POINT('Ctrl Pts',(18.5659777694683,0.0581923424251096,
-333.852310615797)) ;
#45312=CARTESIAN_POINT('Ctrl Pts',(18.5660671239561,-0.00827208619058709,
-333.853163764812)) ;
#45313=CARTESIAN_POINT('Ctrl Pts',(18.5654032119382,-0.173200850197427,
-333.855270567403)) ;
#45314=CARTESIAN_POINT('Ctrl Pts',(18.5642235240493,-0.271661455251548,
-333.85651939813)) ;
#45315=CARTESIAN_POINT('Ctrl Pts',(18.5588104403247,-0.543147194567071,
-333.859943352131)) ;
#45316=CARTESIAN_POINT('Ctrl Pts',(18.5529409609457,-0.71612139748226,-333.862103148148)) ;
#45317=CARTESIAN_POINT('Ctrl Pts',(18.5446545936004,-0.888979980963969,
-333.864249094225)) ;
#45318=CARTESIAN_POINT('Origin',(0.,0.,-315.477129595899)) ;
#45319=CARTESIAN_POINT('',(18.5446545937806,-0.888979977205187,-335.659885874007)) ;
#45320=CARTESIAN_POINT('',(18.5446545935791,-0.888979981409804,-335.363183819487)) ;
#45321=CARTESIAN_POINT('',(18.544654593745,-0.888979977948782,-315.477129595899)) ;
#45322=CARTESIAN_POINT('Ctrl Pts',(18.5446545938163,-0.888979976461604,
-335.659885874007)) ;
#45323=CARTESIAN_POINT('Ctrl Pts',(18.5558655382488,-0.65511296294481,-335.656771309662)) ;
#45324=CARTESIAN_POINT('Ctrl Pts',(18.5626518543671,-0.421047992405619,
-335.653636281598)) ;
#45325=CARTESIAN_POINT('Ctrl Pts',(18.5691905708464,0.22841400672865,-335.644909722255)) ;
#45326=CARTESIAN_POINT('Ctrl Pts',(18.559433775498,0.643761729554131,-335.639295316782)) ;
#45327=CARTESIAN_POINT('Ctrl Pts',(18.5196860659661,1.33984239217039,-335.629952200477)) ;
#45328=CARTESIAN_POINT('Ctrl Pts',(18.4972103671677,1.62085126235232,-335.626199321161)) ;
#45329=CARTESIAN_POINT('Ctrl Pts',(18.4595924780413,1.98626558838669,-335.621385673521)) ;
#45330=CARTESIAN_POINT('Ctrl Pts',(18.4502523234525,2.07123023127707,-335.62027117357)) ;
#45331=CARTESIAN_POINT('Ctrl Pts',(18.4325412217626,2.2227048070847,-335.618294546381)) ;
#45332=CARTESIAN_POINT('Ctrl Pts',(18.424396177365,2.28923963158799,-335.617429921525)) ;
#45333=CARTESIAN_POINT('Ctrl Pts',(18.4059860957794,2.43316027776215,-335.615568223306)) ;
#45334=CARTESIAN_POINT('Ctrl Pts',(18.3955929734265,2.51052828573006,-335.61457257593)) ;
#45335=CARTESIAN_POINT('Ctrl Pts',(18.3619438296115,2.74958192623614,-335.611509233963)) ;
#45336=CARTESIAN_POINT('Ctrl Pts',(18.3370416815569,2.91102808233788,-335.609458813545)) ;
#45337=CARTESIAN_POINT('Ctrl Pts',(18.2265312578581,3.56967555917701,-335.601136108231)) ;
#45338=CARTESIAN_POINT('Ctrl Pts',(18.1228043386915,4.06361789820827,-335.594988014203)) ;
#45339=CARTESIAN_POINT('Ctrl Pts',(17.8809329799853,5.01985117940733,-335.582896268257)) ;
#45340=CARTESIAN_POINT('Ctrl Pts',(17.7446363797407,5.48220289712154,-335.576960508905)) ;
#45341=CARTESIAN_POINT('Ctrl Pts',(17.5311915306416,6.1144265329805,-335.568582205502)) ;
#45342=CARTESIAN_POINT('Ctrl Pts',(17.4692446813531,6.28922717182213,-335.566238104824)) ;
#45343=CARTESIAN_POINT('Ctrl Pts',(17.3607101571914,6.58150462643401,-335.56226712302)) ;
#45344=CARTESIAN_POINT('Ctrl Pts',(17.3155229509453,6.69948693496976,-335.560649911528)) ;
#45345=CARTESIAN_POINT('Ctrl Pts',(17.2204068538475,6.94043941225237,-335.557316755067)) ;
#45346=CARTESIAN_POINT('Ctrl Pts',(17.1703565000958,7.06335395152022,-335.555600038281)) ;
#45347=CARTESIAN_POINT('Ctrl Pts',(17.0356488639269,7.38427637217871,-335.551074142481)) ;
#45348=CARTESIAN_POINT('Ctrl Pts',(16.9488570667261,7.5813662116102,-335.54825046295)) ;
#45349=CARTESIAN_POINT('Ctrl Pts',(16.7441215859397,8.02518888920079,-335.54179452227)) ;
#45350=CARTESIAN_POINT('Ctrl Pts',(16.6241156399017,8.27091549792316,-335.538150198102)) ;
#45351=CARTESIAN_POINT('Ctrl Pts',(16.3379890561044,8.82538800520952,-335.529788190633)) ;
#45352=CARTESIAN_POINT('Ctrl Pts',(16.1684627333268,9.13225998066787,-335.525058628138)) ;
#45353=CARTESIAN_POINT('Ctrl Pts',(15.9424352510938,9.51536387211735,-335.519071482091)) ;
#45354=CARTESIAN_POINT('Ctrl Pts',(15.8939008025664,9.5962132448198,-335.517803280702)) ;
#45355=CARTESIAN_POINT('Ctrl Pts',(15.6768002161025,9.95169691647751,-335.512210655861)) ;
#45356=CARTESIAN_POINT('Ctrl Pts',(15.5017163214388,10.2222858679354,-335.507908830672)) ;
#45357=CARTESIAN_POINT('Ctrl Pts',(15.2644308799062,10.5688795005813,-335.50240034878)) ;
#45358=CARTESIAN_POINT('Ctrl Pts',(15.20854611416,10.649140299531,-335.501124952734)) ;
#45359=CARTESIAN_POINT('Ctrl Pts',(15.1136665873926,10.7831344580485,-335.498998605056)) ;
#45360=CARTESIAN_POINT('Ctrl Pts',(15.0750131059346,10.8371069177214,-335.498142997565)) ;
#45361=CARTESIAN_POINT('Ctrl Pts',(14.9887891621417,10.9561487569534,-335.496258356927)) ;
#45362=CARTESIAN_POINT('Ctrl Pts',(14.9410828507015,11.0211178835974,-335.495231205263)) ;
#45363=CARTESIAN_POINT('Ctrl Pts',(14.7860737756539,11.2293616290605,-335.491940178135)) ;
#45364=CARTESIAN_POINT('Ctrl Pts',(14.6771214687123,11.3713959515619,-335.489697394733)) ;
#45365=CARTESIAN_POINT('Ctrl Pts',(14.3899618382606,11.7347442781482,-335.483937552399)) ;
#45366=CARTESIAN_POINT('Ctrl Pts',(14.2086974671388,11.9535827967356,-335.480446036835)) ;
#45367=CARTESIAN_POINT('Ctrl Pts',(13.558506340965,12.7028564887664,-335.468284339736)) ;
#45368=CARTESIAN_POINT('Ctrl Pts',(13.0643282980803,13.2105633057365,-335.459645514416)) ;
#45369=CARTESIAN_POINT('Ctrl Pts',(12.4274883152737,13.7940679745472,-335.448777684871)) ;
#45370=CARTESIAN_POINT('Ctrl Pts',(12.3112858280405,13.8978781934371,-335.446805845125)) ;
#45371=CARTESIAN_POINT('Ctrl Pts',(12.0984187997336,14.0832793655732,-335.443210778725)) ;
#45372=CARTESIAN_POINT('Ctrl Pts',(12.0022008632722,14.1653686689334,-335.441591929667)) ;
#45373=CARTESIAN_POINT('Ctrl Pts',(11.8034882620262,14.3314241162502,-335.438260106764)) ;
#45374=CARTESIAN_POINT('Ctrl Pts',(11.7009183955691,14.4152891400008,-335.436546410105)) ;
#45375=CARTESIAN_POINT('Ctrl Pts',(11.4302922572453,14.6317717677516,-335.432040264131)) ;
#45376=CARTESIAN_POINT('Ctrl Pts',(11.260824703532,14.7625930275574,-335.42923355503)) ;
#45377=CARTESIAN_POINT('Ctrl Pts',(10.9733449157868,14.9766833149813,-335.424499816349)) ;
#45378=CARTESIAN_POINT('Ctrl Pts',(10.8565550136431,15.0615588479245,-335.42258414024)) ;
#45379=CARTESIAN_POINT('Ctrl Pts',(10.3492663821095,15.4212578778579,-335.414300041746)) ;
#45380=CARTESIAN_POINT('Ctrl Pts',(9.94923571986067,15.6823217775779,-335.407855243476)) ;
#45381=CARTESIAN_POINT('Ctrl Pts',(9.35949150821033,16.0355382770163,-335.398601761999)) ;
#45382=CARTESIAN_POINT('Ctrl Pts',(9.17757834366956,16.1403415386339,-335.395780765775)) ;
#45383=CARTESIAN_POINT('Ctrl Pts',(8.79300287415107,16.3532978103023,-335.389909769287)) ;
#45384=CARTESIAN_POINT('Ctrl Pts',(8.59003108939005,16.4608206069525,-335.386863655496)) ;
#45385=CARTESIAN_POINT('Ctrl Pts',(8.31295942105643,16.6010766490952,-335.382799862364)) ;
#45386=CARTESIAN_POINT('Ctrl Pts',(8.24056431016954,16.6371313668731,-335.381746648795)) ;
#45387=CARTESIAN_POINT('Ctrl Pts',(8.10845978946807,16.7018491679338,-335.379841947244)) ;
#45388=CARTESIAN_POINT('Ctrl Pts',(8.04882822793687,16.7306679476897,-335.378988565922)) ;
#45389=CARTESIAN_POINT('Ctrl Pts',(7.91551299361442,16.7942189105125,-335.377095389019)) ;
#45390=CARTESIAN_POINT('Ctrl Pts',(7.84175251613057,16.8287864169338,-335.376057624167)) ;
#45391=CARTESIAN_POINT('Ctrl Pts',(7.60013399321661,16.9400863705023,-335.372686260311)) ;
#45392=CARTESIAN_POINT('Ctrl Pts',(7.43135868727245,17.0148015337243,-335.370375190869)) ;
#45393=CARTESIAN_POINT('Ctrl Pts',(6.98662777341595,17.2037998721767,-335.364369308555)) ;
#45394=CARTESIAN_POINT('Ctrl Pts',(6.7089792487783,17.3139624459942,-335.360702682872)) ;
#45395=CARTESIAN_POINT('Ctrl Pts',(5.79613710197483,17.6508945495868,-335.348778546037)) ;
#45396=CARTESIAN_POINT('Ctrl Pts',(5.1512265327555,17.8497660523533,-335.340539495933)) ;
#45397=CARTESIAN_POINT('Ctrl Pts',(4.32462111604155,18.0561261845534,-335.329828447429)) ;
#45398=CARTESIAN_POINT('Ctrl Pts',(4.15170295482127,18.0966682852616,-335.327581051997)) ;
#45399=CARTESIAN_POINT('Ctrl Pts',(3.85476386808479,18.1618080706447,-335.323706129004)) ;
#45400=CARTESIAN_POINT('Ctrl Pts',(3.73102448906178,18.1876313213735,-335.322086797838)) ;
#45401=CARTESIAN_POINT('Ctrl Pts',(3.47423462310636,18.2384900652559,-335.318715842315)) ;
#45402=CARTESIAN_POINT('Ctrl Pts',(3.34115451005407,18.2633379356204,-335.316963084381)) ;
#45403=CARTESIAN_POINT('Ctrl Pts',(2.98076800916878,18.3265560850992,-335.312200588201)) ;
#45404=CARTESIAN_POINT('Ctrl Pts',(2.75299966168767,18.3621520639727,-335.309173350557)) ;
#45405=CARTESIAN_POINT('Ctrl Pts',(2.36492155502531,18.4154183256899,-335.303990071552)) ;
#45406=CARTESIAN_POINT('Ctrl Pts',(2.20493652800374,18.435258091332,-335.3018460589)) ;
#45407=CARTESIAN_POINT('Ctrl Pts',(1.4529934456604,18.5185782699569,-335.291744006921)) ;
#45408=CARTESIAN_POINT('Ctrl Pts',(0.858463657234613,18.5556452041077,-335.283672015171)) ;
#45409=CARTESIAN_POINT('Ctrl Pts',(0.0836350694795375,18.5666299792394,
-335.273297028593)) ;
#45410=CARTESIAN_POINT('Ctrl Pts',(-0.0959413081253097,18.5665704699472,
-335.27090368709)) ;
#45411=CARTESIAN_POINT('Ctrl Pts',(-0.414857152040541,18.5618377539163,
-335.266687483408)) ;
#45412=CARTESIAN_POINT('Ctrl Pts',(-0.554198145662138,18.5582001222467,
-335.264856968614)) ;
#45413=CARTESIAN_POINT('Ctrl Pts',(-0.767221322165178,18.5502376123155,
-335.262082794278)) ;
#45414=CARTESIAN_POINT('Ctrl Pts',(-0.840940534724422,18.5470418953215,
-335.261127219382)) ;
#45415=CARTESIAN_POINT('Ctrl Pts',(-0.983553431257418,18.5400076276155,
-335.259288563337)) ;
#45416=CARTESIAN_POINT('Ctrl Pts',(-1.05244855549534,18.5362243247583,-335.258404918397)) ;
#45417=CARTESIAN_POINT('Ctrl Pts',(-1.23556842475216,18.5251442729891,-335.256066790827)) ;
#45418=CARTESIAN_POINT('Ctrl Pts',(-1.34974964382732,18.5171751524668,-335.254619781902)) ;
#45419=CARTESIAN_POINT('Ctrl Pts',(-1.5414543799913,18.5020128071182,-335.252203800741)) ;
#45420=CARTESIAN_POINT('Ctrl Pts',(-1.61901946611997,18.495386870883,-335.251229994438)) ;
#45421=CARTESIAN_POINT('Ctrl Pts',(-1.82368492970421,18.4766061406513,-335.248668034141)) ;
#45422=CARTESIAN_POINT('Ctrl Pts',(-1.95070560465792,18.4636277283922,-335.247085699949)) ;
#45423=CARTESIAN_POINT('Ctrl Pts',(-2.63157552302649,18.3869548869227,-335.238626109414)) ;
#45424=CARTESIAN_POINT('Ctrl Pts',(-3.18247789605013,18.299648514517,-335.23185117434)) ;
#45425=CARTESIAN_POINT('Ctrl Pts',(-4.08843821929149,18.1139196799848,-335.220450284611)) ;
#45426=CARTESIAN_POINT('Ctrl Pts',(-4.44599185360067,18.0294916404773,-335.21588451051)) ;
#45427=CARTESIAN_POINT('Ctrl Pts',(-4.95471813663165,17.8933131202418,-335.209241017136)) ;
#45428=CARTESIAN_POINT('Ctrl Pts',(-5.10809469044629,17.8501331861639,-335.207218878031)) ;
#45429=CARTESIAN_POINT('Ctrl Pts',(-5.38007940568743,17.7697689839347,-335.203595962243)) ;
#45430=CARTESIAN_POINT('Ctrl Pts',(-5.4989058594434,17.7333577884122,-335.20200047228)) ;
#45431=CARTESIAN_POINT('Ctrl Pts',(-5.75475111258785,17.6521420286851,-335.198536927407)) ;
#45432=CARTESIAN_POINT('Ctrl Pts',(-5.89163180330693,17.6069291241693,-335.19666619085)) ;
#45433=CARTESIAN_POINT('Ctrl Pts',(-6.29618725340927,17.4680549051085,-335.191084321221)) ;
#45434=CARTESIAN_POINT('Ctrl Pts',(-6.5622573393476,17.3698501478164,-335.187343483541)) ;
#45435=CARTESIAN_POINT('Ctrl Pts',(-7.22112320227258,17.109366688551,-335.177919699912)) ;
#45436=CARTESIAN_POINT('Ctrl Pts',(-7.6107932800005,16.9396243556441,-335.172198915819)) ;
#45437=CARTESIAN_POINT('Ctrl Pts',(-8.02955406953755,16.7398413084959,-335.165948881032)) ;
#45438=CARTESIAN_POINT('Ctrl Pts',(-8.0647602298304,16.7229084798281,-335.165422651895)) ;
#45439=CARTESIAN_POINT('Ctrl Pts',(-8.48364630451576,16.5198097059098,-335.159153009936)) ;
#45440=CARTESIAN_POINT('Ctrl Pts',(-8.86085608479542,16.3205881570122,-335.153418610567)) ;
#45441=CARTESIAN_POINT('Ctrl Pts',(-9.33122703995194,16.0510460713502,-335.146281354338)) ;
#45442=CARTESIAN_POINT('Ctrl Pts',(-9.43104407875029,15.9926009674279,-335.144767770698)) ;
#45443=CARTESIAN_POINT('Ctrl Pts',(-9.58388844362059,15.9011785601962,-335.142455480551)) ;
#45444=CARTESIAN_POINT('Ctrl Pts',(-9.6373063933843,15.8688601605454,-335.141648379132)) ;
#45445=CARTESIAN_POINT('Ctrl Pts',(-9.75101834568968,15.7992773400052,-335.139933364301)) ;
#45446=CARTESIAN_POINT('Ctrl Pts',(-9.8112640393381,15.7619358331698,-335.139026610432)) ;
#45447=CARTESIAN_POINT('Ctrl Pts',(-9.97657591044811,15.6581571388878,-335.136541739612)) ;
#45448=CARTESIAN_POINT('Ctrl Pts',(-10.0811910610357,15.5910082659753,-335.134972829174)) ;
#45449=CARTESIAN_POINT('Ctrl Pts',(-10.3230319520279,15.4323270170347,-335.131345873768)) ;
#45450=CARTESIAN_POINT('Ctrl Pts',(-10.4597280422189,15.3400063640323,-335.12929571719)) ;
#45451=CARTESIAN_POINT('Ctrl Pts',(-10.9843970389093,14.9753857842908,-335.121395976615)) ;
#45452=CARTESIAN_POINT('Ctrl Pts',(-11.3631175357686,14.6900891316423,-335.115623071099)) ;
#45453=CARTESIAN_POINT('Ctrl Pts',(-12.0820925289846,14.1040168304179,-335.104232612596)) ;
#45454=CARTESIAN_POINT('Ctrl Pts',(-12.4230581271686,13.8046324143305,-335.098622990248)) ;
#45455=CARTESIAN_POINT('Ctrl Pts',(-12.8620620501793,13.3897160660976,-335.091014365331)) ;
#45456=CARTESIAN_POINT('Ctrl Pts',(-12.9701478705579,13.2850442469859,-335.08910852522)) ;
#45457=CARTESIAN_POINT('Ctrl Pts',(-13.1668064692589,13.0899095015855,-335.085577679936)) ;
#45458=CARTESIAN_POINT('Ctrl Pts',(-13.2557492799914,12.9998320885681,-335.083956195253)) ;
#45459=CARTESIAN_POINT('Ctrl Pts',(-13.4376021828007,12.8118523866817,-335.08058859985)) ;
#45460=CARTESIAN_POINT('Ctrl Pts',(-13.5303799442115,12.7138323294396,-335.078841438118)) ;
#45461=CARTESIAN_POINT('Ctrl Pts',(-13.7770941940885,12.4474183657497,-335.074115873475)) ;
#45462=CARTESIAN_POINT('Ctrl Pts',(-13.9290089261635,12.2771844671933,-335.071120453631)) ;
#45463=CARTESIAN_POINT('Ctrl Pts',(-14.1812223124025,11.9838484358036,-335.066002867069)) ;
#45464=CARTESIAN_POINT('Ctrl Pts',(-14.283149556353,11.8621805868552,-335.063892643693)) ;
#45465=CARTESIAN_POINT('Ctrl Pts',(-14.7473399079588,11.2934304211647,-335.054093063119)) ;
#45466=CARTESIAN_POINT('Ctrl Pts',(-15.0902541599651,10.8309663600002,-335.04629668586)) ;
#45467=CARTESIAN_POINT('Ctrl Pts',(-15.572861369413,10.1125958711499,-335.034695197299)) ;
#45468=CARTESIAN_POINT('Ctrl Pts',(-15.7289246302337,9.86810706586958,-335.03083221794)) ;
#45469=CARTESIAN_POINT('Ctrl Pts',(-15.9234651211404,9.54699203720604,-335.025912460148)) ;
#45470=CARTESIAN_POINT('Ctrl Pts',(-15.9672285833637,9.47361651199007,-335.02479850755)) ;
#45471=CARTESIAN_POINT('Ctrl Pts',(-16.0444176408969,9.34214397268195,-335.02282253678)) ;
#45472=CARTESIAN_POINT('Ctrl Pts',(-16.0780380431757,9.28416308365611,-335.021958026319)) ;
#45473=CARTESIAN_POINT('Ctrl Pts',(-16.1501484068445,9.15823692815331,-335.020096112132)) ;
#45474=CARTESIAN_POINT('Ctrl Pts',(-16.188525083951,9.09022842527761,-335.019100139213)) ;
#45475=CARTESIAN_POINT('Ctrl Pts',(-16.3059249618025,8.87907900695379,-335.01603451953)) ;
#45476=CARTESIAN_POINT('Ctrl Pts',(-16.3834872810126,8.73513466074679,-335.013982183281)) ;
#45477=CARTESIAN_POINT('Ctrl Pts',(-16.6926791096162,8.14271070656478,-335.005654647406)) ;
#45478=CARTESIAN_POINT('Ctrl Pts',(-16.9078751841561,7.68589828810875,-334.999503654886)) ;
#45479=CARTESIAN_POINT('Ctrl Pts',(-17.291398207944,6.77744314014036,-334.987414932742)) ;
#45480=CARTESIAN_POINT('Ctrl Pts',(-17.4612904415509,6.32688883870352,-334.98148522021)) ;
#45481=CARTESIAN_POINT('Ctrl Pts',(-17.6721185750458,5.69430566333641,-334.973113098637)) ;
#45482=CARTESIAN_POINT('Ctrl Pts',(-17.7281159708373,5.51749906089888,-334.970768878094)) ;
#45483=CARTESIAN_POINT('Ctrl Pts',(-17.8177920233857,5.21888379894125,-334.966797756639)) ;
#45484=CARTESIAN_POINT('Ctrl Pts',(-17.85289293483,5.09751650313552,-334.965180527014)) ;
#45485=CARTESIAN_POINT('Ctrl Pts',(-17.9223189315593,4.84794749321801,-334.961847385857)) ;
#45486=CARTESIAN_POINT('Ctrl Pts',(-17.9565136593231,4.7197169323728,-334.960130703055)) ;
#45487=CARTESIAN_POINT('Ctrl Pts',(-18.0425774792356,4.38249489724143,-334.955605029565)) ;
#45488=CARTESIAN_POINT('Ctrl Pts',(-18.0921906532526,4.172948685534,-334.952781541077)) ;
#45489=CARTESIAN_POINT('Ctrl Pts',(-18.196501377866,3.69548202369461,-334.946326152874)) ;
#45490=CARTESIAN_POINT('Ctrl Pts',(-18.2489477107355,3.42712077750293,-334.942682193463)) ;
#45491=CARTESIAN_POINT('Ctrl Pts',(-18.3550699083316,2.81225764761921,-334.934320091271)) ;
#45492=CARTESIAN_POINT('Ctrl Pts',(-18.4048958466047,2.46519633404073,-334.92959005641)) ;
#45493=CARTESIAN_POINT('Ctrl Pts',(-18.4556281785574,2.02316491890919,-334.923601266693)) ;
#45494=CARTESIAN_POINT('Ctrl Pts',(-18.4656748793322,1.92931568512083,-334.922331896669)) ;
#45495=CARTESIAN_POINT('Ctrl Pts',(-18.5068379991275,1.51496928309236,-334.916741283838)) ;
#45496=CARTESIAN_POINT('Ctrl Pts',(-18.5303291502361,1.19377007003294,-334.91244260925)) ;
#45497=CARTESIAN_POINT('Ctrl Pts',(-18.5500526863247,0.774354243649999,
-334.90693609709)) ;
#45498=CARTESIAN_POINT('Ctrl Pts',(-18.5538771632842,0.676551114338569,
-334.905659668122)) ;
#45499=CARTESIAN_POINT('Ctrl Pts',(-18.558997681759,0.512359922785138,-334.90353217313)) ;
#45500=CARTESIAN_POINT('Ctrl Pts',(-18.5607112821091,0.445986972133665,
-334.902676438815)) ;
#45501=CARTESIAN_POINT('Ctrl Pts',(-18.5637159208321,0.299065403920491,
-334.9007922355)) ;
#45502=CARTESIAN_POINT('Ctrl Pts',(-18.5648388140045,0.218514848972907,
-334.899765640107)) ;
#45503=CARTESIAN_POINT('Ctrl Pts',(-18.5667653923379,-0.040748022389909,
-334.896478769565)) ;
#45504=CARTESIAN_POINT('Ctrl Pts',(-18.5655129890358,-0.219465687027397,
-334.894239513396)) ;
#45505=CARTESIAN_POINT('Ctrl Pts',(-18.555603492766,-0.681459016635274,
-334.888492195916)) ;
#45506=CARTESIAN_POINT('Ctrl Pts',(-18.5430403599362,-0.964604577339727,
-334.885009546554)) ;
#45507=CARTESIAN_POINT('Ctrl Pts',(-18.4763110929399,-1.95557857740714,
-334.872833236993)) ;
#45508=CARTESIAN_POINT('Ctrl Pts',(-18.3880439379573,-2.66048846941545,
-334.864171681887)) ;
#45509=CARTESIAN_POINT('Ctrl Pts',(-18.2314995654853,-3.5115682418143,-334.853282864372)) ;
#45510=CARTESIAN_POINT('Ctrl Pts',(-18.2014436970678,-3.66416909718802,
-334.851314554047)) ;
#45511=CARTESIAN_POINT('Ctrl Pts',(-18.1434893136446,-3.94008561693026,
-334.847723806858)) ;
#45512=CARTESIAN_POINT('Ctrl Pts',(-18.1162417789462,-4.06352838017884,
-334.84610571001)) ;
#45513=CARTESIAN_POINT('Ctrl Pts',(-18.0578364914556,-4.31585686373898,
-334.842773287736)) ;
#45514=CARTESIAN_POINT('Ctrl Pts',(-18.0265543993462,-4.44470647463516,
-334.841058217131)) ;
#45515=CARTESIAN_POINT('Ctrl Pts',(-17.9410222858601,-4.78124381212508,
-334.83654308645)) ;
#45516=CARTESIAN_POINT('Ctrl Pts',(-17.8845460617282,-4.98834491270067,
-334.833728657251)) ;
#45517=CARTESIAN_POINT('Ctrl Pts',(-17.7483517476163,-5.45569150749847,
-334.827299443169)) ;
#45518=CARTESIAN_POINT('Ctrl Pts',(-17.66647659598,-5.71525711241862,-334.823672755528)) ;
#45519=CARTESIAN_POINT('Ctrl Pts',(-17.4656206151431,-6.30639633022794,
-334.815306417608)) ;
#45520=CARTESIAN_POINT('Ctrl Pts',(-17.3428499747142,-6.63657235056142,
-334.810554264224)) ;
#45521=CARTESIAN_POINT('Ctrl Pts',(-17.1719479848504,-7.05899516766195,
-334.804420666509)) ;
#45522=CARTESIAN_POINT('Ctrl Pts',(-17.1323316724229,-7.15460843429407,
-334.803028856265)) ;
#45523=CARTESIAN_POINT('Ctrl Pts',(-16.9686325099822,-7.54053627696221,
-334.797402016748)) ;
#45524=CARTESIAN_POINT('Ctrl Pts',(-16.8379529937919,-7.82799567563168,
-334.793189220597)) ;
#45525=CARTESIAN_POINT('Ctrl Pts',(-16.6576324496975,-8.19921863509387,
-334.787778046712)) ;
#45526=CARTESIAN_POINT('Ctrl Pts',(-16.6145750401886,-8.28612100615992,
-334.786513517972)) ;
#45527=CARTESIAN_POINT('Ctrl Pts',(-16.5409418945252,-8.43185244127477,
-334.784399206381)) ;
#45528=CARTESIAN_POINT('Ctrl Pts',(-16.5107284164295,-8.49086223785387,
-334.783544898425)) ;
#45529=CARTESIAN_POINT('Ctrl Pts',(-16.4428595308351,-8.62168455555351,
-334.781655488455)) ;
#45530=CARTESIAN_POINT('Ctrl Pts',(-16.4050484981966,-8.69341462961981,
-334.780622352302)) ;
#45531=CARTESIAN_POINT('Ctrl Pts',(-16.2807921051508,-8.92543973732067,
-334.777286270285)) ;
#45532=CARTESIAN_POINT('Ctrl Pts',(-16.1924577370712,-9.08471126219075,
-334.7750052168)) ;
#45533=CARTESIAN_POINT('Ctrl Pts',(-16.0251053456448,-9.37625877157221,
-334.77082590501)) ;
#45534=CARTESIAN_POINT('Ctrl Pts',(-15.9467564671573,-9.50890046969323,
-334.768923016434)) ;
#45535=CARTESIAN_POINT('Ctrl Pts',(-15.431169504156,-10.3574719845986,-334.756700645397)) ;
#45536=CARTESIAN_POINT('Ctrl Pts',(-14.9474851005102,-11.0440441628066,
-334.74653650393)) ;
#45537=CARTESIAN_POINT('Ctrl Pts',(-14.3221177228642,-11.8150375761764,
-334.734040774378)) ;
#45538=CARTESIAN_POINT('Ctrl Pts',(-14.2237196057069,-11.9333134326557,
-334.732093130011)) ;
#45539=CARTESIAN_POINT('Ctrl Pts',(-14.0420522173019,-12.1462404230145,
-334.728527603671)) ;
#45540=CARTESIAN_POINT('Ctrl Pts',(-13.9592672232226,-12.2412926370082,
-334.72691384249)) ;
#45541=CARTESIAN_POINT('Ctrl Pts',(-13.7870155784079,-12.4350490611055,
-334.723577507064)) ;
#45542=CARTESIAN_POINT('Ctrl Pts',(-13.6974415680007,-12.533648237426,-334.721854053729)) ;
#45543=CARTESIAN_POINT('Ctrl Pts',(-13.4583883598942,-12.7911640198104,
-334.717284092982)) ;
#45544=CARTESIAN_POINT('Ctrl Pts',(-13.3071559617381,-12.9484243896679,
-334.714422542752)) ;
#45545=CARTESIAN_POINT('Ctrl Pts',(-12.9564530151125,-13.3004710736074,
-334.707856672908)) ;
#45546=CARTESIAN_POINT('Ctrl Pts',(-12.7552959823839,-13.4935032324896,
-334.704139618936)) ;
#45547=CARTESIAN_POINT('Ctrl Pts',(-12.2455972803217,-13.9610287176639,
-334.694866640363)) ;
#45548=CARTESIAN_POINT('Ctrl Pts',(-11.9320996672972,-14.2298971425154,
-334.689287473819)) ;
#45549=CARTESIAN_POINT('Ctrl Pts',(-11.3448073337259,-14.7005185735621,
-334.679175474132)) ;
#45550=CARTESIAN_POINT('Ctrl Pts',(-11.0739338404125,-14.9056328240651,
-334.674635099578)) ;
#45551=CARTESIAN_POINT('Ctrl Pts',(-10.7165473698945,-15.1611356961604,
-334.668871130383)) ;
#45552=CARTESIAN_POINT('Ctrl Pts',(-10.6350442105427,-15.2184183741542,
-334.667571502045)) ;
#45553=CARTESIAN_POINT('Ctrl Pts',(-10.4982836472523,-15.3129022822457,
-334.665418098418)) ;
#45554=CARTESIAN_POINT('Ctrl Pts',(-10.4432800152174,-15.3504670419113,
-334.664559375342)) ;
#45555=CARTESIAN_POINT('Ctrl Pts',(-10.3221067933255,-15.4322696291284,
-334.662684308674)) ;
#45556=CARTESIAN_POINT('Ctrl Pts',(-10.2558525896091,-15.4763794940035,
-334.661669668119)) ;
#45557=CARTESIAN_POINT('Ctrl Pts',(-10.0450017396543,-15.61480845753,-334.658470891547)) ;
#45558=CARTESIAN_POINT('Ctrl Pts',(-9.8993720055007,-15.7075375916401,-334.65630625538)) ;
#45559=CARTESIAN_POINT('Ctrl Pts',(-9.52429504265865,-15.9390780008328,
-334.650819882003)) ;
#45560=CARTESIAN_POINT('Ctrl Pts',(-9.29309489686995,-16.074974064613,-334.647520889701)) ;
#45561=CARTESIAN_POINT('Ctrl Pts',(-8.40423521688958,-16.5718456359355,
-334.635030408914)) ;
#45562=CARTESIAN_POINT('Ctrl Pts',(-7.72785449681234,-16.8978549643495,
-334.625888748716)) ;
#45563=CARTESIAN_POINT('Ctrl Pts',(-6.88167301169118,-17.2442462894622,
-334.614369620857)) ;
#45564=CARTESIAN_POINT('Ctrl Pts',(-6.72891546106093,-17.3044257384822,
-334.61228849112)) ;
#45565=CARTESIAN_POINT('Ctrl Pts',(-6.45846015792787,-17.4068498773485,
-334.608597874609)) ;
#45566=CARTESIAN_POINT('Ctrl Pts',(-6.34109611966826,-17.4499464243691,
-334.606994385402)) ;
#45567=CARTESIAN_POINT('Ctrl Pts',(-6.09172608314385,-17.5386680652489,
-334.603582379403)) ;
#45568=CARTESIAN_POINT('Ctrl Pts',(-5.95962241660026,-17.5839956993332,
-334.601771936799)) ;
#45569=CARTESIAN_POINT('Ctrl Pts',(-5.58436872933906,-17.7080388145836,
-334.596620649977)) ;
#45570=CARTESIAN_POINT('Ctrl Pts',(-5.34008756417781,-17.783230222862,-334.593256884592)) ;
#45571=CARTESIAN_POINT('Ctrl Pts',(-4.91263407461246,-17.9052011509568,
-334.587359444321)) ;
#45572=CARTESIAN_POINT('Ctrl Pts',(-4.73015483795835,-17.9542707145394,
-334.584838398952)) ;
#45573=CARTESIAN_POINT('Ctrl Pts',(-4.20009954116143,-18.0881632902019,
-334.577515640882)) ;
#45574=CARTESIAN_POINT('Ctrl Pts',(-3.8507806160192,-18.1657363087151,-334.572688826933)) ;
#45575=CARTESIAN_POINT('Ctrl Pts',(-3.45144829283486,-18.2423790138929,
-334.567215090276)) ;
#45576=CARTESIAN_POINT('Ctrl Pts',(-3.40342083171717,-18.2514003311451,
-334.566557519119)) ;
#45577=CARTESIAN_POINT('Ctrl Pts',(-3.01805138687179,-18.3222128254613,
-334.561288281021)) ;
#45578=CARTESIAN_POINT('Ctrl Pts',(-2.67909121276421,-18.3748357275041,
-334.556695716192)) ;
#45579=CARTESIAN_POINT('Ctrl Pts',(-2.22616288534428,-18.4323521430718,
-334.55068732171)) ;
#45580=CARTESIAN_POINT('Ctrl Pts',(-2.11332848287763,-18.445629550162,-334.549201166485)) ;
#45581=CARTESIAN_POINT('Ctrl Pts',(-1.93865279246789,-18.4645600991707,
-334.546920611706)) ;
#45582=CARTESIAN_POINT('Ctrl Pts',(-1.87689313665326,-18.4709400538601,
-334.546118166271)) ;
#45583=CARTESIAN_POINT('Ctrl Pts',(-1.74405316600134,-18.4839896854498,
-334.544401391305)) ;
#45584=CARTESIAN_POINT('Ctrl Pts',(-1.67296401224935,-18.4905594174153,
-334.543488314414)) ;
#45585=CARTESIAN_POINT('Ctrl Pts',(-1.47539718496243,-18.5076689483902,
-334.540964417224)) ;
#45586=CARTESIAN_POINT('Ctrl Pts',(-1.3488465631758,-18.5173221548281,-334.539363278067)) ;
#45587=CARTESIAN_POINT('Ctrl Pts',(-1.05274130264155,-18.5368573038878,
-334.535644106933)) ;
#45588=CARTESIAN_POINT('Ctrl Pts',(-0.883130162201162,-18.5457117469981,
-334.533534522364)) ;
#45589=CARTESIAN_POINT('Ctrl Pts',(-0.207385116840132,-18.5716973408216,
-334.525178411999)) ;
#45590=CARTESIAN_POINT('Ctrl Pts',(0.299235767185004,-18.5704445275094,
-334.519016412708)) ;
#45591=CARTESIAN_POINT('Ctrl Pts',(1.17806417954462,-18.532295477931,-334.508199821747)) ;
#45592=CARTESIAN_POINT('Ctrl Pts',(1.55038398504384,-18.5048674568597,-334.503578921506)) ;
#45593=CARTESIAN_POINT('Ctrl Pts',(2.10397535003999,-18.4472599496149,-334.496588216107)) ;
#45594=CARTESIAN_POINT('Ctrl Pts',(2.28603653196849,-18.4255840815446,-334.494270066832)) ;
#45595=CARTESIAN_POINT('Ctrl Pts',(2.59263787521039,-18.3844664490713,-334.490329271862)) ;
#45596=CARTESIAN_POINT('Ctrl Pts',(2.71735532290006,-18.3664465198158,-334.488715938975)) ;
#45597=CARTESIAN_POINT('Ctrl Pts',(2.97358133457003,-18.3267584413797,-334.485379171281)) ;
#45598=CARTESIAN_POINT('Ctrl Pts',(3.10505952347914,-18.3049410328061,-334.483654843658)) ;
#45599=CARTESIAN_POINT('Ctrl Pts',(3.45147480144925,-18.243617406876,-334.479079161555)) ;
#45600=CARTESIAN_POINT('Ctrl Pts',(3.66596865724095,-18.2017287072936,-334.476212693314)) ;
#45601=CARTESIAN_POINT('Ctrl Pts',(4.55125348137117,-18.0125568991946,-334.464250697676)) ;
#45602=CARTESIAN_POINT('Ctrl Pts',(5.21435352797801,-17.8318990944563,-334.454955756248)) ;
#45603=CARTESIAN_POINT('Ctrl Pts',(6.19458890065182,-17.5054727110899,-334.441072156181)) ;
#45604=CARTESIAN_POINT('Ctrl Pts',(6.52013711864472,-17.3868432815609,-334.436441152158)) ;
#45605=CARTESIAN_POINT('Ctrl Pts',(6.93375071595263,-17.2228715481268,-334.430605207607)) ;
#45606=CARTESIAN_POINT('Ctrl Pts',(7.02503548756114,-17.1858395137953,-334.429320355292)) ;
#45607=CARTESIAN_POINT('Ctrl Pts',(7.17741420547475,-17.122606193807,-334.427183483661)) ;
#45608=CARTESIAN_POINT('Ctrl Pts',(7.23866988640693,-17.0968001642626,-334.426326694641)) ;
#45609=CARTESIAN_POINT('Ctrl Pts',(7.37352489145439,-17.0391332470442,-334.424445957889)) ;
#45610=CARTESIAN_POINT('Ctrl Pts',(7.44705888295391,-17.007123365019,-334.423423820469)) ;
#45611=CARTESIAN_POINT('Ctrl Pts',(7.68168683400369,-16.9031746325087,-334.420170073241)) ;
#45612=CARTESIAN_POINT('Ctrl Pts',(7.84196389482282,-16.8294155494729,-334.417958904565)) ;
#45613=CARTESIAN_POINT('Ctrl Pts',(8.25164397890684,-16.6337584629967,-334.412310700348)) ;
#45614=CARTESIAN_POINT('Ctrl Pts',(8.4994085598984,-16.5085312333746,-334.408898047725)) ;
#45615=CARTESIAN_POINT('Ctrl Pts',(9.38142646674977,-16.0376128787603,-334.396638044146)) ;
#45616=CARTESIAN_POINT('Ctrl Pts',(9.99818703630216,-15.6605378311281,-334.387828880518)) ;
#45617=CARTESIAN_POINT('Ctrl Pts',(10.7181128048373,-15.1604867009398,-334.376796449642)) ;
#45618=CARTESIAN_POINT('Ctrl Pts',(10.8437163370719,-15.0709029263927,-334.374843602471)) ;
#45619=CARTESIAN_POINT('Ctrl Pts',(11.0699608966569,-14.9052465804426,-334.371271738166)) ;
#45620=CARTESIAN_POINT('Ctrl Pts',(11.1709710003382,-14.8296937505098,-334.369656896886)) ;
#45621=CARTESIAN_POINT('Ctrl Pts',(11.3769274072928,-14.6723455480637,-334.366321613404)) ;
#45622=CARTESIAN_POINT('Ctrl Pts',(11.4817801608207,-14.5904395200544,-334.364600326314)) ;
#45623=CARTESIAN_POINT('Ctrl Pts',(11.7555052887966,-14.3718403150183,-334.360044538547)) ;
#45624=CARTESIAN_POINT('Ctrl Pts',(11.9228741949506,-14.2332979069273,-334.357195170265)) ;
#45625=CARTESIAN_POINT('Ctrl Pts',(12.2980492562701,-13.9114785004873,-334.350664752019)) ;
#45626=CARTESIAN_POINT('Ctrl Pts',(12.5042617611538,-13.7264229486378,-334.346971186346)) ;
#45627=CARTESIAN_POINT('Ctrl Pts',(12.9582890673179,-13.3002530034025,-334.338623546852)) ;
#45628=CARTESIAN_POINT('Ctrl Pts',(13.2036664901206,-13.0566908680963,-334.333959319758)) ;
#45629=CARTESIAN_POINT('Ctrl Pts',(13.5285869382446,-12.7156421603863,-334.327619265712)) ;
#45630=CARTESIAN_POINT('Ctrl Pts',(13.6141512864416,-12.6239892612005,-334.325933570971)) ;
#45631=CARTESIAN_POINT('Ctrl Pts',(13.8974877698098,-12.314260053083,-334.320304848645)) ;
#45632=CARTESIAN_POINT('Ctrl Pts',(14.0910006784114,-12.0923474755302,-334.316382160305)) ;
#45633=CARTESIAN_POINT('Ctrl Pts',(14.3400293973394,-11.7926726491013,-334.311275575564)) ;
#45634=CARTESIAN_POINT('Ctrl Pts',(14.4003391777056,-11.7189505899678,-334.310034167337)) ;
#45635=CARTESIAN_POINT('Ctrl Pts',(14.501549326356,-11.5932712467783,-334.307945235598)) ;
#45636=CARTESIAN_POINT('Ctrl Pts',(14.5427442106202,-11.5415537048316,-334.307093465033)) ;
#45637=CARTESIAN_POINT('Ctrl Pts',(14.5870205934659,-11.4853541112165,-334.306176508206)) ;
#45638=CARTESIAN_POINT('Ctrl Pts',(14.5903772125746,-11.4810897413541,-334.306106982867)) ;
#45639=CARTESIAN_POINT('Ctrl Pts',(14.5964088578749,-11.4734200048863,-334.305982030865)) ;
#45640=CARTESIAN_POINT('Ctrl Pts',(14.5990845632339,-11.4700151730643,-334.305926593993)) ;
#45641=CARTESIAN_POINT('Ctrl Pts',(14.6032861400707,-11.4646648196558,-334.30583953231)) ;
#45642=CARTESIAN_POINT('Ctrl Pts',(14.6048128144616,-11.462719928986,-334.305807895535)) ;
#45643=CARTESIAN_POINT('Ctrl Pts',(14.6072011058389,-11.4596761387939,-334.305758400167)) ;
#45644=CARTESIAN_POINT('Ctrl Pts',(14.6080629873956,-11.4585774469935,-334.305740537652)) ;
#45645=CARTESIAN_POINT('Ctrl Pts',(14.6107766949918,-11.4551173183529,-334.305684293679)) ;
#45646=CARTESIAN_POINT('Ctrl Pts',(14.6126280725162,-11.4527555296731,-334.305645918852)) ;
#45647=CARTESIAN_POINT('Ctrl Pts',(14.6161587865224,-11.4482491739567,-334.305572728619)) ;
#45648=CARTESIAN_POINT('Ctrl Pts',(14.6178382238301,-11.4461046860393,-334.305537911733)) ;
#45649=CARTESIAN_POINT('Ctrl Pts',(14.621041680062,-11.4420123103101,-334.305471494467)) ;
#45650=CARTESIAN_POINT('Ctrl Pts',(14.6225657817803,-11.4400644874453,-334.305439892879)) ;
#45651=CARTESIAN_POINT('Ctrl Pts',(14.6254735138087,-11.4363468356861,-334.305379597708)) ;
#45652=CARTESIAN_POINT('Ctrl Pts',(14.6268572122201,-11.4345770600644,-334.305350903136)) ;
#45653=CARTESIAN_POINT('Ctrl Pts',(14.684340900627,-11.3610268618028,-334.304158746142)) ;
#45654=CARTESIAN_POINT('Ctrl Pts',(14.7399121766279,-11.2888346651964,-334.303002929337)) ;
#45655=CARTESIAN_POINT('Ctrl Pts',(14.9705546641567,-10.9846021267888,-334.298185627773)) ;
#45656=CARTESIAN_POINT('Ctrl Pts',(15.1406958325475,-10.7488753480212,-334.294581831229)) ;
#45657=CARTESIAN_POINT('Ctrl Pts',(15.7798840102583,-9.81798848822343,-334.280675628014)) ;
#45658=CARTESIAN_POINT('Ctrl Pts',(16.2071584254526,-9.09536462014561,-334.270520559468)) ;
#45659=CARTESIAN_POINT('Ctrl Pts',(16.6627203593302,-8.1901658754324,-334.257774378502)) ;
#45660=CARTESIAN_POINT('Ctrl Pts',(16.7391077518726,-8.03289103494846,-334.255561053074)) ;
#45661=CARTESIAN_POINT('Ctrl Pts',(16.8667074425404,-7.76044828213136,-334.251725240976)) ;
#45662=CARTESIAN_POINT('Ctrl Pts',(16.9189894217914,-7.6457945554539,-334.250110499529)) ;
#45663=CARTESIAN_POINT('Ctrl Pts',(17.0202127641094,-7.41768972438955,-334.246896087154)) ;
#45664=CARTESIAN_POINT('Ctrl Pts',(17.0691968927181,-7.30426456053074,-334.245296819076)) ;
#45665=CARTESIAN_POINT('Ctrl Pts',(17.1382553962219,-7.13986699418179,-334.242977395412)) ;
#45666=CARTESIAN_POINT('Ctrl Pts',(17.1592420671434,-7.08928137385079,-334.24226350844)) ;
#45667=CARTESIAN_POINT('Ctrl Pts',(17.212711257848,-6.95877239973039,-334.240421235097)) ;
#45668=CARTESIAN_POINT('Ctrl Pts',(17.2448610666167,-6.87871419192239,-334.239290670346)) ;
#45669=CARTESIAN_POINT('Ctrl Pts',(17.4618110502084,-6.32739230861528,-334.231502560684)) ;
#45670=CARTESIAN_POINT('Ctrl Pts',(17.6278278810132,-5.84896743316346,-334.224724982449)) ;
#45671=CARTESIAN_POINT('Ctrl Pts',(17.9441733164718,-4.80079921556183,-334.209987094631)) ;
#45672=CARTESIAN_POINT('Ctrl Pts',(18.0873610074677,-4.22946824820636,-334.202019905579)) ;
#45673=CARTESIAN_POINT('Ctrl Pts',(18.2239350176425,-3.54878010385512,-334.192898809154)) ;
#45674=CARTESIAN_POINT('Ctrl Pts',(18.2438224347482,-3.44508211391819,-334.191519659579)) ;
#45675=CARTESIAN_POINT('Ctrl Pts',(18.2748465935001,-3.27550670364407,-334.189284396455)) ;
#45676=CARTESIAN_POINT('Ctrl Pts',(18.2865142331733,-3.20972887036489,-334.188422285293)) ;
#45677=CARTESIAN_POINT('Ctrl Pts',(18.3082225652916,-3.08338367843785,-334.18677659065)) ;
#45678=CARTESIAN_POINT('Ctrl Pts',(18.3183183308969,-3.0228268140341,-334.185992195983)) ;
#45679=CARTESIAN_POINT('Ctrl Pts',(18.3405660872816,-2.88517354228373,-334.184218065884)) ;
#45680=CARTESIAN_POINT('Ctrl Pts',(18.3525326713659,-2.80804831456253,-334.183230369278)) ;
#45681=CARTESIAN_POINT('Ctrl Pts',(18.3825217873611,-2.60638197280485,-334.180661863784)) ;
#45682=CARTESIAN_POINT('Ctrl Pts',(18.3997650965196,-2.48172897547759,-334.179088250415)) ;
#45683=CARTESIAN_POINT('Ctrl Pts',(18.4781203008743,-1.86949986221311,-334.171410388187)) ;
#45684=CARTESIAN_POINT('Ctrl Pts',(18.5211258234318,-1.37980423008815,-334.16542192462)) ;
#45685=CARTESIAN_POINT('Ctrl Pts',(18.5446545951453,-0.888979948736885,
-334.159397110264)) ;
#45686=CARTESIAN_POINT('Ctrl Pts',(18.5446545936004,-0.888979980963982,
-333.864249094225)) ;
#45687=CARTESIAN_POINT('Ctrl Pts',(18.5364060801737,-1.06104890904447,-333.866385237156)) ;
#45688=CARTESIAN_POINT('Ctrl Pts',(18.5257627102001,-1.23300327160291,-333.868507658875)) ;
#45689=CARTESIAN_POINT('Ctrl Pts',(18.4814882950303,-1.81646298999327,-333.875695449156)) ;
#45690=CARTESIAN_POINT('Ctrl Pts',(18.4365268932318,-2.2269763609594,-333.880731733973)) ;
#45691=CARTESIAN_POINT('Ctrl Pts',(18.3385715194033,-2.91000203681898,-333.889225167194)) ;
#45692=CARTESIAN_POINT('Ctrl Pts',(18.2930869448647,-3.18343947944684,-333.892655512125)) ;
#45693=CARTESIAN_POINT('Ctrl Pts',(18.2010477239368,-3.66927628575645,-333.898836146372)) ;
#45694=CARTESIAN_POINT('Ctrl Pts',(18.1568515815253,-3.88206995265725,-333.901572730302)) ;
#45695=CARTESIAN_POINT('Ctrl Pts',(18.0795887957112,-4.22382209790757,-333.906023971289)) ;
#45696=CARTESIAN_POINT('Ctrl Pts',(18.0488531584613,-4.35328654460257,-333.907723280171)) ;
#45697=CARTESIAN_POINT('Ctrl Pts',(17.9862766986735,-4.60480821919209,-333.911051475793)) ;
#45698=CARTESIAN_POINT('Ctrl Pts',(17.9545784001488,-4.72689355032367,-333.912679331906)) ;
#45699=CARTESIAN_POINT('Ctrl Pts',(17.8813572375459,-4.99753470145266,-333.916316100126)) ;
#45700=CARTESIAN_POINT('Ctrl Pts',(17.839222135693,-5.14591520012333,-333.918328958077)) ;
#45701=CARTESIAN_POINT('Ctrl Pts',(17.5891077884254,-5.98668834988175,-333.92984116475)) ;
#45702=CARTESIAN_POINT('Ctrl Pts',(17.3426753624236,-6.66698978674249,-333.939597839374)) ;
#45703=CARTESIAN_POINT('Ctrl Pts',(16.9477440001816,-7.58586302227325,-333.953058411041)) ;
#45704=CARTESIAN_POINT('Ctrl Pts',(16.8325912294537,-7.83806208814005,-333.956779925646)) ;
#45705=CARTESIAN_POINT('Ctrl Pts',(16.6350450904975,-8.2462626987908,-333.962803818454)) ;
#45706=CARTESIAN_POINT('Ctrl Pts',(16.555999424233,-8.40383584517819,-333.965129106194)) ;
#45707=CARTESIAN_POINT('Ctrl Pts',(16.4377552092092,-8.63140377377534,-333.968475041525)) ;
#45708=CARTESIAN_POINT('Ctrl Pts',(16.4003282117755,-8.70230785445617,-333.969515775402)) ;
#45709=CARTESIAN_POINT('Ctrl Pts',(16.3310320130392,-8.83155205022018,-333.971408009307)) ;
#45710=CARTESIAN_POINT('Ctrl Pts',(16.2993065982752,-8.88996752724849,-333.972261275484)) ;
#45711=CARTESIAN_POINT('Ctrl Pts',(16.21977006569,-9.03455978564466,-333.974369250694)) ;
#45712=CARTESIAN_POINT('Ctrl Pts',(16.1715852078454,-9.12052868042802,-333.975619123293)) ;
#45713=CARTESIAN_POINT('Ctrl Pts',(15.9505704565034,-9.50759320205602,-333.981239269331)) ;
#45714=CARTESIAN_POINT('Ctrl Pts',(15.7699999203731,-9.80418941231599,-333.985527043904)) ;
#45715=CARTESIAN_POINT('Ctrl Pts',(15.3567328172156,-10.4420156282245,-333.994862288099)) ;
#45716=CARTESIAN_POINT('Ctrl Pts',(15.1207524438782,-10.7808987995435,-333.999898473163)) ;
#45717=CARTESIAN_POINT('Ctrl Pts',(14.7083882915456,-11.3328760861695,-334.008380103941)) ;
#45718=CARTESIAN_POINT('Ctrl Pts',(14.5381892058658,-11.5504034908375,-334.01179845341)) ;
#45719=CARTESIAN_POINT('Ctrl Pts',(14.2258347592792,-11.9317694944369,-334.017960472686)) ;
#45720=CARTESIAN_POINT('Ctrl Pts',(14.0855411589775,-12.0970669125876,-334.020690573568)) ;
#45721=CARTESIAN_POINT('Ctrl Pts',(13.8545820268105,-12.359722339258,-334.025134098081)) ;
#45722=CARTESIAN_POINT('Ctrl Pts',(13.7657087651635,-12.4586292011734,-334.0268322776)) ;
#45723=CARTESIAN_POINT('Ctrl Pts',(13.5904397072279,-12.6495205586803,-334.030160069561)) ;
#45724=CARTESIAN_POINT('Ctrl Pts',(13.5041533341459,-12.74159583704,-334.03178867142)) ;
#45725=CARTESIAN_POINT('Ctrl Pts',(13.3101520215797,-12.9444281275674,-334.035429476969)) ;
#45726=CARTESIAN_POINT('Ctrl Pts',(13.2019797081778,-13.054734699573,-334.0374456582)) ;
#45727=CARTESIAN_POINT('Ctrl Pts',(12.5791377785212,-13.6742061411934,-334.048975013189)) ;
#45728=CARTESIAN_POINT('Ctrl Pts',(12.0364116004989,-14.1542717207302,-334.058746182979)) ;
#45729=CARTESIAN_POINT('Ctrl Pts',(11.2498704771485,-14.7719724234797,-334.072205681112)) ;
#45730=CARTESIAN_POINT('Ctrl Pts',(11.0289150869606,-14.9376633829717,-334.075912648649)) ;
#45731=CARTESIAN_POINT('Ctrl Pts',(10.661335665571,-15.2007021647557,-334.081916473074)) ;
#45732=CARTESIAN_POINT('Ctrl Pts',(10.516878082963,-15.3010032367193,-334.084236067762)) ;
#45733=CARTESIAN_POINT('Ctrl Pts',(10.3045730284832,-15.4439856051886,-334.087575520522)) ;
#45734=CARTESIAN_POINT('Ctrl Pts',(10.237839822277,-15.4883037311974,-334.088615360916)) ;
#45735=CARTESIAN_POINT('Ctrl Pts',(10.1151976016924,-15.5686125792083,-334.090506882322)) ;
#45736=CARTESIAN_POINT('Ctrl Pts',(10.0593782291162,-15.6047374152743,-334.091360317701)) ;
#45737=CARTESIAN_POINT('Ctrl Pts',(9.9202427214049,-15.6937254854263,-334.093469975944)) ;
#45738=CARTESIAN_POINT('Ctrl Pts',(9.8366969140021,-15.746225869286,-334.094721342886)) ;
#45739=CARTESIAN_POINT('Ctrl Pts',(9.45586571684599,-15.9813273203421,-334.100364446704)) ;
#45740=CARTESIAN_POINT('Ctrl Pts',(9.15388723672968,-16.1561928988392,-334.104672873246)) ;
#45741=CARTESIAN_POINT('Ctrl Pts',(8.38452932051349,-16.573203516772,-334.115421141634)) ;
#45742=CARTESIAN_POINT('Ctrl Pts',(7.91144540126423,-16.8041792044361,-334.121831058525)) ;
#45743=CARTESIAN_POINT('Ctrl Pts',(7.28992739324099,-17.0755541635573,-334.130224751194)) ;
#45744=CARTESIAN_POINT('Ctrl Pts',(7.14992216220353,-17.1346492348249,-334.132113200787)) ;
#45745=CARTESIAN_POINT('Ctrl Pts',(6.80400139234613,-17.275681561107,-334.136779996954)) ;
#45746=CARTESIAN_POINT('Ctrl Pts',(6.59731426680543,-17.3556634145908,-334.139569291856)) ;
#45747=CARTESIAN_POINT('Ctrl Pts',(6.26360490354329,-17.4779764032883,-334.144083288628)) ;
#45748=CARTESIAN_POINT('Ctrl Pts',(6.13747047776568,-17.5226670804847,-334.145791786265)) ;
#45749=CARTESIAN_POINT('Ctrl Pts',(5.89191572122929,-17.6066928738069,-334.149123630426)) ;
#45750=CARTESIAN_POINT('Ctrl Pts',(5.77255712211019,-17.6461862462551,-334.150745786696)) ;
#45751=CARTESIAN_POINT('Ctrl Pts',(5.47998667982631,-17.7397058542262,-334.154728930388)) ;
#45752=CARTESIAN_POINT('Ctrl Pts',(5.3063663907609,-17.7924111176026,-334.157098603147)) ;
#45753=CARTESIAN_POINT('Ctrl Pts',(4.53173775694455,-18.015215177998,-334.167695090417)) ;
#45754=CARTESIAN_POINT('Ctrl Pts',(3.92314529884862,-18.1574654275551,-334.176098800478)) ;
#45755=CARTESIAN_POINT('Ctrl Pts',(2.84082238948169,-18.3534783872777,-334.19091474368)) ;
#45756=CARTESIAN_POINT('Ctrl Pts',(2.37001671250625,-18.4201917146807,-334.19731311006)) ;
#45757=CARTESIAN_POINT('Ctrl Pts',(1.79531814421084,-18.4792265956159,-334.204897777105)) ;
#45758=CARTESIAN_POINT('Ctrl Pts',(1.69338066734606,-18.4888464965266,-334.206234318073)) ;
#45759=CARTESIAN_POINT('Ctrl Pts',(1.5246318301483,-18.5033641256042,-334.208429432628)) ;
#45760=CARTESIAN_POINT('Ctrl Pts',(1.45786426468749,-18.5087443660465,-334.209293400324)) ;
#45761=CARTESIAN_POINT('Ctrl Pts',(1.3130742312624,-18.5196234563505,-334.211156358076)) ;
#45762=CARTESIAN_POINT('Ctrl Pts',(1.23504331076919,-18.5249908217135,-334.212153894217)) ;
#45763=CARTESIAN_POINT('Ctrl Pts',(0.99304677073675,-18.5401007719236,-334.215230472338)) ;
#45764=CARTESIAN_POINT('Ctrl Pts',(0.828983915114168,-18.5481606729392,
-334.217292028442)) ;
#45765=CARTESIAN_POINT('Ctrl Pts',(0.362822641533809,-18.5648643423225,
-334.223104286098)) ;
#45766=CARTESIAN_POINT('Ctrl Pts',(0.0605900320434588,-18.568310577315,
-334.226819147546)) ;
#45767=CARTESIAN_POINT('Ctrl Pts',(-0.721153041578525,-18.5581371757636,
-334.236404149761)) ;
#45768=CARTESIAN_POINT('Ctrl Pts',(-1.20029231359165,-18.5333163615334,
-334.242259255512)) ;
#45769=CARTESIAN_POINT('Ctrl Pts',(-1.82205415582555,-18.4768926112265,
-334.249995012317)) ;
#45770=CARTESIAN_POINT('Ctrl Pts',(-1.96601924831227,-18.4621290801129,
-334.251795392878)) ;
#45771=CARTESIAN_POINT('Ctrl Pts',(-2.32282785022268,-18.4213177075875,
-334.256286003353)) ;
#45772=CARTESIAN_POINT('Ctrl Pts',(-2.53542039264459,-18.3932628564735,
-334.258986937321)) ;
#45773=CARTESIAN_POINT('Ctrl Pts',(-2.8785683235496,-18.3419168298212,-334.263395753412)) ;
#45774=CARTESIAN_POINT('Ctrl Pts',(-3.00944375969563,-18.320898361752,-334.265088856315)) ;
#45775=CARTESIAN_POINT('Ctrl Pts',(-3.26469715371016,-18.2770959927701,
-334.268414965052)) ;
#45776=CARTESIAN_POINT('Ctrl Pts',(-3.38908972751508,-18.2544393559275,
-334.270047051673)) ;
#45777=CARTESIAN_POINT('Ctrl Pts',(-3.66606851802552,-18.2010621850121,
-334.273706590879)) ;
#45778=CARTESIAN_POINT('Ctrl Pts',(-3.81851942844445,-18.1696899345628,
-334.275738168226)) ;
#45779=CARTESIAN_POINT('Ctrl Pts',(-4.66322470512088,-17.9847607222305,
-334.287089683705)) ;
#45780=CARTESIAN_POINT('Ctrl Pts',(-5.34663356926141,-17.7935601915349,
-334.296654972771)) ;
#45781=CARTESIAN_POINT('Ctrl Pts',(-6.28579369319399,-17.4717993665789,
-334.31001829902)) ;
#45782=CARTESIAN_POINT('Ctrl Pts',(-6.55202096753423,-17.3737156939757,
-334.313828228738)) ;
#45783=CARTESIAN_POINT('Ctrl Pts',(-6.98223753741354,-17.2039192596352,
-334.319973746453)) ;
#45784=CARTESIAN_POINT('Ctrl Pts',(-7.1476219923382,-17.1358682000654,-334.322333296239)) ;
#45785=CARTESIAN_POINT('Ctrl Pts',(-7.3860610225564,-17.0337046583356,-334.325718198654)) ;
#45786=CARTESIAN_POINT('Ctrl Pts',(-7.45991707887951,-17.0014890235164,
-334.326764268105)) ;
#45787=CARTESIAN_POINT('Ctrl Pts',(-7.59424086944535,-16.9418538772457,
-334.328660804968)) ;
#45788=CARTESIAN_POINT('Ctrl Pts',(-7.65477553867067,-16.9145889287314,
-334.329513108642)) ;
#45789=CARTESIAN_POINT('Ctrl Pts',(-7.80415937277042,-16.8463399441307,
-334.331611260977)) ;
#45790=CARTESIAN_POINT('Ctrl Pts',(-7.8928332868889,-16.8049771131737,-334.332852387202)) ;
#45791=CARTESIAN_POINT('Ctrl Pts',(-8.28021454280187,-16.6205367575039,
-334.338263290012)) ;
#45792=CARTESIAN_POINT('Ctrl Pts',(-8.57539026262081,-16.4701814752492,
-334.342358192938)) ;
#45793=CARTESIAN_POINT('Ctrl Pts',(-9.3409387196988,-16.0540679539547,-334.353067645324)) ;
#45794=CARTESIAN_POINT('Ctrl Pts',(-9.80400883300223,-15.775539463952,-334.359642782408)) ;
#45795=CARTESIAN_POINT('Ctrl Pts',(-10.3826217124048,-15.3921853306752,
-334.368230764424)) ;
#45796=CARTESIAN_POINT('Ctrl Pts',(-10.5099047488373,-15.3055579767557,
-334.370143498812)) ;
#45797=CARTESIAN_POINT('Ctrl Pts',(-10.8193306280354,-15.0892863163607,
-334.374858500856)) ;
#45798=CARTESIAN_POINT('Ctrl Pts',(-11.0002373504479,-14.9579161232912,
-334.377671776257)) ;
#45799=CARTESIAN_POINT('Ctrl Pts',(-11.2858399385413,-14.742534190098,-334.382214329645)) ;
#45800=CARTESIAN_POINT('Ctrl Pts',(-11.3920738375009,-14.6605985922271,
-334.383927008033)) ;
#45801=CARTESIAN_POINT('Ctrl Pts',(-11.5959872731738,-14.4997703713686,
-334.387260711737)) ;
#45802=CARTESIAN_POINT('Ctrl Pts',(-11.6937730282488,-14.4210240265024,
-334.388880476053)) ;
#45803=CARTESIAN_POINT('Ctrl Pts',(-11.9077721896485,-14.2450837319193,
-334.392472689701)) ;
#45804=CARTESIAN_POINT('Ctrl Pts',(-12.0236098740814,-14.1474469271071,
-334.394448735454)) ;
#45805=CARTESIAN_POINT('Ctrl Pts',(-12.4968342514946,-13.7385669542848,
-334.402652056966)) ;
#45806=CARTESIAN_POINT('Ctrl Pts',(-12.8434332773064,-13.4151148923754,
-334.408978375996)) ;
#45807=CARTESIAN_POINT('Ctrl Pts',(-13.498746496785,-12.7548654431428,-334.421484800521)) ;
#45808=CARTESIAN_POINT('Ctrl Pts',(-13.8081664109825,-12.4192306423428,
-334.427656766833)) ;
#45809=CARTESIAN_POINT('Ctrl Pts',(-14.2565399962579,-11.8953750017877,
-334.436865522598)) ;
#45810=CARTESIAN_POINT('Ctrl Pts',(-14.4048241148071,-11.7153711717295,
-334.439957907253)) ;
#45811=CARTESIAN_POINT('Ctrl Pts',(-14.6043070908721,-11.4637013278624,
-334.444158313241)) ;
#45812=CARTESIAN_POINT('Ctrl Pts',(-14.6584456478166,-11.3943935757637,
-334.445302506692)) ;
#45813=CARTESIAN_POINT('Ctrl Pts',(-14.7482570584799,-11.2777182465074,
-334.447205892481)) ;
#45814=CARTESIAN_POINT('Ctrl Pts',(-14.7841990102298,-11.2305598592307,
-334.447968969192)) ;
#45815=CARTESIAN_POINT('Ctrl Pts',(-14.8704460065605,-11.1162661242848,
-334.449803283974)) ;
#45816=CARTESIAN_POINT('Ctrl Pts',(-14.9205230524449,-11.048960532472,-334.450871234164)) ;
#45817=CARTESIAN_POINT('Ctrl Pts',(-15.0826689722672,-10.8279171632307,
-334.454342553687)) ;
#45818=CARTESIAN_POINT('Ctrl Pts',(-15.1928313830656,-10.6727957076851,
-334.456722311533)) ;
#45819=CARTESIAN_POINT('Ctrl Pts',(-15.449534817977,-10.2992971383052,-334.462349586075)) ;
#45820=CARTESIAN_POINT('Ctrl Pts',(-15.5938585115071,-10.0794456526334,
-334.465580725262)) ;
#45821=CARTESIAN_POINT('Ctrl Pts',(-15.9223120742536,-9.55515626982791,
-334.473165346432)) ;
#45822=CARTESIAN_POINT('Ctrl Pts',(-16.1024580766535,-9.24834455357784,
-334.477511918964)) ;
#45823=CARTESIAN_POINT('Ctrl Pts',(-16.4031146215664,-8.70084141298767,
-334.485205579039)) ;
#45824=CARTESIAN_POINT('Ctrl Pts',(-16.5274143295523,-8.4623510826058,-334.488536427741)) ;
#45825=CARTESIAN_POINT('Ctrl Pts',(-16.7407702828393,-8.03034504475609,
-334.494562262328)) ;
#45826=CARTESIAN_POINT('Ctrl Pts',(-16.8317598321595,-7.83783719699524,
-334.497244654576)) ;
#45827=CARTESIAN_POINT('Ctrl Pts',(-16.9738807287608,-7.52325536951615,
-334.50163141387)) ;
#45828=CARTESIAN_POINT('Ctrl Pts',(-17.0270533269511,-7.40212491718791,
-334.50332129445)) ;
#45829=CARTESIAN_POINT('Ctrl Pts',(-17.1285734497884,-7.16397234138079,
-334.506646452178)) ;
#45830=CARTESIAN_POINT('Ctrl Pts',(-17.177027451193,-7.0470033361435,-334.508280869247)) ;
#45831=CARTESIAN_POINT('Ctrl Pts',(-17.2826559256686,-6.78445020123704,
-334.511952824053)) ;
#45832=CARTESIAN_POINT('Ctrl Pts',(-17.3391947607239,-6.63862073991387,
-334.513994584264)) ;
#45833=CARTESIAN_POINT('Ctrl Pts',(-17.6452034078317,-5.81874989867252,
-334.525484348613)) ;
#45834=CARTESIAN_POINT('Ctrl Pts',(-17.8572104796468,-5.13138179749463,
-334.535184913434)) ;
#45835=CARTESIAN_POINT('Ctrl Pts',(-18.0948060746764,-4.16519082095492,
-334.54857548798)) ;
#45836=CARTESIAN_POINT('Ctrl Pts',(-18.1547807037349,-3.89547934922758,
-334.552284097521)) ;
#45837=CARTESIAN_POINT('Ctrl Pts',(-18.2430550491769,-3.45201155716157,
-334.558290187986)) ;
#45838=CARTESIAN_POINT('Ctrl Pts',(-18.2749422013507,-3.27901342508881,
-334.560610426075)) ;
#45839=CARTESIAN_POINT('Ctrl Pts',(-18.3177673711693,-3.02660146436936,
-334.563950611575)) ;
#45840=CARTESIAN_POINT('Ctrl Pts',(-18.3306571591814,-2.94752879965032,
-334.564990553045)) ;
#45841=CARTESIAN_POINT('Ctrl Pts',(-18.353306776474,-2.80268626697792,-334.566882154935)) ;
#45842=CARTESIAN_POINT('Ctrl Pts',(-18.3632258551222,-2.73694284368088,
-334.567735571055)) ;
#45843=CARTESIAN_POINT('Ctrl Pts',(-18.3869856787266,-2.57351709098916,
-334.569845038344)) ;
#45844=CARTESIAN_POINT('Ctrl Pts',(-18.4004013739677,-2.47577500698039,
-334.5710962358)) ;
#45845=CARTESIAN_POINT('Ctrl Pts',(-18.4569666177143,-2.03777317124503,
-334.576664774228)) ;
#45846=CARTESIAN_POINT('Ctrl Pts',(-18.4914615690006,-1.69646289845218,
-334.580901805232)) ;
#45847=CARTESIAN_POINT('Ctrl Pts',(-18.546601632436,-0.942619601587035,
-334.590187354682)) ;
#45848=CARTESIAN_POINT('Ctrl Pts',(-18.5629768743386,-0.529956224781748,
-334.595223777141)) ;
#45849=CARTESIAN_POINT('Ctrl Pts',(-18.5673349395481,0.161046040277517,
-334.603728896662)) ;
#45850=CARTESIAN_POINT('Ctrl Pts',(-18.5628386078489,0.439186823947205,
-334.607171077334)) ;
#45851=CARTESIAN_POINT('Ctrl Pts',(-18.5436811086748,0.934795978556484,
-334.613370065815)) ;
#45852=CARTESIAN_POINT('Ctrl Pts',(-18.5314366423763,1.15230564973967,-334.616113032938)) ;
#45853=CARTESIAN_POINT('Ctrl Pts',(-18.5055454482277,1.50233689082579,-334.620571872066)) ;
#45854=CARTESIAN_POINT('Ctrl Pts',(-18.4942951810996,1.63501503434382,-334.622272293172)) ;
#45855=CARTESIAN_POINT('Ctrl Pts',(-18.4696155105787,1.89306574802085,-334.625600896314)) ;
#45856=CARTESIAN_POINT('Ctrl Pts',(-18.4563342380763,2.01844531107866,-334.627228028078)) ;
#45857=CARTESIAN_POINT('Ctrl Pts',(-18.4205569663601,2.32623217401537,-334.631247166166)) ;
#45858=CARTESIAN_POINT('Ctrl Pts',(-18.3966276075011,2.50845920609918,-334.633648243915)) ;
#45859=CARTESIAN_POINT('Ctrl Pts',(-18.277206622158,3.32389338748949,-334.644486639968)) ;
#45860=CARTESIAN_POINT('Ctrl Pts',(-18.1516993285938,3.95225948531527,-334.653110232385)) ;
#45861=CARTESIAN_POINT('Ctrl Pts',(-17.9171599939278,4.87515640878925,-334.665934987984)) ;
#45862=CARTESIAN_POINT('Ctrl Pts',(-17.8327363118529,5.17545053380942,-334.670130313629)) ;
#45863=CARTESIAN_POINT('Ctrl Pts',(-17.6849378879217,5.65449911082292,-334.676799255836)) ;
#45864=CARTESIAN_POINT('Ctrl Pts',(-17.6263199943303,5.83465782853139,-334.679301578091)) ;
#45865=CARTESIAN_POINT('Ctrl Pts',(-17.5383327709844,6.0916449256034,-334.682848012174)) ;
#45866=CARTESIAN_POINT('Ctrl Pts',(-17.5111943223633,6.16922423934497,-334.68391555763)) ;
#45867=CARTESIAN_POINT('Ctrl Pts',(-17.4612960013028,6.30888364768524,-334.685830182909)) ;
#45868=CARTESIAN_POINT('Ctrl Pts',(-17.4387180028674,6.37102702394005,-334.6866793772)) ;
#45869=CARTESIAN_POINT('Ctrl Pts',(-17.3828101705274,6.52238296149466,-334.688741606875)) ;
#45870=CARTESIAN_POINT('Ctrl Pts',(-17.3491249463938,6.61146220988443,-334.689950341215)) ;
#45871=CARTESIAN_POINT('Ctrl Pts',(-17.2083728990571,6.97519147283076,-334.694872318711)) ;
#45872=CARTESIAN_POINT('Ctrl Pts',(-17.0954574713869,7.24753257978813,-334.698526475989)) ;
#45873=CARTESIAN_POINT('Ctrl Pts',(-16.7449739859308,8.03904372989135,-334.709185342693)) ;
#45874=CARTESIAN_POINT('Ctrl Pts',(-16.4898913497585,8.55007966398541,-334.716125255647)) ;
#45875=CARTESIAN_POINT('Ctrl Pts',(-16.1346040966126,9.18662362269907,-334.725139648184)) ;
#45876=CARTESIAN_POINT('Ctrl Pts',(-16.0557774060232,9.32370713590794,-334.727102977928)) ;
#45877=CARTESIAN_POINT('Ctrl Pts',(-15.8592529973868,9.65558831335999,-334.731917893013)) ;
#45878=CARTESIAN_POINT('Ctrl Pts',(-15.7397061963683,9.84926088056226,-334.7347805987)) ;
#45879=CARTESIAN_POINT('Ctrl Pts',(-15.5436941048321,10.1541253151516,-334.739382018417)) ;
#45880=CARTESIAN_POINT('Ctrl Pts',(-15.4695249852774,10.2667659954944,-334.741103306113)) ;
#45881=CARTESIAN_POINT('Ctrl Pts',(-15.3233469350836,10.4835859113985,-334.744459293243)) ;
#45882=CARTESIAN_POINT('Ctrl Pts',(-15.2514862958781,10.5878562781614,-334.746092773423)) ;
#45883=CARTESIAN_POINT('Ctrl Pts',(-15.0753970175753,10.8378503561383,-334.750057271545)) ;
#45884=CARTESIAN_POINT('Ctrl Pts',(-14.9701149257459,10.9828163300826,-334.752396439518)) ;
#45885=CARTESIAN_POINT('Ctrl Pts',(-14.3655955815914,11.7903509726719,-334.765652954175)) ;
#45886=CARTESIAN_POINT('Ctrl Pts',(-13.8244871909281,12.4203966440916,-334.776914533803)) ;
#45887=CARTESIAN_POINT('Ctrl Pts',(-13.1014090935313,13.1563077242409,-334.790746377223)) ;
#45888=CARTESIAN_POINT('Ctrl Pts',(-12.95740392087,13.2981591578323,-334.793444219881)) ;
#45889=CARTESIAN_POINT('Ctrl Pts',(-12.7074064393077,13.5365006882383,-334.798012809579)) ;
#45890=CARTESIAN_POINT('Ctrl Pts',(-12.602560414978,13.6341666556337,-334.799895507527)) ;
#45891=CARTESIAN_POINT('Ctrl Pts',(-12.4414866794291,13.7807641648348,-334.802730783084)) ;
#45892=CARTESIAN_POINT('Ctrl Pts',(-12.3860775970797,13.8305868834271,-334.803696054865)) ;
#45893=CARTESIAN_POINT('Ctrl Pts',(-12.2791137743815,13.9256082389218,-334.805538909772)) ;
#45894=CARTESIAN_POINT('Ctrl Pts',(-12.2276057249237,13.9708574588943,-334.80641720435)) ;
#45895=CARTESIAN_POINT('Ctrl Pts',(-12.0912680675626,14.0892969497332,-334.808719627033)) ;
#45896=CARTESIAN_POINT('Ctrl Pts',(-12.0060244345187,14.1620065440826,-334.810136693374)) ;
#45897=CARTESIAN_POINT('Ctrl Pts',(-11.8106733596294,14.3256021300721,-334.813339530063)) ;
#45898=CARTESIAN_POINT('Ctrl Pts',(-11.7001651441998,14.4159986571247,-334.81511974059)) ;
#45899=CARTESIAN_POINT('Ctrl Pts',(-11.3129673514627,14.7253440942672,-334.821266630856)) ;
#45900=CARTESIAN_POINT('Ctrl Pts',(-11.031087114766,14.9376740724118,-334.825584898947)) ;
#45901=CARTESIAN_POINT('Ctrl Pts',(-10.6331662647779,15.2200039204554,-334.831560752741)) ;
#45902=CARTESIAN_POINT('Ctrl Pts',(-10.5221549149392,15.2969604853562,-334.833215232113)) ;
#45903=CARTESIAN_POINT('Ctrl Pts',(-10.0114837144603,15.6427844347577,-334.840782520056)) ;
#45904=CARTESIAN_POINT('Ctrl Pts',(-9.60229484780592,15.8972464049429,-334.846730793534)) ;
#45905=CARTESIAN_POINT('Ctrl Pts',(-9.05209245154869,16.2103992740447,-334.854703446733)) ;
#45906=CARTESIAN_POINT('Ctrl Pts',(-8.91959807017974,16.2836787169063,-334.856620955008)) ;
#45907=CARTESIAN_POINT('Ctrl Pts',(-8.67563934037428,16.4147354267462,-334.860149937448)) ;
#45908=CARTESIAN_POINT('Ctrl Pts',(-8.5644567821932,16.4730184564934,-334.861757608175)) ;
#45909=CARTESIAN_POINT('Ctrl Pts',(-8.33321214612718,16.5912652568681,-334.865100991801)) ;
#45910=CARTESIAN_POINT('Ctrl Pts',(-8.21307371371956,16.6510638580455,-334.866837788918)) ;
#45911=CARTESIAN_POINT('Ctrl Pts',(-7.89090322448729,16.8070883332038,-334.871495187783)) ;
#45912=CARTESIAN_POINT('Ctrl Pts',(-7.68776226443511,16.9009728424642,-334.874431930134)) ;
#45913=CARTESIAN_POINT('Ctrl Pts',(-7.34187373136741,17.0533035043484,-334.879429125121)) ;
#45914=CARTESIAN_POINT('Ctrl Pts',(-7.20000472379042,17.1136846470925,-334.881477803015)) ;
#45915=CARTESIAN_POINT('Ctrl Pts',(-6.55638293432096,17.3781977745533,-334.890760756644)) ;
#45916=CARTESIAN_POINT('Ctrl Pts',(-6.04659468888901,17.562078631726,-334.89809085744)) ;
#45917=CARTESIAN_POINT('Ctrl Pts',(-5.21517692005276,17.8214714518222,-334.909787442976)) ;
#45918=CARTESIAN_POINT('Ctrl Pts',(-4.89830028389441,17.911157699109,-334.914184676779)) ;
#45919=CARTESIAN_POINT('Ctrl Pts',(-4.48448268482471,18.0164776857446,-334.919784517542)) ;
#45920=CARTESIAN_POINT('Ctrl Pts',(-4.38957009510065,18.0398372379562,-334.921059175655)) ;
#45921=CARTESIAN_POINT('Ctrl Pts',(-4.22989830484183,18.0778003623423,-334.923184703913)) ;
#45922=CARTESIAN_POINT('Ctrl Pts',(-4.1652373305955,18.0928080635579,-334.924040221036)) ;
#45923=CARTESIAN_POINT('Ctrl Pts',(-4.02185386386184,18.1252777304896,-334.925925175342)) ;
#45924=CARTESIAN_POINT('Ctrl Pts',(-3.94309544245242,18.1425742292935,-334.926952725404)) ;
#45925=CARTESIAN_POINT('Ctrl Pts',(-3.68894562083752,18.1966561299096,-334.930246733325)) ;
#45926=CARTESIAN_POINT('Ctrl Pts',(-3.51313330886312,18.2314154320961,-334.932492046634)) ;
#45927=CARTESIAN_POINT('Ctrl Pts',(-3.05682923452235,18.3147842117468,-334.938260883452)) ;
#45928=CARTESIAN_POINT('Ctrl Pts',(-2.7756733597146,18.3594979099268,-334.941758769023)) ;
#45929=CARTESIAN_POINT('Ctrl Pts',(-1.79347841549302,18.492623135642,-334.95390957906)) ;
#45930=CARTESIAN_POINT('Ctrl Pts',(-1.08850959084819,18.5474748060651,-334.962531681146)) ;
#45931=CARTESIAN_POINT('Ctrl Pts',(-0.226137140071919,18.5652284470579,
-334.973384166821)) ;
#45932=CARTESIAN_POINT('Ctrl Pts',(-0.0701043697563229,18.5664732941174,
-334.975358700397)) ;
#45933=CARTESIAN_POINT('Ctrl Pts',(0.21244671517656,18.5651656009107,-334.978957065454)) ;
#45934=CARTESIAN_POINT('Ctrl Pts',(0.338958649907062,18.5632867342027,-334.980576490627)) ;
#45935=CARTESIAN_POINT('Ctrl Pts',(0.5978107187438,18.5567953701525,-334.983907868395)) ;
#45936=CARTESIAN_POINT('Ctrl Pts',(0.730140633484629,18.5520599033789,-334.985620526827)) ;
#45937=CARTESIAN_POINT('Ctrl Pts',(1.07581454084149,18.5359856258674,-334.990119884488)) ;
#45938=CARTESIAN_POINT('Ctrl Pts',(1.28903312566806,18.5223792586798,-334.992920761094)) ;
#45939=CARTESIAN_POINT('Ctrl Pts',(1.64543360628384,18.4934519580819,-334.997642786405)) ;
#45940=CARTESIAN_POINT('Ctrl Pts',(1.78875779975869,18.4801396788161,-334.999552601963)) ;
#45941=CARTESIAN_POINT('Ctrl Pts',(2.40423387420777,18.4157456621252,-335.007795697354)) ;
#45942=CARTESIAN_POINT('Ctrl Pts',(2.87448468528685,18.3482251235911,-335.014204611253)) ;
#45943=CARTESIAN_POINT('Ctrl Pts',(3.39848912335852,18.2523454008388,-335.021375768667)) ;
#45944=CARTESIAN_POINT('Ctrl Pts',(3.45530234345666,18.2416755444744,-335.022153590786)) ;
#45945=CARTESIAN_POINT('Ctrl Pts',(3.84219285405449,18.1671429414192,-335.027451132733)) ;
#45946=CARTESIAN_POINT('Ctrl Pts',(4.17053313509686,18.0945898729303,-335.031951522119)) ;
#45947=CARTESIAN_POINT('Ctrl Pts',(4.60649799103957,17.9857576252338,-335.037864328576)) ;
#45948=CARTESIAN_POINT('Ctrl Pts',(4.71602109080528,17.9573507574365,-335.039344269852)) ;
#45949=CARTESIAN_POINT('Ctrl Pts',(4.88515740810982,17.911827986345,-335.041617645744)) ;
#45950=CARTESIAN_POINT('Ctrl Pts',(4.94495597873575,17.8954115654784,-335.042419047708)) ;
#45951=CARTESIAN_POINT('Ctrl Pts',(5.07353742131262,17.8594185684256,-335.044136307057)) ;
#45952=CARTESIAN_POINT('Ctrl Pts',(5.14229171559571,17.8397435378726,-335.045050889888)) ;
#45953=CARTESIAN_POINT('Ctrl Pts',(5.33334117923825,17.7838757573816,-335.047584099105)) ;
#45954=CARTESIAN_POINT('Ctrl Pts',(5.45537976069907,17.7468193442043,-335.049192929798)) ;
#45955=CARTESIAN_POINT('Ctrl Pts',(5.74013998785896,17.6571384165459,-335.052934228669)) ;
#45956=CARTESIAN_POINT('Ctrl Pts',(5.9025356937898,17.6035171672623,-335.055058112492)) ;
#45957=CARTESIAN_POINT('Ctrl Pts',(6.55056128187799,17.37957074211,-335.063529007624)) ;
#45958=CARTESIAN_POINT('Ctrl Pts',(7.02975633091527,17.1913309416564,-335.069789497846)) ;
#45959=CARTESIAN_POINT('Ctrl Pts',(7.79878571541552,16.8516990447861,-335.080130829806)) ;
#45960=CARTESIAN_POINT('Ctrl Pts',(8.09353731585515,16.7121354863115,-335.084166417869)) ;
#45961=CARTESIAN_POINT('Ctrl Pts',(8.56364763437041,16.4741850441395,-335.090766887485)) ;
#45962=CARTESIAN_POINT('Ctrl Pts',(8.74135166370509,16.3805862096651,-335.093300613804)) ;
#45963=CARTESIAN_POINT('Ctrl Pts',(9.02029785367972,16.2278298594257,-335.097345867512)) ;
#45964=CARTESIAN_POINT('Ctrl Pts',(9.12255836368312,16.1705647450697,-335.098843554123)) ;
#45965=CARTESIAN_POINT('Ctrl Pts',(9.3349146132372,16.0489913487388,-335.101985472813)) ;
#45966=CARTESIAN_POINT('Ctrl Pts',(9.44490399068585,15.984509460715,-335.103630943268)) ;
#45967=CARTESIAN_POINT('Ctrl Pts',(9.71263952343891,15.8238196955139,-335.107681537368)) ;
#45968=CARTESIAN_POINT('Ctrl Pts',(9.86963032907834,15.7263801706782,-335.110095728314)) ;
#45969=CARTESIAN_POINT('Ctrl Pts',(10.608794353554,15.2521748694022,-335.121646920329)) ;
#45970=CARTESIAN_POINT('Ctrl Pts',(11.171010492361,14.8453316983266,-335.131007608716)) ;
#45971=CARTESIAN_POINT('Ctrl Pts',(11.7775881036003,14.3523759763163,-335.141526842396)) ;
#45972=CARTESIAN_POINT('Ctrl Pts',(11.8456338819633,14.2962664932035,-335.142712793918)) ;
#45973=CARTESIAN_POINT('Ctrl Pts',(12.159573251382,14.0336167525546,-335.148208226059)) ;
#45974=CARTESIAN_POINT('Ctrl Pts',(12.400482178262,13.8212033954704,-335.152494796295)) ;
#45975=CARTESIAN_POINT('Ctrl Pts',(12.7072422536448,13.5362480902016,-335.157985287618)) ;
#45976=CARTESIAN_POINT('Ctrl Pts',(12.7781993768155,13.4692850136443,-335.159257552131)) ;
#45977=CARTESIAN_POINT('Ctrl Pts',(12.8965263157421,13.3558418634424,-335.161380424814)) ;
#45978=CARTESIAN_POINT('Ctrl Pts',(12.9441806394015,13.3096615472793,-335.162235651157)) ;
#45979=CARTESIAN_POINT('Ctrl Pts',(13.0492654056539,13.2067289895713,-335.164121633935)) ;
#45980=CARTESIAN_POINT('Ctrl Pts',(13.1065751819114,13.1498557123733,-335.165150484866)) ;
#45981=CARTESIAN_POINT('Ctrl Pts',(13.290362555739,12.96507305494,-335.16845424268)) ;
#45982=CARTESIAN_POINT('Ctrl Pts',(13.4153529347383,12.8356987352135,-335.170707832878)) ;
#45983=CARTESIAN_POINT('Ctrl Pts',(13.7344153334279,12.4956933315431,-335.176506159499)) ;
#45984=CARTESIAN_POINT('Ctrl Pts',(13.9255290044252,12.2823515155602,-335.180024946812)) ;
#45985=CARTESIAN_POINT('Ctrl Pts',(14.5676699450911,11.5312615220473,-335.192138305371)) ;
#45986=CARTESIAN_POINT('Ctrl Pts',(14.9930981765787,10.9724202655962,-335.200703778461)) ;
#45987=CARTESIAN_POINT('Ctrl Pts',(15.4832365987254,10.2466653948714,-335.21172074007)) ;
#45988=CARTESIAN_POINT('Ctrl Pts',(15.5785749733478,10.1011271131525,-335.213923475159)) ;
#45989=CARTESIAN_POINT('Ctrl Pts',(15.7393503430648,9.84800479290957,-335.217747183199)) ;
#45990=CARTESIAN_POINT('Ctrl Pts',(15.8057643995335,9.74105534921626,-335.219360550176)) ;
#45991=CARTESIAN_POINT('Ctrl Pts',(15.9420061327822,9.51659716334298,-335.222742887616)) ;
#45992=CARTESIAN_POINT('Ctrl Pts',(16.0116342319869,9.39897602189123,-335.224513243621)) ;
#45993=CARTESIAN_POINT('Ctrl Pts',(16.1989391232153,9.0744435962426,-335.229392614435)) ;
#45994=CARTESIAN_POINT('Ctrl Pts',(16.3139454326785,8.86602162089748,-335.232520691805)) ;
#45995=CARTESIAN_POINT('Ctrl Pts',(16.7484870171236,8.04141858283041,-335.244864565451)) ;
#45996=CARTESIAN_POINT('Ctrl Pts',(17.0373744834704,7.40972974153398,-335.254273306065)) ;
#45997=CARTESIAN_POINT('Ctrl Pts',(17.4028773753953,6.47533833914841,-335.267736308515)) ;
#45998=CARTESIAN_POINT('Ctrl Pts',(17.5083268686601,6.1845483665394,-335.271861169753)) ;
#45999=CARTESIAN_POINT('Ctrl Pts',(17.6369936157038,5.80001833959915,-335.27717671423)) ;
#46000=CARTESIAN_POINT('Ctrl Pts',(17.6668141086649,5.7085406040964,-335.278431005129)) ;
#46001=CARTESIAN_POINT('Ctrl Pts',(17.7159539974586,5.55372465704394,-335.280534038441)) ;
#46002=CARTESIAN_POINT('Ctrl Pts',(17.7356480328786,5.49050748954687,-335.281387182829)) ;
#46003=CARTESIAN_POINT('Ctrl Pts',(17.7788443887502,5.34919089565252,-335.28328137853)) ;
#46004=CARTESIAN_POINT('Ctrl Pts',(17.8021710712351,5.27103938638333,-335.284320381813)) ;
#46005=CARTESIAN_POINT('Ctrl Pts',(17.8767873112735,5.01490601589579,-335.287701252093)) ;
#46006=CARTESIAN_POINT('Ctrl Pts',(17.9259285651468,4.83630977255176,-335.290020416263)) ;
#46007=CARTESIAN_POINT('Ctrl Pts',(18.1401181458702,4.00970639251432,-335.300632559098)) ;
#46008=CARTESIAN_POINT('Ctrl Pts',(18.272754612018,3.35381502164704,-335.308728569246)) ;
#46009=CARTESIAN_POINT('Ctrl Pts',(18.4216534090388,2.33783205182358,-335.321397904403)) ;
#46010=CARTESIAN_POINT('Ctrl Pts',(18.4633231901178,1.98203657134443,-335.32585448747)) ;
#46011=CARTESIAN_POINT('Ctrl Pts',(18.50833031021,1.46987710301421,-335.332344842534)) ;
#46012=CARTESIAN_POINT('Ctrl Pts',(18.5200261629321,1.3143288773807,-335.334325667501)) ;
#46013=CARTESIAN_POINT('Ctrl Pts',(18.5375033057871,1.03482537456268,-335.33790482575)) ;
#46014=CARTESIAN_POINT('Ctrl Pts',(18.5440046642734,0.910924436206806,-335.339498394796)) ;
#46015=CARTESIAN_POINT('Ctrl Pts',(18.5554770703173,0.640513505423163,-335.342992291914)) ;
#46016=CARTESIAN_POINT('Ctrl Pts',(18.559955810908,0.493990962892338,-335.344895693779)) ;
#46017=CARTESIAN_POINT('Ctrl Pts',(18.5683104299641,0.0476165308628815,
-335.350725534762)) ;
#46018=CARTESIAN_POINT('Ctrl Pts',(18.5666574562054,-0.252289148872367,
-335.354685981898)) ;
#46019=CARTESIAN_POINT('Ctrl Pts',(18.5543991293277,-0.664386315309379,
-335.360177154725)) ;
#46020=CARTESIAN_POINT('Ctrl Pts',(18.5500365024344,-0.776710141285842,
-335.361678784497)) ;
#46021=CARTESIAN_POINT('Ctrl Pts',(18.5446545934131,-0.888979984870959,
-335.363183819487)) ;
#46022=CARTESIAN_POINT('Origin',(0.,0.,-315.477129595899)) ;
#46023=CARTESIAN_POINT('',(18.5446545937554,-0.888979977731322,-337.158465839576)) ;
#46024=CARTESIAN_POINT('',(18.544654593745,-0.888979977948828,-336.86323988221)) ;
#46025=CARTESIAN_POINT('',(18.544654593745,-0.888979977948782,-315.477129595899)) ;
#46026=CARTESIAN_POINT('Ctrl Pts',(18.5446545937658,-0.888979977513935,
-337.158465839576)) ;
#46027=CARTESIAN_POINT('Ctrl Pts',(18.5567562697993,-0.636531769767257,
-337.155292643735)) ;
#46028=CARTESIAN_POINT('Ctrl Pts',(18.5637020684296,-0.383857592640776,
-337.152163036735)) ;
#46029=CARTESIAN_POINT('Ctrl Pts',(18.5663697796789,-0.0061192947651607,
-337.147512304642)) ;
#46030=CARTESIAN_POINT('Ctrl Pts',(18.5659901745631,0.118882716158257,-337.145977908322)) ;
#46031=CARTESIAN_POINT('Ctrl Pts',(18.5597324315834,0.595244166917408,-337.14013704646)) ;
#46032=CARTESIAN_POINT('Ctrl Pts',(18.5451417327675,0.946415148907194,-337.135843235536)) ;
#46033=CARTESIAN_POINT('Ctrl Pts',(18.5015418685101,1.5690214974659,-337.128158002302)) ;
#46034=CARTESIAN_POINT('Ctrl Pts',(18.4764975206981,1.84063005911752,-337.124781065078)) ;
#46035=CARTESIAN_POINT('Ctrl Pts',(18.4210302448419,2.32515666672852,-337.118683393839)) ;
#46036=CARTESIAN_POINT('Ctrl Pts',(18.3928741750221,2.53828449067063,-337.115975760661)) ;
#46037=CARTESIAN_POINT('Ctrl Pts',(18.341368806701,2.88206284969703,-337.111558877197)) ;
#46038=CARTESIAN_POINT('Ctrl Pts',(18.3203086444005,3.01303619058971,-337.109864509858)) ;
#46039=CARTESIAN_POINT('Ctrl Pts',(18.2764450857783,3.26833732425785,-337.106537758219)) ;
#46040=CARTESIAN_POINT('Ctrl Pts',(18.2537720555308,3.3926802869411,-337.104906313498)) ;
#46041=CARTESIAN_POINT('Ctrl Pts',(18.2003958829717,3.66936466357962,-337.101250644211)) ;
#46042=CARTESIAN_POINT('Ctrl Pts',(18.1690461305778,3.82157165818196,-337.099222327372)) ;
#46043=CARTESIAN_POINT('Ctrl Pts',(17.9836530903229,4.66776813269176,-337.087850924263)) ;
#46044=CARTESIAN_POINT('Ctrl Pts',(17.7917609371563,5.35285647313084,-337.078260924487)) ;
#46045=CARTESIAN_POINT('Ctrl Pts',(17.4692148511989,6.29294280349286,-337.064882584481)) ;
#46046=CARTESIAN_POINT('Ctrl Pts',(17.3712584096113,6.55850426742939,-337.06108178205)) ;
#46047=CARTESIAN_POINT('Ctrl Pts',(17.2016573048195,6.98780170118767,-337.05494875179)) ;
#46048=CARTESIAN_POINT('Ctrl Pts',(17.1336522304962,7.15292584092232,-337.052592671772)) ;
#46049=CARTESIAN_POINT('Ctrl Pts',(17.0315351592198,7.39106188012024,-337.04921168884)) ;
#46050=CARTESIAN_POINT('Ctrl Pts',(16.9993133661875,7.46487312000773,-337.048166133859)) ;
#46051=CARTESIAN_POINT('Ctrl Pts',(16.9396529773855,7.59914895596636,-337.046270050309)) ;
#46052=CARTESIAN_POINT('Ctrl Pts',(16.9123684159812,7.65968030700843,-337.045417691896)) ;
#46053=CARTESIAN_POINT('Ctrl Pts',(16.8440486129559,7.80910438499991,-337.043318719734)) ;
#46054=CARTESIAN_POINT('Ctrl Pts',(16.802633799864,7.89782137043411,-337.04207683876)) ;
#46055=CARTESIAN_POINT('Ctrl Pts',(16.6220771512405,8.27675260561849,-337.03678330221)) ;
#46056=CARTESIAN_POINT('Ctrl Pts',(16.4761032282204,8.56365026456009,-337.032801961933)) ;
#46057=CARTESIAN_POINT('Ctrl Pts',(16.2777037036849,8.92971426445733,-337.027682521909)) ;
#46058=CARTESIAN_POINT('Ctrl Pts',(16.2320280035139,9.01247477726652,-337.026522515515)) ;
#46059=CARTESIAN_POINT('Ctrl Pts',(16.0139482573076,9.40058073245432,-337.021064478593)) ;
#46060=CARTESIAN_POINT('Ctrl Pts',(15.8335481805643,9.70135087926533,-337.016779893667)) ;
#46061=CARTESIAN_POINT('Ctrl Pts',(15.4975674229055,10.2271506263078,-337.009096999331)) ;
#46062=CARTESIAN_POINT('Ctrl Pts',(15.3453276903723,10.4541916813073,-337.005712895873)) ;
#46063=CARTESIAN_POINT('Ctrl Pts',(15.0643199055576,10.8538983379358,-336.999604145336)) ;
#46064=CARTESIAN_POINT('Ctrl Pts',(14.9374550057992,11.0278411787421,-336.996892683186)) ;
#46065=CARTESIAN_POINT('Ctrl Pts',(14.7275511370488,11.3053679161451,-336.992471453234)) ;
#46066=CARTESIAN_POINT('Ctrl Pts',(14.6463759817764,11.4103363996441,-336.990776634408)) ;
#46067=CARTESIAN_POINT('Ctrl Pts',(14.4857356215429,11.613523216645,-336.987450264637)) ;
#46068=CARTESIAN_POINT('Ctrl Pts',(14.4063792906671,11.7118185471072,-336.985819667026)) ;
#46069=CARTESIAN_POINT('Ctrl Pts',(14.208070037954,11.9523903358009,-336.981775088934)) ;
#46070=CARTESIAN_POINT('Ctrl Pts',(14.087976904432,12.0937089231611,-336.979351759017)) ;
#46071=CARTESIAN_POINT('Ctrl Pts',(13.6481913655868,12.5957810650133,-336.97057167981)) ;
#46072=CARTESIAN_POINT('Ctrl Pts',(13.3165973381164,12.9458511187139,-336.964120467453)) ;
#46073=CARTESIAN_POINT('Ctrl Pts',(12.6108566173104,13.6350749963717,-336.950844779163)) ;
#46074=CARTESIAN_POINT('Ctrl Pts',(12.2357395372514,13.9726752301543,-336.944022257355)) ;
#46075=CARTESIAN_POINT('Ctrl Pts',(11.7216064221612,14.3987885259726,-336.935165816693)) ;
#46076=CARTESIAN_POINT('Ctrl Pts',(11.5945019994838,14.5013341341481,-336.93301473412)) ;
#46077=CARTESIAN_POINT('Ctrl Pts',(11.4046746967651,14.6503920162474,-336.929868240186)) ;
#46078=CARTESIAN_POINT('Ctrl Pts',(11.342984852882,14.6982068912601,-336.928855816822)) ;
#46079=CARTESIAN_POINT('Ctrl Pts',(11.2277571357391,14.7863606840983,-336.92698495313)) ;
#46080=CARTESIAN_POINT('Ctrl Pts',(11.1742988899914,14.8268013032702,-336.926125126086)) ;
#46081=CARTESIAN_POINT('Ctrl Pts',(11.0521730600659,14.9181525989152,-336.924178265233)) ;
#46082=CARTESIAN_POINT('Ctrl Pts',(10.9833704833917,14.9688803577792,-336.923093772265)) ;
#46083=CARTESIAN_POINT('Ctrl Pts',(10.6789273384906,15.1901154886566,-336.918343633572)) ;
#46084=CARTESIAN_POINT('Ctrl Pts',(10.4396486137258,15.3555473752115,-336.914736844778)) ;
#46085=CARTESIAN_POINT('Ctrl Pts',(10.0746492802615,15.5954233763319,-336.909357438523)) ;
#46086=CARTESIAN_POINT('Ctrl Pts',(9.95177606831765,15.6741169297108,-336.907566836997)) ;
#46087=CARTESIAN_POINT('Ctrl Pts',(9.42794367936804,16.0009598449627,-336.89999874063)) ;
#46088=CARTESIAN_POINT('Ctrl Pts',(9.01853544827729,16.2352350196351,-336.894239840264)) ;
#46089=CARTESIAN_POINT('Ctrl Pts',(8.33480329127769,16.5926351629743,-336.884678171299)) ;
#46090=CARTESIAN_POINT('Ctrl Pts',(8.06562385307727,16.7251367367903,-336.88092859648)) ;
#46091=CARTESIAN_POINT('Ctrl Pts',(7.6602864556012,16.9125989963316,-336.875278541703)) ;
#46092=CARTESIAN_POINT('Ctrl Pts',(7.52649588348654,16.9725617697364,-336.87341316603)) ;
#46093=CARTESIAN_POINT('Ctrl Pts',(7.27819199945763,17.0803341717333,-336.869948370651)) ;
#46094=CARTESIAN_POINT('Ctrl Pts',(7.16388245636576,17.1285925370263,-336.868352235365)) ;
#46095=CARTESIAN_POINT('Ctrl Pts',(6.90480067224838,17.2349225675018,-336.864731485817)) ;
#46096=CARTESIAN_POINT('Ctrl Pts',(6.75976307380804,17.2923229011406,-336.862702340124)) ;
#46097=CARTESIAN_POINT('Ctrl Pts',(6.28507108121731,17.4733029719652,-336.856054341685)) ;
#46098=CARTESIAN_POINT('Ctrl Pts',(5.95262280313957,17.5893352915917,-336.851386464728)) ;
#46099=CARTESIAN_POINT('Ctrl Pts',(4.97366137958809,17.9000806887025,-336.837652218947)) ;
#46100=CARTESIAN_POINT('Ctrl Pts',(4.31958675082728,18.0690720154357,-336.828474708222)) ;
#46101=CARTESIAN_POINT('Ctrl Pts',(3.4763905016348,18.2385151308603,-336.81703926607)) ;
#46102=CARTESIAN_POINT('Ctrl Pts',(3.29447959314486,18.2722502588086,-336.814596710105)) ;
#46103=CARTESIAN_POINT('Ctrl Pts',(3.03172002294195,18.3169271429608,-336.811117675029)) ;
#46104=CARTESIAN_POINT('Ctrl Pts',(2.95125608790527,18.330063660189,-336.810058919755)) ;
#46105=CARTESIAN_POINT('Ctrl Pts',(2.80528283975242,18.352909112998,-336.808151796256)) ;
#46106=CARTESIAN_POINT('Ctrl Pts',(2.73980333612965,18.3627983269661,-336.807301427291)) ;
#46107=CARTESIAN_POINT('Ctrl Pts',(2.57900092377559,18.3862046808985,-336.80522493634)) ;
#46108=CARTESIAN_POINT('Ctrl Pts',(2.48362310448242,18.399331092353,-336.804003282988)) ;
#46109=CARTESIAN_POINT('Ctrl Pts',(2.08093738961163,18.4515626660339,-336.798880220109)) ;
#46110=CARTESIAN_POINT('Ctrl Pts',(1.77277739324593,18.4837151674474,-336.795044236238)) ;
#46111=CARTESIAN_POINT('Ctrl Pts',(0.907565020169588,18.5521517373054,-336.784365830641)) ;
#46112=CARTESIAN_POINT('Ctrl Pts',(0.349471609057681,18.5710494802052,-336.7775769169)) ;
#46113=CARTESIAN_POINT('Ctrl Pts',(-0.43592428748611,18.5622235053451,-336.767862016259)) ;
#46114=CARTESIAN_POINT('Ctrl Pts',(-0.663158423480988,18.555494930888,-336.765033651854)) ;
#46115=CARTESIAN_POINT('Ctrl Pts',(-1.07949910790506,18.5355089896144,-336.759803437191)) ;
#46116=CARTESIAN_POINT('Ctrl Pts',(-1.26863640305428,18.5235248627216,-336.757409259633)) ;
#46117=CARTESIAN_POINT('Ctrl Pts',(-1.58541793185425,18.4985783031037,-336.753363582959)) ;
#46118=CARTESIAN_POINT('Ctrl Pts',(-1.71317115918243,18.487184582256,-336.751722286901)) ;
#46119=CARTESIAN_POINT('Ctrl Pts',(-1.97216889210278,18.4613780488473,-336.748374004994)) ;
#46120=CARTESIAN_POINT('Ctrl Pts',(-2.10339834486485,18.4468871342256,-336.74666659927)) ;
#46121=CARTESIAN_POINT('Ctrl Pts',(-2.44437362391138,18.4055493676765,-336.7422014074)) ;
#46122=CARTESIAN_POINT('Ctrl Pts',(-2.65383490751731,18.376516807677,-336.739429854847)) ;
#46123=CARTESIAN_POINT('Ctrl Pts',(-3.15857874535579,18.2977463968594,-336.732685478952)) ;
#46124=CARTESIAN_POINT('Ctrl Pts',(-3.45324271576011,18.244430851697,-336.728693087521)) ;
#46125=CARTESIAN_POINT('Ctrl Pts',(-4.25515248535949,18.0792118150392,-336.717712723824)) ;
#46126=CARTESIAN_POINT('Ctrl Pts',(-4.75919515028514,17.9531134708476,-336.710678590039)) ;
#46127=CARTESIAN_POINT('Ctrl Pts',(-5.42193805271025,17.7574367696726,-336.701439981366)) ;
#46128=CARTESIAN_POINT('Ctrl Pts',(-5.58590769350217,17.7065413971175,-336.699155829618)) ;
#46129=CARTESIAN_POINT('Ctrl Pts',(-5.87075010631022,17.6137772209458,-336.695203185153)) ;
#46130=CARTESIAN_POINT('Ctrl Pts',(-5.99193998127609,17.5729197956022,-336.693526391886)) ;
#46131=CARTESIAN_POINT('Ctrl Pts',(-6.18028721615459,17.5072463003436,-336.690933260321)) ;
#46132=CARTESIAN_POINT('Ctrl Pts',(-6.24773948238433,17.4832884341897,-336.690007186094)) ;
#46133=CARTESIAN_POINT('Ctrl Pts',(-6.37332284432578,17.4378638346729,-336.688289022035)) ;
#46134=CARTESIAN_POINT('Ctrl Pts',(-6.43148827095938,17.4164949924739,-336.687495671126)) ;
#46135=CARTESIAN_POINT('Ctrl Pts',(-6.5953026184196,17.3553802612759,-336.685266860367)) ;
#46136=CARTESIAN_POINT('Ctrl Pts',(-6.70069769891658,17.3149614798411,-336.683839407664)) ;
#46137=CARTESIAN_POINT('Ctrl Pts',(-7.02358678683696,17.1877445697093,-336.679477887345)) ;
#46138=CARTESIAN_POINT('Ctrl Pts',(-7.23981271987873,17.0977907015879,-336.67657328316)) ;
#46139=CARTESIAN_POINT('Ctrl Pts',(-7.99392065307223,16.7671974887354,-336.666421941636)) ;
#46140=CARTESIAN_POINT('Ctrl Pts',(-8.5219940652943,16.5050688491558,-336.659264380148)) ;
#46141=CARTESIAN_POINT('Ctrl Pts',(-9.1768721728353,16.1401754037574,-336.649997126615)) ;
#46142=CARTESIAN_POINT('Ctrl Pts',(-9.31601836366531,16.0602629715205,-336.648005517679)) ;
#46143=CARTESIAN_POINT('Ctrl Pts',(-9.65188776211912,15.861537479519,-336.643135053198)) ;
#46144=CARTESIAN_POINT('Ctrl Pts',(-9.84747445905211,15.740856237419,-336.640245020884)) ;
#46145=CARTESIAN_POINT('Ctrl Pts',(-10.1545368813124,15.5434286267316,-336.635611046358)) ;
#46146=CARTESIAN_POINT('Ctrl Pts',(-10.2675007687193,15.4690407151842,-336.63388499411)) ;
#46147=CARTESIAN_POINT('Ctrl Pts',(-10.4844904167196,15.3227266391031,-336.630526590696)) ;
#46148=CARTESIAN_POINT('Ctrl Pts',(-10.5886140457514,15.2509587728463,-336.628895536981)) ;
#46149=CARTESIAN_POINT('Ctrl Pts',(-10.8144819938412,15.0918496596646,-336.625313969049)) ;
#46150=CARTESIAN_POINT('Ctrl Pts',(-10.9359186805812,15.0040870921575,-336.623360232306)) ;
#46151=CARTESIAN_POINT('Ctrl Pts',(-11.6525467406019,14.4728559637148,-336.611663134489)) ;
#46152=CARTESIAN_POINT('Ctrl Pts',(-12.2217695931637,13.9954901206591,-336.601643618155)) ;
#46153=CARTESIAN_POINT('Ctrl Pts',(-12.9589093723638,13.2979508370078,-336.587986986086)) ;
#46154=CARTESIAN_POINT('Ctrl Pts',(-13.1527849684153,13.1062228143882,-336.584327958292)) ;
#46155=CARTESIAN_POINT('Ctrl Pts',(-13.463676746494,12.784926317954,-336.578390382288)) ;
#46156=CARTESIAN_POINT('Ctrl Pts',(-13.5832126386779,12.657853968376,-336.576089660141)) ;
#46157=CARTESIAN_POINT('Ctrl Pts',(-13.7548502106752,12.4701634617688,-336.572771700365)) ;
#46158=CARTESIAN_POINT('Ctrl Pts',(-13.8083793848541,12.4108637841577,-336.571734823991)) ;
#46159=CARTESIAN_POINT('Ctrl Pts',(-13.9057904337165,12.3015413394571,-336.569845635621)) ;
#46160=CARTESIAN_POINT('Ctrl Pts',(-13.9497891796328,12.2516247391718,-336.568991608613)) ;
#46161=CARTESIAN_POINT('Ctrl Pts',(-14.0586333753049,12.1267944558571,-336.566876218597)) ;
#46162=CARTESIAN_POINT('Ctrl Pts',(-14.1231493066189,12.0515961540475,-336.56561977761)) ;
#46163=CARTESIAN_POINT('Ctrl Pts',(-14.4138022021324,11.7072783723535,-336.559938952931)) ;
#46164=CARTESIAN_POINT('Ctrl Pts',(-14.6328706427724,11.4322858053713,-336.555599003202)) ;
#46165=CARTESIAN_POINT('Ctrl Pts',(-15.2569942737539,10.6014820992475,-336.542837805108)) ;
#46166=CARTESIAN_POINT('Ctrl Pts',(-15.6391277067598,10.0292064663032,-336.534474030605)) ;
#46167=CARTESIAN_POINT('Ctrl Pts',(-16.097757337041,9.25217787662991,-336.52319229753)) ;
#46168=CARTESIAN_POINT('Ctrl Pts',(-16.2036637890586,9.06542146414458,-336.520488169062)) ;
#46169=CARTESIAN_POINT('Ctrl Pts',(-16.3697043533782,8.76041437548144,-336.516075554971)) ;
#46170=CARTESIAN_POINT('Ctrl Pts',(-16.4318517381587,8.64328230715969,-336.514381899269)) ;
#46171=CARTESIAN_POINT('Ctrl Pts',(-16.5507852195466,8.41320312227444,-336.511055624868)) ;
#46172=CARTESIAN_POINT('Ctrl Pts',(-16.6076830542664,8.30032178143017,-336.509423935506)) ;
#46173=CARTESIAN_POINT('Ctrl Pts',(-16.7319975258299,8.0472940513436,-336.505766510194)) ;
#46174=CARTESIAN_POINT('Ctrl Pts',(-16.7988150144228,7.90686390211875,-336.503736666043)) ;
#46175=CARTESIAN_POINT('Ctrl Pts',(-17.1608143969122,7.12074327833533,-336.492375538771)) ;
#46176=CARTESIAN_POINT('Ctrl Pts',(-17.4205338990276,6.4593750599135,-336.482798126859)) ;
#46177=CARTESIAN_POINT('Ctrl Pts',(-17.730023271277,5.51552875132217,-336.46942760497)) ;
#46178=CARTESIAN_POINT('Ctrl Pts',(-17.8121321647762,5.2443045931346,-336.465622319275)) ;
#46179=CARTESIAN_POINT('Ctrl Pts',(-17.93584988548,4.79913745501913,-336.459483175267)) ;
#46180=CARTESIAN_POINT('Ctrl Pts',(-17.9812101117979,4.62628517669532,-336.457125410538)) ;
#46181=CARTESIAN_POINT('Ctrl Pts',(-18.0433879899686,4.37460149887323,-336.453742539951)) ;
#46182=CARTESIAN_POINT('Ctrl Pts',(-18.062198801569,4.29627314160134,-336.452696750144)) ;
#46183=CARTESIAN_POINT('Ctrl Pts',(-18.095582908199,4.15316588925237,-336.450800445282)) ;
#46184=CARTESIAN_POINT('Ctrl Pts',(-18.1103195698457,4.08842668559268,-336.44994809757)) ;
#46185=CARTESIAN_POINT('Ctrl Pts',(-18.1459211819759,3.92805605074874,-336.447849461296)) ;
#46186=CARTESIAN_POINT('Ctrl Pts',(-18.1663777533453,3.83233600343261,-336.446607900867)) ;
#46187=CARTESIAN_POINT('Ctrl Pts',(-18.2508778676688,3.42105738117352,-336.441312804342)) ;
#46188=CARTESIAN_POINT('Ctrl Pts',(-18.3074634740286,3.10402297325208,-336.437329661554)) ;
#46189=CARTESIAN_POINT('Ctrl Pts',(-18.3699386717705,2.69235262795825,-336.432210067408)) ;
#46190=CARTESIAN_POINT('Ctrl Pts',(-18.3833897152854,2.59892132656995,-336.43105169549)) ;
#46191=CARTESIAN_POINT('Ctrl Pts',(-18.4434339071094,2.15803988468078,-336.425596431966)) ;
#46192=CARTESIAN_POINT('Ctrl Pts',(-18.4808927472196,1.80941804718231,-336.421312987516)) ;
#46193=CARTESIAN_POINT('Ctrl Pts',(-18.5299579981378,1.18739330582407,-336.413630369156)) ;
#46194=CARTESIAN_POINT('Ctrl Pts',(-18.5454339069767,0.914399885724085,
-336.41024536525)) ;
#46195=CARTESIAN_POINT('Ctrl Pts',(-18.5623115221588,0.425973134568299,
-336.404135161628)) ;
#46196=CARTESIAN_POINT('Ctrl Pts',(-18.5660033562227,0.210668697880257,
-336.401423155009)) ;
#46197=CARTESIAN_POINT('Ctrl Pts',(-18.5659161735629,-0.137358097947155,
-336.397001164568)) ;
#46198=CARTESIAN_POINT('Ctrl Pts',(-18.5644600674199,-0.270061020512011,
-336.395306135838)) ;
#46199=CARTESIAN_POINT('Ctrl Pts',(-18.5588407984291,-0.529045351700046,
-336.391979415567)) ;
#46200=CARTESIAN_POINT('Ctrl Pts',(-18.5548110498324,-0.655322528790837,
-336.390348678161)) ;
#46201=CARTESIAN_POINT('Ctrl Pts',(-18.5416858984054,-0.966838532375095,
-336.386303830494)) ;
#46202=CARTESIAN_POINT('Ctrl Pts',(-18.531103222829,-1.15200081721432,-336.383880371292)) ;
#46203=CARTESIAN_POINT('Ctrl Pts',(-18.483089750188,-1.81701145684823,-336.375109608542)) ;
#46204=CARTESIAN_POINT('Ctrl Pts',(-18.4297782597219,-2.29551918311458,
-336.368668198411)) ;
#46205=CARTESIAN_POINT('Ctrl Pts',(-18.2825850409861,-3.27053240538154,
-336.355398101143)) ;
#46206=CARTESIAN_POINT('Ctrl Pts',(-18.1869112130232,-3.76637210749894,
-336.348571176284)) ;
#46207=CARTESIAN_POINT('Ctrl Pts',(-18.0336523692484,-4.41685634927133,
-336.339707462039)) ;
#46208=CARTESIAN_POINT('Ctrl Pts',(-17.9940517843836,-4.57551508804472,
-336.33755352673)) ;
#46209=CARTESIAN_POINT('Ctrl Pts',(-17.9324501406615,-4.80914020858552,
-336.334403681478)) ;
#46210=CARTESIAN_POINT('Ctrl Pts',(-17.9120636184851,-4.88452398323032,
-336.333390713508)) ;
#46211=CARTESIAN_POINT('Ctrl Pts',(-17.8732975390369,-5.02436328813107,
-336.331519418475)) ;
#46212=CARTESIAN_POINT('Ctrl Pts',(-17.8550434264498,-5.08885209058303,
-336.330659697937)) ;
#46213=CARTESIAN_POINT('Ctrl Pts',(-17.812728065778,-5.2353143774279,-336.328713570545)) ;
#46214=CARTESIAN_POINT('Ctrl Pts',(-17.7884493942864,-5.31722351885506,
-336.327629697744)) ;
#46215=CARTESIAN_POINT('Ctrl Pts',(-17.6813555249235,-5.66958259143766,
-336.322981278002)) ;
#46216=CARTESIAN_POINT('Ctrl Pts',(-17.5929312022217,-5.93828867028473,
-336.319472130966)) ;
#46217=CARTESIAN_POINT('Ctrl Pts',(-17.3043095538492,-6.75223285826448,
-336.30883132113)) ;
#46218=CARTESIAN_POINT('Ctrl Pts',(-17.084640688499,-7.29018734870015,-336.301774043995)) ;
#46219=CARTESIAN_POINT('Ctrl Pts',(-16.7730086680608,-7.96153794060978,
-336.292623162396)) ;
#46220=CARTESIAN_POINT('Ctrl Pts',(-16.7040383798498,-8.10524570202314,
-336.29064441308)) ;
#46221=CARTESIAN_POINT('Ctrl Pts',(-16.5315834185869,-8.45302284840997,
-336.285799186626)) ;
#46222=CARTESIAN_POINT('Ctrl Pts',(-16.4261605342635,-8.65610163002536,
-336.282921557853)) ;
#46223=CARTESIAN_POINT('Ctrl Pts',(-16.2525716896902,-8.97589317218265,
-336.278302365516)) ;
#46224=CARTESIAN_POINT('Ctrl Pts',(-16.1868382803381,-9.09389966894386,
-336.276578480985)) ;
#46225=CARTESIAN_POINT('Ctrl Pts',(-16.0570451834132,-9.32104126853999,
-336.273221206447)) ;
#46226=CARTESIAN_POINT('Ctrl Pts',(-15.9931458759472,-9.43025955573592,
-336.271589078608)) ;
#46227=CARTESIAN_POINT('Ctrl Pts',(-15.8509624496447,-9.66768072320648,
-336.268001387954)) ;
#46228=CARTESIAN_POINT('Ctrl Pts',(-15.7722288425241,-9.79560403429044,
-336.266042554703)) ;
#46229=CARTESIAN_POINT('Ctrl Pts',(-15.4510962710633,-10.3034566413096,
-336.258163064071)) ;
#46230=CARTESIAN_POINT('Ctrl Pts',(-15.1964527699241,-10.6754585813738,
-336.25215386373)) ;
#46231=CARTESIAN_POINT('Ctrl Pts',(-14.6450789876428,-11.4211850932865,
-336.239694244621)) ;
#46232=CARTESIAN_POINT('Ctrl Pts',(-14.3469692556618,-11.7934846595732,
-336.233242751879)) ;
#46233=CARTESIAN_POINT('Ctrl Pts',(-13.9265978178705,-12.2789137548389,
-336.224663640599)) ;
#46234=CARTESIAN_POINT('Ctrl Pts',(-13.8166691038514,-12.4024797833195,
-336.22246495281)) ;
#46235=CARTESIAN_POINT('Ctrl Pts',(-13.6210884603511,-12.6164955196736,
-336.218641797016)) ;
#46236=CARTESIAN_POINT('Ctrl Pts',(-13.5361497673482,-12.7075827597181,
-336.217009717293)) ;
#46237=CARTESIAN_POINT('Ctrl Pts',(-13.4014112342618,-12.849190895936,-336.214469463719)) ;
#46238=CARTESIAN_POINT('Ctrl Pts',(-13.3522274458185,-12.9002927100518,
-336.213552157006)) ;
#46239=CARTESIAN_POINT('Ctrl Pts',(-13.2592229408114,-12.9958224154869,
-336.211837323868)) ;
#46240=CARTESIAN_POINT('Ctrl Pts',(-13.2154687116982,-13.0403136461891,
-336.211038654821)) ;
#46241=CARTESIAN_POINT('Ctrl Pts',(-13.0901089262946,-13.1665060684571,
-336.208771918995)) ;
#46242=CARTESIAN_POINT('Ctrl Pts',(-13.0079642387823,-13.2476677259745,
-336.20731230549)) ;
#46243=CARTESIAN_POINT('Ctrl Pts',(-12.6602195939087,-13.5848978849575,
-336.201227786037)) ;
#46244=CARTESIAN_POINT('Ctrl Pts',(-12.3877740321692,-13.8337871335208,
-336.196687072756)) ;
#46245=CARTESIAN_POINT('Ctrl Pts',(-11.7374178303764,-14.3932836272165,
-336.186166061244)) ;
#46246=CARTESIAN_POINT('Ctrl Pts',(-11.3542883848001,-14.6974054206845,
-336.180199361344)) ;
#46247=CARTESIAN_POINT('Ctrl Pts',(-10.712914175235,-15.1664554625799,-336.170356233692)) ;
#46248=CARTESIAN_POINT('Ctrl Pts',(-10.4618096435821,-15.340744435252,-336.166537845105)) ;
#46249=CARTESIAN_POINT('Ctrl Pts',(-10.0833784872978,-15.5897950106231,
-336.160807458966)) ;
#46250=CARTESIAN_POINT('Ctrl Pts',(-9.95927826892772,-15.6693652223449,
-336.158932175915)) ;
#46251=CARTESIAN_POINT('Ctrl Pts',(-9.72904969648478,-15.8131424081075,
-336.155458276502)) ;
#46252=CARTESIAN_POINT('Ctrl Pts',(-9.62320013510729,-15.877780069158,-336.153863075395)) ;
#46253=CARTESIAN_POINT('Ctrl Pts',(-9.38366580608846,-16.0207779117035,
-336.150256844704)) ;
#46254=CARTESIAN_POINT('Ctrl Pts',(-9.24963168175542,-16.0985347938967,
-336.148241439955)) ;
#46255=CARTESIAN_POINT('Ctrl Pts',(-8.88244010399662,-16.3054529315315,
-336.142727129234)) ;
#46256=CARTESIAN_POINT('Ctrl Pts',(-8.64744983524044,-16.4312856588522,
-336.13920531375)) ;
#46257=CARTESIAN_POINT('Ctrl Pts',(-7.82969122251205,-16.846776631901,-336.12699341413)) ;
#46258=CARTESIAN_POINT('Ctrl Pts',(-7.23445637700788,-17.1108323764909,
-336.118164196097)) ;
#46259=CARTESIAN_POINT('Ctrl Pts',(-6.37277447255356,-17.440070897112,-336.105812533271)) ;
#46260=CARTESIAN_POINT('Ctrl Pts',(-6.11685910743164,-17.5314677811533,
-336.102198629731)) ;
#46261=CARTESIAN_POINT('Ctrl Pts',(-5.77177263480566,-17.6462346130356,
-336.097436552554)) ;
#46262=CARTESIAN_POINT('Ctrl Pts',(-5.68430087336002,-17.674605483054,-336.09623895615)) ;
#46263=CARTESIAN_POINT('Ctrl Pts',(-5.53975546378756,-17.7203037732492,
-336.094277652373)) ;
#46264=CARTESIAN_POINT('Ctrl Pts',(-5.48280277303901,-17.7380080671276,
-336.093509447661)) ;
#46265=CARTESIAN_POINT('Ctrl Pts',(-5.34844881763035,-17.7790643946202,
-336.091708281867)) ;
#46266=CARTESIAN_POINT('Ctrl Pts',(-5.27097849655186,-17.8021858550007,
-336.090678104859)) ;
#46267=CARTESIAN_POINT('Ctrl Pts',(-5.01999843318225,-17.8753103596158,
-336.087364379375)) ;
#46268=CARTESIAN_POINT('Ctrl Pts',(-4.84590935068426,-17.9232884117445,
-336.08510232428)) ;
#46269=CARTESIAN_POINT('Ctrl Pts',(-4.57238560123841,-17.9943936403405,
-336.081588115083)) ;
#46270=CARTESIAN_POINT('Ctrl Pts',(-4.47341320665446,-18.0192532274795,
-336.080324649826)) ;
#46271=CARTESIAN_POINT('Ctrl Pts',(-3.8211484267994,-18.1773819480632,-336.072039446597)) ;
#46272=CARTESIAN_POINT('Ctrl Pts',(-3.26218292272399,-18.2859660395737,
-336.065125083936)) ;
#46273=CARTESIAN_POINT('Ctrl Pts',(-2.34258864956133,-18.4210920620614,
-336.053659245367)) ;
#46274=CARTESIAN_POINT('Ctrl Pts',(-1.98461423367481,-18.4630891196864,
-336.049176280948)) ;
#46275=CARTESIAN_POINT('Ctrl Pts',(-1.46960006791021,-18.50835793268,-336.042650674601)) ;
#46276=CARTESIAN_POINT('Ctrl Pts',(-1.31338743287277,-18.5200985709464,
-336.040661642094)) ;
#46277=CARTESIAN_POINT('Ctrl Pts',(-1.03318318949492,-18.5375951378299,
-336.037073880576)) ;
#46278=CARTESIAN_POINT('Ctrl Pts',(-0.909246943366904,-18.5440872232164,
-336.035480019602)) ;
#46279=CARTESIAN_POINT('Ctrl Pts',(-0.639313325296582,-18.5555144102518,
-336.031992632679)) ;
#46280=CARTESIAN_POINT('Ctrl Pts',(-0.493303939459485,-18.5599700349355,
-336.030096114867)) ;
#46281=CARTESIAN_POINT('Ctrl Pts',(-0.0509525005324996,-18.5682452195222,
-336.024319556377)) ;
#46282=CARTESIAN_POINT('Ctrl Pts',(0.24544195023237,-18.5666928749577,-336.020406457729)) ;
#46283=CARTESIAN_POINT('Ctrl Pts',(1.00222184847998,-18.5446040173945,-336.010325388514)) ;
#46284=CARTESIAN_POINT('Ctrl Pts',(1.46211167608331,-18.5140221158868,-336.004111424955)) ;
#46285=CARTESIAN_POINT('Ctrl Pts',(2.04506559064242,-18.4533985866081,-335.996219226975)) ;
#46286=CARTESIAN_POINT('Ctrl Pts',(2.16961129492292,-18.4391702500714,-335.994532517905)) ;
#46287=CARTESIAN_POINT('Ctrl Pts',(2.61270404909148,-18.3839990697948,-335.988537713386)) ;
#46288=CARTESIAN_POINT('Ctrl Pts',(2.93032208277452,-18.336053486963,-335.984250645725)) ;
#46289=CARTESIAN_POINT('Ctrl Pts',(3.34260043567125,-18.2628322302956,-335.978759624777)) ;
#46290=CARTESIAN_POINT('Ctrl Pts',(3.43852840371608,-18.2450141463756,-335.977487313044)) ;
#46291=CARTESIAN_POINT('Ctrl Pts',(3.59945729527878,-18.213808227023,-335.97536438761)) ;
#46292=CARTESIAN_POINT('Ctrl Pts',(3.66453486222498,-18.2008265534706,-335.974509155172)) ;
#46293=CARTESIAN_POINT('Ctrl Pts',(3.80863316193467,-18.1712776475879,-335.972623191489)) ;
#46294=CARTESIAN_POINT('Ctrl Pts',(3.8876180935596,-18.1545433291696,-335.97159436539)) ;
#46295=CARTESIAN_POINT('Ctrl Pts',(4.14220557159471,-18.0988669405723,-335.96829079451)) ;
#46296=CARTESIAN_POINT('Ctrl Pts',(4.31735232574465,-18.0578880444827,-335.966037363104)) ;
#46297=CARTESIAN_POINT('Ctrl Pts',(4.76972153831358,-17.9450899613946,-335.960239603275)) ;
#46298=CARTESIAN_POINT('Ctrl Pts',(5.04592731089906,-17.8693904559283,-335.956721217965)) ;
#46299=CARTESIAN_POINT('Ctrl Pts',(5.99271267098134,-17.5862026731802,-335.944607124163)) ;
#46300=CARTESIAN_POINT('Ctrl Pts',(6.65320780109245,-17.3471022097047,-335.936040546542)) ;
#46301=CARTESIAN_POINT('Ctrl Pts',(7.45852865400606,-17.0027971710733,-335.925022604997)) ;
#46302=CARTESIAN_POINT('Ctrl Pts',(7.61751325109287,-16.9321662247471,-335.922820081268)) ;
#46303=CARTESIAN_POINT('Ctrl Pts',(7.88979697982699,-16.8065895008203,-335.918996614525)) ;
#46304=CARTESIAN_POINT('Ctrl Pts',(8.0035731088039,-16.7527061835142,-335.917383274711)) ;
#46305=CARTESIAN_POINT('Ctrl Pts',(8.23972513215248,-16.6379119077236,-335.914000877156)) ;
#46306=CARTESIAN_POINT('Ctrl Pts',(8.36199413672027,-16.576798149584,-335.912230432631)) ;
#46307=CARTESIAN_POINT('Ctrl Pts',(8.6953331183131,-16.405558672651,-335.907350470768)) ;
#46308=CARTESIAN_POINT('Ctrl Pts',(8.90497699432193,-16.2927148687468,-335.904221882818)) ;
#46309=CARTESIAN_POINT('Ctrl Pts',(9.71993570488659,-15.8336222114342,-335.891834506938)) ;
#46310=CARTESIAN_POINT('Ctrl Pts',(10.307714166003,-15.4574177974468,-335.882380570414)) ;
#46311=CARTESIAN_POINT('Ctrl Pts',(11.1214919922946,-14.8694636076743,-335.868911013355)) ;
#46312=CARTESIAN_POINT('Ctrl Pts',(11.3655652125875,-14.6837481655826,-335.864821910574)) ;
#46313=CARTESIAN_POINT('Ctrl Pts',(11.6797860764473,-14.4321271478439,-335.8595452399)) ;
#46314=CARTESIAN_POINT('Ctrl Pts',(11.7541798796942,-14.3716022835743,-335.858295089916)) ;
#46315=CARTESIAN_POINT('Ctrl Pts',(11.8791140339333,-14.2683401004377,-335.856196600657)) ;
#46316=CARTESIAN_POINT('Ctrl Pts',(11.9299007895305,-14.225904070989,-335.855343909202)) ;
#46317=CARTESIAN_POINT('Ctrl Pts',(12.0429146983721,-14.130441915041,-335.853447692923)) ;
#46318=CARTESIAN_POINT('Ctrl Pts',(12.1050205720342,-14.0772745985223,-335.85240625014)) ;
#46319=CARTESIAN_POINT('Ctrl Pts',(12.3076670394367,-13.9014612364561,-335.84900657256)) ;
#46320=CARTESIAN_POINT('Ctrl Pts',(12.446710883384,-13.7771071299423,-335.846671385337)) ;
#46321=CARTESIAN_POINT('Ctrl Pts',(12.807325210481,-13.4446753640954,-335.840576928652)) ;
#46322=CARTESIAN_POINT('Ctrl Pts',(13.0257010845447,-13.2332152714803,-335.836846826742)) ;
#46323=CARTESIAN_POINT('Ctrl Pts',(13.7055778663635,-12.5417274434548,-335.824964477589)) ;
#46324=CARTESIAN_POINT('Ctrl Pts',(14.1464919548063,-12.0421989850211,-335.816826809427)) ;
#46325=CARTESIAN_POINT('Ctrl Pts',(14.6699574299694,-11.380618175491,-335.806221125627)) ;
#46326=CARTESIAN_POINT('Ctrl Pts',(14.7782873830265,-11.2395882015158,-335.803970938718)) ;
#46327=CARTESIAN_POINT('Ctrl Pts',(14.9601458050896,-10.9956592670613,-335.800092800337)) ;
#46328=CARTESIAN_POINT('Ctrl Pts',(15.0346796097078,-10.8935253341977,-335.79847308245)) ;
#46329=CARTESIAN_POINT('Ctrl Pts',(15.1868012449538,-10.6805371285541,-335.795102755632)) ;
#46330=CARTESIAN_POINT('Ctrl Pts',(15.2642322371292,-10.5695799137498,-335.793351028236)) ;
#46331=CARTESIAN_POINT('Ctrl Pts',(15.4700402476174,-10.2676817847379,-335.788595340753)) ;
#46332=CARTESIAN_POINT('Ctrl Pts',(15.5960919032851,-10.0751849379759,-335.785573970629)) ;
#46333=CARTESIAN_POINT('Ctrl Pts',(15.8040771356618,-9.74430519000732,-335.780402828035)) ;
#46334=CARTESIAN_POINT('Ctrl Pts',(15.8878500417749,-9.60710980012188,-335.778265068858)) ;
#46335=CARTESIAN_POINT('Ctrl Pts',(16.2715385199525,-8.9599938442345,-335.768220117827)) ;
#46336=CARTESIAN_POINT('Ctrl Pts',(16.5487527548252,-8.43701579263089,-335.760200309543)) ;
#46337=CARTESIAN_POINT('Ctrl Pts',(16.8908789576445,-7.70958993684472,-335.749434943328)) ;
#46338=CARTESIAN_POINT('Ctrl Pts',(16.9779308737153,-7.51594521258067,-335.746606649694)) ;
#46339=CARTESIAN_POINT('Ctrl Pts',(17.1101854561587,-7.20771865244227,-335.742184867733)) ;
#46340=CARTESIAN_POINT('Ctrl Pts',(17.1576018031395,-7.09410705839913,-335.740571962958)) ;
#46341=CARTESIAN_POINT('Ctrl Pts',(17.2278428871278,-6.9209818517865,-335.738144291973)) ;
#46342=CARTESIAN_POINT('Ctrl Pts',(17.2514968684681,-6.86180851861114,-335.737319828005)) ;
#46343=CARTESIAN_POINT('Ctrl Pts',(17.300265986958,-6.73796034533484,-335.735606211945)) ;
#46344=CARTESIAN_POINT('Ctrl Pts',(17.3253241798233,-6.67326418608659,-335.734717908428)) ;
#46345=CARTESIAN_POINT('Ctrl Pts',(17.3914889007665,-6.49955283060892,-335.732349387754)) ;
#46346=CARTESIAN_POINT('Ctrl Pts',(17.4319329461844,-6.39028849167808,-335.730876997474)) ;
#46347=CARTESIAN_POINT('Ctrl Pts',(17.6036438507278,-5.91262769005917,-335.724502665087)) ;
#46348=CARTESIAN_POINT('Ctrl Pts',(17.7242808599766,-5.54051553966805,-335.719695670775)) ;
#46349=CARTESIAN_POINT('Ctrl Pts',(18.026714909058,-4.49628245723896,-335.70636980271)) ;
#46350=CARTESIAN_POINT('Ctrl Pts',(18.182600991019,-3.81733244457233,-335.697872688997)) ;
#46351=CARTESIAN_POINT('Ctrl Pts',(18.3295148688494,-2.95871905123448,-335.686916465868)) ;
#46352=CARTESIAN_POINT('Ctrl Pts',(18.3565928806566,-2.78579098872454,-335.684700782015)) ;
#46353=CARTESIAN_POINT('Ctrl Pts',(18.3989566947429,-2.48772521732273,-335.680862270824)) ;
#46354=CARTESIAN_POINT('Ctrl Pts',(18.4154206037213,-2.36276705304418,-335.679247219785)) ;
#46355=CARTESIAN_POINT('Ctrl Pts',(18.4470366554315,-2.10235864654082,-335.675868449205)) ;
#46356=CARTESIAN_POINT('Ctrl Pts',(18.4619722249938,-1.9668896109491,-335.674103419246)) ;
#46357=CARTESIAN_POINT('Ctrl Pts',(18.498667463784,-1.59667642803706,-335.669259552181)) ;
#46358=CARTESIAN_POINT('Ctrl Pts',(18.5174497915935,-1.3616631154694,-335.666162133276)) ;
#46359=CARTESIAN_POINT('Ctrl Pts',(18.5365593472123,-1.04725680702123,-335.661991743979)) ;
#46360=CARTESIAN_POINT('Ctrl Pts',(18.5408603713437,-0.968129729065171,
-335.660939964508)) ;
#46361=CARTESIAN_POINT('Ctrl Pts',(18.5446545938163,-0.888979976461629,
-335.659885874007)) ;
#46362=CARTESIAN_POINT('Ctrl Pts',(18.5446545934131,-0.888979984870909,
-335.363183819487)) ;
#46363=CARTESIAN_POINT('Ctrl Pts',(18.5274773631996,-1.24730728875046,-335.367987381273)) ;
#46364=CARTESIAN_POINT('Ctrl Pts',(18.4999170091639,-1.6050846689973,-335.372827203657)) ;
#46365=CARTESIAN_POINT('Ctrl Pts',(18.4457968108924,-2.11438034440564,-335.379722413713)) ;
#46366=CARTESIAN_POINT('Ctrl Pts',(18.4276999900379,-2.26669304111968,-335.381785006543)) ;
#46367=CARTESIAN_POINT('Ctrl Pts',(18.3707061504084,-2.70043792830454,-335.387647964213)) ;
#46368=CARTESIAN_POINT('Ctrl Pts',(18.3272339112023,-2.9812257895604,-335.391430876734)) ;
#46369=CARTESIAN_POINT('Ctrl Pts',(18.2623382693532,-3.34496505956417,-335.396272411271)) ;
#46370=CARTESIAN_POINT('Ctrl Pts',(18.2467612735903,-3.42892014569708,-335.397385731343)) ;
#46371=CARTESIAN_POINT('Ctrl Pts',(18.2179264561967,-3.57856756232574,-335.399360943711)) ;
#46372=CARTESIAN_POINT('Ctrl Pts',(18.204891069443,-3.64430121574535,-335.400225322137)) ;
#46373=CARTESIAN_POINT('Ctrl Pts',(18.1758898581029,-3.78650628010723,-335.402087486718)) ;
#46374=CARTESIAN_POINT('Ctrl Pts',(18.1597967253699,-3.86295027907294,-335.403083836486)) ;
#46375=CARTESIAN_POINT('Ctrl Pts',(18.1084913710847,-4.09924775802851,-335.406152095274)) ;
#46376=CARTESIAN_POINT('Ctrl Pts',(18.0716472468421,-4.25873899896801,-335.408206651624)) ;
#46377=CARTESIAN_POINT('Ctrl Pts',(17.9125266788189,-4.90825317797366,-335.416539785052)) ;
#46378=CARTESIAN_POINT('Ctrl Pts',(17.7723889353657,-5.39367732076572,-335.422694136307)) ;
#46379=CARTESIAN_POINT('Ctrl Pts',(17.4605826181039,-6.32879280746731,-335.43477852423)) ;
#46380=CARTESIAN_POINT('Ctrl Pts',(17.2908779858376,-6.77872414270108,-335.440700389258)) ;
#46381=CARTESIAN_POINT('Ctrl Pts',(17.0317533885978,-7.39244777852428,-335.449064846342)) ;
#46382=CARTESIAN_POINT('Ctrl Pts',(16.9570450434212,-7.56224377337838,-335.451409589574)) ;
#46383=CARTESIAN_POINT('Ctrl Pts',(16.8271948528679,-7.84576164285713,-335.455381319778)) ;
#46384=CARTESIAN_POINT('Ctrl Pts',(16.7734135892526,-7.96009163788595,-335.456998628237)) ;
#46385=CARTESIAN_POINT('Ctrl Pts',(16.6607630390207,-8.19335601743633,-335.460331702028)) ;
#46386=CARTESIAN_POINT('Ctrl Pts',(16.6017771400517,-8.31222615191562,-335.462048236235)) ;
#46387=CARTESIAN_POINT('Ctrl Pts',(16.4437758770691,-8.62224284836822,-335.466572938997)) ;
#46388=CARTESIAN_POINT('Ctrl Pts',(16.342701735866,-8.812317320173,-335.469395593491)) ;
#46389=CARTESIAN_POINT('Ctrl Pts',(16.1058578282291,-9.23961739762066,-335.475848570329)) ;
#46390=CARTESIAN_POINT('Ctrl Pts',(15.9681089109282,-9.47568907453852,-335.479490937868)) ;
#46391=CARTESIAN_POINT('Ctrl Pts',(15.6418076838945,-10.0075643369964,-335.487853451055)) ;
#46392=CARTESIAN_POINT('Ctrl Pts',(15.4499828815418,-10.3012387707321,-335.492585545034)) ;
#46393=CARTESIAN_POINT('Ctrl Pts',(15.1958746987544,-10.6671871760292,-335.498582258604)) ;
#46394=CARTESIAN_POINT('Ctrl Pts',(15.1411975319602,-10.7446557606444,-335.499857480419)) ;
#46395=CARTESIAN_POINT('Ctrl Pts',(14.8982625584874,-11.0833178125441,-335.505453372739)) ;
#46396=CARTESIAN_POINT('Ctrl Pts',(14.7038218711425,-11.3400081181365,-335.509751453207)) ;
#46397=CARTESIAN_POINT('Ctrl Pts',(14.4417884144324,-11.6678531738936,-335.515255348585)) ;
#46398=CARTESIAN_POINT('Ctrl Pts',(14.3801703610754,-11.7437111136783,-335.51652981205)) ;
#46399=CARTESIAN_POINT('Ctrl Pts',(14.2757002239312,-11.8702690999123,-335.518655124242)) ;
#46400=CARTESIAN_POINT('Ctrl Pts',(14.2331700339669,-11.9212321597634,-335.519510617606)) ;
#46401=CARTESIAN_POINT('Ctrl Pts',(14.1383659690171,-12.0336033840814,-335.521395654992)) ;
#46402=CARTESIAN_POINT('Ctrl Pts',(14.085963553445,-12.0949011353684,-335.522423310406)) ;
#46403=CARTESIAN_POINT('Ctrl Pts',(13.9157946651901,-12.2913503115116,-335.525718106856)) ;
#46404=CARTESIAN_POINT('Ctrl Pts',(13.7964695249517,-12.4251383288522,-335.527964089446)) ;
#46405=CARTESIAN_POINT('Ctrl Pts',(13.4826055391519,-12.7669476885797,-335.533735307216)) ;
#46406=CARTESIAN_POINT('Ctrl Pts',(13.2851841418668,-12.9722584054192,-335.537234879398)) ;
#46407=CARTESIAN_POINT('Ctrl Pts',(12.582090180083,-13.6705578557767,-335.54938275708)) ;
#46408=CARTESIAN_POINT('Ctrl Pts',(12.053080119611,-14.1391797697511,-335.558000380931)) ;
#46409=CARTESIAN_POINT('Ctrl Pts',(11.3761172157347,-14.6732007749142,-335.568848770328)) ;
#46410=CARTESIAN_POINT('Ctrl Pts',(11.2523524476432,-14.768325165274,-335.570824037677)) ;
#46411=CARTESIAN_POINT('Ctrl Pts',(11.0261121421737,-14.9377160827822,-335.574423301638)) ;
#46412=CARTESIAN_POINT('Ctrl Pts',(10.9240486928393,-15.0125171388613,-335.576042884117)) ;
#46413=CARTESIAN_POINT('Ctrl Pts',(10.7136513598514,-15.1634330253873,-335.579374142734)) ;
#46414=CARTESIAN_POINT('Ctrl Pts',(10.6052518880291,-15.2394441796742,-335.581086520098)) ;
#46415=CARTESIAN_POINT('Ctrl Pts',(10.3199258518366,-15.434999842403,-335.585584039716)) ;
#46416=CARTESIAN_POINT('Ctrl Pts',(10.1417339144932,-15.5526628807797,-335.588383337061)) ;
#46417=CARTESIAN_POINT('Ctrl Pts',(9.64470771898151,-15.8686826094302,-335.596161233655)) ;
#46418=CARTESIAN_POINT('Ctrl Pts',(9.32182533424749,-16.0604808817661,-335.60118204392)) ;
#46419=CARTESIAN_POINT('Ctrl Pts',(8.43138312839876,-16.553516424503,-335.614865367491)) ;
#46420=CARTESIAN_POINT('Ctrl Pts',(7.85364586991162,-16.8353014189392,-335.623581211539)) ;
#46421=CARTESIAN_POINT('Ctrl Pts',(7.16059530128688,-17.1298752943899,-335.633485576558)) ;
#46422=CARTESIAN_POINT('Ctrl Pts',(7.05833585889369,-17.1722639051843,-335.634932838381)) ;
#46423=CARTESIAN_POINT('Ctrl Pts',(6.8985797834561,-17.236817927763,-335.637168539028)) ;
#46424=CARTESIAN_POINT('Ctrl Pts',(6.84134158923589,-17.2596158874615,-335.637964534974)) ;
#46425=CARTESIAN_POINT('Ctrl Pts',(6.71679082019853,-17.308507508772,-335.639684892952)) ;
#46426=CARTESIAN_POINT('Ctrl Pts',(6.64943739023208,-17.334494325333,-335.640607859626)) ;
#46427=CARTESIAN_POINT('Ctrl Pts',(6.45942240965936,-17.4065369380194,-335.643193163933)) ;
#46428=CARTESIAN_POINT('Ctrl Pts',(6.33642233361407,-17.45168811715,-335.644845054755)) ;
#46429=CARTESIAN_POINT('Ctrl Pts',(6.04552526660874,-17.5549904965224,-335.648711106168)) ;
#46430=CARTESIAN_POINT('Ctrl Pts',(5.8772509338337,-17.6120410142795,-335.650915890014)) ;
#46431=CARTESIAN_POINT('Ctrl Pts',(5.17102826160835,-17.8402248897353,-335.660078304486)) ;
#46432=CARTESIAN_POINT('Ctrl Pts',(4.62623668279112,-17.9891937885443,-335.666937277826)) ;
#46433=CARTESIAN_POINT('Ctrl Pts',(3.72117205385357,-18.1928361365434,-335.678378221337)) ;
#46434=CARTESIAN_POINT('Ctrl Pts',(3.36457578229734,-18.2621476583946,-335.682895061056)) ;
#46435=CARTESIAN_POINT('Ctrl Pts',(2.85058591928489,-18.3464852148715,-335.68946799442)) ;
#46436=CARTESIAN_POINT('Ctrl Pts',(2.69467594077538,-18.3700321528772,-335.691469659938)) ;
#46437=CARTESIAN_POINT('Ctrl Pts',(2.4154879284857,-18.4085668640108,-335.695070752324)) ;
#46438=CARTESIAN_POINT('Ctrl Pts',(2.29232363194527,-18.4243091657438,-335.696665151404)) ;
#46439=CARTESIAN_POINT('Ctrl Pts',(2.02469447952201,-18.4557911525432,-335.700142995389)) ;
#46440=CARTESIAN_POINT('Ctrl Pts',(1.88018397643718,-18.4710725983935,-335.702029310084)) ;
#46441=CARTESIAN_POINT('Ctrl Pts',(1.44555132452498,-18.5118799003401,-335.70772793962)) ;
#46442=CARTESIAN_POINT('Ctrl Pts',(1.15499370184704,-18.5322773837841,-335.71157194813)) ;
#46443=CARTESIAN_POINT('Ctrl Pts',(0.418580504240088,-18.5665879464058,
-335.721384087056)) ;
#46444=CARTESIAN_POINT('Ctrl Pts',(-0.0275189157587249,-18.5712853371342,
-335.727394752062)) ;
#46445=CARTESIAN_POINT('Ctrl Pts',(-0.547625919799585,-18.5580205132199,
-335.734402122302)) ;
#46446=CARTESIAN_POINT('Ctrl Pts',(-0.621887209276719,-18.5556804191639,
-335.735402516399)) ;
#46447=CARTESIAN_POINT('Ctrl Pts',(-0.796446928902621,-18.5491306764911,
-335.737752723704)) ;
#46448=CARTESIAN_POINT('Ctrl Pts',(-0.896729258491385,-18.5445531952714,
-335.739101856017)) ;
#46449=CARTESIAN_POINT('Ctrl Pts',(-1.29584885458761,-18.5230899776942,
-335.744462456376)) ;
#46450=CARTESIAN_POINT('Ctrl Pts',(-1.59429641616559,-18.4997920571509,
-335.74845173471)) ;
#46451=CARTESIAN_POINT('Ctrl Pts',(-1.98680889456779,-18.4595818814092,
-335.753622882504)) ;
#46452=CARTESIAN_POINT('Ctrl Pts',(-2.08149144948029,-18.4491454057727,
-335.754864395207)) ;
#46453=CARTESIAN_POINT('Ctrl Pts',(-2.24175311720873,-18.4302309839971,
-335.756953440762)) ;
#46454=CARTESIAN_POINT('Ctrl Pts',(-2.30737476773423,-18.4221305194097,
-335.757805221927)) ;
#46455=CARTESIAN_POINT('Ctrl Pts',(-2.45445262988278,-18.4031767462576,
-335.759705817049)) ;
#46456=CARTESIAN_POINT('Ctrl Pts',(-2.53588271326722,-18.3921328550058,
-335.760752476517)) ;
#46457=CARTESIAN_POINT('Ctrl Pts',(-2.8046982342454,-18.3538557665272,-335.764192751267)) ;
#46458=CARTESIAN_POINT('Ctrl Pts',(-2.991740622067,-18.3242964930456,-335.766562565817)) ;
#46459=CARTESIAN_POINT('Ctrl Pts',(-3.48533201525628,-18.2385327238313,
-335.77278579663)) ;
#46460=CARTESIAN_POINT('Ctrl Pts',(-3.79097429135877,-18.1774621329308,
-335.776608593526)) ;
#46461=CARTESIAN_POINT('Ctrl Pts',(-4.71916399508871,-17.9675701867732,
-335.788267426841)) ;
#46462=CARTESIAN_POINT('Ctrl Pts',(-5.33567720882668,-17.794230384558,-335.79609392181)) ;
#46463=CARTESIAN_POINT('Ctrl Pts',(-6.11643702438022,-17.5304762243907,
-335.806443482945)) ;
#46464=CARTESIAN_POINT('Ctrl Pts',(-6.28998338880483,-17.4689583931982,
-335.808771247093)) ;
#46465=CARTESIAN_POINT('Ctrl Pts',(-6.58082767941278,-17.3609652722419,
-335.812723215026)) ;
#46466=CARTESIAN_POINT('Ctrl Pts',(-6.69861897412264,-17.3158572388618,
-335.814337974192)) ;
#46467=CARTESIAN_POINT('Ctrl Pts',(-6.93970998732344,-17.2207035160282,
-335.817673334951)) ;
#46468=CARTESIAN_POINT('Ctrl Pts',(-7.06294976816604,-17.1705254667594,
-335.819394784002)) ;
#46469=CARTESIAN_POINT('Ctrl Pts',(-7.38602440691943,-17.0349162500238,
-335.823951632333)) ;
#46470=CARTESIAN_POINT('Ctrl Pts',(-7.58491684124977,-16.9472937201395,
-335.826801912308)) ;
#46471=CARTESIAN_POINT('Ctrl Pts',(-7.91181944834641,-16.7963682684946,
-335.831558958492)) ;
#46472=CARTESIAN_POINT('Ctrl Pts',(-8.04071964325235,-16.7350441155975,
-335.833453609637)) ;
#46473=CARTESIAN_POINT('Ctrl Pts',(-8.60617386456888,-16.4579884277976,
-335.841843707323)) ;
#46474=CARTESIAN_POINT('Ctrl Pts',(-9.03484927405166,-16.2266172929978,
-335.84841857797)) ;
#46475=CARTESIAN_POINT('Ctrl Pts',(-9.55214617044281,-15.9205535669559,
-335.856507433423)) ;
#46476=CARTESIAN_POINT('Ctrl Pts',(-9.6498233279977,-15.8615393986178,-335.858041525314)) ;
#46477=CARTESIAN_POINT('Ctrl Pts',(-10.0011107363825,-15.6448540810405,
-335.863576908721)) ;
#46478=CARTESIAN_POINT('Ctrl Pts',(-10.2514523652854,-15.4819701660421,
-335.86755685313)) ;
#46479=CARTESIAN_POINT('Ctrl Pts',(-10.5763018442078,-15.2592728362574,
-335.872718632993)) ;
#46480=CARTESIAN_POINT('Ctrl Pts',(-10.654431945796,-15.2048231867766,-335.873959822097)) ;
#46481=CARTESIAN_POINT('Ctrl Pts',(-10.7860910685688,-15.1115555229098,
-335.876048514775)) ;
#46482=CARTESIAN_POINT('Ctrl Pts',(-10.8398378396984,-15.0730483480079,
-335.876900262769)) ;
#46483=CARTESIAN_POINT('Ctrl Pts',(-10.9599339440802,-14.9860302496266,
-335.8788010264)) ;
#46484=CARTESIAN_POINT('Ctrl Pts',(-11.0261690136788,-14.9373642791632,
-335.879847884793)) ;
#46485=CARTESIAN_POINT('Ctrl Pts',(-11.2440096604312,-14.7750682412346,
-335.883289717874)) ;
#46486=CARTESIAN_POINT('Ctrl Pts',(-11.394199259038,-14.6595572325294,-335.885660862677)) ;
#46487=CARTESIAN_POINT('Ctrl Pts',(-11.7869160745852,-14.347836459618,-335.891889079029)) ;
#46488=CARTESIAN_POINT('Ctrl Pts',(-12.0263114861197,-14.1477784177621,
-335.895715474379)) ;
#46489=CARTESIAN_POINT('Ctrl Pts',(-12.741458630008,-13.5188704277034,-335.907383067258)) ;
#46490=CARTESIAN_POINT('Ctrl Pts',(-13.2001604398673,-13.0713575821924,
-335.915214904207)) ;
#46491=CARTESIAN_POINT('Ctrl Pts',(-13.7595132417925,-12.466116006806,-335.925565434011)) ;
#46492=CARTESIAN_POINT('Ctrl Pts',(-13.8821984303031,-12.3293478958293,
-335.927888319434)) ;
#46493=CARTESIAN_POINT('Ctrl Pts',(-14.0856125680081,-12.095698048235,-335.931834616302)) ;
#46494=CARTESIAN_POINT('Ctrl Pts',(-14.1674210769188,-11.9997738589716,
-335.933448650069)) ;
#46495=CARTESIAN_POINT('Ctrl Pts',(-14.3336223336374,-11.80082639626,-335.936784714158)) ;
#46496=CARTESIAN_POINT('Ctrl Pts',(-14.417896388251,-11.6977133027227,-335.938507614875)) ;
#46497=CARTESIAN_POINT('Ctrl Pts',(-14.6371428266436,-11.4234864662596,
-335.943073960606)) ;
#46498=CARTESIAN_POINT('Ctrl Pts',(-14.7702241001134,-11.2508876513431,
-335.945932403682)) ;
#46499=CARTESIAN_POINT('Ctrl Pts',(-15.0662739311693,-10.8526195284953,
-335.952489223089)) ;
#46500=CARTESIAN_POINT('Ctrl Pts',(-15.227268150274,-10.6255477530029,-335.956200277765)) ;
#46501=CARTESIAN_POINT('Ctrl Pts',(-15.614263666664,-10.0528472290745,-335.965466934884)) ;
#46502=CARTESIAN_POINT('Ctrl Pts',(-15.8339549721789,-9.70313540812938,
-335.971045912676)) ;
#46503=CARTESIAN_POINT('Ctrl Pts',(-16.2141427265182,-9.05059507603661,
-335.981193433851)) ;
#46504=CARTESIAN_POINT('Ctrl Pts',(-16.378267773699,-8.75008806551203,-335.985769092919)) ;
#46505=CARTESIAN_POINT('Ctrl Pts',(-16.5789288923932,-8.35723495954348,
-335.991555631055)) ;
#46506=CARTESIAN_POINT('Ctrl Pts',(-16.623164444904,-8.26889734288747,-335.992844266301)) ;
#46507=CARTESIAN_POINT('Ctrl Pts',(-16.6959944930646,-8.12051045233272,
-335.994985360415)) ;
#46508=CARTESIAN_POINT('Ctrl Pts',(-16.7249751591501,-8.06065308030398,
-335.995842634557)) ;
#46509=CARTESIAN_POINT('Ctrl Pts',(-16.7881255011991,-7.928413964869,-335.997721870492)) ;
#46510=CARTESIAN_POINT('Ctrl Pts',(-16.8221499134748,-7.85596449549852,
-335.998742049887)) ;
#46511=CARTESIAN_POINT('Ctrl Pts',(-16.9292489038866,-7.62402822017504,
-336.001981353258)) ;
#46512=CARTESIAN_POINT('Ctrl Pts',(-17.0005320599442,-7.46372458089711,
-336.004180285562)) ;
#46513=CARTESIAN_POINT('Ctrl Pts',(-17.1777265373408,-7.04953026332026,
-336.009785651805)) ;
#46514=CARTESIAN_POINT('Ctrl Pts',(-17.2802865345593,-6.79425224676871,
-336.013168141533)) ;
#46515=CARTESIAN_POINT('Ctrl Pts',(-17.6330566245216,-5.85646254593097,
-336.02545477956)) ;
#46516=CARTESIAN_POINT('Ctrl Pts',(-17.8488030819397,-5.16169234639476,
-336.034318009026)) ;
#46517=CARTESIAN_POINT('Ctrl Pts',(-18.0602310403077,-4.30653922511104,
-336.045405715722)) ;
#46518=CARTESIAN_POINT('Ctrl Pts',(-18.0953384416368,-4.15655529482406,
-336.047355614413)) ;
#46519=CARTESIAN_POINT('Ctrl Pts',(-18.1557819366841,-3.88303735394985,
-336.050923885749)) ;
#46520=CARTESIAN_POINT('Ctrl Pts',(-18.1817336200057,-3.75964883237853,
-336.052538113747)) ;
#46521=CARTESIAN_POINT('Ctrl Pts',(-18.2325005158333,-3.50544577534052,
-336.055873987054)) ;
#46522=CARTESIAN_POINT('Ctrl Pts',(-18.2571694661401,-3.37460933522918,
-336.05759649659)) ;
#46523=CARTESIAN_POINT('Ctrl Pts',(-18.3184733648802,-3.02910139661202,
-336.062160282979)) ;
#46524=CARTESIAN_POINT('Ctrl Pts',(-18.3527422708443,-2.81403137325167,
-336.065016526234)) ;
#46525=CARTESIAN_POINT('Ctrl Pts',(-18.4221286336303,-2.32313678465176,
-336.071566941386)) ;
#46526=CARTESIAN_POINT('Ctrl Pts',(-18.4548495404508,-2.04702611783494,
-336.075273752073)) ;
#46527=CARTESIAN_POINT('Ctrl Pts',(-18.5207255910791,-1.359295863721,-336.084535941677)) ;
#46528=CARTESIAN_POINT('Ctrl Pts',(-18.5463729221208,-0.94710751380241,
-336.090114790525)) ;
#46529=CARTESIAN_POINT('Ctrl Pts',(-18.5681415683955,-0.191153551558178,
-336.100276631728)) ;
#46530=CARTESIAN_POINT('Ctrl Pts',(-18.5685008398542,0.152310163944746,
-336.104866549654)) ;
#46531=CARTESIAN_POINT('Ctrl Pts',(-18.5567027574909,0.594139617409694,
-336.110664000756)) ;
#46532=CARTESIAN_POINT('Ctrl Pts',(-18.5532861372631,0.692670675679252,
-336.111949918189)) ;
#46533=CARTESIAN_POINT('Ctrl Pts',(-18.5462519442838,0.857588271429485,
-336.114087977898)) ;
#46534=CARTESIAN_POINT('Ctrl Pts',(-18.5430623035918,0.923990944389028,
-336.11494490271)) ;
#46535=CARTESIAN_POINT('Ctrl Pts',(-18.535240397903,1.07041457494002,-336.116825213065)) ;
#46536=CARTESIAN_POINT('Ctrl Pts',(-18.5304464430942,1.15042540549828,-336.117846796191)) ;
#46537=CARTESIAN_POINT('Ctrl Pts',(-18.5134611721284,1.40615827878428,-336.121096448638)) ;
#46538=CARTESIAN_POINT('Ctrl Pts',(-18.4992872112119,1.58173908876808,-336.123304147702)) ;
#46539=CARTESIAN_POINT('Ctrl Pts',(-18.4564140903844,2.03271579750189,-336.128940184567)) ;
#46540=CARTESIAN_POINT('Ctrl Pts',(-18.4240491012346,2.30771958733761,-336.132344264429)) ;
#46541=CARTESIAN_POINT('Ctrl Pts',(-18.2849234231809,3.29842597660611,-336.1446115221)) ;
#46542=CARTESIAN_POINT('Ctrl Pts',(-18.1424992023407,4.00846117673017,-336.153435746986)) ;
#46543=CARTESIAN_POINT('Ctrl Pts',(-17.9198941579576,4.8575378789742,-336.164483661252)) ;
#46544=CARTESIAN_POINT('Ctrl Pts',(-17.8789285313958,5.00621567220246,-336.166435780378)) ;
#46545=CARTESIAN_POINT('Ctrl Pts',(-17.8011003243769,5.27553162138632,-336.170006757127)) ;
#46546=CARTESIAN_POINT('Ctrl Pts',(-17.7648514804252,5.39633750540368,-336.171621446599)) ;
#46547=CARTESIAN_POINT('Ctrl Pts',(-17.6878335820268,5.64382407506593,-336.174956873903)) ;
#46548=CARTESIAN_POINT('Ctrl Pts',(-17.6469277639348,5.77045470022852,-336.176678461387)) ;
#46549=CARTESIAN_POINT('Ctrl Pts',(-17.5356232918261,6.10275914538369,-336.181236215306)) ;
#46550=CARTESIAN_POINT('Ctrl Pts',(-17.4629677138333,6.30765501476063,-336.184087273612)) ;
#46551=CARTESIAN_POINT('Ctrl Pts',(-17.1448779018516,7.15704049088048,-336.196070358147)) ;
#46552=CARTESIAN_POINT('Ctrl Pts',(-16.8672308176833,7.7888757224233,-336.205404486304)) ;
#46553=CARTESIAN_POINT('Ctrl Pts',(-16.3985788646021,8.71209822607914,-336.219317387319)) ;
#46554=CARTESIAN_POINT('Ctrl Pts',(-16.2334933985647,9.0159712295388,-336.223939282063)) ;
#46555=CARTESIAN_POINT('Ctrl Pts',(-16.010611222847,9.40024069076365,-336.229765982323)) ;
#46556=CARTESIAN_POINT('Ctrl Pts',(-15.9605264372088,9.4850299241349,-336.23105038965)) ;
#46557=CARTESIAN_POINT('Ctrl Pts',(-15.8755114120268,9.62637285886781,-336.233186764962)) ;
#46558=CARTESIAN_POINT('Ctrl Pts',(-15.8409478042327,9.68314461891534,-336.234043497295)) ;
#46559=CARTESIAN_POINT('Ctrl Pts',(-15.763998094957,9.80802213478902,-336.235924412564)) ;
#46560=CARTESIAN_POINT('Ctrl Pts',(-15.7214740329294,9.8760411294199,-336.236946781887)) ;
#46561=CARTESIAN_POINT('Ctrl Pts',(-15.5839550353451,10.0928693889064,-336.240202244278)) ;
#46562=CARTESIAN_POINT('Ctrl Pts',(-15.4872777640754,10.24060030934,-336.242414866493)) ;
#46563=CARTESIAN_POINT('Ctrl Pts',(-15.2330470546021,10.6172497446688,-336.248068173139)) ;
#46564=CARTESIAN_POINT('Ctrl Pts',(-15.072434542249,10.8440505379828,-336.251484422158)) ;
#46565=CARTESIAN_POINT('Ctrl Pts',(-14.7678052807181,11.2543676073785,-336.257750556726)) ;
#46566=CARTESIAN_POINT('Ctrl Pts',(-14.6253043346455,11.4389394693402,-336.260602454362)) ;
#46567=CARTESIAN_POINT('Ctrl Pts',(-14.4083345819757,11.7092814509909,-336.264854180674)) ;
#46568=CARTESIAN_POINT('Ctrl Pts',(-14.3364942413808,11.7971314470239,-336.26624782126)) ;
#46569=CARTESIAN_POINT('Ctrl Pts',(-14.0994474180707,12.0816409379055,-336.270805883876)) ;
#46570=CARTESIAN_POINT('Ctrl Pts',(-13.930965093299,12.2755316200063,-336.273983147639)) ;
#46571=CARTESIAN_POINT('Ctrl Pts',(-13.6046076231195,12.635730802631,-336.280049652995)) ;
#46572=CARTESIAN_POINT('Ctrl Pts',(-13.4475680449257,12.8027323215245,-336.282932536417)) ;
#46573=CARTESIAN_POINT('Ctrl Pts',(-13.193085597127,13.0635086168393,-336.287557984781)) ;
#46574=CARTESIAN_POINT('Ctrl Pts',(-13.0976411462376,13.1592006328394,-336.289282781318)) ;
#46575=CARTESIAN_POINT('Ctrl Pts',(-12.910854236077,13.3424264939033,-336.292640513232)) ;
#46576=CARTESIAN_POINT('Ctrl Pts',(-12.8196450589781,13.43008571671,-336.294272171413)) ;
#46577=CARTESIAN_POINT('Ctrl Pts',(-12.5977567893812,13.6390177276984,-336.298223205011)) ;
#46578=CARTESIAN_POINT('Ctrl Pts',(-12.4662130066133,13.7593536849493,-336.30055058827)) ;
#46579=CARTESIAN_POINT('Ctrl Pts',(-12.1770991684383,14.0162845057729,-336.305632819249)) ;
#46580=CARTESIAN_POINT('Ctrl Pts',(-12.0189195114307,14.1521570467785,-336.308392910177)) ;
#46581=CARTESIAN_POINT('Ctrl Pts',(-11.5060443348556,14.5779028983082,-336.317267704812)) ;
#46582=CARTESIAN_POINT('Ctrl Pts',(-11.1428976606122,14.8573261240034,-336.323444534676)) ;
#46583=CARTESIAN_POINT('Ctrl Pts',(-10.4187841022637,15.3729999290968,-336.335415600943)) ;
#46584=CARTESIAN_POINT('Ctrl Pts',(-10.0591804804814,15.6106719318834,-336.341206478574)) ;
#46585=CARTESIAN_POINT('Ctrl Pts',(-9.60028067702208,15.8915254620212,-336.348277332331)) ;
#46586=CARTESIAN_POINT('Ctrl Pts',(-9.50844566604864,15.9466432723273,-336.349676715036)) ;
#46587=CARTESIAN_POINT('Ctrl Pts',(-9.35835608112252,16.0349669767516,-336.351935263997)) ;
#46588=CARTESIAN_POINT('Ctrl Pts',(-9.30038951846853,16.0686573593127,-336.35280067625)) ;
#46589=CARTESIAN_POINT('Ctrl Pts',(-9.1764029695416,16.1398231325885,-336.354636234313)) ;
#46590=CARTESIAN_POINT('Ctrl Pts',(-9.11033314604264,16.1772090361517,-336.355605247957)) ;
#46591=CARTESIAN_POINT('Ctrl Pts',(-8.91218267164981,16.2877344546401,-336.358486869147)) ;
#46592=CARTESIAN_POINT('Ctrl Pts',(-8.77943710279873,16.3596692485729,-336.360384983473)) ;
#46593=CARTESIAN_POINT('Ctrl Pts',(-8.54340766658229,16.4838733234786,-336.363714561511)) ;
#46594=CARTESIAN_POINT('Ctrl Pts',(-8.44048473989926,16.5368108079078,-336.36515144791)) ;
#46595=CARTESIAN_POINT('Ctrl Pts',(-7.92799232610451,16.7943756369697,-336.372245535503)) ;
#46596=CARTESIAN_POINT('Ctrl Pts',(-7.51144580523368,16.9847666551633,-336.377824732685)) ;
#46597=CARTESIAN_POINT('Ctrl Pts',(-6.65203920224582,17.3397710790753,-336.389236300615)) ;
#46598=CARTESIAN_POINT('Ctrl Pts',(-6.20907781673635,17.5032750621506,-336.395067643566)) ;
#46599=CARTESIAN_POINT('Ctrl Pts',(-5.61637812750229,17.696715459099,-336.402919173305)) ;
#46600=CARTESIAN_POINT('Ctrl Pts',(-5.47181755365528,17.7419461695852,-336.404837451913)) ;
#46601=CARTESIAN_POINT('Ctrl Pts',(-5.20645536693862,17.8214220208331,-336.408367364496)) ;
#46602=CARTESIAN_POINT('Ctrl Pts',(-5.08582873106328,17.8562203839036,-336.409975186948)) ;
#46603=CARTESIAN_POINT('Ctrl Pts',(-4.83557718357955,17.9256713587492,-336.413318368301)) ;
#46604=CARTESIAN_POINT('Ctrl Pts',(-4.70591082589835,17.9601476495753,-336.415054806015)) ;
#46605=CARTESIAN_POINT('Ctrl Pts',(-4.359162905314,18.0483296469286,-336.419709846822)) ;
#46606=CARTESIAN_POINT('Ctrl Pts',(-4.14146582230994,18.0995238843538,-336.422644560534)) ;
#46607=CARTESIAN_POINT('Ctrl Pts',(-3.77235242304641,18.1793173565713,-336.427637610606)) ;
#46608=CARTESIAN_POINT('Ctrl Pts',(-3.62140831640021,18.2099869325782,-336.429684178304)) ;
#46609=CARTESIAN_POINT('Ctrl Pts',(-2.93905272368347,18.3398115688181,-336.438950116827)) ;
#46610=CARTESIAN_POINT('Ctrl Pts',(-2.40384617198713,18.4176068208539,-336.446264957943)) ;
#46611=CARTESIAN_POINT('Ctrl Pts',(-1.53704327125577,18.5051701383092,-336.457965816601)) ;
#46612=CARTESIAN_POINT('Ctrl Pts',(-1.20724530034186,18.5296082914501,-336.462381810492)) ;
#46613=CARTESIAN_POINT('Ctrl Pts',(-0.779263766545773,18.5498467749549,
-336.468000768131)) ;
#46614=CARTESIAN_POINT('Ctrl Pts',(-0.681521750322263,18.553694929485,-336.469276396151)) ;
#46615=CARTESIAN_POINT('Ctrl Pts',(-0.517398984326241,18.5588578585254,
-336.471403001518)) ;
#46616=CARTESIAN_POINT('Ctrl Pts',(-0.451033429609828,18.5605893118278,
-336.472258637513)) ;
#46617=CARTESIAN_POINT('Ctrl Pts',(-0.304084826244664,18.5636345291202,
-336.47414318028)) ;
#46618=CARTESIAN_POINT('Ctrl Pts',(-0.223499784666542,18.5647796211695,
-336.475170207338)) ;
#46619=CARTESIAN_POINT('Ctrl Pts',(0.036020094517566,18.566777311963,-336.478460301196)) ;
#46620=CARTESIAN_POINT('Ctrl Pts',(0.214960839268421,18.5655678403829,-336.480702292379)) ;
#46621=CARTESIAN_POINT('Ctrl Pts',(0.677749457253094,18.555748076693,-336.486459320058)) ;
#46622=CARTESIAN_POINT('Ctrl Pts',(0.961467449650487,18.5432120131931,-336.489948842773)) ;
#46623=CARTESIAN_POINT('Ctrl Pts',(1.95154972364018,18.476680525379,-336.50211387363)) ;
#46624=CARTESIAN_POINT('Ctrl Pts',(2.6550166336632,18.3887779855933,-336.510757857971)) ;
#46625=CARTESIAN_POINT('Ctrl Pts',(3.50492264461624,18.2327801975812,-336.521630436128)) ;
#46626=CARTESIAN_POINT('Ctrl Pts',(3.65775039657228,18.2027365640732,-336.523601459922)) ;
#46627=CARTESIAN_POINT('Ctrl Pts',(3.93394980712235,18.1448210340557,-336.527195527761)) ;
#46628=CARTESIAN_POINT('Ctrl Pts',(4.05744924656672,18.1176046154292,-336.52881420291)) ;
#46629=CARTESIAN_POINT('Ctrl Pts',(4.30976856864022,18.0592899481375,-336.532146163601)) ;
#46630=CARTESIAN_POINT('Ctrl Pts',(4.43855298618197,18.0280699430895,-336.533860177119)) ;
#46631=CARTESIAN_POINT('Ctrl Pts',(4.77461467731618,17.9427823278538,-336.538368393595)) ;
#46632=CARTESIAN_POINT('Ctrl Pts',(4.98130956522554,17.8865015513902,-336.541176881499)) ;
#46633=CARTESIAN_POINT('Ctrl Pts',(5.53186207879498,17.7263084730677,-336.548749409958)) ;
#46634=CARTESIAN_POINT('Ctrl Pts',(5.87375485722929,17.6159732378403,-336.553550047724)) ;
#46635=CARTESIAN_POINT('Ctrl Pts',(6.78764964243154,17.2914765934202,-336.566582584134)) ;
#46636=CARTESIAN_POINT('Ctrl Pts',(7.35263823070325,17.0588997643321,-336.574864915176)) ;
#46637=CARTESIAN_POINT('Ctrl Pts',(8.02910400955891,16.7405722441362,-336.58474407851)) ;
#46638=CARTESIAN_POINT('Ctrl Pts',(8.15242160551762,16.6808660543016,-336.586542788729)) ;
#46639=CARTESIAN_POINT('Ctrl Pts',(8.34071868836916,16.5871121598808,-336.589279634255)) ;
#46640=CARTESIAN_POINT('Ctrl Pts',(8.4061760203606,16.5540352414931,-336.590229219872)) ;
#46641=CARTESIAN_POINT('Ctrl Pts',(8.53309748956789,16.4889523188703,-336.59206562258)) ;
#46642=CARTESIAN_POINT('Ctrl Pts',(8.5945817621173,16.4569883536608,-336.592952910309)) ;
#46643=CARTESIAN_POINT('Ctrl Pts',(8.75856320618787,16.3705693459544,-336.595314854343)) ;
#46644=CARTESIAN_POINT('Ctrl Pts',(8.86073123510505,16.3154960755063,-336.596781760389)) ;
#46645=CARTESIAN_POINT('Ctrl Pts',(9.33009219305828,16.0567797758318,-336.603512783883)) ;
#46646=CARTESIAN_POINT('Ctrl Pts',(9.69082746740933,15.8416748433257,-336.608666026154)) ;
#46647=CARTESIAN_POINT('Ctrl Pts',(10.6006441670877,15.2564401155219,-336.621920671892)) ;
#46648=CARTESIAN_POINT('Ctrl Pts',(11.1377812130958,14.8688415977146,-336.630012512024)) ;
#46649=CARTESIAN_POINT('Ctrl Pts',(11.7913923492662,14.341866570518,-336.640567700127)) ;
#46650=CARTESIAN_POINT('Ctrl Pts',(11.9281074994823,14.2283632791518,-336.642816125266)) ;
#46651=CARTESIAN_POINT('Ctrl Pts',(12.1592659193274,14.0307780337073,-336.646692232955)) ;
#46652=CARTESIAN_POINT('Ctrl Pts',(12.2545181618922,13.9476616138505,-336.648311705373)) ;
#46653=CARTESIAN_POINT('Ctrl Pts',(12.4499808924639,13.7735541584542,-336.651682424056)) ;
#46654=CARTESIAN_POINT('Ctrl Pts',(12.5500601956619,13.6824269556898,-336.653434798297)) ;
#46655=CARTESIAN_POINT('Ctrl Pts',(12.8177502724778,13.4332735769396,-336.658194765053)) ;
#46656=CARTESIAN_POINT('Ctrl Pts',(12.9834308579745,13.2732092536153,-336.661219823784)) ;
#46657=CARTESIAN_POINT('Ctrl Pts',(13.3596863137221,12.8959210111008,-336.668270300761)) ;
#46658=CARTESIAN_POINT('Ctrl Pts',(13.5680161862333,12.6765505313175,-336.672311651406)) ;
#46659=CARTESIAN_POINT('Ctrl Pts',(14.2302096695341,11.9442298308755,-336.685569231387)) ;
#46660=CARTESIAN_POINT('Ctrl Pts',(14.6610688071018,11.4112468122039,-336.694877026294)) ;
#46661=CARTESIAN_POINT('Ctrl Pts',(15.1261539172385,10.7659739666095,-336.705338237633)) ;
#46662=CARTESIAN_POINT('Ctrl Pts',(15.1900095341653,10.6756891199396,-336.706783999225)) ;
#46663=CARTESIAN_POINT('Ctrl Pts',(15.288170164031,10.5342368548669,-336.709017973716)) ;
#46664=CARTESIAN_POINT('Ctrl Pts',(15.3230335492272,10.4834601133414,-336.709813725017)) ;
#46665=CARTESIAN_POINT('Ctrl Pts',(15.385586565875,10.3913761498993,-336.711245000505)) ;
#46666=CARTESIAN_POINT('Ctrl Pts',(15.4133641151279,10.35012941587,-336.711881879415)) ;
#46667=CARTESIAN_POINT('Ctrl Pts',(15.441858489285,10.3074491668673,-336.712536798886)) ;
#46668=CARTESIAN_POINT('Ctrl Pts',(15.4427411789722,10.3061266637827,-336.712557088373)) ;
#46669=CARTESIAN_POINT('Ctrl Pts',(15.4444221621669,10.3036074046309,-336.712595730481)) ;
#46670=CARTESIAN_POINT('Ctrl Pts',(15.4452204864739,10.3024106691689,-336.712614083518)) ;
#46671=CARTESIAN_POINT('Ctrl Pts',(15.4994420847522,10.2211088117034,-336.713860698078)) ;
#46672=CARTESIAN_POINT('Ctrl Pts',(15.5522415945285,10.1405893172973,-336.715080549578)) ;
#46673=CARTESIAN_POINT('Ctrl Pts',(15.6724090207215,9.95418723447399,-336.717874633862)) ;
#46674=CARTESIAN_POINT('Ctrl Pts',(15.7393345548186,9.84802497187523,-336.719444054811)) ;
#46675=CARTESIAN_POINT('Ctrl Pts',(15.9514215635742,9.50391174913691,-336.724472639074)) ;
#46676=CARTESIAN_POINT('Ctrl Pts',(16.0923027449555,9.2633677026108,-336.727899145572)) ;
#46677=CARTESIAN_POINT('Ctrl Pts',(16.5758995830656,8.39331280436065,-336.740104247365)) ;
#46678=CARTESIAN_POINT('Ctrl Pts',(16.8875197914619,7.74724608133012,-336.748846084691)) ;
#46679=CARTESIAN_POINT('Ctrl Pts',(17.2204232560578,6.94087623535054,-336.759822984308)) ;
#46680=CARTESIAN_POINT('Ctrl Pts',(17.2780235925646,6.79622252973804,-336.76179335756)) ;
#46681=CARTESIAN_POINT('Ctrl Pts',(17.3790949499431,6.53280546375797,-336.765386629941)) ;
#46682=CARTESIAN_POINT('Ctrl Pts',(17.4231849996114,6.41428974418798,-336.767005167114)) ;
#46683=CARTESIAN_POINT('Ctrl Pts',(17.5069715585861,6.18182846812967,-336.770184421531)) ;
#46684=CARTESIAN_POINT('Ctrl Pts',(17.5467748201958,6.0679279597706,-336.771744310635)) ;
#46685=CARTESIAN_POINT('Ctrl Pts',(17.6174090954213,5.85929341465668,-336.774605731026)) ;
#46686=CARTESIAN_POINT('Ctrl Pts',(17.6485932820567,5.7646836594305,-336.775904834849)) ;
#46687=CARTESIAN_POINT('Ctrl Pts',(17.7324738574679,5.50313674499995,-336.779500214258)) ;
#46688=CARTESIAN_POINT('Ctrl Pts',(17.7835729263924,5.33569835938262,-336.781806494656)) ;
#46689=CARTESIAN_POINT('Ctrl Pts',(17.9228055462893,4.85523251205596,-336.788433577623)) ;
#46690=CARTESIAN_POINT('Ctrl Pts',(18.0050932671665,4.54057895175931,-336.792785514256)) ;
#46691=CARTESIAN_POINT('Ctrl Pts',(18.2253194808984,3.59797609250834,-336.805798716501)) ;
#46692=CARTESIAN_POINT('Ctrl Pts',(18.3389572516868,2.96485225607021,-336.814520758419)) ;
#46693=CARTESIAN_POINT('Ctrl Pts',(18.4333941711011,2.2173667532049,-336.824429859012)) ;
#46694=CARTESIAN_POINT('Ctrl Pts',(18.4462784148842,2.10749820449643,-336.825876115381)) ;
#46695=CARTESIAN_POINT('Ctrl Pts',(18.4648074636674,1.93627971815218,-336.828110659655)) ;
#46696=CARTESIAN_POINT('Ctrl Pts',(18.4711301000094,1.87500577749903,-336.828906492121)) ;
#46697=CARTESIAN_POINT('Ctrl Pts',(18.483054996078,1.75352047544371,-336.830475967602)) ;
#46698=CARTESIAN_POINT('Ctrl Pts',(18.4886682591311,1.6933109756913,-336.831249776767)) ;
#46699=CARTESIAN_POINT('Ctrl Pts',(18.5004714635441,1.55964393623653,-336.832959678667)) ;
#46700=CARTESIAN_POINT('Ctrl Pts',(18.5065182621756,1.48617475751466,-336.833894173919)) ;
#46701=CARTESIAN_POINT('Ctrl Pts',(18.5208048449971,1.29895851735991,-336.836263861446)) ;
#46702=CARTESIAN_POINT('Ctrl Pts',(18.5284344295844,1.18516791004337,-336.837693260093)) ;
#46703=CARTESIAN_POINT('Ctrl Pts',(18.5727468430842,0.418510199645596,-336.847268754458)) ;
#46704=CARTESIAN_POINT('Ctrl Pts',(18.5759646867155,-0.235832692476801,
-336.855190346612)) ;
#46705=CARTESIAN_POINT('Ctrl Pts',(18.544654593745,-0.888979977948838,-336.86323988221)) ;
#46706=CARTESIAN_POINT('Origin',(0.,0.,-315.477129595899)) ;
#46707=CARTESIAN_POINT('',(1.74714810520642,18.4835595300519,-338.)) ;
#46708=CARTESIAN_POINT('Ctrl Pts',(18.544654593745,-0.88897997794884,-336.86323988221)) ;
#46709=CARTESIAN_POINT('Ctrl Pts',(18.5265686305932,-1.26626399779565,-336.867889616222)) ;
#46710=CARTESIAN_POINT('Ctrl Pts',(18.4969733686538,-1.64290749982776,-336.872575171038)) ;
#46711=CARTESIAN_POINT('Ctrl Pts',(18.4415834579998,-2.14938732150166,-336.878990748352)) ;
#46712=CARTESIAN_POINT('Ctrl Pts',(18.4258623126442,-2.28023338170186,-336.880658333735)) ;
#46713=CARTESIAN_POINT('Ctrl Pts',(18.393655079212,-2.52615593426246,-336.883813539215)) ;
#46714=CARTESIAN_POINT('Ctrl Pts',(18.3774786508234,-2.64126662313804,-336.885299110609)) ;
#46715=CARTESIAN_POINT('Ctrl Pts',(18.3414912639957,-2.88099239673001,-336.888411946457)) ;
#46716=CARTESIAN_POINT('Ctrl Pts',(18.3214887815987,-3.00557278223992,-336.890040393454)) ;
#46717=CARTESIAN_POINT('Ctrl Pts',(18.2691318471016,-3.31169477659058,-336.894068946227)) ;
#46718=CARTESIAN_POINT('Ctrl Pts',(18.2353397246696,-3.49297662515185,-336.896478224894)) ;
#46719=CARTESIAN_POINT('Ctrl Pts',(18.1060003392576,-4.13369649534109,-336.905075295906)) ;
#46720=CARTESIAN_POINT('Ctrl Pts',(17.9957429284565,-4.58998140408656,-336.911351892757)) ;
#46721=CARTESIAN_POINT('Ctrl Pts',(17.7119139045931,-5.5959221044881,-336.925414311519)) ;
#46722=CARTESIAN_POINT('Ctrl Pts',(17.5297990794366,-6.14266904028077,-336.93321430086)) ;
#46723=CARTESIAN_POINT('Ctrl Pts',(17.2810249938321,-6.7877834091317,-336.942337520284)) ;
#46724=CARTESIAN_POINT('Ctrl Pts',(17.2384814132826,-6.8951132746513,-336.943852235716)) ;
#46725=CARTESIAN_POINT('Ctrl Pts',(17.171257265604,-7.06019591400926,-336.946173375537)) ;
#46726=CARTESIAN_POINT('Ctrl Pts',(17.1472801556599,-7.11823192237263,-336.946987727237)) ;
#46727=CARTESIAN_POINT('Ctrl Pts',(17.0974213867107,-7.23719999332893,-336.94865279573)) ;
#46728=CARTESIAN_POINT('Ctrl Pts',(17.0715074014463,-7.29811735020341,-336.949502912958)) ;
#46729=CARTESIAN_POINT('Ctrl Pts',(17.0071843443249,-7.44710762215979,-336.951576730206)) ;
#46730=CARTESIAN_POINT('Ctrl Pts',(16.9684163292498,-7.53502346202996,-336.952795992257)) ;
#46731=CARTESIAN_POINT('Ctrl Pts',(16.8024443076704,-7.90362764754281,-336.95789645455)) ;
#46732=CARTESIAN_POINT('Ctrl Pts',(16.6689442964888,-8.18142784433175,-336.961712887694)) ;
#46733=CARTESIAN_POINT('Ctrl Pts',(16.4869757416514,-8.53712360864424,-336.966629076275)) ;
#46734=CARTESIAN_POINT('Ctrl Pts',(16.4447598828384,-8.61816227620197,-336.967751106731)) ;
#46735=CARTESIAN_POINT('Ctrl Pts',(16.1701554218104,-9.13593523586149,-336.974940055253)) ;
#46736=CARTESIAN_POINT('Ctrl Pts',(15.9209872872141,-9.56354551294087,-336.980975123815)) ;
#46737=CARTESIAN_POINT('Ctrl Pts',(15.5389315482835,-10.1628123343842,-336.98977773544)) ;
#46738=CARTESIAN_POINT('Ctrl Pts',(15.4196541204778,-10.3428919946753,-336.99246887544)) ;
#46739=CARTESIAN_POINT('Ctrl Pts',(15.200159035679,-10.6620367470411,-336.99733432259)) ;
#46740=CARTESIAN_POINT('Ctrl Pts',(15.1011060513966,-10.8018729027347,-336.999500238586)) ;
#46741=CARTESIAN_POINT('Ctrl Pts',(14.9358094690646,-11.0285089633956,-337.003070634853)) ;
#46742=CARTESIAN_POINT('Ctrl Pts',(14.8707108383856,-11.116131232529,-337.004466034893)) ;
#46743=CARTESIAN_POINT('Ctrl Pts',(14.728750532445,-11.3037298578851,-337.007486879867)) ;
#46744=CARTESIAN_POINT('Ctrl Pts',(14.6516353065675,-11.4035075190406,-337.009114336854)) ;
#46745=CARTESIAN_POINT('Ctrl Pts',(14.4780317605986,-11.6234609876665,-337.012748953348)) ;
#46746=CARTESIAN_POINT('Ctrl Pts',(14.381051499472,-11.7432366350648,-337.014760041866)) ;
#46747=CARTESIAN_POINT('Ctrl Pts',(13.771784871978,-12.4768447721432,-337.027275009489)) ;
#46748=CARTESIAN_POINT('Ctrl Pts',(13.2217835308721,-13.0582595354045,-337.038103053513)) ;
#46749=CARTESIAN_POINT('Ctrl Pts',(12.4671662859456,-13.7592653897275,-337.051937970139)) ;
#46750=CARTESIAN_POINT('Ctrl Pts',(12.2953997165666,-13.912971117315,-337.055021905454)) ;
#46751=CARTESIAN_POINT('Ctrl Pts',(12.0356866446258,-14.1368092786094,-337.059565249018)) ;
#46752=CARTESIAN_POINT('Ctrl Pts',(11.9498927894016,-14.2094050529352,-337.06104724391)) ;
#46753=CARTESIAN_POINT('Ctrl Pts',(11.8622583982412,-14.2822031730269,-337.062539867073)) ;
#46754=CARTESIAN_POINT('Ctrl Pts',(11.8610716462739,-14.2831887610653,-337.062560076389)) ;
#46755=CARTESIAN_POINT('Ctrl Pts',(11.8588167939988,-14.2850609230665,-337.062598467058)) ;
#46756=CARTESIAN_POINT('Ctrl Pts',(11.857748717066,-14.2859475251827,-337.062616648757)) ;
#46757=CARTESIAN_POINT('Ctrl Pts',(11.8557184002759,-14.2876324903445,-337.06265120448)) ;
#46758=CARTESIAN_POINT('Ctrl Pts',(11.8547561791747,-14.2884308759957,-337.062667578783)) ;
#46759=CARTESIAN_POINT('Ctrl Pts',(11.8529262878602,-14.2899488833151,-337.062698713501)) ;
#46760=CARTESIAN_POINT('Ctrl Pts',(11.8520586327732,-14.2906685231487,-337.06271347414)) ;
#46761=CARTESIAN_POINT('Ctrl Pts',(11.8504079135291,-14.2920373887053,-337.062741552363)) ;
#46762=CARTESIAN_POINT('Ctrl Pts',(11.8496248615414,-14.2926866291094,-337.062754870128)) ;
#46763=CARTESIAN_POINT('Ctrl Pts',(11.8481345415857,-14.2939220695666,-337.062780213511)) ;
#46764=CARTESIAN_POINT('Ctrl Pts',(11.8474272834421,-14.2945082815013,-337.062792239277)) ;
#46765=CARTESIAN_POINT('Ctrl Pts',(11.8460807488733,-14.2956241900424,-337.062815132237)) ;
#46766=CARTESIAN_POINT('Ctrl Pts',(11.8454414803834,-14.2961538962955,-337.062825999552)) ;
#46767=CARTESIAN_POINT('Ctrl Pts',(11.8427935936528,-14.2983476704235,-337.062871007874)) ;
#46768=CARTESIAN_POINT('Ctrl Pts',(11.8407846602433,-14.3000113578946,-337.062905144134)) ;
#46769=CARTESIAN_POINT('Ctrl Pts',(11.8368450296075,-14.3032725425738,-337.062972065145)) ;
#46770=CARTESIAN_POINT('Ctrl Pts',(11.8349143594196,-14.3048700723667,-337.063004850307)) ;
#46771=CARTESIAN_POINT('Ctrl Pts',(11.8311267191055,-14.3080028572933,-337.063069148663)) ;
#46772=CARTESIAN_POINT('Ctrl Pts',(11.8292697734438,-14.3095381419155,-337.06310066223)) ;
#46773=CARTESIAN_POINT('Ctrl Pts',(11.8256253309633,-14.3125500980742,-337.063162491824)) ;
#46774=CARTESIAN_POINT('Ctrl Pts',(11.8238378562684,-14.3140267963588,-337.06319280819)) ;
#46775=CARTESIAN_POINT('Ctrl Pts',(11.8203283695737,-14.3169250058793,-337.063252313057)) ;
#46776=CARTESIAN_POINT('Ctrl Pts',(11.8186063776903,-14.3183465413342,-337.063281501867)) ;
#46777=CARTESIAN_POINT('Ctrl Pts',(11.8152241172785,-14.3211376326448,-337.06333881689)) ;
#46778=CARTESIAN_POINT('Ctrl Pts',(11.8135638669432,-14.3225072105525,-337.063366943385)) ;
#46779=CARTESIAN_POINT('Ctrl Pts',(11.8103015799519,-14.3251973914358,-337.063422194947)) ;
#46780=CARTESIAN_POINT('Ctrl Pts',(11.8086995598674,-14.3265180144305,-337.063449320272)) ;
#46781=CARTESIAN_POINT('Ctrl Pts',(11.8055504375172,-14.3291131019168,-337.063502626861)) ;
#46782=CARTESIAN_POINT('Ctrl Pts',(11.8040033503379,-14.3303875846223,-337.06352880836)) ;
#46783=CARTESIAN_POINT('Ctrl Pts',(11.8009609970708,-14.3328930331323,-337.063580281127)) ;
#46784=CARTESIAN_POINT('Ctrl Pts',(11.7994657446899,-14.3341240155611,-337.06360557261)) ;
#46785=CARTESIAN_POINT('Ctrl Pts',(11.7965241496713,-14.3365449427886,-337.063655315887)) ;
#46786=CARTESIAN_POINT('Ctrl Pts',(11.795077819522,-14.3377349027591,-337.063679767879)) ;
#46787=CARTESIAN_POINT('Ctrl Pts',(11.7922313302171,-14.3400761135696,-337.063727879664)) ;
#46788=CARTESIAN_POINT('Ctrl Pts',(11.790831182477,-14.3412273782494,-337.063751539637)) ;
#46789=CARTESIAN_POINT('Ctrl Pts',(11.788074480017,-14.3434933868624,-337.063798112034)) ;
#46790=CARTESIAN_POINT('Ctrl Pts',(11.7867179357019,-14.3446081434663,-337.063821024624)) ;
#46791=CARTESIAN_POINT('Ctrl Pts',(11.7840460118055,-14.3468031941408,-337.063866144261)) ;
#46792=CARTESIAN_POINT('Ctrl Pts',(11.7827306417714,-14.3478834997786,-337.063888351462)) ;
#46793=CARTESIAN_POINT('Ctrl Pts',(11.7801387775574,-14.3500115857538,-337.063932099874)) ;
#46794=CARTESIAN_POINT('Ctrl Pts',(11.7788622921383,-14.3510593766671,-337.063953641226)) ;
#46795=CARTESIAN_POINT('Ctrl Pts',(11.7763460381555,-14.3531242579314,-337.063996095212)) ;
#46796=CARTESIAN_POINT('Ctrl Pts',(11.7751062775822,-14.3541413580069,-337.064017007974)) ;
#46797=CARTESIAN_POINT('Ctrl Pts',(11.7726614351801,-14.3561465778156,-337.064058239928)) ;
#46798=CARTESIAN_POINT('Ctrl Pts',(11.7714563606991,-14.3571347064538,-337.064078559237)) ;
#46799=CARTESIAN_POINT('Ctrl Pts',(11.7690789649703,-14.3590836064218,-337.064118637456)) ;
#46800=CARTESIAN_POINT('Ctrl Pts',(11.7679066504242,-14.3600443859628,-337.064138396474)) ;
#46801=CARTESIAN_POINT('Ctrl Pts',(11.7655929538511,-14.3619401204602,-337.064177385446)) ;
#46802=CARTESIAN_POINT('Ctrl Pts',(11.7644515779945,-14.3628750829497,-337.064196615501)) ;
#46803=CARTESIAN_POINT('Ctrl Pts',(11.7621980356222,-14.3647206321386,-337.064234576172)) ;
#46804=CARTESIAN_POINT('Ctrl Pts',(11.7610858748104,-14.3656312257386,-337.064253306882)) ;
#46805=CARTESIAN_POINT('Ctrl Pts',(11.7588891301807,-14.3674294078918,-337.064290296904)) ;
#46806=CARTESIAN_POINT('Ctrl Pts',(11.7578045515846,-14.3683170028146,-337.064308556302)) ;
#46807=CARTESIAN_POINT('Ctrl Pts',(11.7556614235258,-14.3700704858472,-337.064344630265)) ;
#46808=CARTESIAN_POINT('Ctrl Pts',(11.7546028788573,-14.370936379831,-337.06436244491)) ;
#46809=CARTESIAN_POINT('Ctrl Pts',(11.7525103493197,-14.3726476919004,-337.064397654559)) ;
#46810=CARTESIAN_POINT('Ctrl Pts',(11.7514763688978,-14.3734931153702,-337.064415049637)) ;
#46811=CARTESIAN_POINT('Ctrl Pts',(11.6920605738015,-14.4220631330692,-337.065414450741)) ;
#46812=CARTESIAN_POINT('Ctrl Pts',(11.6333885845426,-14.4694317627552,-337.066391622801)) ;
#46813=CARTESIAN_POINT('Ctrl Pts',(11.5218290913369,-14.5583817636873,-337.068229968658)) ;
#46814=CARTESIAN_POINT('Ctrl Pts',(11.4690010690042,-14.6000356046604,-337.069092143294)) ;
#46815=CARTESIAN_POINT('Ctrl Pts',(11.3303910663484,-14.7081102701367,-337.071333973471)) ;
#46816=CARTESIAN_POINT('Ctrl Pts',(11.2442511345906,-14.774068021703,-337.07270707896)) ;
#46817=CARTESIAN_POINT('Ctrl Pts',(10.9625272986188,-14.9858941441139,-337.077141026413)) ;
#46818=CARTESIAN_POINT('Ctrl Pts',(10.7646448538793,-15.1286631809299,-337.080167777639)) ;
#46819=CARTESIAN_POINT('Ctrl Pts',(10.0803296811316,-15.6021600812877,-337.090426481884)) ;
#46820=CARTESIAN_POINT('Ctrl Pts',(9.58102302231907,-15.9136559291941,-337.097571645627)) ;
#46821=CARTESIAN_POINT('Ctrl Pts',(8.92787418422019,-16.2792280331928,-337.106824502396)) ;
#46822=CARTESIAN_POINT('Ctrl Pts',(8.78696583365569,-16.3557156422516,-337.108814518315)) ;
#46823=CARTESIAN_POINT('Ctrl Pts',(8.44182682730863,-16.537315702751,-337.113681850263)) ;
#46824=CARTESIAN_POINT('Ctrl Pts',(8.23660228988048,-16.640481762122,-337.116570339585)) ;
#46825=CARTESIAN_POINT('Ctrl Pts',(7.9075873222291,-16.7982990067202,-337.121202475483)) ;
#46826=CARTESIAN_POINT('Ctrl Pts',(7.78502249357073,-16.8554504979229,-337.12292825858)) ;
#46827=CARTESIAN_POINT('Ctrl Pts',(7.54664839825791,-16.9634486868319,-337.126286523949)) ;
#46828=CARTESIAN_POINT('Ctrl Pts',(7.43092229329707,-17.0144611203132,-337.127917713177)) ;
#46829=CARTESIAN_POINT('Ctrl Pts',(7.17693372168415,-17.123334474387,-337.131500046504)) ;
#46830=CARTESIAN_POINT('Ctrl Pts',(7.03847352728636,-17.1807116117197,-337.133454419095)) ;
#46831=CARTESIAN_POINT('Ctrl Pts',(6.4693413726946,-17.4085220274516,-337.141492907344)) ;
#46832=CARTESIAN_POINT('Ctrl Pts',(6.03306002502255,-17.564486941311,-337.147671475266)) ;
#46833=CARTESIAN_POINT('Ctrl Pts',(5.5451686283761,-17.7185765615315,-337.154547432412)) ;
#46834=CARTESIAN_POINT('Ctrl Pts',(5.49887484141452,-17.7329982225645,-337.15519947808)) ;
#46835=CARTESIAN_POINT('Ctrl Pts',(5.04014202546078,-17.8739357667677,-337.161656023324)) ;
#46836=CARTESIAN_POINT('Ctrl Pts',(4.6234682830375,-17.9862211861031,-337.167486666762)) ;
#46837=CARTESIAN_POINT('Ctrl Pts',(3.98240262974287,-18.135224923981,-337.176271801821)) ;
#46838=CARTESIAN_POINT('Ctrl Pts',(3.76062041774433,-18.1825094024561,-337.179277074822)) ;
#46839=CARTESIAN_POINT('Ctrl Pts',(3.45244364155189,-18.2423335387018,-337.183382237448)) ;
#46840=CARTESIAN_POINT('Ctrl Pts',(3.36674362992775,-18.2583443224037,-337.18451626699)) ;
#46841=CARTESIAN_POINT('Ctrl Pts',(3.22261795783564,-18.2842211560227,-337.186408893294)) ;
#46842=CARTESIAN_POINT('Ctrl Pts',(3.16425228019977,-18.294412188025,-337.18717125781)) ;
#46843=CARTESIAN_POINT('Ctrl Pts',(3.02247713089083,-18.3184682929686,-337.189013191714)) ;
#46844=CARTESIAN_POINT('Ctrl Pts',(2.93901992079468,-18.3320432723602,-337.19008936472)) ;
#46845=CARTESIAN_POINT('Ctrl Pts',(2.6731990927211,-18.3734192428039,-337.193495147808)) ;
#46846=CARTESIAN_POINT('Ctrl Pts',(2.49051232565694,-18.3990727110932,-337.195803066356)) ;
#46847=CARTESIAN_POINT('Ctrl Pts',(2.02627700329742,-18.457221158992,-337.201614160078)) ;
#46848=CARTESIAN_POINT('Ctrl Pts',(1.74431061402484,-18.4859998991031,-337.205094199303)) ;
#46849=CARTESIAN_POINT('Ctrl Pts',(0.996331021764724,-18.5450757085032,
-337.214289850893)) ;
#46850=CARTESIAN_POINT('Ctrl Pts',(0.529644850950633,-18.56426633708,-337.219993725895)) ;
#46851=CARTESIAN_POINT('Ctrl Pts',(-0.235706945328343,-18.5668524318551,
-337.229480335364)) ;
#46852=CARTESIAN_POINT('Ctrl Pts',(-0.534127537944787,-18.5606647030296,
-337.233211113626)) ;
#46853=CARTESIAN_POINT('Ctrl Pts',(-0.978497295567214,-18.5407245906999,
-337.238839077589)) ;
#46854=CARTESIAN_POINT('Ctrl Pts',(-1.12464317494191,-18.5324338108651,
-337.240701587462)) ;
#46855=CARTESIAN_POINT('Ctrl Pts',(-1.39446233738143,-18.5139236649315,
-337.244163571441)) ;
#46856=CARTESIAN_POINT('Ctrl Pts',(-1.51816075258351,-18.5041909458274,
-337.245759796679)) ;
#46857=CARTESIAN_POINT('Ctrl Pts',(-1.79737939195762,-18.4794030593261,
-337.249384109079)) ;
#46858=CARTESIAN_POINT('Ctrl Pts',(-1.95282580772015,-18.4636231918855,
-337.25141676978)) ;
#46859=CARTESIAN_POINT('Ctrl Pts',(-2.45317658527703,-18.4064415098261,
-337.258007388268)) ;
#46860=CARTESIAN_POINT('Ctrl Pts',(-2.79712308874901,-18.357321859942,-337.262612671676)) ;
#46861=CARTESIAN_POINT('Ctrl Pts',(-3.80889548323213,-18.1837320594787,
-337.276337332927)) ;
#46862=CARTESIAN_POINT('Ctrl Pts',(-4.47149450999833,-18.0322358609752,
-337.28557207522)) ;
#46863=CARTESIAN_POINT('Ctrl Pts',(-5.30201063540625,-17.7937452062654,
-337.297060982794)) ;
#46864=CARTESIAN_POINT('Ctrl Pts',(-5.47895084124401,-17.7400615312942,
-337.299502097368)) ;
#46865=CARTESIAN_POINT('Ctrl Pts',(-5.73269425455235,-17.6589172785579,
-337.30297944206)) ;
#46866=CARTESIAN_POINT('Ctrl Pts',(-5.81016442807697,-17.6335796765932,
-337.304037923689)) ;
#46867=CARTESIAN_POINT('Ctrl Pts',(-5.95027316648523,-17.5867317746885,
-337.305944827105)) ;
#46868=CARTESIAN_POINT('Ctrl Pts',(-6.01296807900864,-17.5653949613401,
-337.306795246113)) ;
#46869=CARTESIAN_POINT('Ctrl Pts',(-6.16655045187865,-17.5122080175102,
-337.308872168392)) ;
#46870=CARTESIAN_POINT('Ctrl Pts',(-6.25730681961934,-17.4799852839671,
-337.310094198476)) ;
#46871=CARTESIAN_POINT('Ctrl Pts',(-6.63915278250707,-17.3410572739465,
-337.315220708546)) ;
#46872=CARTESIAN_POINT('Ctrl Pts',(-6.92779702139999,-17.227775431521,-337.319059669787)) ;
#46873=CARTESIAN_POINT('Ctrl Pts',(-7.72750271517918,-16.8905716541226,
-337.329737712685)) ;
#46874=CARTESIAN_POINT('Ctrl Pts',(-8.23150561821859,-16.6507665024935,
-337.33652349363)) ;
#46875=CARTESIAN_POINT('Ctrl Pts',(-8.92456338412012,-16.2818401990359,
-337.346234643413)) ;
#46876=CARTESIAN_POINT('Ctrl Pts',(-9.12320383029136,-16.171372963148,-337.349062498541)) ;
#46877=CARTESIAN_POINT('Ctrl Pts',(-9.48364583691386,-15.9621698076591,
-337.354291929071)) ;
#46878=CARTESIAN_POINT('Ctrl Pts',(-9.6460598693921,-15.8645495416576,-337.356685837561)) ;
#46879=CARTESIAN_POINT('Ctrl Pts',(-9.91585921733149,-15.6967094195172,
-337.360731313816)) ;
#46880=CARTESIAN_POINT('Ctrl Pts',(-10.0240623959671,-15.6278317000411,
-337.362372684548)) ;
#46881=CARTESIAN_POINT('Ctrl Pts',(-10.2290641077171,-15.4943309127415,
-337.365519765013)) ;
#46882=CARTESIAN_POINT('Ctrl Pts',(-10.325985789075,-15.4299079840115,-337.367023877579)) ;
#46883=CARTESIAN_POINT('Ctrl Pts',(-10.584066772803,-15.2548432216093,-337.371073092722)) ;
#46884=CARTESIAN_POINT('Ctrl Pts',(-10.7440948709388,-15.1425604301122,
-337.373630714292)) ;
#46885=CARTESIAN_POINT('Ctrl Pts',(-11.1775747870512,-14.8280802293311,
-337.380685921552)) ;
#46886=CARTESIAN_POINT('Ctrl Pts',(-11.4472908159555,-14.6208643235309,
-337.385218821993)) ;
#46887=CARTESIAN_POINT('Ctrl Pts',(-12.108585815896,-14.0832868764024,-337.396651785194)) ;
#46888=CARTESIAN_POINT('Ctrl Pts',(-12.4924694559441,-13.743908685068,-337.403587703407)) ;
#46889=CARTESIAN_POINT('Ctrl Pts',(-12.9849056572438,-13.2708647267054,
-337.412715766089)) ;
#46890=CARTESIAN_POINT('Ctrl Pts',(-13.1063463126288,-13.150943387666,-337.414986140838)) ;
#46891=CARTESIAN_POINT('Ctrl Pts',(-13.3154922174194,-12.9386392466927,
-337.41891798456)) ;
#46892=CARTESIAN_POINT('Ctrl Pts',(-13.4039322894773,-12.8469964508616,
-337.420587640591)) ;
#46893=CARTESIAN_POINT('Ctrl Pts',(-13.5405272124373,-12.7025088645293,
-337.423172378803)) ;
#46894=CARTESIAN_POINT('Ctrl Pts',(-13.5893315541714,-12.6502836558196,
-337.424097098684)) ;
#46895=CARTESIAN_POINT('Ctrl Pts',(-13.6858676359047,-12.545777687681,-337.425927414341)) ;
#46896=CARTESIAN_POINT('Ctrl Pts',(-13.7336043834825,-12.4935031671368,
-337.426833075017)) ;
#46897=CARTESIAN_POINT('Ctrl Pts',(-13.8640542818238,-12.3490017901589,
-337.429311513389)) ;
#46898=CARTESIAN_POINT('Ctrl Pts',(-13.9461452137241,-12.2562180176238,
-337.430875159676)) ;
#46899=CARTESIAN_POINT('Ctrl Pts',(-14.3307413724206,-11.8126584497127,
-337.438237118602)) ;
#46900=CARTESIAN_POINT('Ctrl Pts',(-14.6209792888549,-11.4514634335351,
-337.443905122343)) ;
#46901=CARTESIAN_POINT('Ctrl Pts',(-15.2475728792096,-10.6089730350663,
-337.456764864175)) ;
#46902=CARTESIAN_POINT('Ctrl Pts',(-15.5752232609312,-10.1218183474588,
-337.463957871749)) ;
#46903=CARTESIAN_POINT('Ctrl Pts',(-15.9754219479083,-9.46122825371702,
-337.473655222031)) ;
#46904=CARTESIAN_POINT('Ctrl Pts',(-16.0692045420226,-9.30105433343085,
-337.476001246936)) ;
#46905=CARTESIAN_POINT('Ctrl Pts',(-16.2227691078573,-9.0295197336975,-337.479974349549)) ;
#46906=CARTESIAN_POINT('Ctrl Pts',(-16.2838441178181,-8.91890603389366,
-337.481591728708)) ;
#46907=CARTESIAN_POINT('Ctrl Pts',(-16.4067146228485,-8.69090391719736,
-337.484924261849)) ;
#46908=CARTESIAN_POINT('Ctrl Pts',(-16.4683906917594,-8.57345925369965,
-337.4866401775)) ;
#46909=CARTESIAN_POINT('Ctrl Pts',(-16.6267413860339,-8.26391049300647,
-337.491161467706)) ;
#46910=CARTESIAN_POINT('Ctrl Pts',(-16.7213460209501,-8.07077026994344,
-337.493981290446)) ;
#46911=CARTESIAN_POINT('Ctrl Pts',(-16.9283433989182,-7.6289031758779,-337.500426189572)) ;
#46912=CARTESIAN_POINT('Ctrl Pts',(-17.0386498298657,-7.37925372014498,
-337.504063264857)) ;
#46913=CARTESIAN_POINT('Ctrl Pts',(-17.27823779395,-6.80296591064329,-337.51242712722)) ;
#46914=CARTESIAN_POINT('Ctrl Pts',(-17.4038334501075,-6.47490751718258,
-337.517166050968)) ;
#46915=CARTESIAN_POINT('Ctrl Pts',(-17.6466274330943,-5.7825053639327,-337.527042224929)) ;
#46916=CARTESIAN_POINT('Ctrl Pts',(-17.76202027054,-5.41769922020092,-337.53217516624)) ;
#46917=CARTESIAN_POINT('Ctrl Pts',(-17.8973433960072,-4.93890952795463,
-337.538724687259)) ;
#46918=CARTESIAN_POINT('Ctrl Pts',(-17.92759631809,-4.82794141198704,-337.540229592352)) ;
#46919=CARTESIAN_POINT('Ctrl Pts',(-17.9726487986361,-4.65642335048746,
-337.542531799876)) ;
#46920=CARTESIAN_POINT('Ctrl Pts',(-17.9881778285759,-4.5960680671048,-337.543337387056)) ;
#46921=CARTESIAN_POINT('Ctrl Pts',(-18.0207565375332,-4.46675265129384,
-337.545052846509)) ;
#46922=CARTESIAN_POINT('Ctrl Pts',(-18.0377149310502,-4.39777051644626,
-337.545961530433)) ;
#46923=CARTESIAN_POINT('Ctrl Pts',(-18.0834437031337,-4.20704320568332,
-337.548458233123)) ;
#46924=CARTESIAN_POINT('Ctrl Pts',(-18.1113801670703,-4.08510186161933,
-337.55003690287)) ;
#46925=CARTESIAN_POINT('Ctrl Pts',(-18.1736031830096,-3.80030795651262,
-337.553691663373)) ;
#46926=CARTESIAN_POINT('Ctrl Pts',(-18.206936780322,-3.63725809095476,-337.555759699621)) ;
#46927=CARTESIAN_POINT('Ctrl Pts',(-18.3285272357752,-2.9988830609984,-337.563793052122)) ;
#46928=CARTESIAN_POINT('Ctrl Pts',(-18.4003974450696,-2.5206319216884,-337.569679408035)) ;
#46929=CARTESIAN_POINT('Ctrl Pts',(-18.4955769143574,-1.65970475933777,
-337.580319714443)) ;
#46930=CARTESIAN_POINT('Ctrl Pts',(-18.5258602755883,-1.27807884560058,
-337.585050441076)) ;
#46931=CARTESIAN_POINT('Ctrl Pts',(-18.5536265740605,-0.703271364018113,
-337.592267949947)) ;
#46932=CARTESIAN_POINT('Ctrl Pts',(-18.559927741788,-0.510618945880516,
-337.594702036229)) ;
#46933=CARTESIAN_POINT('Ctrl Pts',(-18.5652136896176,-0.201958564616765,
-337.598631289096)) ;
#46934=CARTESIAN_POINT('Ctrl Pts',(-18.5661129745813,-0.0859975408256846,
-337.60011409432)) ;
#46935=CARTESIAN_POINT('Ctrl Pts',(-18.5657180975435,0.158669720775562,
-337.603257501209)) ;
#46936=CARTESIAN_POINT('Ctrl Pts',(-18.5641720332945,0.287369481770842,
-337.604919654319)) ;
#46937=CARTESIAN_POINT('Ctrl Pts',(-18.5569820045037,0.608144766603883,
-337.609084567169)) ;
#46938=CARTESIAN_POINT('Ctrl Pts',(-18.5496941171968,0.80016820018835,-337.611597635363)) ;
#46939=CARTESIAN_POINT('Ctrl Pts',(-18.5270390753093,1.22354827122444,-337.617180564022)) ;
#46940=CARTESIAN_POINT('Ctrl Pts',(-18.5103161295274,1.45480025580107,-337.620257828346)) ;
#46941=CARTESIAN_POINT('Ctrl Pts',(-18.4359831066122,2.27011795631746,-337.631188282154)) ;
#46942=CARTESIAN_POINT('Ctrl Pts',(-18.3550185601147,2.85170125926168,-337.639142900375)) ;
#46943=CARTESIAN_POINT('Ctrl Pts',(-18.1992201466161,3.68087530499706,-337.650444836503)) ;
#46944=CARTESIAN_POINT('Ctrl Pts',(-18.1465620100062,3.93226964993906,-337.653864249844)) ;
#46945=CARTESIAN_POINT('Ctrl Pts',(-18.0655154317374,4.28278511303226,-337.658587995002)) ;
#46946=CARTESIAN_POINT('Ctrl Pts',(-18.0414915030655,4.38288495512111,-337.659931884344)) ;
#46947=CARTESIAN_POINT('Ctrl Pts',(-18.0005995517078,4.54723284426785,-337.662126996871)) ;
#46948=CARTESIAN_POINT('Ctrl Pts',(-17.9842170348184,4.61159933694331,-337.662983785051)) ;
#46949=CARTESIAN_POINT('Ctrl Pts',(-17.9479255697805,4.75105265245432,-337.664832950561)) ;
#46950=CARTESIAN_POINT('Ctrl Pts',(-17.9278900880458,4.82610511464074,-337.665823872147)) ;
#46951=CARTESIAN_POINT('Ctrl Pts',(-17.864884077229,5.05631650141751,-337.668853042459)) ;
#46952=CARTESIAN_POINT('Ctrl Pts',(-17.8203658314698,5.21104417927811,-337.67087457091)) ;
#46953=CARTESIAN_POINT('Ctrl Pts',(-17.7370323068503,5.48711294392608,-337.674469438548)) ;
#46954=CARTESIAN_POINT('Ctrl Pts',(-17.6989699714832,5.60867056538357,-337.676048098802)) ;
#46955=CARTESIAN_POINT('Ctrl Pts',(-17.4884455814695,6.25751897518943,-337.68447088185)) ;
#46956=CARTESIAN_POINT('Ctrl Pts',(-17.2936652738147,6.77727198264912,-337.691213435586)) ;
#46957=CARTESIAN_POINT('Ctrl Pts',(-16.9306458308721,7.62788834156565,-337.702613668866)) ;
#46958=CARTESIAN_POINT('Ctrl Pts',(-16.7752431429694,7.96383484331001,-337.707213261177)) ;
#46959=CARTESIAN_POINT('Ctrl Pts',(-16.5387156677983,8.43746242199008,-337.713891698462)) ;
#46960=CARTESIAN_POINT('Ctrl Pts',(-16.465694324304,8.57909076646474,-337.715913921227)) ;
#46961=CARTESIAN_POINT('Ctrl Pts',(-16.3324841324128,8.82949090562173,-337.719537102852)) ;
#46962=CARTESIAN_POINT('Ctrl Pts',(-16.2730088718536,8.93863131544694,-337.72113277668)) ;
#46963=CARTESIAN_POINT('Ctrl Pts',(-16.1421833388425,9.17306952012986,-337.724596908037)) ;
#46964=CARTESIAN_POINT('Ctrl Pts',(-16.0704602772,9.29815001843839,-337.726468049733)) ;
#46965=CARTESIAN_POINT('Ctrl Pts',(-15.8533064937878,9.66683295239111,-337.732051961852)) ;
#46966=CARTESIAN_POINT('Ctrl Pts',(-15.7037414723527,9.90795081395331,-337.735794467603)) ;
#46967=CARTESIAN_POINT('Ctrl Pts',(-15.3163663682105,10.5016283984981,-337.745223608137)) ;
#46968=CARTESIAN_POINT('Ctrl Pts',(-15.0718592724392,10.8496237119391,-337.750948142807)) ;
#46969=CARTESIAN_POINT('Ctrl Pts',(-14.7941044717809,11.2174082147167,-337.757156588435)) ;
#46970=CARTESIAN_POINT('Ctrl Pts',(-14.7725050348352,11.2458378600002,-337.757637532124)) ;
#46971=CARTESIAN_POINT('Ctrl Pts',(-14.6726897587314,11.3764331028436,-337.759851359177)) ;
#46972=CARTESIAN_POINT('Ctrl Pts',(-14.5934951752647,11.4778462040384,-337.761583385516)) ;
#46973=CARTESIAN_POINT('Ctrl Pts',(-14.3045982507987,11.8399708502171,-337.767806282188)) ;
#46974=CARTESIAN_POINT('Ctrl Pts',(-14.0889114889462,12.0958263341312,-337.772276350352)) ;
#46975=CARTESIAN_POINT('Ctrl Pts',(-13.8008091834959,12.4194163832969,-337.777959490908)) ;
#46976=CARTESIAN_POINT('Ctrl Pts',(-13.7346028249548,12.4925947145931,-337.77924665296)) ;
#46977=CARTESIAN_POINT('Ctrl Pts',(-13.6228442058364,12.6141599246285,-337.781385572522)) ;
#46978=CARTESIAN_POINT('Ctrl Pts',(-13.5776099528982,12.6628362882938,-337.782242135847)) ;
#46979=CARTESIAN_POINT('Ctrl Pts',(-13.4773947780995,12.7695229846536,-337.784119160409)) ;
#46980=CARTESIAN_POINT('Ctrl Pts',(-13.4222987196319,12.8274231381388,-337.78513784651)) ;
#46981=CARTESIAN_POINT('Ctrl Pts',(-13.2452956139777,13.0110457063218,-337.788371702654)) ;
#46982=CARTESIAN_POINT('Ctrl Pts',(-13.1219828043096,13.1354000222848,-337.790566714488)) ;
#46983=CARTESIAN_POINT('Ctrl Pts',(-12.8010380576781,13.4500250669684,-337.796158611634)) ;
#46984=CARTESIAN_POINT('Ctrl Pts',(-12.6009147774146,13.6376939697119,-337.799531626368)) ;
#46985=CARTESIAN_POINT('Ctrl Pts',(-11.8531490633726,14.3084071101835,-337.811848320548)) ;
#46986=CARTESIAN_POINT('Ctrl Pts',(-11.2813020189845,14.7634644109396,-337.820749647775)) ;
#46987=CARTESIAN_POINT('Ctrl Pts',(-10.5582643959879,15.272237722145,-337.831877368254)) ;
#46988=CARTESIAN_POINT('Ctrl Pts',(-10.4312850065132,15.3592475440648,-337.833825869107)) ;
#46989=CARTESIAN_POINT('Ctrl Pts',(-10.1984291940722,15.5145871689236,-337.837391514242)) ;
#46990=CARTESIAN_POINT('Ctrl Pts',(-10.092911006511,15.5834373746747,-337.839004514752)) ;
#46991=CARTESIAN_POINT('Ctrl Pts',(-9.89476589075203,15.709869524002,-337.842029224401)) ;
#46992=CARTESIAN_POINT('Ctrl Pts',(-9.80231648317952,15.7677196836731,-337.843438783243)) ;
#46993=CARTESIAN_POINT('Ctrl Pts',(-9.56350988578535,15.9142407737393,-337.847075775736)) ;
#46994=CARTESIAN_POINT('Ctrl Pts',(-9.41642690528055,16.00170881338,-337.849312028745)) ;
#46995=CARTESIAN_POINT('Ctrl Pts',(-9.08121571305503,16.1948314793187,-337.854398898427)) ;
#46996=CARTESIAN_POINT('Ctrl Pts',(-8.8924125852895,16.2992651263362,-337.857257337435)) ;
#46997=CARTESIAN_POINT('Ctrl Pts',(-8.265594563013,16.6318466902534,-337.866713649771)) ;
#46998=CARTESIAN_POINT('Ctrl Pts',(-7.82029558364206,16.8458111484877,-337.87338359454)) ;
#46999=CARTESIAN_POINT('Ctrl Pts',(-7.00680726113727,17.1974746421768,-337.885307792654)) ;
#47000=CARTESIAN_POINT('Ctrl Pts',(-6.64176914850144,17.341723838742,-337.890566815487)) ;
#47001=CARTESIAN_POINT('Ctrl Pts',(-6.17849982963986,17.5080153045906,-337.897024894798)) ;
#47002=CARTESIAN_POINT('Ctrl Pts',(-6.08429460441766,17.5409754363863,-337.898326983859)) ;
#47003=CARTESIAN_POINT('Ctrl Pts',(-5.92768903227221,17.5943545492179,-337.900470442245)) ;
#47004=CARTESIAN_POINT('Ctrl Pts',(-5.86543801244742,17.6152049725359,-337.901316908699)) ;
#47005=CARTESIAN_POINT('Ctrl Pts',(-5.75459145447676,17.6516792978701,-337.902813814101)) ;
#47006=CARTESIAN_POINT('Ctrl Pts',(-5.7060397964305,17.6674337324536,-337.903466051801)) ;
#47007=CARTESIAN_POINT('Ctrl Pts',(-5.65495066307624,17.6837789836597,-337.904149068195)) ;
#47008=CARTESIAN_POINT('Ctrl Pts',(-5.65247740102427,17.6845696972152,-337.904182125374)) ;
#47009=CARTESIAN_POINT('Ctrl Pts',(-5.64753933790878,17.6861472775638,-337.904248110464)) ;
#47010=CARTESIAN_POINT('Ctrl Pts',(-5.64507453808973,17.6869341480177,-337.904281038414)) ;
#47011=CARTESIAN_POINT('Ctrl Pts',(-5.64008304778363,17.6885264974097,-337.904347704905)) ;
#47012=CARTESIAN_POINT('Ctrl Pts',(-5.63755634902524,17.6893319502752,-337.90438144315)) ;
#47013=CARTESIAN_POINT('Ctrl Pts',(-5.63236943636784,17.6909841933274,-337.904450685226)) ;
#47014=CARTESIAN_POINT('Ctrl Pts',(-5.62970920386892,17.6918309249259,-337.904486188398)) ;
#47015=CARTESIAN_POINT('Ctrl Pts',(-5.62417464033936,17.6935911593359,-337.90456003285)) ;
#47016=CARTESIAN_POINT('Ctrl Pts',(-5.62130027747067,17.6945045618484,-337.904598373009)) ;
#47017=CARTESIAN_POINT('Ctrl Pts',(-5.61523925041663,17.6964289827091,-337.904679196381)) ;
#47018=CARTESIAN_POINT('Ctrl Pts',(-5.61205253544679,17.6974398408039,-337.904721677817)) ;
#47019=CARTESIAN_POINT('Ctrl Pts',(-5.60523954148687,17.6995989658937,-337.904812472392)) ;
#47020=CARTESIAN_POINT('Ctrl Pts',(-5.60161318226705,17.7007469793557,-337.904860782741)) ;
#47021=CARTESIAN_POINT('Ctrl Pts',(-5.59374793180748,17.7032342593022,-337.904965527017)) ;
#47022=CARTESIAN_POINT('Ctrl Pts',(-5.58950891177702,17.7045731179687,-337.90502195649)) ;
#47023=CARTESIAN_POINT('Ctrl Pts',(-5.58017406068875,17.7075177650895,-337.905146170901)) ;
#47024=CARTESIAN_POINT('Ctrl Pts',(-5.57507801642473,17.7091228766229,-337.905213948518)) ;
#47025=CARTESIAN_POINT('Ctrl Pts',(-5.56367286026134,17.712709771202,-337.905365564398)) ;
#47026=CARTESIAN_POINT('Ctrl Pts',(-5.55736338079426,17.7146903836523,-337.905449390146)) ;
#47027=CARTESIAN_POINT('Ctrl Pts',(-5.54299761743427,17.7191915185861,-337.905640136348)) ;
#47028=CARTESIAN_POINT('Ctrl Pts',(-5.534940669784,17.7217099186622,-337.905747034437)) ;
#47029=CARTESIAN_POINT('Ctrl Pts',(-5.51626417783073,17.7275337433994,-337.905994646337)) ;
#47030=CARTESIAN_POINT('Ctrl Pts',(-5.50564337478121,17.7308351222599,-337.906135318309)) ;
#47031=CARTESIAN_POINT('Ctrl Pts',(-5.393457645564,17.7655965054165,-337.907619782775)) ;
#47032=CARTESIAN_POINT('Ctrl Pts',(-5.29162711782083,17.7961930495159,-337.908954867205)) ;
#47033=CARTESIAN_POINT('Ctrl Pts',(-4.98817806958313,17.8845341486628,-337.912903326114)) ;
#47034=CARTESIAN_POINT('Ctrl Pts',(-4.78583774015009,17.9397391147446,-337.91549711237)) ;
#47035=CARTESIAN_POINT('Ctrl Pts',(-3.76877363567561,18.1987949158494,-337.928417984037)) ;
#47036=CARTESIAN_POINT('Ctrl Pts',(-2.94181595956697,18.3506270718738,-337.938599472441)) ;
#47037=CARTESIAN_POINT('Ctrl Pts',(-1.95738059961305,18.4630974589892,-337.951080077392)) ;
#47038=CARTESIAN_POINT('Ctrl Pts',(-1.80713276387469,18.4784084184793,-337.95299305859)) ;
#47039=CARTESIAN_POINT('Ctrl Pts',(-1.53029649992009,18.5032105848156,-337.95653542175)) ;
#47040=CARTESIAN_POINT('Ctrl Pts',(-1.40376527731856,18.5132399194726,-337.958161249225)) ;
#47041=CARTESIAN_POINT('Ctrl Pts',(-1.16102092305774,18.5299778161289,-337.961294173287)) ;
#47042=CARTESIAN_POINT('Ctrl Pts',(-1.04482793301391,18.536892457972,-337.962799858185)) ;
#47043=CARTESIAN_POINT('Ctrl Pts',(-0.794579205922912,18.5494243553547,
-337.966056002095)) ;
#47044=CARTESIAN_POINT('Ctrl Pts',(-0.660512033239542,18.5546819919181,
-337.967808648295)) ;
#47045=CARTESIAN_POINT('Ctrl Pts',(0.232271529319654,18.5800052363997,-337.979533061582)) ;
#47046=CARTESIAN_POINT('Ctrl Pts',(0.991546553996248,18.5549823431925,-337.989794133195)) ;
#47047=CARTESIAN_POINT('Ctrl Pts',(1.74714810520653,18.4835595300519,-338.)) ;
#47048=CARTESIAN_POINT('',(-16.8928031616863,7.70244771115141,-338.)) ;
#47049=CARTESIAN_POINT('Origin',(0.,0.,-338.)) ;
#47050=CARTESIAN_POINT('Ctrl Pts',(-16.8928031616863,7.70244771115143,-337.999999999999)) ;
#47051=CARTESIAN_POINT('Ctrl Pts',(-16.9188581960729,7.64530450372309,-337.99919244096)) ;
#47052=CARTESIAN_POINT('Ctrl Pts',(-16.9446190476498,7.58803854460336,-337.998388608593)) ;
#47053=CARTESIAN_POINT('Ctrl Pts',(-17.0038275925238,7.45461358547285,-337.996527305167)) ;
#47054=CARTESIAN_POINT('Ctrl Pts',(-17.0370510917385,7.37836747688368,-337.995472358634)) ;
#47055=CARTESIAN_POINT('Ctrl Pts',(-17.2554492358772,6.8678149048698,-337.988459126563)) ;
#47056=CARTESIAN_POINT('Ctrl Pts',(-17.4245119701244,6.42680284526227,-337.982641320138)) ;
#47057=CARTESIAN_POINT('Ctrl Pts',(-17.7535182551691,5.45975044350684,-337.970040429329)) ;
#47058=CARTESIAN_POINT('Ctrl Pts',(-17.9072859597764,4.932078039822,-337.963258239092)) ;
#47059=CARTESIAN_POINT('Ctrl Pts',(-18.0693340115061,4.26752905602644,-337.954633063947)) ;
#47060=CARTESIAN_POINT('Ctrl Pts',(-18.0998138504038,4.13634795285629,-337.952927002217)) ;
#47061=CARTESIAN_POINT('Ctrl Pts',(-18.154499088932,3.88880260477542,-337.949698628977)) ;
#47062=CARTESIAN_POINT('Ctrl Pts',(-18.1790196208309,3.77251487095066,-337.948178370506)) ;
#47063=CARTESIAN_POINT('Ctrl Pts',(-18.2277242807706,3.53002504267113,-337.944999295962)) ;
#47064=CARTESIAN_POINT('Ctrl Pts',(-18.2517181472502,3.40379110325536,-337.943339333239)) ;
#47065=CARTESIAN_POINT('Ctrl Pts',(-18.3077469514219,3.09137325465647,-337.939217610156)) ;
#47066=CARTESIAN_POINT('Ctrl Pts',(-18.3382542000407,2.90493024922351,-337.936746038841)) ;
#47067=CARTESIAN_POINT('Ctrl Pts',(-18.4731594511183,1.99337462635964,-337.924604442218)) ;
#47068=CARTESIAN_POINT('Ctrl Pts',(-18.5374222240515,1.26298472956102,-337.914670290704)) ;
#47069=CARTESIAN_POINT('Ctrl Pts',(-18.5677967501832,0.200835039614022,
-337.900263869959)) ;
#47070=CARTESIAN_POINT('Ctrl Pts',(-18.5684331098627,-0.129240748430358,
-337.895797453102)) ;
#47071=CARTESIAN_POINT('Ctrl Pts',(-18.5568696865713,-0.596662274280294,
-337.889550433306)) ;
#47072=CARTESIAN_POINT('Ctrl Pts',(-18.5519400413342,-0.734124802416489,
-337.887722984908)) ;
#47073=CARTESIAN_POINT('Ctrl Pts',(-18.5435270028039,-0.913149806758578,
-337.885360738916)) ;
#47074=CARTESIAN_POINT('Ctrl Pts',(-18.541430496892,-0.954772960078674,
-337.884812772039)) ;
#47075=CARTESIAN_POINT('Ctrl Pts',(-18.5381926376051,-1.01501782226077,
-337.884021632401)) ;
#47076=CARTESIAN_POINT('Ctrl Pts',(-18.5371633378414,-1.03364541064481,
-337.883777287968)) ;
#47077=CARTESIAN_POINT('Ctrl Pts',(-18.5351704879708,-1.06875011431447,
-337.88331734451)) ;
#47078=CARTESIAN_POINT('Ctrl Pts',(-18.5342130389737,-1.08522755730566,
-337.883101679288)) ;
#47079=CARTESIAN_POINT('Ctrl Pts',(-18.5324800310322,-1.11438080504803,
-337.882720514291)) ;
#47080=CARTESIAN_POINT('Ctrl Pts',(-18.5317134367886,-1.12705713081293,
-337.882554913701)) ;
#47081=CARTESIAN_POINT('Ctrl Pts',(-18.530436352407,-1.14782126872729,-337.882283884815)) ;
#47082=CARTESIAN_POINT('Ctrl Pts',(-18.529933572153,-1.15590954973787,-337.882178367521)) ;
#47083=CARTESIAN_POINT('Ctrl Pts',(-18.5291171570826,-1.16890588540298,
-337.882008914125)) ;
#47084=CARTESIAN_POINT('Ctrl Pts',(-18.5288068675271,-1.1738141487093,-337.881944938776)) ;
#47085=CARTESIAN_POINT('Ctrl Pts',(-18.5247310790322,-1.23788201776811,
-337.881110145112)) ;
#47086=CARTESIAN_POINT('Ctrl Pts',(-18.5206842105924,-1.29702345425174,
-337.880342692485)) ;
#47087=CARTESIAN_POINT('Ctrl Pts',(-18.5113245475063,-1.4248172221504,-337.878691746081)) ;
#47088=CARTESIAN_POINT('Ctrl Pts',(-18.5059129440674,-1.49346132935088,
-337.877809409628)) ;
#47089=CARTESIAN_POINT('Ctrl Pts',(-18.4906740763074,-1.67393991952697,
-337.875499592387)) ;
#47090=CARTESIAN_POINT('Ctrl Pts',(-18.480214100079,-1.78571820928802,-337.874079138758)) ;
#47091=CARTESIAN_POINT('Ctrl Pts',(-18.4184518411596,-2.38689574520511,
-337.866479324765)) ;
#47092=CARTESIAN_POINT('Ctrl Pts',(-18.3487216540359,-2.87420527469133,
-337.860455916264)) ;
#47093=CARTESIAN_POINT('Ctrl Pts',(-18.1874349418463,-3.75118602144865,
-337.849521072117)) ;
#47094=CARTESIAN_POINT('Ctrl Pts',(-18.1024847220203,-4.14176686824144,
-337.844617313402)) ;
#47095=CARTESIAN_POINT('Ctrl Pts',(-17.9575661950423,-4.71785083528004,
-337.837234282909)) ;
#47096=CARTESIAN_POINT('Ctrl Pts',(-17.9071762018885,-4.9056437372042,-337.834803917681)) ;
#47097=CARTESIAN_POINT('Ctrl Pts',(-17.817558584524,-5.21982822230585,-337.830689705542)) ;
#47098=CARTESIAN_POINT('Ctrl Pts',(-17.7799124228897,-5.34665453913763,
-337.829015650587)) ;
#47099=CARTESIAN_POINT('Ctrl Pts',(-17.7065941232427,-5.58431534615988,
-337.825851622708)) ;
#47100=CARTESIAN_POINT('Ctrl Pts',(-17.6712285945077,-5.69523776939787,
-337.824363735064)) ;
#47101=CARTESIAN_POINT('Ctrl Pts',(-17.5953559582878,-5.92569624326049,
-337.821248168713)) ;
#47102=CARTESIAN_POINT('Ctrl Pts',(-17.5546685132985,-6.0451667140607,-337.819619327982)) ;
#47103=CARTESIAN_POINT('Ctrl Pts',(-17.4615841985422,-6.30962283433346,
-337.815982651812)) ;
#47104=CARTESIAN_POINT('Ctrl Pts',(-17.4085932633193,-6.45438947780506,
-337.813970889814)) ;
#47105=CARTESIAN_POINT('Ctrl Pts',(-17.0927548541525,-7.28503517459725,
-337.802307573286)) ;
#47106=CARTESIAN_POINT('Ctrl Pts',(-16.7911922035276,-7.95549251413836,
-337.792387711098)) ;
#47107=CARTESIAN_POINT('Ctrl Pts',(-16.323774399633,-8.84894751894135,-337.778812818181)) ;
#47108=CARTESIAN_POINT('Ctrl Pts',(-16.1914864699571,-9.0887429847299,-337.77513612963)) ;
#47109=CARTESIAN_POINT('Ctrl Pts',(-15.966183818221,-9.47660276504974,-337.769177278606)) ;
#47110=CARTESIAN_POINT('Ctrl Pts',(-15.8762961464612,-9.62643477818321,
-337.76687247728)) ;
#47111=CARTESIAN_POINT('Ctrl Pts',(-15.7424397449059,-9.84258165761327,
-337.763555351717)) ;
#47112=CARTESIAN_POINT('Ctrl Pts',(-15.7001385782781,-9.90991783291571,
-337.762523098242)) ;
#47113=CARTESIAN_POINT('Ctrl Pts',(-15.6216173634878,-10.0331453545823,
-337.760637676208)) ;
#47114=CARTESIAN_POINT('Ctrl Pts',(-15.5855267590846,-10.0891174237195,
-337.759782834516)) ;
#47115=CARTESIAN_POINT('Ctrl Pts',(-15.4950212842524,-10.2278356693535,
-337.757667034972)) ;
#47116=CARTESIAN_POINT('Ctrl Pts',(-15.4402439855551,-10.3103430004259,
-337.756410973078)) ;
#47117=CARTESIAN_POINT('Ctrl Pts',(-15.1979323683554,-10.6690585084154,
-337.750952284421)) ;
#47118=CARTESIAN_POINT('Ctrl Pts',(-15.0036270228117,-10.9406185793828,
-337.746824769584)) ;
#47119=CARTESIAN_POINT('Ctrl Pts',(-14.4783565129213,-11.6344040394412,
-337.736127632206)) ;
#47120=CARTESIAN_POINT('Ctrl Pts',(-14.1362305270345,-12.0477861713762,
-337.729594818879)) ;
#47121=CARTESIAN_POINT('Ctrl Pts',(-13.6264495250558,-12.6120816009759,
-337.720182202701)) ;
#47122=CARTESIAN_POINT('Ctrl Pts',(-13.4732110501547,-12.7756531243153,
-337.717391692523)) ;
#47123=CARTESIAN_POINT('Ctrl Pts',(-13.1860457861014,-13.0712678967762,
-337.712217592317)) ;
#47124=CARTESIAN_POINT('Ctrl Pts',(-13.0530017661685,-13.2041278634552,
-337.709841228432)) ;
#47125=CARTESIAN_POINT('Ctrl Pts',(-12.8253750001033,-13.4246367860071,
-337.705804973176)) ;
#47126=CARTESIAN_POINT('Ctrl Pts',(-12.7318554801358,-13.5133627460517,
-337.704154833109)) ;
#47127=CARTESIAN_POINT('Ctrl Pts',(-12.5391174070485,-13.6924446266258,
-337.700769390557)) ;
#47128=CARTESIAN_POINT('Ctrl Pts',(-12.4398279715769,-13.7827132733262,
-337.699033464451)) ;
#47129=CARTESIAN_POINT('Ctrl Pts',(-12.1758902405054,-14.0174957017878,
-337.694439584705)) ;
#47130=CARTESIAN_POINT('Ctrl Pts',(-12.0096478356262,-14.1601852918689,
-337.691566677777)) ;
#47131=CARTESIAN_POINT('Ctrl Pts',(-11.5277336506861,-14.5592305565574,
-337.683301407167)) ;
#47132=CARTESIAN_POINT('Ctrl Pts',(-11.2061133370042,-14.8082024617246,
-337.677857999014)) ;
#47133=CARTESIAN_POINT('Ctrl Pts',(-10.4678344223743,-15.3418811029349,
-337.665608110429)) ;
#47134=CARTESIAN_POINT('Ctrl Pts',(-10.0472196716053,-15.6205713864155,
-337.658791566909)) ;
#47135=CARTESIAN_POINT('Ctrl Pts',(-9.47517696226214,-15.9669201060522,
-337.64992499468)) ;
#47136=CARTESIAN_POINT('Ctrl Pts',(-9.33344809165379,-16.050179532163,-337.647760383374)) ;
#47137=CARTESIAN_POINT('Ctrl Pts',(-9.12221936603019,-16.1705229585972,
-337.64459154668)) ;
#47138=CARTESIAN_POINT('Ctrl Pts',(-9.05355920175741,-16.2090642764882,
-337.643570336987)) ;
#47139=CARTESIAN_POINT('Ctrl Pts',(-8.92579414819752,-16.279718132154,-337.641687842569)) ;
#47140=CARTESIAN_POINT('Ctrl Pts',(-8.86675606676054,-16.3119483962873,
-337.640825123939)) ;
#47141=CARTESIAN_POINT('Ctrl Pts',(-8.73191435216094,-16.3846132717879,
-337.638870047247)) ;
#47142=CARTESIAN_POINT('Ctrl Pts',(-8.65600256777216,-16.424843983839,-337.637780254346)) ;
#47143=CARTESIAN_POINT('Ctrl Pts',(-8.31409188125779,-16.6030165312821,
-337.632914766127)) ;
#47144=CARTESIAN_POINT('Ctrl Pts',(-8.04505566291371,-16.7350339677029,
-337.62920175647)) ;
#47145=CARTESIAN_POINT('Ctrl Pts',(-7.25829576949921,-17.0977423961332,
-337.618537622511)) ;
#47146=CARTESIAN_POINT('Ctrl Pts',(-6.73305628867108,-17.3113144089846,
-337.611647857577)) ;
#47147=CARTESIAN_POINT('Ctrl Pts',(-6.05050393443399,-17.5530816852706,
-337.602693858556)) ;
#47148=CARTESIAN_POINT('Ctrl Pts',(-5.90147321729994,-17.6037464281009,
-337.600739523138)) ;
#47149=CARTESIAN_POINT('Ctrl Pts',(-5.53637856621129,-17.722707268024,-337.595946058512)) ;
#47150=CARTESIAN_POINT('Ctrl Pts',(-5.31967403037213,-17.7889546763883,
-337.593095852704)) ;
#47151=CARTESIAN_POINT('Ctrl Pts',(-4.97275729339706,-17.8881021826791,
-337.58851520856)) ;
#47152=CARTESIAN_POINT('Ctrl Pts',(-4.84330691640878,-17.92358482132,-337.586802121521)) ;
#47153=CARTESIAN_POINT('Ctrl Pts',(-4.59169872284972,-17.9896263310643,
-337.583463649905)) ;
#47154=CARTESIAN_POINT('Ctrl Pts',(-4.46959223747947,-18.0203523236862,
-337.581839493758)) ;
#47155=CARTESIAN_POINT('Ctrl Pts',(-4.20178716293336,-18.0848513998054,
-337.578268158141)) ;
#47156=CARTESIAN_POINT('Ctrl Pts',(-4.05597391173209,-18.1181108577903,
-337.576317706154)) ;
#47157=CARTESIAN_POINT('Ctrl Pts',(-3.17494126956148,-18.3079022791802,
-337.564498191089)) ;
#47158=CARTESIAN_POINT('Ctrl Pts',(-2.43117433725998,-18.4214255466751,
-337.5543428602)) ;
#47159=CARTESIAN_POINT('Ctrl Pts',(-1.41255871919411,-18.5141214936157,
-337.540572616883)) ;
#47160=CARTESIAN_POINT('Ctrl Pts',(-1.14202733898975,-18.5327761189988,
-337.536932398543)) ;
#47161=CARTESIAN_POINT('Ctrl Pts',(-0.697612801291283,-18.5536527238791,
-337.531022334191)) ;
#47162=CARTESIAN_POINT('Ctrl Pts',(-0.523934894895575,-18.559369208769,
-337.528730277034)) ;
#47163=CARTESIAN_POINT('Ctrl Pts',(-0.270782387465692,-18.5641451742232,
-337.525426782088)) ;
#47164=CARTESIAN_POINT('Ctrl Pts',(-0.191353718588193,-18.5651337977623,
-337.524395659643)) ;
#47165=CARTESIAN_POINT('Ctrl Pts',(-0.0455977369839269,-18.5660124742976,
-337.522514896667)) ;
#47166=CARTESIAN_POINT('Ctrl Pts',(0.0207271590437921,-18.5660568976193,
-337.521663564146)) ;
#47167=CARTESIAN_POINT('Ctrl Pts',(0.185563508850104,-18.5652840142503,
-337.519557938232)) ;
#47168=CARTESIAN_POINT('Ctrl Pts',(0.284070969452338,-18.5640380324628,
-337.518308504251)) ;
#47169=CARTESIAN_POINT('Ctrl Pts',(0.727223939508055,-18.5549046272341,
-337.512719425601)) ;
#47170=CARTESIAN_POINT('Ctrl Pts',(1.07162016243955,-18.5382030339172,-337.50846103083)) ;
#47171=CARTESIAN_POINT('Ctrl Pts',(1.82721153944864,-18.4804333664853,-337.499151998639)) ;
#47172=CARTESIAN_POINT('Ctrl Pts',(2.23790565233202,-18.4352081062668,-337.494113170103)) ;
#47173=CARTESIAN_POINT('Ctrl Pts',(2.92175035722675,-18.3367136906023,-337.485609014814)) ;
#47174=CARTESIAN_POINT('Ctrl Pts',(3.19582783508557,-18.2909370518057,-337.482170365039)) ;
#47175=CARTESIAN_POINT('Ctrl Pts',(3.68275729956908,-18.1983307755493,-337.475975111973)) ;
#47176=CARTESIAN_POINT('Ctrl Pts',(3.89600731066712,-18.1538720701245,-337.473232269572)) ;
#47177=CARTESIAN_POINT('Ctrl Pts',(4.23848192736388,-18.0761598801779,-337.468770858266)) ;
#47178=CARTESIAN_POINT('Ctrl Pts',(4.36821665871895,-18.0452478016478,-337.467067682485)) ;
#47179=CARTESIAN_POINT('Ctrl Pts',(4.62029597270353,-17.9823067363904,-337.463731430486)) ;
#47180=CARTESIAN_POINT('Ctrl Pts',(4.7426687030866,-17.9504201609849,-337.462099382753)) ;
#47181=CARTESIAN_POINT('Ctrl Pts',(5.04301789487366,-17.868872625104,-337.458062461319)) ;
#47182=CARTESIAN_POINT('Ctrl Pts',(5.22059689339074,-17.8178002653068,-337.45564840873)) ;
#47183=CARTESIAN_POINT('Ctrl Pts',(6.00993472971528,-17.5779703516544,-337.444798602224)) ;
#47184=CARTESIAN_POINT('Ctrl Pts',(6.61244745600688,-17.3602963749601,-337.436177849526)) ;
#47185=CARTESIAN_POINT('Ctrl Pts',(7.48630099871245,-16.9924867040809,-337.423413137357)) ;
#47186=CARTESIAN_POINT('Ctrl Pts',(7.76708008626951,-16.8659946133317,-337.419273212102)) ;
#47187=CARTESIAN_POINT('Ctrl Pts',(8.21402726250655,-16.6511141724765,-337.412678438344)) ;
#47188=CARTESIAN_POINT('Ctrl Pts',(8.38222426430207,-16.5670807222096,-337.410195755635)) ;
#47189=CARTESIAN_POINT('Ctrl Pts',(8.6220390612338,-16.4426789350177,-337.406669094071)) ;
#47190=CARTESIAN_POINT('Ctrl Pts',(8.69471024507359,-16.4043671597866,-337.40560218554)) ;
#47191=CARTESIAN_POINT('Ctrl Pts',(8.82556352928745,-16.3342683624853,-337.40368597192)) ;
#47192=CARTESIAN_POINT('Ctrl Pts',(8.88383401057819,-16.3026497177098,-337.402834588802)) ;
#47193=CARTESIAN_POINT('Ctrl Pts',(9.02603877402914,-16.2244979430392,-337.400760949613)) ;
#47194=CARTESIAN_POINT('Ctrl Pts',(9.10978398404738,-16.1776248335793,-337.399543092827)) ;
#47195=CARTESIAN_POINT('Ctrl Pts',(9.45975445794345,-15.9781633055454,-337.394460462082)) ;
#47196=CARTESIAN_POINT('Ctrl Pts',(9.72253968998316,-15.8196358939966,-337.390659893475)) ;
#47197=CARTESIAN_POINT('Ctrl Pts',(10.4538864334989,-15.3533358057312,-337.379986569922)) ;
#47198=CARTESIAN_POINT('Ctrl Pts',(10.9126092192951,-15.0307558976382,-337.373169450775)) ;
#47199=CARTESIAN_POINT('Ctrl Pts',(11.5361176770485,-14.5486873504796,-337.363421697105)) ;
#47200=CARTESIAN_POINT('Ctrl Pts',(11.7136243296819,-14.4061556121394,-337.360589535784)) ;
#47201=CARTESIAN_POINT('Ctrl Pts',(12.0341315003098,-14.138958388649,-337.355353767798)) ;
#47202=CARTESIAN_POINT('Ctrl Pts',(12.1779285884804,-14.0152959444733,-337.352957875584)) ;
#47203=CARTESIAN_POINT('Ctrl Pts',(12.4157196223072,-13.8043776698329,-337.348911106477)) ;
#47204=CARTESIAN_POINT('Ctrl Pts',(12.51074966661,-13.718311824526,-337.34727047152)) ;
#47205=CARTESIAN_POINT('Ctrl Pts',(12.6902062354176,-13.5523677244138,-337.344126241697)) ;
#47206=CARTESIAN_POINT('Ctrl Pts',(12.7747891388532,-13.4726674289487,-337.342624257522)) ;
#47207=CARTESIAN_POINT('Ctrl Pts',(12.9991890250577,-13.2572078996217,-337.33858503919)) ;
#47208=CARTESIAN_POINT('Ctrl Pts',(13.1376259631285,-13.1200327920946,-337.336035370251)) ;
#47209=CARTESIAN_POINT('Ctrl Pts',(13.5146768202029,-12.7344661147369,-337.328931082637)) ;
#47210=CARTESIAN_POINT('Ctrl Pts',(13.7485772278788,-12.4815760279498,-337.324339548349)) ;
#47211=CARTESIAN_POINT('Ctrl Pts',(14.311797528098,-11.8375761819423,-337.31285989267)) ;
#47212=CARTESIAN_POINT('Ctrl Pts',(14.6322550023209,-11.4390939878017,-337.305937237945)) ;
#47213=CARTESIAN_POINT('Ctrl Pts',(15.0371540915819,-10.8907105851356,-337.296824122601)) ;
#47214=CARTESIAN_POINT('Ctrl Pts',(15.1365521504998,-10.7521332464124,-337.294555377617)) ;
#47215=CARTESIAN_POINT('Ctrl Pts',(15.3067700124038,-10.5077822153238,-337.290626306693)) ;
#47216=CARTESIAN_POINT('Ctrl Pts',(15.3784374653548,-10.4026129651448,-337.288957787267)) ;
#47217=CARTESIAN_POINT('Ctrl Pts',(15.4886130381895,-10.2373073899003,-337.286375275318)) ;
#47218=CARTESIAN_POINT('Ctrl Pts',(15.5278650910516,-10.1776717462217,-337.285451637359)) ;
#47219=CARTESIAN_POINT('Ctrl Pts',(15.6005474331487,-10.0658462289691,-337.283735773406)) ;
#47220=CARTESIAN_POINT('Ctrl Pts',(15.6340622560933,-10.0137124934336,-337.282942304692)) ;
#47221=CARTESIAN_POINT('Ctrl Pts',(15.7279697342368,-9.86601474770796,-337.280711249282)) ;
#47222=CARTESIAN_POINT('Ctrl Pts',(15.7877515570531,-9.77006549592708,-337.279281702452)) ;
#47223=CARTESIAN_POINT('Ctrl Pts',(16.0208961687605,-9.38814243113036,-337.273658454331)) ;
#47224=CARTESIAN_POINT('Ctrl Pts',(16.187395595678,-9.09805238087904,-337.269533630386)) ;
#47225=CARTESIAN_POINT('Ctrl Pts',(16.5907389650162,-8.34915186103024,-337.259091233833)) ;
#47226=CARTESIAN_POINT('Ctrl Pts',(16.8164487050611,-7.8846692613911,-337.252800595879)) ;
#47227=CARTESIAN_POINT('Ctrl Pts',(17.0825826789671,-7.27341147551144,-337.244547449132)) ;
#47228=CARTESIAN_POINT('Ctrl Pts',(17.1409757950113,-7.13471052018993,-337.24267692565)) ;
#47229=CARTESIAN_POINT('Ctrl Pts',(17.2806318328654,-6.79137226132306,-337.238045680028)) ;
#47230=CARTESIAN_POINT('Ctrl Pts',(17.3599530449357,-6.58597022196559,-337.235274052071)) ;
#47231=CARTESIAN_POINT('Ctrl Pts',(17.4814971694678,-6.25376667161011,-337.230780955979)) ;
#47232=CARTESIAN_POINT('Ctrl Pts',(17.526037015956,-6.12783545161441,-337.229075401567)) ;
#47233=CARTESIAN_POINT('Ctrl Pts',(17.6099016254636,-5.88232161245492,-337.225744476818)) ;
#47234=CARTESIAN_POINT('Ctrl Pts',(17.6493768315202,-5.76279795035246,-337.224120242884)) ;
#47235=CARTESIAN_POINT('Ctrl Pts',(17.7430592433604,-5.4691501119875,-337.220122817102)) ;
#47236=CARTESIAN_POINT('Ctrl Pts',(17.79592222525,-5.29461105811313,-337.217740791508)) ;
#47237=CARTESIAN_POINT('Ctrl Pts',(18.0230514555489,-4.50282749600444,-337.206910386925)) ;
#47238=CARTESIAN_POINT('Ctrl Pts',(18.1678332642373,-3.87758533821819,-337.198274397823)) ;
#47239=CARTESIAN_POINT('Ctrl Pts',(18.3346749270021,-2.93804249638003,-337.185422898827)) ;
#47240=CARTESIAN_POINT('Ctrl Pts',(18.3815845547712,-2.62863994926851,-337.181213998003)) ;
#47241=CARTESIAN_POINT('Ctrl Pts',(18.4443520264968,-2.12988322781615,-337.174526848438)) ;
#47242=CARTESIAN_POINT('Ctrl Pts',(18.4651621523447,-1.94121383536933,-337.172019742339)) ;
#47243=CARTESIAN_POINT('Ctrl Pts',(18.4908392449272,-1.67036813412586,-337.168467697072)) ;
#47244=CARTESIAN_POINT('Ctrl Pts',(18.4980584112429,-1.58842712297686,-337.167399243618)) ;
#47245=CARTESIAN_POINT('Ctrl Pts',(18.5100986649796,-1.44052772890319,-337.165483537371)) ;
#47246=CARTESIAN_POINT('Ctrl Pts',(18.5151123225321,-1.37458663145747,-337.164634162172)) ;
#47247=CARTESIAN_POINT('Ctrl Pts',(18.5264847267926,-1.21364277579546,-337.162572001626)) ;
#47248=CARTESIAN_POINT('Ctrl Pts',(18.5324651673801,-1.1186152048318,-337.161363511053)) ;
#47249=CARTESIAN_POINT('Ctrl Pts',(18.5401905767133,-0.978698224377128,
-337.159595047726)) ;
#47250=CARTESIAN_POINT('Ctrl Pts',(18.5425039991331,-0.933842669186298,
-337.159029749726)) ;
#47251=CARTESIAN_POINT('Ctrl Pts',(18.5446545937658,-0.888979977513938,
-337.158465839576)) ;
#47252=CARTESIAN_POINT('Origin',(0.,0.,5.8748638224677)) ;
#47253=CARTESIAN_POINT('',(16.4056275812262,12.0157134421436,-20.)) ;
#47254=CARTESIAN_POINT('Ctrl Pts',(18.131496419296,-9.20710722510904,-17.3804829797999)) ;
#47255=CARTESIAN_POINT('Ctrl Pts',(18.0392880697976,-9.38869252849294,-17.3854844732659)) ;
#47256=CARTESIAN_POINT('Ctrl Pts',(17.9443414885465,-9.56891311233099,-17.3905038146911)) ;
#47257=CARTESIAN_POINT('Ctrl Pts',(17.5701229759926,-10.2540548051986,-17.4098161311144)) ;
#47258=CARTESIAN_POINT('Ctrl Pts',(17.2721382230938,-10.7483995960656,-17.4242445936442)) ;
#47259=CARTESIAN_POINT('Ctrl Pts',(16.5616564939481,-11.8210463754899,-17.4567247969065)) ;
#47260=CARTESIAN_POINT('Ctrl Pts',(16.1390709365163,-12.391770864015,-17.474830898209)) ;
#47261=CARTESIAN_POINT('Ctrl Pts',(15.396419929138,-13.2921607900915,-17.5044848954197)) ;
#47262=CARTESIAN_POINT('Ctrl Pts',(15.093490552431,-13.6351689547094,-17.5160634408531)) ;
#47263=CARTESIAN_POINT('Ctrl Pts',(14.5312552237131,-14.2300725343671,-17.536478745888)) ;
#47264=CARTESIAN_POINT('Ctrl Pts',(14.276316555976,-14.4858250926356,-17.5453598107132)) ;
#47265=CARTESIAN_POINT('Ctrl Pts',(13.6077030429862,-15.1217694594513,-17.5679043430281)) ;
#47266=CARTESIAN_POINT('Ctrl Pts',(13.1848361514893,-15.4918556985779,-17.5814829713099)) ;
#47267=CARTESIAN_POINT('Ctrl Pts',(12.2020625357566,-16.2825420008217,-17.6120991133579)) ;
#47268=CARTESIAN_POINT('Ctrl Pts',(11.6346663983223,-16.6926939839877,-17.6291545250614)) ;
#47269=CARTESIAN_POINT('Ctrl Pts',(10.5604626099482,-17.3877776884551,-17.66081384543)) ;
#47270=CARTESIAN_POINT('Ctrl Pts',(10.060414857346,-17.6818049869029,-17.6753187988438)) ;
#47271=CARTESIAN_POINT('Ctrl Pts',(8.91168051373702,-18.2927353017547,-17.7081734961953)) ;
#47272=CARTESIAN_POINT('Ctrl Pts',(8.2573031096123,-18.5972888434117,-17.726582045578)) ;
#47273=CARTESIAN_POINT('Ctrl Pts',(7.17828568172708,-19.0312729818496,-17.7561200695308)) ;
#47274=CARTESIAN_POINT('Ctrl Pts',(6.76317000345207,-19.1827180624439,-17.767292775253)) ;
#47275=CARTESIAN_POINT('Ctrl Pts',(5.99488528466534,-19.4349667135265,-17.7874535544521)) ;
#47276=CARTESIAN_POINT('Ctrl Pts',(5.64328678425831,-19.5399563845945,-17.7964725552866)) ;
#47277=CARTESIAN_POINT('Ctrl Pts',(4.72567730241938,-19.7871262705653,-17.8196808131403)) ;
#47278=CARTESIAN_POINT('Ctrl Pts',(4.15604272880859,-19.9145601152025,-17.833778605361)) ;
#47279=CARTESIAN_POINT('Ctrl Pts',(2.88299967990383,-20.1423468344708,-17.8651814896079)) ;
#47280=CARTESIAN_POINT('Ctrl Pts',(2.17822030411272,-20.230698674791,-17.8825061012518)) ;
#47281=CARTESIAN_POINT('Ctrl Pts',(0.868602317683623,-20.325634622103,-17.9150486797655)) ;
#47282=CARTESIAN_POINT('Ctrl Pts',(0.265296097316439,-20.3424556284699,
-17.9301722993868)) ;
#47283=CARTESIAN_POINT('Ctrl Pts',(-1.15491770306433,-20.3188562510556,
-17.9661045858041)) ;
#47284=CARTESIAN_POINT('Ctrl Pts',(-1.97041103215487,-20.2560417526877,
-17.987010027909)) ;
#47285=CARTESIAN_POINT('Ctrl Pts',(-3.14179443961057,-20.0943915262186,
-18.0169122951184)) ;
#47286=CARTESIAN_POINT('Ctrl Pts',(-3.50227553174102,-20.0347077715174,
-18.026089141357)) ;
#47287=CARTESIAN_POINT('Ctrl Pts',(-4.48000236353235,-19.845632091754,-18.0507675729864)) ;
#47288=CARTESIAN_POINT('Ctrl Pts',(-5.09315032155366,-19.6971918472939,
-18.0660601840092)) ;
#47289=CARTESIAN_POINT('Ctrl Pts',(-6.56815585253354,-19.2666092102568,
-18.1033282900962)) ;
#47290=CARTESIAN_POINT('Ctrl Pts',(-7.41995221080844,-18.9548726938288,
-18.125293132673)) ;
#47291=CARTESIAN_POINT('Ctrl Pts',(-8.78032793496401,-18.351208549296,-18.1621268936952)) ;
#47292=CARTESIAN_POINT('Ctrl Pts',(-9.30214924559862,-18.0922918502793,
-18.1766965533733)) ;
#47293=CARTESIAN_POINT('Ctrl Pts',(-10.4524800009425,-17.4585831937094,
-18.2098677701355)) ;
#47294=CARTESIAN_POINT('Ctrl Pts',(-11.0733330166196,-17.0715480773121,
-18.2285319087131)) ;
#47295=CARTESIAN_POINT('Ctrl Pts',(-12.0439042771515,-16.3912365423604,
-18.2586242274562)) ;
#47296=CARTESIAN_POINT('Ctrl Pts',(-12.4069834564716,-16.118158452108,-18.2701015482033)) ;
#47297=CARTESIAN_POINT('Ctrl Pts',(-13.0811835987641,-15.5747916610563,
-18.2916452857559)) ;
#47298=CARTESIAN_POINT('Ctrl Pts',(-13.3938332058954,-15.3067545477776,
-18.3017315576952)) ;
#47299=CARTESIAN_POINT('Ctrl Pts',(-14.6291706417642,-14.1808411900583,
-18.3424506717248)) ;
#47300=CARTESIAN_POINT('Ctrl Pts',(-15.4793433494829,-13.2475971267835,
-18.3727075587436)) ;
#47301=CARTESIAN_POINT('Ctrl Pts',(-16.620333960294,-11.7341595692838,-18.4197532774729)) ;
#47302=CARTESIAN_POINT('Ctrl Pts',(-16.9789651519995,-11.2089577085238,
-18.4357241466243)) ;
#47303=CARTESIAN_POINT('Ctrl Pts',(-17.7233698885513,-10.0008919602952,
-18.4716835909609)) ;
#47304=CARTESIAN_POINT('Ctrl Pts',(-18.0954493625316,-9.31076737217195,
-18.4917221776513)) ;
#47305=CARTESIAN_POINT('Ctrl Pts',(-18.5733098220373,-8.28698742482051,
-18.5202511192266)) ;
#47306=CARTESIAN_POINT('Ctrl Pts',(-18.7117895166592,-7.96937496976673,
-18.528935573816)) ;
#47307=CARTESIAN_POINT('Ctrl Pts',(-19.0774375610909,-7.06858593448309,
-18.5529948971681)) ;
#47308=CARTESIAN_POINT('Ctrl Pts',(-19.2859010918836,-6.47823755171429,
-18.5681650384943)) ;
#47309=CARTESIAN_POINT('Ctrl Pts',(-19.7235806666917,-5.02902603547314,
-18.6048806464667)) ;
#47310=CARTESIAN_POINT('Ctrl Pts',(-19.9243744415255,-4.16293504547565,
-18.6264206249536)) ;
#47311=CARTESIAN_POINT('Ctrl Pts',(-20.1618437593218,-2.71290870931743,
-18.6627820931617)) ;
#47312=CARTESIAN_POINT('Ctrl Pts',(-20.2311443524559,-2.13555772365329,
-18.6773243644515)) ;
#47313=CARTESIAN_POINT('Ctrl Pts',(-20.3312334377397,-0.831367206766867,
-18.7103583237921)) ;
#47314=CARTESIAN_POINT('Ctrl Pts',(-20.3479569346091,-0.104238561547288,
-18.7289109228162)) ;
#47315=CARTESIAN_POINT('Ctrl Pts',(-20.3116316681115,1.08238597041301,-18.7590567051804)) ;
#47316=CARTESIAN_POINT('Ctrl Pts',(-20.2819215890569,1.54194745073483,-18.7706938389194)) ;
#47317=CARTESIAN_POINT('Ctrl Pts',(-20.1964218123784,2.40701582080961,-18.7923238442201)) ;
#47318=CARTESIAN_POINT('Ctrl Pts',(-20.1439404616109,2.8126223988546,-18.802342674701)) ;
#47319=CARTESIAN_POINT('Ctrl Pts',(-19.8777793350564,4.47422145692789,-18.8433429946405)) ;
#47320=CARTESIAN_POINT('Ctrl Pts',(-19.5585444436011,5.71035190922039,-18.8739342271753)) ;
#47321=CARTESIAN_POINT('Ctrl Pts',(-18.9064149085717,7.51574001898014,-18.9215985866594)) ;
#47322=CARTESIAN_POINT('Ctrl Pts',(-18.6582669194175,8.1122091081497,-18.9378313896639)) ;
#47323=CARTESIAN_POINT('Ctrl Pts',(-18.042613859589,9.41363785633099,-18.9743314254983)) ;
#47324=CARTESIAN_POINT('Ctrl Pts',(-17.6613113815884,10.1109134205892,-18.9946466873114)) ;
#47325=CARTESIAN_POINT('Ctrl Pts',(-17.062985930353,11.0674381369411,-19.0231005806699)) ;
#47326=CARTESIAN_POINT('Ctrl Pts',(-16.8787946855523,11.3463637879838,-19.0314635066024)) ;
#47327=CARTESIAN_POINT('Ctrl Pts',(-16.3482877364534,12.1081986931649,-19.0544110746184)) ;
#47328=CARTESIAN_POINT('Ctrl Pts',(-15.9875575837926,12.5806597499504,-19.0688219222257)) ;
#47329=CARTESIAN_POINT('Ctrl Pts',(-15.027264263384,13.7302625779835,-19.1051518820726)) ;
#47330=CARTESIAN_POINT('Ctrl Pts',(-14.4022799806571,14.3844743018147,-19.1270626367402)) ;
#47331=CARTESIAN_POINT('Ctrl Pts',(-13.3066276267042,15.3881280367831,-19.1638352984844)) ;
#47332=CARTESIAN_POINT('Ctrl Pts',(-12.860715339133,15.7627033012444,-19.1784005190965)) ;
#47333=CARTESIAN_POINT('Ctrl Pts',(-11.8204440375694,16.5629878757434,-19.2115495917081)) ;
#47334=CARTESIAN_POINT('Ctrl Pts',(-11.2179617554914,16.9768310124098,-19.2301957471706)) ;
#47335=CARTESIAN_POINT('Ctrl Pts',(-10.2059338281782,17.5945493022491,-19.2602986820123)) ;
#47336=CARTESIAN_POINT('Ctrl Pts',(-9.80948093800944,17.8186233743188,-19.2718037416389)) ;
#47337=CARTESIAN_POINT('Ctrl Pts',(-9.03996607034749,18.2200795073311,-19.2933981553172)) ;
#47338=CARTESIAN_POINT('Ctrl Pts',(-8.66836432068795,18.3997757310214,-19.3035075428875)) ;
#47339=CARTESIAN_POINT('Ctrl Pts',(-7.14632614940413,19.0794412868354,-19.3441158933636)) ;
#47340=CARTESIAN_POINT('Ctrl Pts',(-5.95624797314513,19.4837926646047,-19.3742441947023)) ;
#47341=CARTESIAN_POINT('Ctrl Pts',(-4.12108653028286,19.9233309719072,-19.4210791918915)) ;
#47342=CARTESIAN_POINT('Ctrl Pts',(-3.49911297105361,20.0419227756955,-19.4369773843277)) ;
#47343=CARTESIAN_POINT('Ctrl Pts',(-2.09862764729727,20.241764340111,-19.4728226578717)) ;
#47344=CARTESIAN_POINT('Ctrl Pts',(-1.31890353021939,20.3074801811141,-19.4928210962884)) ;
#47345=CARTESIAN_POINT('Ctrl Pts',(-0.187803421990395,20.337378771627,-19.5214014161937)) ;
#47346=CARTESIAN_POINT('Ctrl Pts',(0.161914956698301,20.3376015066546,-19.5301707882459)) ;
#47347=CARTESIAN_POINT('Ctrl Pts',(1.15595780452201,20.312591554997,-19.5547863673276)) ;
#47348=CARTESIAN_POINT('Ctrl Pts',(1.79931576067825,20.2657368425544,-19.5704073318224)) ;
#47349=CARTESIAN_POINT('Ctrl Pts',(3.30625118125827,20.0836539576361,-19.607215050388)) ;
#47350=CARTESIAN_POINT('Ctrl Pts',(4.16548676969294,19.923181500246,-19.6283980813291)) ;
#47351=CARTESIAN_POINT('Ctrl Pts',(5.57236233053807,19.5654130363426,-19.6643152294202)) ;
#47352=CARTESIAN_POINT('Ctrl Pts',(6.12664242751008,19.3989910319172,-19.6787849902183)) ;
#47353=CARTESIAN_POINT('Ctrl Pts',(7.3512118882454,18.9735881024619,-19.7115176714718)) ;
#47354=CARTESIAN_POINT('Ctrl Pts',(8.01640277169513,18.7022629887867,-19.7298383725935)) ;
#47355=CARTESIAN_POINT('Ctrl Pts',(9.06919283051794,18.206331787221,-19.7593974306874)) ;
#47356=CARTESIAN_POINT('Ctrl Pts',(9.4661845219242,18.0031144675481,-19.7706756191561)) ;
#47357=CARTESIAN_POINT('Ctrl Pts',(10.1794300911626,17.6078893296198,-19.7910070494607)) ;
#47358=CARTESIAN_POINT('Ctrl Pts',(10.4977411847119,17.4199883525408,-19.8000923211161)) ;
#47359=CARTESIAN_POINT('Ctrl Pts',(11.8216570136236,16.5890007556669,-19.838268640101)) ;
#47360=CARTESIAN_POINT('Ctrl Pts',(12.774733576001,15.8667174416586,-19.8668885241356)) ;
#47361=CARTESIAN_POINT('Ctrl Pts',(14.05552448074,14.7054672911806,-19.9095925665322)) ;
#47362=CARTESIAN_POINT('Ctrl Pts',(14.4377408826382,14.3303931535161,-19.9229461035312)) ;
#47363=CARTESIAN_POINT('Ctrl Pts',(15.3773834578425,13.3325123212659,-19.9574605973473)) ;
#47364=CARTESIAN_POINT('Ctrl Pts',(15.9120360749949,12.6896375056191,-19.9787923753823)) ;
#47365=CARTESIAN_POINT('Ctrl Pts',(16.4056275812262,12.0157134421436,-20.)) ;
#47366=CARTESIAN_POINT('',(-6.42208446149247,19.2945281628512,-20.)) ;
#47367=CARTESIAN_POINT('Origin',(0.,0.,-20.)) ;
#47368=CARTESIAN_POINT('Ctrl Pts',(-6.42208446149245,19.2945281628512,-20.)) ;
#47369=CARTESIAN_POINT('Ctrl Pts',(-7.54571498564493,18.9205335220539,-19.9705725095626)) ;
#47370=CARTESIAN_POINT('Ctrl Pts',(-8.63452990372283,18.4491019182255,-19.9421975689781)) ;
#47371=CARTESIAN_POINT('Ctrl Pts',(-10.1459115821159,17.6314420079567,-19.9000036142141)) ;
#47372=CARTESIAN_POINT('Ctrl Pts',(-10.6054902547094,17.3588835819478,-19.8867846332647)) ;
#47373=CARTESIAN_POINT('Ctrl Pts',(-11.9472687509246,16.4899314064032,-19.8467902829131)) ;
#47374=CARTESIAN_POINT('Ctrl Pts',(-12.7939173067031,15.8420548380586,-19.8195712878972)) ;
#47375=CARTESIAN_POINT('Ctrl Pts',(-13.9842075231014,14.7733010061046,-19.7787395703855)) ;
#47376=CARTESIAN_POINT('Ctrl Pts',(-14.3682039091627,14.4001113127303,-19.7651257336831)) ;
#47377=CARTESIAN_POINT('Ctrl Pts',(-14.9683002199986,13.768973175322,-19.7433693969149)) ;
#47378=CARTESIAN_POINT('Ctrl Pts',(-15.1935127722465,13.520051913782,-19.7350962864897)) ;
#47379=CARTESIAN_POINT('Ctrl Pts',(-15.9335392446829,12.6602665613523,-19.7073313067766)) ;
#47380=CARTESIAN_POINT('Ctrl Pts',(-16.4184954931035,12.0246845484445,-19.6881006359245)) ;
#47381=CARTESIAN_POINT('Ctrl Pts',(-17.2171424766637,10.8392629004378,-19.6532888760962)) ;
#47382=CARTESIAN_POINT('Ctrl Pts',(-17.5449572090063,10.300198181734,-19.6378172777258)) ;
#47383=CARTESIAN_POINT('Ctrl Pts',(-18.3925895184266,8.74811018225945,-19.5938446790031)) ;
#47384=CARTESIAN_POINT('Ctrl Pts',(-18.8531967406469,7.70543268113117,-19.5648555002104)) ;
#47385=CARTESIAN_POINT('Ctrl Pts',(-19.3390435870962,6.29662912142951,-19.5270029720676)) ;
#47386=CARTESIAN_POINT('Ctrl Pts',(-19.4452445627443,5.96058812792489,-19.5180795762446)) ;
#47387=CARTESIAN_POINT('Ctrl Pts',(-19.6305781766564,5.31634412890872,-19.5012577483459)) ;
#47388=CARTESIAN_POINT('Ctrl Pts',(-19.7113142315708,5.00871318993154,-19.4933601878428)) ;
#47389=CARTESIAN_POINT('Ctrl Pts',(-19.976994825352,3.89015795895933,-19.4650831866032)) ;
#47390=CARTESIAN_POINT('Ctrl Pts',(-20.1193671996939,3.06997267309098,-19.4450654003448)) ;
#47391=CARTESIAN_POINT('Ctrl Pts',(-20.2856203357511,1.57215683266874,-19.4084118232149)) ;
#47392=CARTESIAN_POINT('Ctrl Pts',(-20.3266397573979,0.897649872820425,
-19.3918768530545)) ;
#47393=CARTESIAN_POINT('Ctrl Pts',(-20.3411464537278,-0.4289457122021,-19.358925212286)) ;
#47394=CARTESIAN_POINT('Ctrl Pts',(-20.316972380584,-1.08021060794756,-19.3425451896674)) ;
#47395=CARTESIAN_POINT('Ctrl Pts',(-20.2047868624575,-2.39473514853497,
-19.3090962526814)) ;
#47396=CARTESIAN_POINT('Ctrl Pts',(-20.1152286599606,-3.05708074427671,
-19.2920406744007)) ;
#47397=CARTESIAN_POINT('Ctrl Pts',(-19.9221328784407,-4.09660761996546,
-19.2652764658035)) ;
#47398=CARTESIAN_POINT('Ctrl Pts',(-19.8400481041837,-4.47728374715785,
-19.2554806275714)) ;
#47399=CARTESIAN_POINT('Ctrl Pts',(-19.6242251330395,-5.355048577903,-19.2330595194619)) ;
#47400=CARTESIAN_POINT('Ctrl Pts',(-19.4824433060686,-5.84988613599767,
-19.2205251144961)) ;
#47401=CARTESIAN_POINT('Ctrl Pts',(-19.1080581525078,-6.99109103039179,
-19.191361003802)) ;
#47402=CARTESIAN_POINT('Ctrl Pts',(-18.8611800192939,-7.63211157594126,
-19.1747723303905)) ;
#47403=CARTESIAN_POINT('Ctrl Pts',(-18.3513642252671,-8.779115095633,-19.1440765904924)) ;
#47404=CARTESIAN_POINT('Ctrl Pts',(-18.098672083105,-9.2888907775145,-19.1300488599284)) ;
#47405=CARTESIAN_POINT('Ctrl Pts',(-17.3838252732944,-10.590779540001,-19.092982809457)) ;
#47406=CARTESIAN_POINT('Ctrl Pts',(-16.8888974076893,-11.3634108985209,
-19.0696867614093)) ;
#47407=CARTESIAN_POINT('Ctrl Pts',(-15.9795337904982,-12.591693677508,-19.0307844809173)) ;
#47408=CARTESIAN_POINT('Ctrl Pts',(-15.5935090752394,-13.0667031896461,
-19.0152319620333)) ;
#47409=CARTESIAN_POINT('Ctrl Pts',(-14.9408962332899,-13.7995714139715,
-18.9907698364742)) ;
#47410=CARTESIAN_POINT('Ctrl Pts',(-14.6876572894402,-14.0688050518226,
-18.9816878457799)) ;
#47411=CARTESIAN_POINT('Ctrl Pts',(-13.8758016307955,-14.8861124076801,
-18.9535595955181)) ;
#47412=CARTESIAN_POINT('Ctrl Pts',(-13.292799794239,-15.408948506576,-18.9347128214389)) ;
#47413=CARTESIAN_POINT('Ctrl Pts',(-12.1995339469984,-16.2810586743814,
-18.9006225636591)) ;
#47414=CARTESIAN_POINT('Ctrl Pts',(-11.700739747079,-16.6431421471916,-18.8854887862647)) ;
#47415=CARTESIAN_POINT('Ctrl Pts',(-10.5940858660567,-17.3721097278627,
-18.8525118436365)) ;
#47416=CARTESIAN_POINT('Ctrl Pts',(-9.98189435482839,-17.7309509640586,
-18.8346221442252)) ;
#47417=CARTESIAN_POINT('Ctrl Pts',(-8.82726945297243,-18.3289604427553,
-18.8015896385066)) ;
#47418=CARTESIAN_POINT('Ctrl Pts',(-8.29071525236168,-18.5778232834481,
-18.7865055273131)) ;
#47419=CARTESIAN_POINT('Ctrl Pts',(-7.4025904895691,-18.9436015118526,-18.762216332225)) ;
#47420=CARTESIAN_POINT('Ctrl Pts',(-7.05732577562666,-19.0749192245182,
-18.7529378888639)) ;
#47421=CARTESIAN_POINT('Ctrl Pts',(-6.28728242922303,-19.3440254796917,
-18.7327229980836)) ;
#47422=CARTESIAN_POINT('Ctrl Pts',(-5.8611544756378,-19.4773744475153,-18.721828990046)) ;
#47423=CARTESIAN_POINT('Ctrl Pts',(-4.73953746200831,-19.788218377024,-18.6935374442036)) ;
#47424=CARTESIAN_POINT('Ctrl Pts',(-4.03843667378955,-19.9431148823256,
-18.6762152167227)) ;
#47425=CARTESIAN_POINT('Ctrl Pts',(-2.76005634444794,-20.1553613272529,
-18.6445452508762)) ;
#47426=CARTESIAN_POINT('Ctrl Pts',(-2.18571633844797,-20.2257048668193,
-18.6302907601886)) ;
#47427=CARTESIAN_POINT('Ctrl Pts',(-0.923294002832888,-20.3259168481181,
-18.598704599547)) ;
#47428=CARTESIAN_POINT('Ctrl Pts',(-0.235108075118919,-20.3455174101044,
-18.5813167925383)) ;
#47429=CARTESIAN_POINT('Ctrl Pts',(1.02241373347908,-20.317513281118,-18.5493380518093)) ;
#47430=CARTESIAN_POINT('Ctrl Pts',(1.59130339713737,-20.2808882980299,-18.534798406541)) ;
#47431=CARTESIAN_POINT('Ctrl Pts',(2.51888859506176,-20.1818973626806,-18.5112095472917)) ;
#47432=CARTESIAN_POINT('Ctrl Pts',(2.87878247588108,-20.1337129863791,-18.5020908386088)) ;
#47433=CARTESIAN_POINT('Ctrl Pts',(3.67771435434724,-20.0048869989137,-18.4820370164804)) ;
#47434=CARTESIAN_POINT('Ctrl Pts',(4.11577711690003,-19.919374249163,-18.4711476139617)) ;
#47435=CARTESIAN_POINT('Ctrl Pts',(5.25042337946643,-19.6588530614843,-18.4428501496224)) ;
#47436=CARTESIAN_POINT('Ctrl Pts',(5.94117238174564,-19.4612414859511,-18.4255175039371)) ;
#47437=CARTESIAN_POINT('Ctrl Pts',(7.16761236786596,-19.0389789873187,-18.3938184776607)) ;
#47438=CARTESIAN_POINT('Ctrl Pts',(7.70689567547357,-18.8271383639402,-18.3795452897704)) ;
#47439=CARTESIAN_POINT('Ctrl Pts',(8.85389579923341,-18.3190241824908,-18.3482561934812)) ;
#47440=CARTESIAN_POINT('Ctrl Pts',(9.45737807719095,-18.0148856618515,-18.3311935019025)) ;
#47441=CARTESIAN_POINT('Ctrl Pts',(10.5452420009221,-17.3968786234229,-18.2993935396737)) ;
#47442=CARTESIAN_POINT('Ctrl Pts',(11.0335764341507,-17.0913342525883,-18.2847025827745)) ;
#47443=CARTESIAN_POINT('Ctrl Pts',(11.8091211314112,-16.558979096446,-18.2609167990149)) ;
#47444=CARTESIAN_POINT('Ctrl Pts',(12.1043472471194,-16.3444153955662,-18.2517514945396)) ;
#47445=CARTESIAN_POINT('Ctrl Pts',(12.7495456306156,-15.8484255848568,-18.231585389155)) ;
#47446=CARTESIAN_POINT('Ctrl Pts',(13.0962931409228,-15.5631172451814,-18.2206311136396)) ;
#47447=CARTESIAN_POINT('Ctrl Pts',(13.9708355679073,-14.7935922487522,-18.1923172717652)) ;
#47448=CARTESIAN_POINT('Ctrl Pts',(14.4830007830972,-14.2925612255671,-18.1750308200972)) ;
#47449=CARTESIAN_POINT('Ctrl Pts',(15.3592998966792,-13.339737377673,-18.1433928139863)) ;
#47450=CARTESIAN_POINT('Ctrl Pts',(15.7325739393583,-12.8973949257823,-18.1291335339469)) ;
#47451=CARTESIAN_POINT('Ctrl Pts',(16.4991502949351,-11.906095263746,-18.0978771568599)) ;
#47452=CARTESIAN_POINT('Ctrl Pts',(16.8850095394674,-11.3522467141343,-18.0808334142567)) ;
#47453=CARTESIAN_POINT('Ctrl Pts',(17.5481505136909,-10.2915765998809,-18.0490381106713)) ;
#47454=CARTESIAN_POINT('Ctrl Pts',(17.8327627888323,-9.79013316761127,-18.0343325139809)) ;
#47455=CARTESIAN_POINT('Ctrl Pts',(18.1076721718333,-9.25391181964499,-18.0190947825227)) ;
#47456=CARTESIAN_POINT('Ctrl Pts',(18.1196070436432,-9.23052089544325,-18.0184310503742)) ;
#47457=CARTESIAN_POINT('Ctrl Pts',(18.1314964403967,-9.20710718355568,-18.0177676543358)) ;
#47458=CARTESIAN_POINT('Origin',(0.,0.,-10.)) ;
#47459=CARTESIAN_POINT('',(-15.4053915293257,-15.8878358795928,-19.9995644016859)) ;
#47460=CARTESIAN_POINT('Ctrl Pts',(0.000517204814065366,-22.1295393890992,
-19.6112894184499)) ;
#47461=CARTESIAN_POINT('Ctrl Pts',(-0.443938333285866,-22.1294510254483,
-19.6216081794502)) ;
#47462=CARTESIAN_POINT('Ctrl Pts',(-0.888412087382889,-22.1159901751952,
-19.631889439891)) ;
#47463=CARTESIAN_POINT('Ctrl Pts',(-1.33208775265979,-22.089181583779,-19.6421021187407)) ;
#47464=CARTESIAN_POINT('Ctrl Pts',(-1.77574594138311,-22.0623740483635,
-19.6523143953091)) ;
#47465=CARTESIAN_POINT('Ctrl Pts',(-2.21860527133772,-22.0222244031857,
-19.6624606548461)) ;
#47466=CARTESIAN_POINT('Ctrl Pts',(-2.6598611774855,-21.9688516945317,-19.6725658729284)) ;
#47467=CARTESIAN_POINT('Ctrl Pts',(-3.10116451285207,-21.9154732490119,
-19.682672177189)) ;
#47468=CARTESIAN_POINT('Ctrl Pts',(-3.54085748810537,-21.8488099814255,
-19.6927032784351)) ;
#47469=CARTESIAN_POINT('Ctrl Pts',(-3.97813233981979,-21.7689943996938,
-19.7026926516773)) ;
#47470=CARTESIAN_POINT('Ctrl Pts',(-4.41541786596682,-21.6891768695626,
-19.7126822687728)) ;
#47471=CARTESIAN_POINT('Ctrl Pts',(-4.85028556482805,-21.5962062291834,
-19.7226302422428)) ;
#47472=CARTESIAN_POINT('Ctrl Pts',(-5.28192893157152,-21.490233790291,-19.7325803346779)) ;
#47473=CARTESIAN_POINT('Ctrl Pts',(-5.7136591075495,-21.3842400389287,-19.7425324282092)) ;
#47474=CARTESIAN_POINT('Ctrl Pts',(-6.14216362728143,-21.2652390974891,
-19.7524867832956)) ;
#47475=CARTESIAN_POINT('Ctrl Pts',(-6.56663819984437,-21.133423656613,-19.7625076025576)) ;
#47476=CARTESIAN_POINT('Ctrl Pts',(-6.85602864659768,-21.0435569560147,
-19.7693394119297)) ;
#47477=CARTESIAN_POINT('Ctrl Pts',(-7.14354602853844,-20.9477349414254,
-19.7762025441723)) ;
#47478=CARTESIAN_POINT('Ctrl Pts',(-7.4289363685051,-20.8460303363535,-19.7831221737644)) ;
#47479=CARTESIAN_POINT('Ctrl Pts',(-7.84649270955411,-20.6972257104976,
-19.793246325879)) ;
#47480=CARTESIAN_POINT('Ctrl Pts',(-8.25960939184134,-20.5357846370997,
-19.8034926402938)) ;
#47481=CARTESIAN_POINT('Ctrl Pts',(-8.66753180167299,-20.3620402476045,
-19.8137830126411)) ;
#47482=CARTESIAN_POINT('Ctrl Pts',(-9.07538988208743,-20.1883232576222,
-19.8240717621953)) ;
#47483=CARTESIAN_POINT('Ctrl Pts',(-9.47805541762666,-20.0023069804755,
-19.8344044009316)) ;
#47484=CARTESIAN_POINT('Ctrl Pts',(-9.87479772637341,-19.8043587983951,
-19.8447226647033)) ;
#47485=CARTESIAN_POINT('Ctrl Pts',(-10.2714974529698,-19.6064318619925,
-19.8550398210211)) ;
#47486=CARTESIAN_POINT('Ctrl Pts',(-10.6622752997502,-19.3965756633295,
-19.865342510328)) ;
#47487=CARTESIAN_POINT('Ctrl Pts',(-11.0464231416791,-19.1751901534458,
-19.8755941555047)) ;
#47488=CARTESIAN_POINT('Ctrl Pts',(-11.4416425018511,-18.9474240956482,
-19.8861412631681)) ;
#47489=CARTESIAN_POINT('Ctrl Pts',(-11.8298441287601,-18.7074544386025,
-19.8966341791439)) ;
#47490=CARTESIAN_POINT('Ctrl Pts',(-12.2102804888824,-18.4557519688425,
-19.9070581446796)) ;
#47491=CARTESIAN_POINT('Ctrl Pts',(-12.5800624893015,-18.2110985851639,
-19.9171901805)) ;
#47492=CARTESIAN_POINT('Ctrl Pts',(-12.942508194326,-17.9553604838846,-19.927257195051)) ;
#47493=CARTESIAN_POINT('Ctrl Pts',(-13.2969522795948,-17.6890023990348,
-19.9372689073098)) ;
#47494=CARTESIAN_POINT('Ctrl Pts',(-13.6667150179138,-17.4111326336167,
-19.9477133139)) ;
#47495=CARTESIAN_POINT('Ctrl Pts',(-14.0277693542131,-17.1217047382201,
-19.9580974249735)) ;
#47496=CARTESIAN_POINT('Ctrl Pts',(-14.3793841502957,-16.8212842661519,
-19.9684582702009)) ;
#47497=CARTESIAN_POINT('Ctrl Pts',(-14.7309989463784,-16.5208637940836,
-19.9788191154282)) ;
#47498=CARTESIAN_POINT('Ctrl Pts',(-15.0731741100143,-16.209450612742,-19.9891568361822)) ;
#47499=CARTESIAN_POINT('Ctrl Pts',(-15.4052041408659,-15.8876506360391,
-19.9995334132552)) ;
#47500=CARTESIAN_POINT('Origin',(0.,0.,-20.)) ;
#47501=CARTESIAN_POINT('Origin',(0.,0.,-328.125)) ;
#47502=CARTESIAN_POINT('',(1.53120055501316,-19.364905768565,-337.99978912964)) ;
#47503=CARTESIAN_POINT('Ctrl Pts',(2.0594453916303E-9,-19.425,-336.519643262718)) ;
#47504=CARTESIAN_POINT('Ctrl Pts',(-0.0932399363564652,-19.4250000000099,
-336.520817928714)) ;
#47505=CARTESIAN_POINT('Ctrl Pts',(-0.186482031227195,-19.4243286729344,
-336.521988828568)) ;
#47506=CARTESIAN_POINT('Ctrl Pts',(-0.437812431282591,-19.420709152349,
-336.525134336585)) ;
#47507=CARTESIAN_POINT('Ctrl Pts',(-0.595872264667102,-19.4165022608218,
-336.527101170528)) ;
#47508=CARTESIAN_POINT('Ctrl Pts',(-0.877973804678461,-19.4055459512161,
-336.530591059154)) ;
#47509=CARTESIAN_POINT('Ctrl Pts',(-1.00203536493703,-19.399535480021,-336.532118765596)) ;
#47510=CARTESIAN_POINT('Ctrl Pts',(-1.27015707153849,-19.3839667876486,
-336.535405727605)) ;
#47511=CARTESIAN_POINT('Ctrl Pts',(-1.41418564513392,-19.3739914948649,
-336.537162194948)) ;
#47512=CARTESIAN_POINT('Ctrl Pts',(-1.83867860905591,-19.3398326232978,
-336.542314408147)) ;
#47513=CARTESIAN_POINT('Ctrl Pts',(-2.11874382755672,-19.3111571366231,
-336.545681488894)) ;
#47514=CARTESIAN_POINT('Ctrl Pts',(-2.80579095317782,-19.2256848282012,
-336.553891732014)) ;
#47515=CARTESIAN_POINT('Ctrl Pts',(-3.21178331669986,-19.1620423860537,
-336.558698785826)) ;
#47516=CARTESIAN_POINT('Ctrl Pts',(-4.15907185381896,-18.9825939798755,
-336.569960638012)) ;
#47517=CARTESIAN_POINT('Ctrl Pts',(-4.69804248177032,-18.8564351352946,
-336.576400596075)) ;
#47518=CARTESIAN_POINT('Ctrl Pts',(-5.34085268612161,-18.6766955049485,
-336.584413229374)) ;
#47519=CARTESIAN_POINT('Ctrl Pts',(-5.45054292064655,-18.6449790617679,
-336.585792685071)) ;
#47520=CARTESIAN_POINT('Ctrl Pts',(-5.61962219651297,-18.5944709599256,
-336.587941886695)) ;
#47521=CARTESIAN_POINT('Ctrl Pts',(-5.67921127609178,-18.576357640339,-336.588703753552)) ;
#47522=CARTESIAN_POINT('Ctrl Pts',(-5.80618975223359,-18.5370918480951,
-336.590337599799)) ;
#47523=CARTESIAN_POINT('Ctrl Pts',(-5.87355296840774,-18.5158577746769,
-336.591210649143)) ;
#47524=CARTESIAN_POINT('Ctrl Pts',(-6.05719493870232,-18.4568675697922,
-336.593606392374)) ;
#47525=CARTESIAN_POINT('Ctrl Pts',(-6.17323538701914,-18.4183803794854,
-336.595137448162)) ;
#47526=CARTESIAN_POINT('Ctrl Pts',(-6.69814358877089,-18.2387659571691,
-336.602129414365)) ;
#47527=CARTESIAN_POINT('Ctrl Pts',(-7.10259073286086,-18.0851020201597,
-336.607697398786)) ;
#47528=CARTESIAN_POINT('Ctrl Pts',(-8.14504514366601,-17.6486685146565,
-336.622273874247)) ;
#47529=CARTESIAN_POINT('Ctrl Pts',(-8.77354446913076,-17.3448028278548,
-336.631274998696)) ;
#47530=CARTESIAN_POINT('Ctrl Pts',(-9.54353642583983,-16.9199467795189,
-336.642327423058)) ;
#47531=CARTESIAN_POINT('Ctrl Pts',(-9.70149727682105,-16.829873358518,-336.644597576333)) ;
#47532=CARTESIAN_POINT('Ctrl Pts',(-9.96663503107536,-16.673711551087,-336.648411961506)) ;
#47533=CARTESIAN_POINT('Ctrl Pts',(-10.0744762034533,-16.6087747894376,
-336.649964558199)) ;
#47534=CARTESIAN_POINT('Ctrl Pts',(-10.2951897376559,-16.4729310964918,
-336.653144959106)) ;
#47535=CARTESIAN_POINT('Ctrl Pts',(-10.4079788399579,-16.4019013278264,
-336.654771724497)) ;
#47536=CARTESIAN_POINT('Ctrl Pts',(-10.7026634114779,-16.2120578610165,
-336.659027533178)) ;
#47537=CARTESIAN_POINT('Ctrl Pts',(-10.8833122174686,-16.0913436227656,
-336.661641959856)) ;
#47538=CARTESIAN_POINT('Ctrl Pts',(-11.1823562497442,-15.8841747560948,
-336.665986907985)) ;
#47539=CARTESIAN_POINT('Ctrl Pts',(-11.3018661284412,-15.7993645773874,
-336.667728062783)) ;
#47540=CARTESIAN_POINT('Ctrl Pts',(-11.8073219637408,-15.4319978673641,
-336.675121317241)) ;
#47541=CARTESIAN_POINT('Ctrl Pts',(-12.1837204501755,-15.1365903169809,
-336.680696112652)) ;
#47542=CARTESIAN_POINT('Ctrl Pts',(-12.8827794222124,-14.5449654146986,
-336.691396514641)) ;
#47543=CARTESIAN_POINT('Ctrl Pts',(-13.2070842919666,-14.2511384541469,
-336.696517709031)) ;
#47544=CARTESIAN_POINT('Ctrl Pts',(-13.6071877956029,-13.8632395980686,
-336.703199766062)) ;
#47545=CARTESIAN_POINT('Ctrl Pts',(-13.6924122803886,-13.7790717299404,
-336.704645401288)) ;
#47546=CARTESIAN_POINT('Ctrl Pts',(-13.8214511986546,-13.6492532364941,
-336.706873235367)) ;
#47547=CARTESIAN_POINT('Ctrl Pts',(-13.8658301763447,-13.6041677680148,
-336.707646616925)) ;
#47548=CARTESIAN_POINT('Ctrl Pts',(-13.9584666964118,-13.5091323235117,
-336.709277089246)) ;
#47549=CARTESIAN_POINT('Ctrl Pts',(-14.0066781541244,-13.4591387430914,
-336.710135019795)) ;
#47550=CARTESIAN_POINT('Ctrl Pts',(-14.1348614913577,-13.3247824730548,
-336.712439903972)) ;
#47551=CARTESIAN_POINT('Ctrl Pts',(-14.2143459513204,-13.2399587027821,
-336.713894223156)) ;
#47552=CARTESIAN_POINT('Ctrl Pts',(-14.5497838709389,-12.8754855253364,
-336.720129798047)) ;
#47553=CARTESIAN_POINT('Ctrl Pts',(-14.7982826011156,-12.5890892999906,
-336.724994902363)) ;
#47554=CARTESIAN_POINT('Ctrl Pts',(-15.5393599941566,-11.6827085792831,
-336.74008021623)) ;
#47555=CARTESIAN_POINT('Ctrl Pts',(-16.0025444915835,-11.0397449952403,
-336.750323075549)) ;
#47556=CARTESIAN_POINT('Ctrl Pts',(-16.5066143176558,-10.2413653851955,
-336.762164130865)) ;
#47557=CARTESIAN_POINT('Ctrl Pts',(-16.5865072431808,-10.111461750974,-336.764065870962)) ;
#47558=CARTESIAN_POINT('Ctrl Pts',(-16.7295214137403,-9.87266807926668,
-336.767516173564)) ;
#47559=CARTESIAN_POINT('Ctrl Pts',(-16.79312990494,-9.76407956648395,-336.769068295499)) ;
#47560=CARTESIAN_POINT('Ctrl Pts',(-16.9219603268634,-9.53916490331754,
-336.772249007843)) ;
#47561=CARTESIAN_POINT('Ctrl Pts',(-16.9870485830582,-9.42276970164219,
-336.773876546069)) ;
#47562=CARTESIAN_POINT('Ctrl Pts',(-17.1551866137313,-9.11468904250896,
-336.778137517084)) ;
#47563=CARTESIAN_POINT('Ctrl Pts',(-17.2562226619409,-8.92192601160737,
-336.780756263977)) ;
#47564=CARTESIAN_POINT('Ctrl Pts',(-17.4200006206966,-8.59626567971618,
-336.78510972126)) ;
#47565=CARTESIAN_POINT('Ctrl Pts',(-17.4845118295128,-8.4642809146057,-336.786855079297)) ;
#47566=CARTESIAN_POINT('Ctrl Pts',(-17.7535687328234,-7.89760772597241,
-336.794276859595)) ;
#47567=CARTESIAN_POINT('Ctrl Pts',(-17.9434481261956,-7.45614378709459,
-336.799875357001)) ;
#47568=CARTESIAN_POINT('Ctrl Pts',(-18.2783043009703,-6.59050055233403,
-336.810720433661)) ;
#47569=CARTESIAN_POINT('Ctrl Pts',(-18.4253553299155,-6.16744554815007,
-336.81596267458)) ;
#47570=CARTESIAN_POINT('Ctrl Pts',(-18.5909222067315,-5.63213207966579,
-336.822691517152)) ;
#47571=CARTESIAN_POINT('Ctrl Pts',(-18.6232528645947,-5.52428755110498,
-336.824052080844)) ;
#47572=CARTESIAN_POINT('Ctrl Pts',(-18.6719336766177,-5.35661860306861,
-336.826178946924)) ;
#47573=CARTESIAN_POINT('Ctrl Pts',(-18.6889379856181,-5.29698660022334,
-336.82693763165)) ;
#47574=CARTESIAN_POINT('Ctrl Pts',(-18.7248065741668,-5.16887692633256,
-336.828573314663)) ;
#47575=CARTESIAN_POINT('Ctrl Pts',(-18.7435813891906,-5.1003751440834,-336.829451452423)) ;
#47576=CARTESIAN_POINT('Ctrl Pts',(-18.7941633921243,-4.91176991077936,
-336.831877348192)) ;
#47577=CARTESIAN_POINT('Ctrl Pts',(-18.8251946493792,-4.79146194903191,
-336.833433805025)) ;
#47578=CARTESIAN_POINT('Ctrl Pts',(-18.8944370392451,-4.51194837952161,
-336.837064297007)) ;
#47579=CARTESIAN_POINT('Ctrl Pts',(-18.9317938281932,-4.35254081475044,
-336.839145477567)) ;
#47580=CARTESIAN_POINT('Ctrl Pts',(-19.0646827902067,-3.75136873252276,
-336.847012439797)) ;
#47581=CARTESIAN_POINT('Ctrl Pts',(-19.1468027682881,-3.30678710058974,
-336.852863885669)) ;
#47582=CARTESIAN_POINT('Ctrl Pts',(-19.2246853040365,-2.78352972482662,
-336.859680770063)) ;
#47583=CARTESIAN_POINT('Ctrl Pts',(-19.2355759996943,-2.70724559876217,
-336.860672957291)) ;
#47584=CARTESIAN_POINT('Ctrl Pts',(-19.3082840794795,-2.17535867310543,
-336.867577301558)) ;
#47585=CARTESIAN_POINT('Ctrl Pts',(-19.3543626779806,-1.71775049508685,
-336.873443741863)) ;
#47586=CARTESIAN_POINT('Ctrl Pts',(-19.3941296516603,-1.10544937641824,
-336.881140759919)) ;
#47587=CARTESIAN_POINT('Ctrl Pts',(-19.4022748737262,-0.951847193779062,
-336.88305930149)) ;
#47588=CARTESIAN_POINT('Ctrl Pts',(-19.4137775513485,-0.672141883388968,
-336.886530025245)) ;
#47589=CARTESIAN_POINT('Ctrl Pts',(-19.4177325949734,-0.546071830203471,
-336.888085926079)) ;
#47590=CARTESIAN_POINT('Ctrl Pts',(-19.4233317105399,-0.287156076884228,
-336.891264417035)) ;
#47591=CARTESIAN_POINT('Ctrl Pts',(-19.4248413276285,-0.15431397456903,
-336.892886058407)) ;
#47592=CARTESIAN_POINT('Ctrl Pts',(-19.4252255241112,0.193340499314378,
-336.897107539617)) ;
#47593=CARTESIAN_POINT('Ctrl Pts',(-19.4218997918328,0.408137110628826,
-336.899693220993)) ;
#47594=CARTESIAN_POINT('Ctrl Pts',(-19.4103906319138,0.766900900875649,
-336.903981670201)) ;
#47595=CARTESIAN_POINT('Ctrl Pts',(-19.4041655807187,0.91091143649217,-336.905694974084)) ;
#47596=CARTESIAN_POINT('Ctrl Pts',(-19.371101702899,1.51888849071464,-336.912902078713)) ;
#47597=CARTESIAN_POINT('Ctrl Pts',(-19.3292199688169,1.98188273930557,-336.918322554117)) ;
#47598=CARTESIAN_POINT('Ctrl Pts',(-19.2559858084066,2.55958247990601,-336.92512500964)) ;
#47599=CARTESIAN_POINT('Ctrl Pts',(-19.240138773627,2.67610012650855,-336.926499271397)) ;
#47600=CARTESIAN_POINT('Ctrl Pts',(-19.1732660256986,3.13644959152543,-336.931946149509)) ;
#47601=CARTESIAN_POINT('Ctrl Pts',(-19.1140734604698,3.47902873041371,-336.9360368036)) ;
#47602=CARTESIAN_POINT('Ctrl Pts',(-19.0229289232856,3.93347609997459,-336.941598865425)) ;
#47603=CARTESIAN_POINT('Ctrl Pts',(-18.9991200440024,4.04691197644356,-336.942998710324)) ;
#47604=CARTESIAN_POINT('Ctrl Pts',(-18.9608952318669,4.22125492561033,-336.945172078281)) ;
#47605=CARTESIAN_POINT('Ctrl Pts',(-18.9471977708225,4.28231686861727,-336.945937437026)) ;
#47606=CARTESIAN_POINT('Ctrl Pts',(-18.9175017472154,4.41176669421849,-336.947569760949)) ;
#47607=CARTESIAN_POINT('Ctrl Pts',(-18.9014268759759,4.48013613065623,-336.948437722995)) ;
#47608=CARTESIAN_POINT('Ctrl Pts',(-18.8568240761534,4.66532651464416,-336.950803163031)) ;
#47609=CARTESIAN_POINT('Ctrl Pts',(-18.8275815835364,4.78197212226039,-336.952308667788)) ;
#47610=CARTESIAN_POINT('Ctrl Pts',(-18.6928706717891,5.29892205193121,-336.959038826722)) ;
#47611=CARTESIAN_POINT('Ctrl Pts',(-18.5757051307394,5.69606590667437,-336.964362233717)) ;
#47612=CARTESIAN_POINT('Ctrl Pts',(-18.2190052609059,6.77661939431064,-336.979035108164)) ;
#47613=CARTESIAN_POINT('Ctrl Pts',(-17.953814835661,7.4508565854904,-336.988385055213)) ;
#47614=CARTESIAN_POINT('Ctrl Pts',(-17.5764752896891,8.27227528831179,-336.999742246111)) ;
#47615=CARTESIAN_POINT('Ctrl Pts',(-17.4990702768557,8.43478284480902,-337.001988909423)) ;
#47616=CARTESIAN_POINT('Ctrl Pts',(-17.3638367771565,8.70882151620314,-337.005776342066)) ;
#47617=CARTESIAN_POINT('Ctrl Pts',(-17.3071645599781,8.82091008723147,-337.007325189855)) ;
#47618=CARTESIAN_POINT('Ctrl Pts',(-17.1878709717617,9.05127756119131,-337.010508195806)) ;
#47619=CARTESIAN_POINT('Ctrl Pts',(-17.1251062666605,9.16947487288916,-337.012141207953)) ;
#47620=CARTESIAN_POINT('Ctrl Pts',(-16.9558324021988,9.48044700104593,-337.016438833474)) ;
#47621=CARTESIAN_POINT('Ctrl Pts',(-16.8472575684354,9.67207529140804,-337.019088264878)) ;
#47622=CARTESIAN_POINT('Ctrl Pts',(-16.6595544060381,9.99060652608387,-337.023502313373)) ;
#47623=CARTESIAN_POINT('Ctrl Pts',(-16.5821769365317,10.118516683347,-337.025277677188)) ;
#47624=CARTESIAN_POINT('Ctrl Pts',(-16.2419306873566,10.6665802097644,-337.032906647488)) ;
#47625=CARTESIAN_POINT('Ctrl Pts',(-15.9645121626727,11.0774815469406,-337.038677730783)) ;
#47626=CARTESIAN_POINT('Ctrl Pts',(-15.6020939760801,11.5723446442803,-337.045847318519)) ;
#47627=CARTESIAN_POINT('Ctrl Pts',(-15.5316408375656,11.6667317567326,-337.047225373313)) ;
#47628=CARTESIAN_POINT('Ctrl Pts',(-15.2576708533874,12.0268930907225,-337.052533094905)) ;
#47629=CARTESIAN_POINT('Ctrl Pts',(-15.0481555965974,12.2880303329275,-337.056485097318)) ;
#47630=CARTESIAN_POINT('Ctrl Pts',(-14.7680945245478,12.6191839013059,-337.061709953994)) ;
#47631=CARTESIAN_POINT('Ctrl Pts',(-14.7036145813474,12.6942560406728,-337.062909198853)) ;
#47632=CARTESIAN_POINT('Ctrl Pts',(-14.5948240913371,12.8189766513426,-337.06492929665)) ;
#47633=CARTESIAN_POINT('Ctrl Pts',(-14.5508269920663,12.8688960870743,-337.065745449478)) ;
#47634=CARTESIAN_POINT('Ctrl Pts',(-14.4540721229268,12.9775443097679,-337.067539251871)) ;
#47635=CARTESIAN_POINT('Ctrl Pts',(-14.4012111900408,13.0361794052395,-337.068518417823)) ;
#47636=CARTESIAN_POINT('Ctrl Pts',(-14.2354383726852,13.2178212515843,-337.071584096622)) ;
#47637=CARTESIAN_POINT('Ctrl Pts',(-14.1212970547502,13.3396954103467,-337.073687756638)) ;
#47638=CARTESIAN_POINT('Ctrl Pts',(-13.9132447483226,13.5561797537833,-337.077497611279)) ;
#47639=CARTESIAN_POINT('Ctrl Pts',(-13.8199040787608,13.6513237506652,-337.079198274931)) ;
#47640=CARTESIAN_POINT('Ctrl Pts',(-13.3099664473865,14.160522833174,-337.088427065569)) ;
#47641=CARTESIAN_POINT('Ctrl Pts',(-12.8757312236508,14.5564817439944,-337.096054398083)) ;
#47642=CARTESIAN_POINT('Ctrl Pts',(-12.3479303372895,14.9956357558583,-337.10485421796)) ;
#47643=CARTESIAN_POINT('Ctrl Pts',(-12.2711515105281,15.0585296745026,-337.10612355679)) ;
#47644=CARTESIAN_POINT('Ctrl Pts',(-11.945087914446,15.3214771646536,-337.111466894374)) ;
#47645=CARTESIAN_POINT('Ctrl Pts',(-11.6913670941144,15.5159506307828,-337.115508352529)) ;
#47646=CARTESIAN_POINT('Ctrl Pts',(-11.3116032948264,15.7924282601706,-337.121376512292)) ;
#47647=CARTESIAN_POINT('Ctrl Pts',(-11.1892233030353,15.8793715684466,-337.123241042065)) ;
#47648=CARTESIAN_POINT('Ctrl Pts',(-10.9639990229506,16.0354827570472,-337.126624455108)) ;
#47649=CARTESIAN_POINT('Ctrl Pts',(-10.8614770186616,16.1051016403574,-337.128146816652)) ;
#47650=CARTESIAN_POINT('Ctrl Pts',(-10.6324475662309,16.2574453400723,-337.131509175431)) ;
#47651=CARTESIAN_POINT('Ctrl Pts',(-10.5056265021067,16.3396842721349,-337.133345350818)) ;
#47652=CARTESIAN_POINT('Ctrl Pts',(-10.101409512572,16.5951529466455,-337.139120625776)) ;
#47653=CARTESIAN_POINT('Ctrl Pts',(-9.8205920893311,16.7628621397094,-337.143018620762)) ;
#47654=CARTESIAN_POINT('Ctrl Pts',(-9.06285985566667,17.1898145876359,-337.153292347504)) ;
#47655=CARTESIAN_POINT('Ctrl Pts',(-8.57908789853119,17.4362956180977,-337.159597424921)) ;
#47656=CARTESIAN_POINT('Ctrl Pts',(-7.76701170969713,17.808058549328,-337.170054129785)) ;
#47657=CARTESIAN_POINT('Ctrl Pts',(-7.44450265829797,17.945272340401,-337.174177318783)) ;
#47658=CARTESIAN_POINT('Ctrl Pts',(-7.01043634613248,18.1162326784918,-337.179775428474)) ;
#47659=CARTESIAN_POINT('Ctrl Pts',(-6.90203370641882,18.1578091982948,-337.181177576077)) ;
#47660=CARTESIAN_POINT('Ctrl Pts',(-6.73460577951777,18.2203081853747,-337.18335367559)) ;
#47661=CARTESIAN_POINT('Ctrl Pts',(-6.67584107059158,18.2419212629816,-337.18411943076)) ;
#47662=CARTESIAN_POINT('Ctrl Pts',(-6.55098358702901,18.2871584796726,-337.185751567099)) ;
#47663=CARTESIAN_POINT('Ctrl Pts',(-6.48486521753937,18.3107092791357,-337.186618936748)) ;
#47664=CARTESIAN_POINT('Ctrl Pts',(-6.30533538774961,18.3735619081618,-337.188980944462)) ;
#47665=CARTESIAN_POINT('Ctrl Pts',(-6.19168498276405,18.412171750099,-337.190483572315)) ;
#47666=CARTESIAN_POINT('Ctrl Pts',(-5.68643268984749,18.5786112907339,-337.19718507131)) ;
#47667=CARTESIAN_POINT('Ctrl Pts',(-5.29118084729902,18.6950185484329,-337.202481808619)) ;
#47668=CARTESIAN_POINT('Ctrl Pts',(-4.1888230164595,18.9819158715144,-337.217169350238)) ;
#47669=CARTESIAN_POINT('Ctrl Pts',(-3.47538560463534,19.1254038215622,-337.22656164516)) ;
#47670=CARTESIAN_POINT('Ctrl Pts',(-2.57772929742838,19.2540442355816,-337.237954489448)) ;
#47671=CARTESIAN_POINT('Ctrl Pts',(-2.39952706875236,19.2770635144706,-337.240197090344)) ;
#47672=CARTESIAN_POINT('Ctrl Pts',(-2.0963074048896,19.3119621556334,-337.2439798348)) ;
#47673=CARTESIAN_POINT('Ctrl Pts',(-1.97144749576689,19.3251075509596,-337.245528008096)) ;
#47674=CARTESIAN_POINT('Ctrl Pts',(-1.71316020523088,19.3497710669643,-337.248711408511)) ;
#47675=CARTESIAN_POINT('Ctrl Pts',(-1.57972340281974,19.3611216684549,-337.250345471092)) ;
#47676=CARTESIAN_POINT('Ctrl Pts',(-1.22604286094508,19.3875262547419,-337.254650306721)) ;
#47677=CARTESIAN_POINT('Ctrl Pts',(-1.00564154611199,19.4002072330722,-337.257305798409)) ;
#47678=CARTESIAN_POINT('Ctrl Pts',(-0.635190896935972,19.415191437799,-337.261731862867)) ;
#47679=CARTESIAN_POINT('Ctrl Pts',(-0.485244701709166,19.419517596499,-337.263513201341)) ;
#47680=CARTESIAN_POINT('Ctrl Pts',(0.16336220447468,19.4307138145487,-337.271184261728)) ;
#47681=CARTESIAN_POINT('Ctrl Pts',(0.662134599086393,19.4201159752898,-337.276990505297)) ;
#47682=CARTESIAN_POINT('Ctrl Pts',(1.20783267635062,19.3874719004165,-337.283380895291)) ;
#47683=CARTESIAN_POINT('Ctrl Pts',(1.25570985958266,19.3844298139345,-337.283941931733)) ;
#47684=CARTESIAN_POINT('Ctrl Pts',(1.395782743042,19.3750085474562,-337.285584852241)) ;
#47685=CARTESIAN_POINT('Ctrl Pts',(1.48794475547531,19.368148751909,-337.286667738227)) ;
#47686=CARTESIAN_POINT('Ctrl Pts',(1.88838266320089,19.3354683289965,-337.291385896569)) ;
#47687=CARTESIAN_POINT('Ctrl Pts',(2.19606541730352,19.3029433116019,-337.29504426411)) ;
#47688=CARTESIAN_POINT('Ctrl Pts',(2.60014212586808,19.2504419077123,-337.299954209917)) ;
#47689=CARTESIAN_POINT('Ctrl Pts',(2.69734790130677,19.2370623271617,-337.301143502725)) ;
#47690=CARTESIAN_POINT('Ctrl Pts',(2.86019102082799,19.213389753102,-337.303152330722)) ;
#47691=CARTESIAN_POINT('Ctrl Pts',(2.92588448927209,19.2034954746021,-337.303967295423)) ;
#47692=CARTESIAN_POINT('Ctrl Pts',(3.069978889725,19.1810364420111,-337.305765633271)) ;
#47693=CARTESIAN_POINT('Ctrl Pts',(3.14835597542005,19.168327626682,-337.306750599416)) ;
#47694=CARTESIAN_POINT('Ctrl Pts',(3.39396437152533,19.1269552801246,-337.309856105849)) ;
#47695=CARTESIAN_POINT('Ctrl Pts',(3.56089924296837,19.0965810779338,-337.311994403014)) ;
#47696=CARTESIAN_POINT('Ctrl Pts',(4.24480424374507,18.9628633802921,-337.320839658585)) ;
#47697=CARTESIAN_POINT('Ctrl Pts',(4.75786115287742,18.8406822483589,-337.32766953999)) ;
#47698=CARTESIAN_POINT('Ctrl Pts',(5.79705977888661,18.5480430759569,-337.341585146711)) ;
#47699=CARTESIAN_POINT('Ctrl Pts',(6.32218009726688,18.3756862808139,-337.348659829125)) ;
#47700=CARTESIAN_POINT('Ctrl Pts',(6.98316398906478,18.1270430833586,-337.357518497918)) ;
#47701=CARTESIAN_POINT('Ctrl Pts',(7.12644009423608,18.071195918201,-337.359436493387)) ;
#47702=CARTESIAN_POINT('Ctrl Pts',(7.3859998816988,17.96645592234,-337.362906624052)) ;
#47703=CARTESIAN_POINT('Ctrl Pts',(7.50249928539296,17.9181203585504,-337.364462471747)) ;
#47704=CARTESIAN_POINT('Ctrl Pts',(7.74074988192156,17.8165392927236,-337.367641257893)) ;
#47705=CARTESIAN_POINT('Ctrl Pts',(7.8624421385309,17.7631721485228,-337.369263243321)) ;
#47706=CARTESIAN_POINT('Ctrl Pts',(8.1795219363518,17.6202225803425,-337.373486617498)) ;
#47707=CARTESIAN_POINT('Ctrl Pts',(8.3739870365675,17.5286384015881,-337.376073825126)) ;
#47708=CARTESIAN_POINT('Ctrl Pts',(8.69636839493244,17.3702220413318,-337.380365228753)) ;
#47709=CARTESIAN_POINT('Ctrl Pts',(8.82513170059193,17.3051578307364,-337.382079966096)) ;
#47710=CARTESIAN_POINT('Ctrl Pts',(9.36618704376962,17.024152655507,-337.389296405992)) ;
#47711=CARTESIAN_POINT('Ctrl Pts',(9.77137318787817,16.7948652796383,-337.394724590126)) ;
#47712=CARTESIAN_POINT('Ctrl Pts',(10.2506937447463,16.5004041543493,-337.401296060926)) ;
#47713=CARTESIAN_POINT('Ctrl Pts',(10.3330728971278,16.4489411210363,-337.402431181123)) ;
#47714=CARTESIAN_POINT('Ctrl Pts',(10.4970816763267,16.3447649892405,-337.40470492403)) ;
#47715=CARTESIAN_POINT('Ctrl Pts',(10.5787087060405,16.2920529208536,-337.405843515871)) ;
#47716=CARTESIAN_POINT('Ctrl Pts',(10.9158725803599,16.0707212380225,-337.410580805371)) ;
#47717=CARTESIAN_POINT('Ctrl Pts',(11.1678002286557,15.8966849562444,-337.414202277922)) ;
#47718=CARTESIAN_POINT('Ctrl Pts',(11.4946003574772,15.6593212896827,-337.41906970904)) ;
#47719=CARTESIAN_POINT('Ctrl Pts',(11.5732574072799,15.6012785879781,-337.420254641382)) ;
#47720=CARTESIAN_POINT('Ctrl Pts',(11.7045901431073,15.5028256000307,-337.422258507024)) ;
#47721=CARTESIAN_POINT('Ctrl Pts',(11.7575028574325,15.4627345113222,-337.423072925929)) ;
#47722=CARTESIAN_POINT('Ctrl Pts',(11.8733950277655,15.3739861211554,-337.42487304485)) ;
#47723=CARTESIAN_POINT('Ctrl Pts',(11.9362829281707,15.325211534463,-337.425860370187)) ;
#47724=CARTESIAN_POINT('Ctrl Pts',(12.1332173947047,15.1705255638806,-337.428982981354)) ;
#47725=CARTESIAN_POINT('Ctrl Pts',(12.2661674205437,15.0632316214504,-337.431136296907)) ;
#47726=CARTESIAN_POINT('Ctrl Pts',(12.8050036585797,14.6165128023483,-337.440021943715)) ;
#47727=CARTESIAN_POINT('Ctrl Pts',(13.198355784914,14.2623269309345,-337.446877316693)) ;
#47728=CARTESIAN_POINT('Ctrl Pts',(13.9648139426531,13.5132899410866,-337.460690061848)) ;
#47729=CARTESIAN_POINT('Ctrl Pts',(14.3368116993991,13.1179597125527,-337.467638608945)) ;
#47730=CARTESIAN_POINT('Ctrl Pts',(14.7939145599327,12.5894835434343,-337.476407665366)) ;
#47731=CARTESIAN_POINT('Ctrl Pts',(14.8946301218606,12.4701642940459,-337.47835597195)) ;
#47732=CARTESIAN_POINT('Ctrl Pts',(15.074408188939,12.2518929203845,-337.481862923775)) ;
#47733=CARTESIAN_POINT('Ctrl Pts',(15.1539623131608,12.1533570934209,-337.48342557294)) ;
#47734=CARTESIAN_POINT('Ctrl Pts',(15.3144572905008,11.9505416693763,-337.486600761112)) ;
#47735=CARTESIAN_POINT('Ctrl Pts',(15.3953102058076,11.8462007418484,-337.488212528314)) ;
#47736=CARTESIAN_POINT('Ctrl Pts',(15.6021035715943,11.5736400806449,-337.492368320408)) ;
#47737=CARTESIAN_POINT('Ctrl Pts',(15.726389120725,11.4041863366053,-337.494899045294)) ;
#47738=CARTESIAN_POINT('Ctrl Pts',(15.9286325223914,11.1188480541375,-337.499080127157)) ;
#47739=CARTESIAN_POINT('Ctrl Pts',(16.0081337859861,11.0040796445726,-337.500740824433)) ;
#47740=CARTESIAN_POINT('Ctrl Pts',(16.3331325634966,10.5239331943914,-337.507609150096)) ;
#47741=CARTESIAN_POINT('Ctrl Pts',(16.5674121801883,10.1511202984857,-337.512750377675)) ;
#47742=CARTESIAN_POINT('Ctrl Pts',(16.853072742282,9.66027327562971,-337.519383277446)) ;
#47743=CARTESIAN_POINT('Ctrl Pts',(16.9162310729595,9.54924431010841,-337.520875193007)) ;
#47744=CARTESIAN_POINT('Ctrl Pts',(17.0230269867075,9.35711793672063,-337.523446932676)) ;
#47745=CARTESIAN_POINT('Ctrl Pts',(17.0671914236388,9.27631827682224,-337.524525523965)) ;
#47746=CARTESIAN_POINT('Ctrl Pts',(17.2610199150946,8.91563511160627,-337.529331919052)) ;
#47747=CARTESIAN_POINT('Ctrl Pts',(17.4043854383439,8.63242287166826,-337.533082992207)) ;
#47748=CARTESIAN_POINT('Ctrl Pts',(17.5831957620059,8.25661027154145,-337.53809699867)) ;
#47749=CARTESIAN_POINT('Ctrl Pts',(17.6249631048044,8.16707180681088,-337.539294333569)) ;
#47750=CARTESIAN_POINT('Ctrl Pts',(17.6937042573408,8.01672496429396,-337.541312228957)) ;
#47751=CARTESIAN_POINT('Ctrl Pts',(17.7210520972795,7.95608962197797,-337.542128113579)) ;
#47752=CARTESIAN_POINT('Ctrl Pts',(17.7802073843699,7.82311288135791,-337.543922645513)) ;
#47753=CARTESIAN_POINT('Ctrl Pts',(17.8118858492631,7.75071559647389,-337.544902823159)) ;
#47754=CARTESIAN_POINT('Ctrl Pts',(17.9093048273225,7.52432462206485,-337.547975404492)) ;
#47755=CARTESIAN_POINT('Ctrl Pts',(17.9734965838463,7.36967304658117,-337.550085060593)) ;
#47756=CARTESIAN_POINT('Ctrl Pts',(18.085387465715,7.08994347194395,-337.553908160173)) ;
#47757=CARTESIAN_POINT('Ctrl Pts',(18.133808447491,6.9651654221299,-337.555616078197)) ;
#47758=CARTESIAN_POINT('Ctrl Pts',(18.389625055928,6.28518656532974,-337.564920679992)) ;
#47759=CARTESIAN_POINT('Ctrl Pts',(18.57281810745,5.72121569961133,-337.572617637987)) ;
#47760=CARTESIAN_POINT('Ctrl Pts',(18.8307872349467,4.7829675983396,-337.585085442069)) ;
#47761=CARTESIAN_POINT('Ctrl Pts',(18.9208384729872,4.41329803828753,-337.589916870298)) ;
#47762=CARTESIAN_POINT('Ctrl Pts',(19.0331797067387,3.88512102122246,-337.596678763912)) ;
#47763=CARTESIAN_POINT('Ctrl Pts',(19.0644569198124,3.72861603666048,-337.59866529174)) ;
#47764=CARTESIAN_POINT('Ctrl Pts',(19.1167065649677,3.44930022317928,-337.602180030141)) ;
#47765=CARTESIAN_POINT('Ctrl Pts',(19.1384328238181,3.32663959816111,-337.603713073483)) ;
#47766=CARTESIAN_POINT('Ctrl Pts',(19.1823460880826,3.0640330293644,-337.606973445629)) ;
#47767=CARTESIAN_POINT('Ctrl Pts',(19.2041847784371,2.92403606526248,-337.608698414885)) ;
#47768=CARTESIAN_POINT('Ctrl Pts',(19.2624764725422,2.52148451402979,-337.613623062732)) ;
#47769=CARTESIAN_POINT('Ctrl Pts',(19.2950896924794,2.25840610683482,-337.616798053456)) ;
#47770=CARTESIAN_POINT('Ctrl Pts',(19.3856405529217,1.38127449765102,-337.627271882569)) ;
#47771=CARTESIAN_POINT('Ctrl Pts',(19.4197204569346,0.765137940033008,-337.634436772549)) ;
#47772=CARTESIAN_POINT('Ctrl Pts',(19.4250288628456,0.0704377258478807,
-337.642566019914)) ;
#47773=CARTESIAN_POINT('Ctrl Pts',(19.4251551013299,-0.00755514414413087,
-337.643479601952)) ;
#47774=CARTESIAN_POINT('Ctrl Pts',(19.423378799504,-0.410894534108805,-337.648212343182)) ;
#47775=CARTESIAN_POINT('Ctrl Pts',(19.4137722757462,-0.736154497479361,
-337.652055527468)) ;
#47776=CARTESIAN_POINT('Ctrl Pts',(19.3905843014776,-1.16004341642344,-337.657169549116)) ;
#47777=CARTESIAN_POINT('Ctrl Pts',(19.3844090824792,-1.2590253236515,-337.658371313284)) ;
#47778=CARTESIAN_POINT('Ctrl Pts',(19.3728216180188,-1.42437376003337,-337.660394431619)) ;
#47779=CARTESIAN_POINT('Ctrl Pts',(19.3678256397745,-1.49076760344238,-337.66121105553)) ;
#47780=CARTESIAN_POINT('Ctrl Pts',(19.3561650874913,-1.63576297692322,-337.663004535752)) ;
#47781=CARTESIAN_POINT('Ctrl Pts',(19.3493628925497,-1.71435207654343,-337.663982894112)) ;
#47782=CARTESIAN_POINT('Ctrl Pts',(19.3267137023345,-1.9586953823791,-337.667041913255)) ;
#47783=CARTESIAN_POINT('Ctrl Pts',(19.3092140658688,-2.12428861987821,-337.669139607738)) ;
#47784=CARTESIAN_POINT('Ctrl Pts',(19.2739436468233,-2.42143271303208,-337.672936202221)) ;
#47785=CARTESIAN_POINT('Ctrl Pts',(19.2569493122032,-2.55306545557215,-337.674629568155)) ;
#47786=CARTESIAN_POINT('Ctrl Pts',(19.158147945621,-3.26112695382692,-337.683784288383)) ;
#47787=CARTESIAN_POINT('Ctrl Pts',(19.0518061448702,-3.83383173886034,-337.691343720935)) ;
#47788=CARTESIAN_POINT('Ctrl Pts',(18.8710604105343,-4.61087650934077,-337.701570707971)) ;
#47789=CARTESIAN_POINT('Ctrl Pts',(18.8187247777371,-4.82003123637859,-337.704321703155)) ;
#47790=CARTESIAN_POINT('Ctrl Pts',(18.699415622909,-5.26523152325532,-337.710163781735)) ;
#47791=CARTESIAN_POINT('Ctrl Pts',(18.6314294828479,-5.5009674961467,-337.713248835298)) ;
#47792=CARTESIAN_POINT('Ctrl Pts',(18.5177961075829,-5.86867311400223,-337.71804331602)) ;
#47793=CARTESIAN_POINT('Ctrl Pts',(18.4751602237666,-6.00154576531985,-337.71977224667)) ;
#47794=CARTESIAN_POINT('Ctrl Pts',(18.3916264722974,-6.2525454030299,-337.723031577909)) ;
#47795=CARTESIAN_POINT('Ctrl Pts',(18.3510127988556,-6.37075957928543,-337.724563813404)) ;
#47796=CARTESIAN_POINT('Ctrl Pts',(18.2536965123682,-6.645363736268,-337.728117337735)) ;
#47797=CARTESIAN_POINT('Ctrl Pts',(18.1961203046822,-6.80143378384901,-337.7301325414)) ;
#47798=CARTESIAN_POINT('Ctrl Pts',(17.9656966456587,-7.40215859360995,-337.737878292566)) ;
#47799=CARTESIAN_POINT('Ctrl Pts',(17.7784962285236,-7.84112753817686,-337.743510764866)) ;
#47800=CARTESIAN_POINT('Ctrl Pts',(17.3953448438544,-8.65512564404414,-337.754049919798)) ;
#47801=CARTESIAN_POINT('Ctrl Pts',(17.2029338957534,-9.03151632359954,-337.758964239384)) ;
#47802=CARTESIAN_POINT('Ctrl Pts',(16.8465190735595,-9.67594443290407,-337.767610170652)) ;
#47803=CARTESIAN_POINT('Ctrl Pts',(16.688005909082,-9.94683686084418,-337.771320054849)) ;
#47804=CARTESIAN_POINT('Ctrl Pts',(16.4712252339049,-10.2975269018185,-337.776287484352)) ;
#47805=CARTESIAN_POINT('Ctrl Pts',(16.4188140152371,-10.3808895233145,-337.777480888215)) ;
#47806=CARTESIAN_POINT('Ctrl Pts',(16.3299831404541,-10.5198236429627,-337.779493866971)) ;
#47807=CARTESIAN_POINT('Ctrl Pts',(16.2939081144171,-10.5756133256486,-337.780308809749)) ;
#47808=CARTESIAN_POINT('Ctrl Pts',(16.2142944310176,-10.6973607463315,-337.782102523974)) ;
#47809=CARTESIAN_POINT('Ctrl Pts',(16.1706381198371,-10.7632399215596,-337.783082839436)) ;
#47810=CARTESIAN_POINT('Ctrl Pts',(16.0329876166242,-10.9682323107964,-337.786161332381)) ;
#47811=CARTESIAN_POINT('Ctrl Pts',(15.9375912427134,-11.1063944268197,-337.788276904272)) ;
#47812=CARTESIAN_POINT('Ctrl Pts',(15.5341777262881,-11.6747539505318,-337.79712238335)) ;
#47813=CARTESIAN_POINT('Ctrl Pts',(15.2104400300485,-12.0935136001958,-337.803977800465)) ;
#47814=CARTESIAN_POINT('Ctrl Pts',(14.5158755752377,-12.9198651109586,-337.817894000775)) ;
#47815=CARTESIAN_POINT('Ctrl Pts',(14.143990343901,-13.3259558286898,-337.824944474059)) ;
#47816=CARTESIAN_POINT('Ctrl Pts',(13.6455313489594,-13.8258560376481,-337.833803399733)) ;
#47817=CARTESIAN_POINT('Ctrl Pts',(13.5343802059128,-13.9346823968351,-337.835744256679)) ;
#47818=CARTESIAN_POINT('Ctrl Pts',(13.3305276830712,-14.1295309583979,-337.839241357412)) ;
#47819=CARTESIAN_POINT('Ctrl Pts',(13.2382705233153,-14.2160053114218,-337.840801544594)) ;
#47820=CARTESIAN_POINT('Ctrl Pts',(13.0655495863411,-14.3747603711127,-337.843681483417)) ;
#47821=CARTESIAN_POINT('Ctrl Pts',(12.9853137199658,-14.4472817285672,-337.845003317439)) ;
#47822=CARTESIAN_POINT('Ctrl Pts',(12.7792615853497,-14.6304190811857,-337.848358120345)) ;
#47823=CARTESIAN_POINT('Ctrl Pts',(12.652612293352,-14.7400845119042,-337.850382936227)) ;
#47824=CARTESIAN_POINT('Ctrl Pts',(12.3654495801427,-14.9823099252617,-337.854895579216)) ;
#47825=CARTESIAN_POINT('Ctrl Pts',(12.2041917960066,-15.1139556963398,-337.857376236079)) ;
#47826=CARTESIAN_POINT('Ctrl Pts',(11.6914709470792,-15.5189678843399,-337.865115078004)) ;
#47827=CARTESIAN_POINT('Ctrl Pts',(11.3327070999895,-15.7828580212535,-337.870313771805)) ;
#47828=CARTESIAN_POINT('Ctrl Pts',(10.5614813047907,-16.3102711070265,-337.881226384946)) ;
#47829=CARTESIAN_POINT('Ctrl Pts',(10.1474871481526,-16.5710088104313,-337.886936250085)) ;
#47830=CARTESIAN_POINT('Ctrl Pts',(9.62105156827939,-16.8754306810581,-337.894229141809)) ;
#47831=CARTESIAN_POINT('Ctrl Pts',(9.51746124238996,-16.9340699593464,-337.895665975063)) ;
#47832=CARTESIAN_POINT('Ctrl Pts',(9.35810298882791,-17.0223535623432,-337.89788351065)) ;
#47833=CARTESIAN_POINT('Ctrl Pts',(9.30271850351345,-17.0526842691746,-337.898655525394)) ;
#47834=CARTESIAN_POINT('Ctrl Pts',(9.18879212812195,-17.1143546011128,-337.900247202577)) ;
#47835=CARTESIAN_POINT('Ctrl Pts',(9.13023547909524,-17.1456651740403,-337.901067298396)) ;
#47836=CARTESIAN_POINT('Ctrl Pts',(9.06606251051121,-17.17955685227,-337.901967734198)) ;
#47837=CARTESIAN_POINT('Ctrl Pts',(9.06060413306961,-17.1824362599913,-337.902044336065)) ;
#47838=CARTESIAN_POINT('Ctrl Pts',(9.04958456724378,-17.188242599348,-337.902199008658)) ;
#47839=CARTESIAN_POINT('Ctrl Pts',(9.04402332873731,-17.1911694344214,-337.902277080563)) ;
#47840=CARTESIAN_POINT('Ctrl Pts',(9.03267677446241,-17.1971340049961,-337.902436396597)) ;
#47841=CARTESIAN_POINT('Ctrl Pts',(9.02689134429441,-17.2001715211215,-337.902517643385)) ;
#47842=CARTESIAN_POINT('Ctrl Pts',(9.01497191707914,-17.2064218907538,-337.902685060046)) ;
#47843=CARTESIAN_POINT('Ctrl Pts',(9.00883773257188,-17.2096343847425,-337.902771234227)) ;
#47844=CARTESIAN_POINT('Ctrl Pts',(8.99608488712258,-17.2163044078818,-337.902950419322)) ;
#47845=CARTESIAN_POINT('Ctrl Pts',(8.98946594761668,-17.2197614018833,-337.903043436559)) ;
#47846=CARTESIAN_POINT('Ctrl Pts',(8.97558855136614,-17.2269992203051,-337.903238492989)) ;
#47847=CARTESIAN_POINT('Ctrl Pts',(8.96832969536919,-17.2307792759047,-337.903340541123)) ;
#47848=CARTESIAN_POINT('Ctrl Pts',(8.9589461933142,-17.2356582069534,-337.903472483073)) ;
#47849=CARTESIAN_POINT('Ctrl Pts',(8.95682372965082,-17.2367612792422,-337.903502328782)) ;
#47850=CARTESIAN_POINT('Ctrl Pts',(8.95196222830745,-17.2392867250484,-337.903570694032)) ;
#47851=CARTESIAN_POINT('Ctrl Pts',(8.9492230553523,-17.2407088378356,-337.903609216545)) ;
#47852=CARTESIAN_POINT('Ctrl Pts',(8.94289952007592,-17.2439899523679,-337.90369815401)) ;
#47853=CARTESIAN_POINT('Ctrl Pts',(8.93931491686858,-17.2458484894362,-337.903748574223)) ;
#47854=CARTESIAN_POINT('Ctrl Pts',(8.93096187477265,-17.2501760520133,-337.90386607647)) ;
#47855=CARTESIAN_POINT('Ctrl Pts',(8.92619299117249,-17.2526442181607,-337.903933168145)) ;
#47856=CARTESIAN_POINT('Ctrl Pts',(8.91495806009663,-17.2584530232681,-337.904091246069)) ;
#47857=CARTESIAN_POINT('Ctrl Pts',(8.90849115757613,-17.2617920061912,-337.904182250673)) ;
#47858=CARTESIAN_POINT('Ctrl Pts',(8.80826529037772,-17.3134691757035,-337.905592871701)) ;
#47859=CARTESIAN_POINT('Ctrl Pts',(8.7141160559612,-17.3610464444985,-337.906920752603)) ;
#47860=CARTESIAN_POINT('Ctrl Pts',(8.43574439803903,-17.4988835292732,-337.910850172303)) ;
#47861=CARTESIAN_POINT('Ctrl Pts',(8.25047444042984,-17.5869946166852,-337.913469461293)) ;
#47862=CARTESIAN_POINT('Ctrl Pts',(7.33160715050241,-18.0062758340354,-337.926426155621)) ;
#47863=CARTESIAN_POINT('Ctrl Pts',(6.57930689612149,-18.2945665075286,-337.93689276559)) ;
#47864=CARTESIAN_POINT('Ctrl Pts',(5.60189958709704,-18.6010081373859,-337.949832343576)) ;
#47865=CARTESIAN_POINT('Ctrl Pts',(5.39140373704929,-18.6631066197335,-337.952584002111)) ;
#47866=CARTESIAN_POINT('Ctrl Pts',(5.05086177376709,-18.7573277964724,-337.9569769935)) ;
#47867=CARTESIAN_POINT('Ctrl Pts',(4.9214570522249,-18.7916952738028,-337.958632868949)) ;
#47868=CARTESIAN_POINT('Ctrl Pts',(4.67692817944004,-18.8539384648727,-337.961736862916)) ;
#47869=CARTESIAN_POINT('Ctrl Pts',(4.56188419248772,-18.882104371263,-337.963186848473)) ;
#47870=CARTESIAN_POINT('Ctrl Pts',(4.32476558709997,-18.9378639085973,-337.966154868259)) ;
#47871=CARTESIAN_POINT('Ctrl Pts',(4.20266735727822,-18.9653334780393,-337.967672033542)) ;
#47872=CARTESIAN_POINT('Ctrl Pts',(3.90121292933478,-19.0301003635033,-337.971392103434)) ;
#47873=CARTESIAN_POINT('Ctrl Pts',(3.72157823831249,-19.0660441021907,-337.973586477635)) ;
#47874=CARTESIAN_POINT('Ctrl Pts',(2.87644088366972,-19.2227513923221,-337.983820717492)) ;
#47875=CARTESIAN_POINT('Ctrl Pts',(2.20543290841547,-19.3112440804199,-337.991668592314)) ;
#47876=CARTESIAN_POINT('Ctrl Pts',(1.53118156877294,-19.3645580379065,-337.999588035935)) ;
#47877=CARTESIAN_POINT('',(16.0043568677506,-11.0086868540114,-338.)) ;
#47878=CARTESIAN_POINT('Origin',(0.,0.,-338.)) ;
#47879=CARTESIAN_POINT('Ctrl Pts',(16.0043568677512,-11.0086868540105,-338.)) ;
#47880=CARTESIAN_POINT('Ctrl Pts',(16.2343017349983,-10.6743945115965,-337.995013456726)) ;
#47881=CARTESIAN_POINT('Ctrl Pts',(16.4537823394767,-10.3328760929934,-337.990026913451)) ;
#47882=CARTESIAN_POINT('Ctrl Pts',(16.6623602288354,-9.98480728930328,-337.985040370177)) ;
#47883=CARTESIAN_POINT('Ctrl Pts',(16.8709240018669,-9.63676204253544,-337.980054164386)) ;
#47884=CARTESIAN_POINT('Ctrl Pts',(17.0685864148693,-9.2821674950807,-337.975067958596)) ;
#47885=CARTESIAN_POINT('Ctrl Pts',(17.2549536395104,-8.92172628465741,-337.970081752805)) ;
#47886=CARTESIAN_POINT('Ctrl Pts',(17.4413144679775,-8.56129744467485,-337.965095718143)) ;
#47887=CARTESIAN_POINT('Ctrl Pts',(17.6163807764168,-8.19502254852781,-337.96010968348)) ;
#47888=CARTESIAN_POINT('Ctrl Pts',(17.7798050182231,-7.82362821930908,-337.955123648818)) ;
#47889=CARTESIAN_POINT('Ctrl Pts',(17.9432291025103,-7.45223424806482,-337.950137618961)) ;
#47890=CARTESIAN_POINT('Ctrl Pts',(18.0950110498037,-7.075721065873,-337.945151589104)) ;
#47891=CARTESIAN_POINT('Ctrl Pts',(18.2348510554591,-6.69483621795347,-337.940165559248)) ;
#47892=CARTESIAN_POINT('Ctrl Pts',(18.3747130970232,-6.3138913504159,-337.935178743695)) ;
#47893=CARTESIAN_POINT('Ctrl Pts',(18.5026293537671,-5.92857365703956,-337.930191928143)) ;
#47894=CARTESIAN_POINT('Ctrl Pts',(18.6183489284098,-5.53964874157018,-337.92520511259)) ;
#47895=CARTESIAN_POINT('Ctrl Pts',(18.7340719628011,-5.15071219814223,-337.920218147944)) ;
#47896=CARTESIAN_POINT('Ctrl Pts',(18.8375975227664,-4.7581684399421,-337.915231183297)) ;
#47897=CARTESIAN_POINT('Ctrl Pts',(18.9287248027228,-4.36279753630466,-337.91024421865)) ;
#47898=CARTESIAN_POINT('Ctrl Pts',(19.0198727933892,-3.96733677579774,-337.905256120604)) ;
#47899=CARTESIAN_POINT('Ctrl Pts',(19.0986168186598,-3.56904781118808,-337.900268022559)) ;
#47900=CARTESIAN_POINT('Ctrl Pts',(19.1648069165423,-3.16872227430096,-337.895279924513)) ;
#47901=CARTESIAN_POINT('Ctrl Pts',(19.2283855015679,-2.78419147590161,-337.89048863056)) ;
#47902=CARTESIAN_POINT('Ctrl Pts',(19.2803815197814,-2.39778188479241,-337.885697336607)) ;
#47903=CARTESIAN_POINT('Ctrl Pts',(19.3207068719133,-2.01020172360925,-337.880906042654)) ;
#47904=CARTESIAN_POINT('Ctrl Pts',(19.362471040198,-1.60879262933786,-337.875943794431)) ;
#47905=CARTESIAN_POINT('Ctrl Pts',(19.3917280541838,-1.20601620829655,-337.870981546209)) ;
#47906=CARTESIAN_POINT('Ctrl Pts',(19.4084091842075,-0.802669258394608,
-337.866019297986)) ;
#47907=CARTESIAN_POINT('Ctrl Pts',(19.4250365960367,-0.400621205500163,
-337.861073029677)) ;
#47908=CARTESIAN_POINT('Ctrl Pts',(19.4291689995692,0.00199346573810244,
-337.856126761368)) ;
#47909=CARTESIAN_POINT('Ctrl Pts',(19.4207904046784,0.40438231607356,-337.851180493058)) ;
#47910=CARTESIAN_POINT('Ctrl Pts',(19.412412909012,0.806718375258068,-337.846234873672)) ;
#47911=CARTESIAN_POINT('Ctrl Pts',(19.3915276979543,1.20882843310241,-337.841289254285)) ;
#47912=CARTESIAN_POINT('Ctrl Pts',(19.3581708977425,1.60992064829172,-337.836343634898)) ;
#47913=CARTESIAN_POINT('Ctrl Pts',(19.3248167459013,2.01098101867452,-337.83139840817)) ;
#47914=CARTESIAN_POINT('Ctrl Pts',(19.278993002637,2.41102346896342,-337.826453181442)) ;
#47915=CARTESIAN_POINT('Ctrl Pts',(19.2207877568638,2.80926022390157,-337.821507954714)) ;
#47916=CARTESIAN_POINT('Ctrl Pts',(19.1622361315391,3.20986688668423,-337.81653329893)) ;
#47917=CARTESIAN_POINT('Ctrl Pts',(19.0911551833977,3.60864604900755,-337.811558643146)) ;
#47918=CARTESIAN_POINT('Ctrl Pts',(19.0076872531245,4.00480340184232,-337.806583987363)) ;
#47919=CARTESIAN_POINT('Ctrl Pts',(18.9247063336755,4.39864929303818,-337.801638357232)) ;
#47920=CARTESIAN_POINT('Ctrl Pts',(18.8294826609021,4.78990365494282,-337.796692727102)) ;
#47921=CARTESIAN_POINT('Ctrl Pts',(18.7222072098571,5.17779704036152,-337.791747096972)) ;
#47922=CARTESIAN_POINT('Ctrl Pts',(18.6139873675078,5.56910521580501,-337.786757928361)) ;
#47923=CARTESIAN_POINT('Ctrl Pts',(18.4935026142637,5.95699271935316,-337.781768759751)) ;
#47924=CARTESIAN_POINT('Ctrl Pts',(18.3610006351633,6.34068455890482,-337.77677959114)) ;
#47925=CARTESIAN_POINT('Ctrl Pts',(18.2284986560629,6.72437639845648,-337.77179042253)) ;
#47926=CARTESIAN_POINT('Ctrl Pts',(18.0839795396159,7.10387233988891,-337.766801253919)) ;
#47927=CARTESIAN_POINT('Ctrl Pts',(17.9277416233235,7.47841596110801,-337.761812085309)) ;
#47928=CARTESIAN_POINT('Ctrl Pts',(17.7722615228434,7.85114289732963,-337.756847116143)) ;
#47929=CARTESIAN_POINT('Ctrl Pts',(17.6051348821206,8.21906435576997,-337.751882146978)) ;
#47930=CARTESIAN_POINT('Ctrl Pts',(17.426684576462,8.58145032453731,-337.746917177812)) ;
#47931=CARTESIAN_POINT('Ctrl Pts',(17.248259600405,8.94378485549855,-337.741952913385)) ;
#47932=CARTESIAN_POINT('Ctrl Pts',(17.0585142738589,9.30058525420489,-337.736988648957)) ;
#47933=CARTESIAN_POINT('Ctrl Pts',(16.8578184523581,9.6511440786745,-337.73202438453)) ;
#47934=CARTESIAN_POINT('Ctrl Pts',(16.6571422865929,10.0016685701346,-337.727060606292)) ;
#47935=CARTESIAN_POINT('Ctrl Pts',(16.4455178853756,10.3459525034175,-337.722096828054)) ;
#47936=CARTESIAN_POINT('Ctrl Pts',(16.2233604970649,10.6833140542752,-337.717133049817)) ;
#47937=CARTESIAN_POINT('Ctrl Pts',(16.0012150938113,11.0206574049845,-337.712169539367)) ;
#47938=CARTESIAN_POINT('Ctrl Pts',(15.7685379686291,11.3510789221508,-337.707206028918)) ;
#47939=CARTESIAN_POINT('Ctrl Pts',(15.5257879761034,11.67392533474,-337.702242518468)) ;
#47940=CARTESIAN_POINT('Ctrl Pts',(15.2830131018267,11.9968048389226,-337.697278499262)) ;
#47941=CARTESIAN_POINT('Ctrl Pts',(15.030163436591,12.3121074963065,-337.692314480055)) ;
#47942=CARTESIAN_POINT('Ctrl Pts',(14.7677396345522,12.6192111911195,-337.687350460849)) ;
#47943=CARTESIAN_POINT('Ctrl Pts',(14.5053145445756,12.9263163931527,-337.682386417279)) ;
#47944=CARTESIAN_POINT('Ctrl Pts',(14.2333153789608,13.2252223739513,-337.67742237371)) ;
#47945=CARTESIAN_POINT('Ctrl Pts',(13.9522822298859,13.515341119543,-337.672458330141)) ;
#47946=CARTESIAN_POINT('Ctrl Pts',(13.6711888550596,13.8055220379407,-337.667493222771)) ;
#47947=CARTESIAN_POINT('Ctrl Pts',(13.3810577905449,14.0869117864317,-337.662528115401)) ;
#47948=CARTESIAN_POINT('Ctrl Pts',(13.082466514253,14.358958698438,-337.657563008031)) ;
#47949=CARTESIAN_POINT('Ctrl Pts',(12.7848863979647,14.6300843412099,-337.652614714675)) ;
#47950=CARTESIAN_POINT('Ctrl Pts',(12.4789034688143,14.8919301874873,-337.647666421319)) ;
#47951=CARTESIAN_POINT('Ctrl Pts',(12.1651233976083,15.143988831248,-337.642718127963)) ;
#47952=CARTESIAN_POINT('Ctrl Pts',(11.850458423498,15.3967583150089,-337.637755879741)) ;
#47953=CARTESIAN_POINT('Ctrl Pts',(11.5278693550387,15.6397518520347,-337.632793631518)) ;
#47954=CARTESIAN_POINT('Ctrl Pts',(11.1979882450328,15.8724819818486,-337.627831383295)) ;
#47955=CARTESIAN_POINT('Ctrl Pts',(10.8685001565858,16.1049348361361,-337.622875047113)) ;
#47956=CARTESIAN_POINT('Ctrl Pts',(10.531737588431,16.3271485899504,-337.617918710931)) ;
#47957=CARTESIAN_POINT('Ctrl Pts',(10.188361177574,16.5386795577913,-337.612962374749)) ;
#47958=CARTESIAN_POINT('Ctrl Pts',(9.84502269901286,16.7501871581119,-337.608006586086)) ;
#47959=CARTESIAN_POINT('Ctrl Pts',(9.49507203939322,16.9510142048205,-337.603050797424)) ;
#47960=CARTESIAN_POINT('Ctrl Pts',(9.1391974995517,17.1407611868373,-337.598095008761)) ;
#47961=CARTESIAN_POINT('Ctrl Pts',(8.7833453758918,17.3304962168814,-337.593139532258)) ;
#47962=CARTESIAN_POINT('Ctrl Pts',(8.42157032719244,17.5091524646376,-337.588184055756)) ;
#47963=CARTESIAN_POINT('Ctrl Pts',(8.05458533401213,17.6763763282274,-337.583228579253)) ;
#47964=CARTESIAN_POINT('Ctrl Pts',(7.68674442969674,17.843990204405,-337.5782615452)) ;
#47965=CARTESIAN_POINT('Ctrl Pts',(7.31366946010517,18.0001181892563,-337.573294511147)) ;
#47966=CARTESIAN_POINT('Ctrl Pts',(6.93610020148422,18.1444520169381,-337.568327477094)) ;
#47967=CARTESIAN_POINT('Ctrl Pts',(6.55937125107006,18.2884646190511,-337.563371497542)) ;
#47968=CARTESIAN_POINT('Ctrl Pts',(6.17816822458658,18.4207354381156,-337.558415517989)) ;
#47969=CARTESIAN_POINT('Ctrl Pts',(5.79324431870531,18.5410071264694,-337.553459538437)) ;
#47970=CARTESIAN_POINT('Ctrl Pts',(5.40703253177549,18.6616812206643,-337.548486977134)) ;
#47971=CARTESIAN_POINT('Ctrl Pts',(5.01707514759405,18.7702756607823,-337.543514415831)) ;
#47972=CARTESIAN_POINT('Ctrl Pts',(4.62414806207482,18.8665810283689,-337.538541854528)) ;
#47973=CARTESIAN_POINT('Ctrl Pts',(4.23122097655567,18.9628863959555,-337.533569293225)) ;
#47974=CARTESIAN_POINT('Ctrl Pts',(3.83532442586498,19.0469026401326,-337.528596731922)) ;
#47975=CARTESIAN_POINT('Ctrl Pts',(3.43724593561117,19.1184718368944,-337.523624170618)) ;
#47976=CARTESIAN_POINT('Ctrl Pts',(3.03999305919983,19.1898925993122,-337.518661922396)) ;
#47977=CARTESIAN_POINT('Ctrl Pts',(2.64046091834604,19.2489370421643,-337.513699674173)) ;
#47978=CARTESIAN_POINT('Ctrl Pts',(2.23943738365606,19.2954799164126,-337.50873742595)) ;
#47979=CARTESIAN_POINT('Ctrl Pts',(1.83867898436969,19.3419920189913,-337.503778458502)) ;
#47980=CARTESIAN_POINT('Ctrl Pts',(1.43643139837477,19.3760190500696,-337.498819491053)) ;
#47981=CARTESIAN_POINT('Ctrl Pts',(1.03348786716827,19.3974876679537,-337.493860523605)) ;
#47982=CARTESIAN_POINT('Ctrl Pts',(0.630587385590106,19.4189539921765,-337.488902085962)) ;
#47983=CARTESIAN_POINT('Ctrl Pts',(0.226991344155984,19.4278645704372,-337.483943648319)) ;
#47984=CARTESIAN_POINT('Ctrl Pts',(-0.1765038782194,19.4241980884919,-337.478985210676)) ;
#47985=CARTESIAN_POINT('Ctrl Pts',(-0.579974687761069,19.4205318283813,
-337.474027073035)) ;
#47986=CARTESIAN_POINT('Ctrl Pts',(-0.983344453241035,19.4042900304248,
-337.469068935394)) ;
#47987=CARTESIAN_POINT('Ctrl Pts',(-1.38581710366883,19.3755035019784,-337.464110797754)) ;
#47988=CARTESIAN_POINT('Ctrl Pts',(-1.78885075407456,19.3466768484657,-337.459145749047)) ;
#47989=CARTESIAN_POINT('Ctrl Pts',(-2.190984548107,19.3052704731956,-337.45418070034)) ;
#47990=CARTESIAN_POINT('Ctrl Pts',(-2.59142281899507,19.2513675559216,-337.449215651633)) ;
#47991=CARTESIAN_POINT('Ctrl Pts',(-2.9913446005162,19.1975341631802,-337.444257006897)) ;
#47992=CARTESIAN_POINT('Ctrl Pts',(-3.38957499610439,19.1312364889784,-337.439298362161)) ;
#47993=CARTESIAN_POINT('Ctrl Pts',(-3.78532867959759,19.0526090545997,-337.434339717424)) ;
#47994=CARTESIAN_POINT('Ctrl Pts',(-4.18184902264361,18.973829302059,-337.429371466732)) ;
#47995=CARTESIAN_POINT('Ctrl Pts',(-4.57588281161247,18.8826720066114,-337.42440321604)) ;
#47996=CARTESIAN_POINT('Ctrl Pts',(-4.96665098629062,18.7793238158454,-337.419434965348)) ;
#47997=CARTESIAN_POINT('Ctrl Pts',(-5.35741916096867,18.6759756250794,-337.414466714656)) ;
#47998=CARTESIAN_POINT('Ctrl Pts',(-5.74492149171522,18.5604366065672,-337.409498463964)) ;
#47999=CARTESIAN_POINT('Ctrl Pts',(-6.12839324434191,18.4329439114512,-337.404530213272)) ;
#48000=CARTESIAN_POINT('Ctrl Pts',(-6.51140169961259,18.3056052486156,-337.399567965049)) ;
#48001=CARTESIAN_POINT('Ctrl Pts',(-6.89049071154255,18.1663080725525,-337.394605716827)) ;
#48002=CARTESIAN_POINT('Ctrl Pts',(-7.26490843457078,18.0153193265427,-337.389643468604)) ;
#48003=CARTESIAN_POINT('Ctrl Pts',(-7.63904959350638,17.8644421085482,-337.384684885752)) ;
#48004=CARTESIAN_POINT('Ctrl Pts',(-8.00852614156413,17.7018906748922,-337.379726302899)) ;
#48005=CARTESIAN_POINT('Ctrl Pts',(-8.3726065231162,17.5279800607221,-337.374767720047)) ;
#48006=CARTESIAN_POINT('Ctrl Pts',(-8.73664794995709,17.3540880540851,-337.369809667737)) ;
#48007=CARTESIAN_POINT('Ctrl Pts',(-9.0952941493864,17.1688393966988,-337.364851615428)) ;
#48008=CARTESIAN_POINT('Ctrl Pts',(-9.44783570051987,16.9725963121728,-337.359893563118)) ;
#48009=CARTESIAN_POINT('Ctrl Pts',(-9.80035592538492,16.7763650989643,-337.354935810736)) ;
#48010=CARTESIAN_POINT('Ctrl Pts',(-10.1467720323834,16.569140902698,-337.349978058353)) ;
#48011=CARTESIAN_POINT('Ctrl Pts',(-10.4863998065743,16.3513315695291,-337.345020305971)) ;
#48012=CARTESIAN_POINT('Ctrl Pts',(-10.8265471948195,16.1331889986239,-337.340054968467)) ;
#48013=CARTESIAN_POINT('Ctrl Pts',(-11.1598852547188,15.9044289941104,-337.335089630963)) ;
#48014=CARTESIAN_POINT('Ctrl Pts',(-11.4857549166979,15.6655053858326,-337.330124293459)) ;
#48015=CARTESIAN_POINT('Ctrl Pts',(-11.8111603124545,15.4269221718106,-337.325166030068)) ;
#48016=CARTESIAN_POINT('Ctrl Pts',(-12.129118392427,15.1782044459368,-337.320207766676)) ;
#48017=CARTESIAN_POINT('Ctrl Pts',(-12.4390040007212,14.9198459935095,-337.315249503284)) ;
#48018=CARTESIAN_POINT('Ctrl Pts',(-12.7495527944879,14.6609346287566,-337.310280628725)) ;
#48019=CARTESIAN_POINT('Ctrl Pts',(-13.0519943349544,14.3923413713668,-337.305311754165)) ;
#48020=CARTESIAN_POINT('Ctrl Pts',(-13.3457335522706,14.1146031099638,-337.300342879605)) ;
#48021=CARTESIAN_POINT('Ctrl Pts',(-13.6394727695868,13.8368648485608,-337.295374005045)) ;
#48022=CARTESIAN_POINT('Ctrl Pts',(-13.9245094942263,13.5499817525959,-337.290405130486)) ;
#48023=CARTESIAN_POINT('Ctrl Pts',(-14.2002854317668,13.2545282321307,-337.285436255926)) ;
#48024=CARTESIAN_POINT('Ctrl Pts',(-14.4756936030728,12.9594687193142,-337.280474007703)) ;
#48025=CARTESIAN_POINT('Ctrl Pts',(-14.7419390172365,12.6557830606652,-337.275511759481)) ;
#48026=CARTESIAN_POINT('Ctrl Pts',(-14.9984890994669,12.34406536491,-337.270549511258)) ;
#48027=CARTESIAN_POINT('Ctrl Pts',(-15.2548349838703,12.0325957769535,-337.265591212675)) ;
#48028=CARTESIAN_POINT('Ctrl Pts',(-15.5015008131982,11.7131071164413,-337.260632914091)) ;
#48029=CARTESIAN_POINT('Ctrl Pts',(-15.737994926772,11.3862259192807,-337.255674615508)) ;
#48030=CARTESIAN_POINT('Ctrl Pts',(-15.9744635701517,11.0593799269182,-337.250716850929)) ;
#48031=CARTESIAN_POINT('Ctrl Pts',(-16.2007625467101,10.7251431803851,-337.245759086349)) ;
#48032=CARTESIAN_POINT('Ctrl Pts',(-16.4164422069112,10.3841730661207,-337.24080132177)) ;
#48033=CARTESIAN_POINT('Ctrl Pts',(-16.6321086950101,10.0432237757631,-337.235843859974)) ;
#48034=CARTESIAN_POINT('Ctrl Pts',(-16.8371570355162,9.69554213976692,-337.230886398178)) ;
#48035=CARTESIAN_POINT('Ctrl Pts',(-17.0311815382854,9.34181355037479,-337.225928936382)) ;
#48036=CARTESIAN_POINT('Ctrl Pts',(-17.2255227194305,8.98750762052518,-337.220963383232)) ;
#48037=CARTESIAN_POINT('Ctrl Pts',(-17.4088039209296,8.62713518445671,-337.215997830082)) ;
#48038=CARTESIAN_POINT('Ctrl Pts',(-17.5806634233294,8.26141020623035,-337.211032276932)) ;
#48039=CARTESIAN_POINT('Ctrl Pts',(-17.7522604231468,7.89624384565332,-337.206074308294)) ;
#48040=CARTESIAN_POINT('Ctrl Pts',(-17.9124705016481,7.52574150354035,-337.201116339656)) ;
#48041=CARTESIAN_POINT('Ctrl Pts',(-18.0609809485656,7.15063578820439,-337.196158371019)) ;
#48042=CARTESIAN_POINT('Ctrl Pts',(-18.2098321739573,6.77466933912253,-337.191189025612)) ;
#48043=CARTESIAN_POINT('Ctrl Pts',(-18.3469299105402,6.3940785832791,-337.186219680206)) ;
#48044=CARTESIAN_POINT('Ctrl Pts',(-18.4720083696769,6.00961993728291,-337.1812503348)) ;
#48045=CARTESIAN_POINT('Ctrl Pts',(-18.5970868288136,5.62516129128671,-337.176280989393)) ;
#48046=CARTESIAN_POINT('Ctrl Pts',(-18.7101459426383,5.23683498527479,-337.171311643987)) ;
#48047=CARTESIAN_POINT('Ctrl Pts',(-18.8109701982584,4.84541279977611,-337.166342298581)) ;
#48048=CARTESIAN_POINT('Ctrl Pts',(-18.9116504573976,4.45454964064387,-337.161380050358)) ;
#48049=CARTESIAN_POINT('Ctrl Pts',(-19.0001575430551,4.06049559657047,-337.156417802135)) ;
#48050=CARTESIAN_POINT('Ctrl Pts',(-19.0763080860834,3.66402712937957,-337.151455553913)) ;
#48051=CARTESIAN_POINT('Ctrl Pts',(-19.1524030914331,3.26784781230418,-337.146496924728)) ;
#48052=CARTESIAN_POINT('Ctrl Pts',(-19.2161595261519,2.86925782576096,-337.141538295544)) ;
#48053=CARTESIAN_POINT('Ctrl Pts',(-19.2674454258209,2.46904268148838,-337.13657966636)) ;
#48054=CARTESIAN_POINT('Ctrl Pts',(-19.3187258345555,2.06887038632536,-337.131621568072)) ;
#48055=CARTESIAN_POINT('Ctrl Pts',(-19.3575383448397,1.66707351628882,-337.126663469785)) ;
#48056=CARTESIAN_POINT('Ctrl Pts',(-19.3838026435953,1.26444457140185,-337.121705371497)) ;
#48057=CARTESIAN_POINT('Ctrl Pts',(-19.410065351173,0.861840019105448,-337.116747573587)) ;
#48058=CARTESIAN_POINT('Ctrl Pts',(-19.4237813504955,0.458403729426894,
-337.111789775677)) ;
#48059=CARTESIAN_POINT('Ctrl Pts',(-19.4249223293586,0.054931761158904,
-337.106831977768)) ;
#48060=CARTESIAN_POINT('Ctrl Pts',(-19.4260650354402,-0.349150984618357,
-337.101866674723)) ;
#48061=CARTESIAN_POINT('Ctrl Pts',(-19.414594606145,-0.753269278588067,
-337.096901371679)) ;
#48062=CARTESIAN_POINT('Ctrl Pts',(-19.3905349991719,-1.15662329471983,
-337.091936068635)) ;
#48063=CARTESIAN_POINT('Ctrl Pts',(-19.3665092900312,-1.55940902115316,
-337.086977761258)) ;
#48064=CARTESIAN_POINT('Ctrl Pts',(-19.3299298808642,-1.96143238532242,
-337.082019453881)) ;
#48065=CARTESIAN_POINT('Ctrl Pts',(-19.2808726908508,-2.36190035336035,
-337.077061146504)) ;
#48066=CARTESIAN_POINT('Ctrl Pts',(-19.2317116787782,-2.76321585076371,
-337.072092345626)) ;
#48067=CARTESIAN_POINT('Ctrl Pts',(-19.1700200304732,-3.1629691223927,-337.067123544748)) ;
#48068=CARTESIAN_POINT('Ctrl Pts',(-19.0959261857177,-3.56036909738586,
-337.06215474387)) ;
#48069=CARTESIAN_POINT('Ctrl Pts',(-19.0218323409622,-3.95776907237912,
-337.057185942992)) ;
#48070=CARTESIAN_POINT('Ctrl Pts',(-18.9353363501988,-4.35281551644903,
-337.052217142113)) ;
#48071=CARTESIAN_POINT('Ctrl Pts',(-18.8366181158727,-4.74472791177481,
-337.047248341235)) ;
#48072=CARTESIAN_POINT('Ctrl Pts',(-18.7380300671962,-5.13612346874673,
-337.042286093013)) ;
#48073=CARTESIAN_POINT('Ctrl Pts',(-18.6272257920955,-5.52449728803654,
-337.03732384479)) ;
#48074=CARTESIAN_POINT('Ctrl Pts',(-18.5044157247767,-5.9090797663118,-337.032361596567)) ;
#48075=CARTESIAN_POINT('Ctrl Pts',(-18.3817005203881,-6.29336517919538,
-337.027403181364)) ;
#48076=CARTESIAN_POINT('Ctrl Pts',(-18.246998136401,-6.67386487967097,-337.022444766161)) ;
#48077=CARTESIAN_POINT('Ctrl Pts',(-18.1005684515657,-7.04982600708585,
-337.017486350958)) ;
#48078=CARTESIAN_POINT('Ctrl Pts',(-17.9541544989108,-7.42574674181475,
-337.01252846848)) ;
#48079=CARTESIAN_POINT('Ctrl Pts',(-17.7960158480842,-7.79712965630204,
-337.007570586001)) ;
#48080=CARTESIAN_POINT('Ctrl Pts',(-17.6264610784141,-8.16324046265651,
-337.002612703523)) ;
#48081=CARTESIAN_POINT('Ctrl Pts',(-17.4569166283541,-8.52932898641299,
-336.997655122796)) ;
#48082=CARTESIAN_POINT('Ctrl Pts',(-17.2759575472525,-8.89014582773247,
-336.992697542069)) ;
#48083=CARTESIAN_POINT('Ctrl Pts',(-17.0839397811535,-9.24497845070083,
-336.987739961342)) ;
#48084=CARTESIAN_POINT('Ctrl Pts',(-16.8916166484252,-9.6003753654231,-336.982774496554)) ;
#48085=CARTESIAN_POINT('Ctrl Pts',(-16.6881997307688,-9.94976879672292,
-336.977809031767)) ;
#48086=CARTESIAN_POINT('Ctrl Pts',(-16.474092771076,-10.2924677492807,-336.972843566979)) ;
#48087=CARTESIAN_POINT('Ctrl Pts',(-16.2603038521978,-10.6346576466718,
-336.96788547804)) ;
#48088=CARTESIAN_POINT('Ctrl Pts',(-16.0358567651614,-10.9701727451947,
-336.962927389101)) ;
#48089=CARTESIAN_POINT('Ctrl Pts',(-15.8011975416849,-11.298353032573,-336.957969300161)) ;
#48090=CARTESIAN_POINT('Ctrl Pts',(-15.566014685756,-11.6272656408298,-336.95300014745)) ;
#48091=CARTESIAN_POINT('Ctrl Pts',(-15.3205741935904,-11.9488104632796,
-336.948030994738)) ;
#48092=CARTESIAN_POINT('Ctrl Pts',(-15.0653674490457,-12.2623541224854,
-336.943061842026)) ;
#48093=CARTESIAN_POINT('Ctrl Pts',(-14.8101607045009,-12.5758977816913,
-336.938092689314)) ;
#48094=CARTESIAN_POINT('Ctrl Pts',(-14.5451878640831,-12.8814400959192,
-336.933123536602)) ;
#48095=CARTESIAN_POINT('Ctrl Pts',(-14.2709804714685,-13.1783815919469,
-336.92815438389)) ;
#48096=CARTESIAN_POINT('Ctrl Pts',(-13.9971540818256,-13.474910496646,-336.923192135668)) ;
#48097=CARTESIAN_POINT('Ctrl Pts',(-13.7140459973768,-13.7629413078253,
-336.918229887445)) ;
#48098=CARTESIAN_POINT('Ctrl Pts',(-13.4222092028062,-14.041898914182,-336.913267639222)) ;
#48099=CARTESIAN_POINT('Ctrl Pts',(-13.1305916962671,-14.3206469100115,
-336.908309119664)) ;
#48100=CARTESIAN_POINT('Ctrl Pts',(-12.8302587639553,-14.5903351670511,
-336.903350600107)) ;
#48101=CARTESIAN_POINT('Ctrl Pts',(-12.5217988324315,-14.8504268962248,
-336.898392080549)) ;
#48102=CARTESIAN_POINT('Ctrl Pts',(-12.2133719893451,-15.1104907254088,
-336.893434092891)) ;
#48103=CARTESIAN_POINT('Ctrl Pts',(-11.896820069674,-15.3609599298619,-336.888476105232)) ;
#48104=CARTESIAN_POINT('Ctrl Pts',(-11.5727653789981,-15.6013373299427,
-336.883518117574)) ;
#48105=CARTESIAN_POINT('Ctrl Pts',(-11.2487303713828,-15.8417001295161,
-336.878560431063)) ;
#48106=CARTESIAN_POINT('Ctrl Pts',(-10.9171936937525,-16.0719722079235,
-336.873602744553)) ;
#48107=CARTESIAN_POINT('Ctrl Pts',(-10.5788088385077,-16.2916981483917,
-336.868645058042)) ;
#48108=CARTESIAN_POINT('Ctrl Pts',(-10.2398984606226,-16.5117653303624,
-336.863679672084)) ;
#48109=CARTESIAN_POINT('Ctrl Pts',(-9.89411881045544,-16.7212534506777,
-336.858714286126)) ;
#48110=CARTESIAN_POINT('Ctrl Pts',(-9.54215496921257,-16.9197489208183,
-336.853748900168)) ;
#48111=CARTESIAN_POINT('Ctrl Pts',(-9.19070083574343,-17.1179569333501,
-336.848790704993)) ;
#48112=CARTESIAN_POINT('Ctrl Pts',(-8.83308062432166,-17.3052040074392,
-336.843832509819)) ;
#48113=CARTESIAN_POINT('Ctrl Pts',(-8.47000180393536,-17.4811239467413,
-336.838874314644)) ;
#48114=CARTESIAN_POINT('Ctrl Pts',(-8.10613313326873,-17.6574265864532,
-336.833905333294)) ;
#48115=CARTESIAN_POINT('Ctrl Pts',(-7.7367822872336,-17.8223526376824,-336.828936351944)) ;
#48116=CARTESIAN_POINT('Ctrl Pts',(-7.36268369354387,-17.975581042871,-336.823967370594)) ;
#48117=CARTESIAN_POINT('Ctrl Pts',(-6.98858509985413,-18.1288094480596,
-336.818998389244)) ;
#48118=CARTESIAN_POINT('Ctrl Pts',(-6.60973898280513,-18.2703401225257,
-336.814029407894)) ;
#48119=CARTESIAN_POINT('Ctrl Pts',(-6.22689881125947,-18.3999009832753,
-336.809060426544)) ;
#48120=CARTESIAN_POINT('Ctrl Pts',(-5.84457801049804,-18.5292860784421,
-336.804098186241)) ;
#48121=CARTESIAN_POINT('Ctrl Pts',(-5.45817133665694,-18.6467685768008,
-336.799135945939)) ;
#48122=CARTESIAN_POINT('Ctrl Pts',(-5.06843896709861,-18.7521079198259,
-336.794173705636)) ;
#48123=CARTESIAN_POINT('Ctrl Pts',(-4.678771758865,-18.8574296506337,-336.789212294996)) ;
#48124=CARTESIAN_POINT('Ctrl Pts',(-4.28578019389307,-18.9506122193553,
-336.784250884355)) ;
#48125=CARTESIAN_POINT('Ctrl Pts',(-3.89023860289182,-19.0314652250574,
-336.779289473715)) ;
#48126=CARTESIAN_POINT('Ctrl Pts',(-3.49473589180154,-19.1123102832827,
-336.774328550758)) ;
#48127=CARTESIAN_POINT('Ctrl Pts',(-3.09668388704589,-19.1808281510339,
-336.769367627801)) ;
#48128=CARTESIAN_POINT('Ctrl Pts',(-2.6968677880342,-19.236879402176,-336.764406704844)) ;
#48129=CARTESIAN_POINT('Ctrl Pts',(-2.29708549967659,-19.2929259133152,
-336.75944620141)) ;
#48130=CARTESIAN_POINT('Ctrl Pts',(-1.89553964953067,-19.3365078815061,
-336.754485697977)) ;
#48131=CARTESIAN_POINT('Ctrl Pts',(-1.49302284378186,-19.3675374735134,
-336.749525194543)) ;
#48132=CARTESIAN_POINT('Ctrl Pts',(-1.09050631887719,-19.3985670438707,
-336.74456469457)) ;
#48133=CARTESIAN_POINT('Ctrl Pts',(-0.68701907567866,-19.4170442368549,
-336.739604194598)) ;
#48134=CARTESIAN_POINT('Ctrl Pts',(-0.28335779853895,-19.4229331811137,
-336.734643694625)) ;
#48135=CARTESIAN_POINT('Ctrl Pts',(-0.188776922157074,-19.4243130050911,
-336.733481412134)) ;
#48136=CARTESIAN_POINT('Ctrl Pts',(-0.0941865001972844,-19.4250019592322,
-336.732319129643)) ;
#48137=CARTESIAN_POINT('Ctrl Pts',(0.000403208488304671,-19.4249999958153,
-336.731156847152)) ;
#48138=CARTESIAN_POINT('Origin',(0.,0.,-341.375)) ;
#48139=CARTESIAN_POINT('',(-1.61653377487451E-15,-13.2000000000001,-341.25)) ;
#48140=CARTESIAN_POINT('',(1.61653377487452E-15,13.2000000000001,-341.25)) ;
#48141=CARTESIAN_POINT('Origin',(0.,0.,-341.25)) ;
#48142=CARTESIAN_POINT('',(1.6471499448532E-15,13.4500000000001,-341.5)) ;
#48143=CARTESIAN_POINT('',(1.63184185986386E-15,13.3250000000001,-341.375)) ;
#48144=CARTESIAN_POINT('Origin',(0.,0.,-341.5)) ;
#48145=CARTESIAN_POINT('Origin',(0.,0.,-341.25)) ;
#48146=CARTESIAN_POINT('Origin',(0.,13.2000000000001,-341.5)) ;
#48147=CARTESIAN_POINT('',(-2.11251572852918E-15,17.25,-341.5)) ;
#48148=CARTESIAN_POINT('Origin',(0.,0.,-341.5)) ;
#48149=CARTESIAN_POINT('Origin',(0.,0.,-219.9625)) ;
#48150=CARTESIAN_POINT('',(-1.61653377487451E-15,-13.2000000000001,-98.425)) ;
#48151=CARTESIAN_POINT('Origin',(0.,0.,-98.425)) ;
#48152=CARTESIAN_POINT('',(-1.61653377487452E-15,-13.2000000000001,-219.9625)) ;
#48153=CARTESIAN_POINT('Origin',(0.,0.,-341.375)) ;
#48154=CARTESIAN_POINT('',(-2.14313189850786E-15,-17.5,-341.25)) ;
#48155=CARTESIAN_POINT('',(-2.14313189850787E-15,17.5,-341.25)) ;
#48156=CARTESIAN_POINT('Origin',(0.,0.,-341.25)) ;
#48157=CARTESIAN_POINT('',(-2.12782381351853E-15,17.375,-341.375)) ;
#48158=CARTESIAN_POINT('Origin',(0.,0.,-341.25)) ;
#48159=CARTESIAN_POINT('Origin',(0.,0.,-339.75)) ;
#48160=CARTESIAN_POINT('',(-2.14313189850786E-15,-17.5,-338.)) ;
#48161=CARTESIAN_POINT('',(-2.14313189850787E-15,-17.5,-339.75)) ;
#48162=CARTESIAN_POINT('Origin',(0.,0.,-338.)) ;
#48163=CARTESIAN_POINT('Origin',(0.,0.,-315.875)) ;
#48164=CARTESIAN_POINT('',(-2.44929359829469E-15,-19.9999999999999,-315.75)) ;
#48165=CARTESIAN_POINT('',(-2.44929359829469E-15,19.9999999999999,-315.75)) ;
#48166=CARTESIAN_POINT('Origin',(0.,0.,-315.75)) ;
#48167=CARTESIAN_POINT('',(-2.41867742831599E-15,19.7499999999997,-316.)) ;
#48168=CARTESIAN_POINT('',(-2.43398551330534E-15,19.8749999999998,-315.875)) ;
#48169=CARTESIAN_POINT('Origin',(0.,0.,-316.)) ;
#48170=CARTESIAN_POINT('Origin',(0.,0.,-315.75)) ;
#48171=CARTESIAN_POINT('Origin',(0.,0.,-281.)) ;
#48172=CARTESIAN_POINT('',(-2.44929359829469E-15,-19.9999999999999,-246.)) ;
#48173=CARTESIAN_POINT('',(-2.44929359829469E-15,-19.9999999999999,-281.)) ;
#48174=CARTESIAN_POINT('Origin',(0.,0.,-246.)) ;
#48175=CARTESIAN_POINT('',(5.00000000000251,19.3649167310363,-303.5)) ;
#48176=CARTESIAN_POINT('',(5.00000000000251,19.3649167310363,-258.5)) ;
#48177=CARTESIAN_POINT('',(5.00000000000251,19.3649167310363,-281.)) ;
#48178=CARTESIAN_POINT('',(-5.00000000000251,19.3649167310363,-258.5)) ;
#48179=CARTESIAN_POINT('Ctrl Pts',(5.00000000000251,19.3649167310363,-258.5)) ;
#48180=CARTESIAN_POINT('Ctrl Pts',(5.00000000000251,19.3649167310363,-257.869252946608)) ;
#48181=CARTESIAN_POINT('Ctrl Pts',(4.87339527045222,19.3989431732835,-257.198391459947)) ;
#48182=CARTESIAN_POINT('Ctrl Pts',(4.36231992558286,19.5202238889459,-255.967346574847)) ;
#48183=CARTESIAN_POINT('Ctrl Pts',(3.97798553913109,19.6055530258166,-255.406917727262)) ;
#48184=CARTESIAN_POINT('Ctrl Pts',(3.0931441353592,19.7644752333869,-254.52207632349)) ;
#48185=CARTESIAN_POINT('Ctrl Pts',(2.5326895230115,19.8486251890166,-254.137693703462)) ;
#48186=CARTESIAN_POINT('Ctrl Pts',(1.30155327908315,19.9671830048977,-253.626583144847)) ;
#48187=CARTESIAN_POINT('Ctrl Pts',(0.630658863716503,19.9999999999999,-253.499999999998)) ;
#48188=CARTESIAN_POINT('Ctrl Pts',(-0.630658863716505,19.9999999999999,
-253.499999999997)) ;
#48189=CARTESIAN_POINT('Ctrl Pts',(-1.30155327908312,19.9671830048977,-253.626583144847)) ;
#48190=CARTESIAN_POINT('Ctrl Pts',(-2.53268952301149,19.8486251890166,-254.137693703461)) ;
#48191=CARTESIAN_POINT('Ctrl Pts',(-3.0931441353592,19.7644752333869,-254.52207632349)) ;
#48192=CARTESIAN_POINT('Ctrl Pts',(-3.97798553913109,19.6055530258166,-255.406917727262)) ;
#48193=CARTESIAN_POINT('Ctrl Pts',(-4.36231992558286,19.5202238889459,-255.967346574847)) ;
#48194=CARTESIAN_POINT('Ctrl Pts',(-4.87339527045222,19.3989431732835,-257.198391459947)) ;
#48195=CARTESIAN_POINT('Ctrl Pts',(-5.00000000000251,19.3649167310363,-257.869252946608)) ;
#48196=CARTESIAN_POINT('Ctrl Pts',(-5.00000000000251,19.3649167310363,-258.5)) ;
#48197=CARTESIAN_POINT('',(-5.00000000000251,19.3649167310363,-303.5)) ;
#48198=CARTESIAN_POINT('',(-5.00000000000251,19.3649167310363,-281.)) ;
#48199=CARTESIAN_POINT('Ctrl Pts',(-5.00000000000251,19.3649167310363,-303.5)) ;
#48200=CARTESIAN_POINT('Ctrl Pts',(-5.00000000000251,19.3649167310363,-304.130747053392)) ;
#48201=CARTESIAN_POINT('Ctrl Pts',(-4.87339527045224,19.3989431732835,-304.801608540053)) ;
#48202=CARTESIAN_POINT('Ctrl Pts',(-4.36231992558289,19.5202238889459,-306.032653425153)) ;
#48203=CARTESIAN_POINT('Ctrl Pts',(-3.97798553913108,19.6055530258166,-306.593082272738)) ;
#48204=CARTESIAN_POINT('Ctrl Pts',(-3.0931441353592,19.7644752333869,-307.47792367651)) ;
#48205=CARTESIAN_POINT('Ctrl Pts',(-2.53268952301149,19.8486251890166,-307.862306296539)) ;
#48206=CARTESIAN_POINT('Ctrl Pts',(-1.30155327908312,19.9671830048977,-308.373416855153)) ;
#48207=CARTESIAN_POINT('Ctrl Pts',(-0.630658863716505,19.9999999999999,
-308.500000000003)) ;
#48208=CARTESIAN_POINT('Ctrl Pts',(0.630658863716504,19.9999999999999,-308.500000000003)) ;
#48209=CARTESIAN_POINT('Ctrl Pts',(1.30155327908312,19.9671830048977,-308.373416855153)) ;
#48210=CARTESIAN_POINT('Ctrl Pts',(2.53268952301149,19.8486251890166,-307.862306296539)) ;
#48211=CARTESIAN_POINT('Ctrl Pts',(3.0931441353592,19.7644752333869,-307.47792367651)) ;
#48212=CARTESIAN_POINT('Ctrl Pts',(3.97798553913108,19.6055530258166,-306.593082272738)) ;
#48213=CARTESIAN_POINT('Ctrl Pts',(4.36231992558286,19.5202238889459,-306.032653425153)) ;
#48214=CARTESIAN_POINT('Ctrl Pts',(4.87339527045222,19.3989431732835,-304.801608540053)) ;
#48215=CARTESIAN_POINT('Ctrl Pts',(5.00000000000251,19.3649167310363,-304.130747053392)) ;
#48216=CARTESIAN_POINT('Ctrl Pts',(5.00000000000251,19.3649167310363,-303.5)) ;
#48217=CARTESIAN_POINT('Origin',(0.,18.,-316.)) ;
#48218=CARTESIAN_POINT('',(-2.20436423846523E-15,-18.,-316.)) ;
#48219=CARTESIAN_POINT('Origin',(0.,0.,-316.)) ;
#48220=CARTESIAN_POINT('Origin',(0.,0.,-245.875)) ;
#48221=CARTESIAN_POINT('',(-2.75545529808154E-15,-22.5,-245.75)) ;
#48222=CARTESIAN_POINT('',(-2.75545529808155E-15,22.5,-245.75)) ;
#48223=CARTESIAN_POINT('Origin',(0.,0.,-245.75)) ;
#48224=CARTESIAN_POINT('',(-2.72483912810286E-15,22.25,-246.)) ;
#48225=CARTESIAN_POINT('',(-2.7401472130922E-15,22.375,-245.875)) ;
#48226=CARTESIAN_POINT('Origin',(0.,0.,-246.)) ;
#48227=CARTESIAN_POINT('Origin',(0.,0.,-245.75)) ;
#48228=CARTESIAN_POINT('Origin',(0.,0.,-225.)) ;
#48229=CARTESIAN_POINT('',(-2.75545529808154E-15,-22.5,-204.)) ;
#48230=CARTESIAN_POINT('',(-2.75545529808154E-15,-22.5,-225.)) ;
#48231=CARTESIAN_POINT('Origin',(0.,0.,-204.)) ;
#48232=CARTESIAN_POINT('Origin',(0.,20.,-246.)) ;
#48233=CARTESIAN_POINT('Origin',(-1.0184458207166E-15,0.,-36.917598465851)) ;
#48234=CARTESIAN_POINT('',(-4.10256677714363E-15,-33.5,-36.75)) ;
#48235=CARTESIAN_POINT('',(-3.08053568558583E-15,33.5000000000001,-36.7499999999998)) ;
#48236=CARTESIAN_POINT('Origin',(0.,0.,-36.75)) ;
#48237=CARTESIAN_POINT('',(-5.09581437442459E-15,33.2649649327683,-37.0851969317022)) ;
#48238=CARTESIAN_POINT('',(-4.08817503000501E-15,33.3824824663842,-36.917598465851)) ;
#48239=CARTESIAN_POINT('',(-4.07378328286638E-15,-33.2649649327684,-37.0851969317021)) ;
#48240=CARTESIAN_POINT('Origin',(-2.03689164143319E-15,0.,-37.0851969317021)) ;
#48241=CARTESIAN_POINT('Origin',(-2.03689164143319E-15,0.,-37.0851969317021)) ;
#48242=CARTESIAN_POINT('Origin',(0.,0.,-36.75)) ;
#48243=CARTESIAN_POINT('Origin',(0.,0.,-35.5)) ;
#48244=CARTESIAN_POINT('',(-4.10256677714363E-15,-33.5,-34.25)) ;
#48245=CARTESIAN_POINT('',(-4.10256677714363E-15,-33.5,-35.5)) ;
#48246=CARTESIAN_POINT('',(-4.10256677714363E-15,33.5,-34.25)) ;
#48247=CARTESIAN_POINT('Origin',(0.,0.,-34.25)) ;
#48248=CARTESIAN_POINT('Origin',(0.,0.,-34.25)) ;
#48249=CARTESIAN_POINT('Origin',(0.,0.,-39.435)) ;
#48250=CARTESIAN_POINT('',(-2.45725380248917E-15,-20.065,-41.87)) ;
#48251=CARTESIAN_POINT('',(3.2799102898164E-15,-26.7825,-39.435)) ;
#48252=CARTESIAN_POINT('Origin',(0.,0.,-41.87)) ;
#48253=CARTESIAN_POINT('Origin',(0.,0.,-34.125)) ;
#48254=CARTESIAN_POINT('',(4.07195060716495E-15,33.25,-34.)) ;
#48255=CARTESIAN_POINT('',(4.08725869215429E-15,33.375,-34.125)) ;
#48256=CARTESIAN_POINT('Origin',(0.,0.,-34.)) ;
#48257=CARTESIAN_POINT('Origin',(0.,33.5,-34.)) ;
#48258=CARTESIAN_POINT('',(-2.81668763803891E-15,-23.,-34.)) ;
#48259=CARTESIAN_POINT('Origin',(0.,0.,-34.)) ;
#48260=CARTESIAN_POINT('Origin',(-4.78454817191255E-16,0.,-0.124961805206562)) ;
#48261=CARTESIAN_POINT('',(-1.91381926876502E-15,-15.6275202784794,-0.249923610413125)) ;
#48262=CARTESIAN_POINT('',(-2.39616382493652E-15,15.6275202784794,-0.249923610413161)) ;
#48263=CARTESIAN_POINT('Origin',(-9.56909634382509E-16,0.,-0.249923610413125)) ;
#48264=CARTESIAN_POINT('',(-1.94519223636168E-15,15.8837,9.71445146547012E-16)) ;
#48265=CARTESIAN_POINT('',(-1.92950575256335E-15,15.7556101392397,-0.124961805206562)) ;
#48266=CARTESIAN_POINT('Origin',(0.,0.,9.71445146547012E-16)) ;
#48267=CARTESIAN_POINT('Origin',(-9.56909634382509E-16,0.,-0.249923610413125)) ;
#48268=CARTESIAN_POINT('Origin',(0.,0.,-49.2125)) ;
#48269=CARTESIAN_POINT('',(1.76555492062875E-15,-14.41685,-49.2125)) ;
#48270=CARTESIAN_POINT('Origin',(0.,22.225,9.73307724266206E-16)) ;
#48271=CARTESIAN_POINT('Ctrl Pts',(19.8220328557588,-9.83935203800092,1.06632628357545E-15)) ;
#48272=CARTESIAN_POINT('Ctrl Pts',(18.7256935583061,-11.8448496981576,1.06632628357545E-15)) ;
#48273=CARTESIAN_POINT('Ctrl Pts',(17.312558092614,-13.6768414356383,1.8727957933688E-14)) ;
#48274=CARTESIAN_POINT('Ctrl Pts',(14.015585104321,-16.8064082536566,1.87419927850467E-14)) ;
#48275=CARTESIAN_POINT('Ctrl Pts',(12.1519545368752,-18.0953645953734,1.88595907275818E-14)) ;
#48276=CARTESIAN_POINT('Ctrl Pts',(7.64400019407915,-20.2482066689093,1.8890824010698E-14)) ;
#48277=CARTESIAN_POINT('Ctrl Pts',(4.95667918313636,-20.9612135442109,1.93508252162319E-14)) ;
#48278=CARTESIAN_POINT('Ctrl Pts',(-0.455353294293309,-21.3054222919409,
1.93680485543092E-14)) ;
#48279=CARTESIAN_POINT('Ctrl Pts',(-3.17087267179517,-20.9577083375656,
1.9003901490213E-14)) ;
#48280=CARTESIAN_POINT('Ctrl Pts',(-8.50806489536336,-19.201173436068,1.90220305273563E-14)) ;
#48281=CARTESIAN_POINT('Ctrl Pts',(-10.5078011878526,-17.8999277787963,
1.90472637662253E-14)) ;
#48282=CARTESIAN_POINT('Ctrl Pts',(-13.6119178368781,-15.531364223185,1.90472637662253E-14)) ;
#48283=CARTESIAN_POINT('Ctrl Pts',(-15.1685873535527,-13.8859540469984,
1.06094944223971E-15)) ;
#48284=CARTESIAN_POINT('Ctrl Pts',(-16.4382148282781,-11.9710934804215,
1.06094944223971E-15)) ;
#48285=CARTESIAN_POINT('Ctrl Pts',(19.8228138270522,9.84020336516649,1.34055093414798E-14)) ;
#48286=CARTESIAN_POINT('Ctrl Pts',(19.6074231646947,10.2350439781308,-1.20645810543802E-14)) ;
#48287=CARTESIAN_POINT('Ctrl Pts',(19.3802577079734,10.622633695729,-2.56087321916339E-14)) ;
#48288=CARTESIAN_POINT('Ctrl Pts',(19.1415354306511,11.0024033777635,2.41473507855972E-15)) ;
#48289=CARTESIAN_POINT('Ctrl Pts',(19.1139547928099,11.0462798445128,5.65240988001737E-15)) ;
#48290=CARTESIAN_POINT('Ctrl Pts',(19.0862198398917,11.0900519047123,-5.99600758964009E-16)) ;
#48291=CARTESIAN_POINT('Ctrl Pts',(19.0583308674199,11.1337186616126,-1.60982338570648E-15)) ;
#48292=CARTESIAN_POINT('Ctrl Pts',(18.8185994249655,11.5090747142446,-1.67263190955323E-14)) ;
#48293=CARTESIAN_POINT('Ctrl Pts',(18.5674911810468,11.8766522063334,6.20331908650578E-15)) ;
#48294=CARTESIAN_POINT('Ctrl Pts',(18.305518211608,12.2360701986977,-3.88578058618805E-16)) ;
#48295=CARTESIAN_POINT('Ctrl Pts',(18.0280899316194,12.6166923507932,-7.36936959124135E-15)) ;
#48296=CARTESIAN_POINT('Ctrl Pts',(17.7384771323971,12.9881646223063,-2.38201952126546E-14)) ;
#48297=CARTESIAN_POINT('Ctrl Pts',(17.4372377992249,13.3499967502053,-2.71727085277007E-14)) ;
#48298=CARTESIAN_POINT('Ctrl Pts',(17.150352123501,13.6945880537969,-3.03654789990466E-14)) ;
#48299=CARTESIAN_POINT('Ctrl Pts',(16.8529207396947,14.0304360740663,-1.60020091492236E-14)) ;
#48300=CARTESIAN_POINT('Ctrl Pts',(16.5453886606796,14.3570789058094,-2.22044604925031E-15)) ;
#48301=CARTESIAN_POINT('Ctrl Pts',(16.2391851977278,14.6823105582225,1.15015772258955E-14)) ;
#48302=CARTESIAN_POINT('Ctrl Pts',(15.9229677023102,14.9984167156392,-1.2744609087233E-14)) ;
#48303=CARTESIAN_POINT('Ctrl Pts',(15.5971461057912,15.3048990809629,-2.96984659087229E-15)) ;
#48304=CARTESIAN_POINT('Ctrl Pts',(15.2750178968041,15.6079072807955,6.69411298045808E-15)) ;
#48305=CARTESIAN_POINT('Ctrl Pts',(14.9435016656073,15.9015088957369,-1.53065317057012E-14)) ;
#48306=CARTESIAN_POINT('Ctrl Pts',(14.6029711553433,16.1851766092926,-4.90996132640475E-14)) ;
#48307=CARTESIAN_POINT('Ctrl Pts',(14.5441544529413,16.234171923916,-5.49363813695624E-14)) ;
#48308=CARTESIAN_POINT('Ctrl Pts',(14.4850687865257,16.2828707685809,-3.91470895560732E-14)) ;
#48309=CARTESIAN_POINT('Ctrl Pts',(14.4257160273708,16.3312702768893,-2.78943534937071E-14)) ;
#48310=CARTESIAN_POINT('Ctrl Pts',(14.3863249576248,16.3633919243846,-2.14168009086151E-14)) ;
#48311=CARTESIAN_POINT('Ctrl Pts',(14.3468162906582,16.3953816143755,2.55660740366257E-14)) ;
#48312=CARTESIAN_POINT('Ctrl Pts',(14.3072086441427,16.4272241757195,1.9151347174784E-14)) ;
#48313=CARTESIAN_POINT('Ctrl Pts',(13.9605448541076,16.7059244765716,-3.87855050643946E-14)) ;
#48314=CARTESIAN_POINT('Ctrl Pts',(13.6059581611611,16.9736384700472,-5.8062702315595E-15)) ;
#48315=CARTESIAN_POINT('Ctrl Pts',(13.2439289076318,17.2299784476699,-1.18238752122579E-14)) ;
#48316=CARTESIAN_POINT('Ctrl Pts',(12.8825651717075,17.4858471960581,-2.02521983471332E-14)) ;
#48317=CARTESIAN_POINT('Ctrl Pts',(12.5137857853607,17.7303840336224,-2.6898344299621E-15)) ;
#48318=CARTESIAN_POINT('Ctrl Pts',(12.1380355501591,17.9631634907815,4.9960036108132E-16)) ;
#48319=CARTESIAN_POINT('Ctrl Pts',(11.8446125856444,18.1449407246962,2.99022664375559E-15)) ;
#48320=CARTESIAN_POINT('Ctrl Pts',(11.5469380627986,18.3195475322449,-8.13343317425171E-15)) ;
#48321=CARTESIAN_POINT('Ctrl Pts',(11.2452123078566,18.4867623983207,8.49320613838245E-15)) ;
#48322=CARTESIAN_POINT('Ctrl Pts',(10.857561087322,18.7015967167841,2.95407530613509E-14)) ;
#48323=CARTESIAN_POINT('Ctrl Pts',(10.4632229713425,18.9042311381886,9.732185371864E-15)) ;
#48324=CARTESIAN_POINT('Ctrl Pts',(10.0628171189943,19.0945064137273,-4.9960036108132E-16)) ;
#48325=CARTESIAN_POINT('Ctrl Pts',(9.66298658844184,19.2845082928793,-8.45008909837143E-15)) ;
#48326=CARTESIAN_POINT('Ctrl Pts',(9.25710520567581,19.4621866299123,1.22637826195654E-14)) ;
#48327=CARTESIAN_POINT('Ctrl Pts',(8.8457760432505,19.627332765732,-5.55111512312578E-17)) ;
#48328=CARTESIAN_POINT('Ctrl Pts',(8.53780141147367,19.7509826914229,-9.2793404086585E-15)) ;
#48329=CARTESIAN_POINT('Ctrl Pts',(8.22677244688017,19.8676060859205,1.04033125354434E-15)) ;
#48330=CARTESIAN_POINT('Ctrl Pts',(7.91294008103285,19.977096345354,-8.71525074330748E-15)) ;
#48331=CARTESIAN_POINT('Ctrl Pts',(7.63833676091647,20.0729003223583,-1.75224632892377E-14)) ;
#48332=CARTESIAN_POINT('Ctrl Pts',(7.36158700918664,20.1632427620598,1.52212933278802E-14)) ;
#48333=CARTESIAN_POINT('Ctrl Pts',(7.08285900561331,20.2480417027558,8.82627304576999E-15)) ;
#48334=CARTESIAN_POINT('Ctrl Pts',(7.02245463792221,20.266418852981,9.81933546972611E-15)) ;
#48335=CARTESIAN_POINT('Ctrl Pts',(6.96195203920544,20.2845371110464,6.60519354014801E-15)) ;
#48336=CARTESIAN_POINT('Ctrl Pts',(6.90139191111684,20.3023843105404,2.60902410786912E-15)) ;
#48337=CARTESIAN_POINT('Ctrl Pts',(6.4810143637177,20.4262704743915,-2.51303476199288E-14)) ;
#48338=CARTESIAN_POINT('Ctrl Pts',(6.05750679718693,20.5372117643199,4.43698005455285E-15)) ;
#48339=CARTESIAN_POINT('Ctrl Pts',(5.63148115000663,20.6351157318689,8.38218383591993E-15)) ;
#48340=CARTESIAN_POINT('Ctrl Pts',(5.20377541173699,20.733405797261,1.23429460743014E-14)) ;
#48341=CARTESIAN_POINT('Ctrl Pts',(4.77353116434053,20.8185556423175,6.00693556424402E-16)) ;
#48342=CARTESIAN_POINT('Ctrl Pts',(4.34135215828707,20.8904217445994,-5.82867087928207E-15)) ;
#48343=CARTESIAN_POINT('Ctrl Pts',(3.91039323098268,20.9620849626529,-1.2239884662578E-14)) ;
#48344=CARTESIAN_POINT('Ctrl Pts',(3.47750992241484,21.0205394167474,-1.30572816134376E-14)) ;
#48345=CARTESIAN_POINT('Ctrl Pts',(3.04329351149669,21.0655916653857,-1.51545442861334E-14)) ;
#48346=CARTESIAN_POINT('Ctrl Pts',(2.6136131553603,21.110173274355,-1.72298978413111E-14)) ;
#48347=CARTESIAN_POINT('Ctrl Pts',(2.18262690328141,21.1416312474094,-1.65856428524431E-14)) ;
#48348=CARTESIAN_POINT('Ctrl Pts',(1.75090813930699,21.1597273498772,-1.80966353013901E-14)) ;
#48349=CARTESIAN_POINT('Ctrl Pts',(1.52712976980441,21.1691073366708,-1.88798475561534E-14)) ;
#48350=CARTESIAN_POINT('Ctrl Pts',(1.30315464273741,21.1748964269943,-1.84395128730138E-15)) ;
#48351=CARTESIAN_POINT('Ctrl Pts',(1.07906332965069,21.1770559515521,1.4432899320127E-15)) ;
#48352=CARTESIAN_POINT('Ctrl Pts',(0.641773282680246,21.1812700309928,8.82403367971152E-15)) ;
#48353=CARTESIAN_POINT('Ctrl Pts',(0.204039724449181,21.1716658755645,3.6105059716605E-16)) ;
#48354=CARTESIAN_POINT('Ctrl Pts',(-0.233502727656554,21.1483303925341,
-2.20934381900406E-14)) ;
#48355=CARTESIAN_POINT('Ctrl Pts',(-0.513863661777233,21.1333778826941,
-3.64814396771792E-14)) ;
#48356=CARTESIAN_POINT('Ctrl Pts',(-0.794145855950668,21.1127866005285,
-1.39896370025936E-14)) ;
#48357=CARTESIAN_POINT('Ctrl Pts',(-1.07417808744935,21.0865689806994,-1.18793863634892E-14)) ;
#48358=CARTESIAN_POINT('Ctrl Pts',(-1.14281457396794,21.0801429871617,-1.17339881484418E-14)) ;
#48359=CARTESIAN_POINT('Ctrl Pts',(-1.21144568059705,21.0733778889363,-1.76353721084238E-15)) ;
#48360=CARTESIAN_POINT('Ctrl Pts',(-1.28002014750725,21.066279033268,-2.99760216648792E-15)) ;
#48361=CARTESIAN_POINT('Ctrl Pts',(-1.70928825621511,21.0218410305531,-1.07227038464811E-14)) ;
#48362=CARTESIAN_POINT('Ctrl Pts',(-2.13658153340179,20.9643096570965,-1.92478364575703E-15)) ;
#48363=CARTESIAN_POINT('Ctrl Pts',(-2.56131517767835,20.893916388905,-6.88338275267597E-15)) ;
#48364=CARTESIAN_POINT('Ctrl Pts',(-2.98873827821317,20.8230773834421,-1.18733802090783E-14)) ;
#48365=CARTESIAN_POINT('Ctrl Pts',(-3.41356976186588,20.73921296819,2.40111047890402E-14)) ;
#48366=CARTESIAN_POINT('Ctrl Pts',(-3.83520895094919,20.6425063982639,2.66453525910038E-15)) ;
#48367=CARTESIAN_POINT('Ctrl Pts',(-4.27817603871496,20.540908091567,-1.97618140539818E-14)) ;
#48368=CARTESIAN_POINT('Ctrl Pts',(-4.71762046092072,20.4251358631229,6.40030023097509E-15)) ;
#48369=CARTESIAN_POINT('Ctrl Pts',(-5.15283049846049,20.2953424105776,-1.14352971536391E-14)) ;
#48370=CARTESIAN_POINT('Ctrl Pts',(-5.56435027920578,20.1726141448519,-2.83000302527855E-14)) ;
#48371=CARTESIAN_POINT('Ctrl Pts',(-5.9720844719591,20.0373489532768,-1.23970021057823E-14)) ;
#48372=CARTESIAN_POINT('Ctrl Pts',(-6.37541049791806,19.8896279309333,-1.36557432028894E-14)) ;
#48373=CARTESIAN_POINT('Ctrl Pts',(-6.77519136264614,19.7432053490764,-1.49034201983767E-14)) ;
#48374=CARTESIAN_POINT('Ctrl Pts',(-7.17064166815835,19.5845447436151,-2.78931875295902E-14)) ;
#48375=CARTESIAN_POINT('Ctrl Pts',(-7.5611279233789,19.4136819694644,-3.05311331771918E-14)) ;
#48376=CARTESIAN_POINT('Ctrl Pts',(-7.9453202571054,19.2455731895258,-3.31265599842719E-14)) ;
#48377=CARTESIAN_POINT('Ctrl Pts',(-8.3247076496214,19.0656521971063,-2.66868924829354E-15)) ;
#48378=CARTESIAN_POINT('Ctrl Pts',(-8.6986542569747,18.8739144354475,4.9960036108132E-15)) ;
#48379=CARTESIAN_POINT('Ctrl Pts',(-8.77774295260813,18.8333624176592,6.61706541144845E-15)) ;
#48380=CARTESIAN_POINT('Ctrl Pts',(-8.85658814700664,18.7922816896624,5.54102316483117E-15)) ;
#48381=CARTESIAN_POINT('Ctrl Pts',(-8.93518360999352,18.7506719960506,1.16573417585641E-14)) ;
#48382=CARTESIAN_POINT('Ctrl Pts',(-9.03512384585114,18.6977620387133,1.74862619942157E-14)) ;
#48383=CARTESIAN_POINT('Ctrl Pts',(-9.13460192966983,18.6440276319535,2.15689584339014E-14)) ;
#48384=CARTESIAN_POINT('Ctrl Pts',(-9.23360112208329,18.5894827195556,1.88737914186277E-14)) ;
#48385=CARTESIAN_POINT('Ctrl Pts',(-9.60858213954734,18.3828819761573,8.66525895502832E-15)) ;
#48386=CARTESIAN_POINT('Ctrl Pts',(-9.97673794510111,18.16463371319,-3.538201205195E-15)) ;
#48387=CARTESIAN_POINT('Ctrl Pts',(-10.337640427971,17.9352025800157,6.43929354282591E-15)) ;
#48388=CARTESIAN_POINT('Ctrl Pts',(-10.6998376712863,17.7049483481643,1.64525831832557E-14)) ;
#48389=CARTESIAN_POINT('Ctrl Pts',(-11.0547298655919,17.4634304923052,-8.11039614496874E-15)) ;
#48390=CARTESIAN_POINT('Ctrl Pts',(-11.4018536678929,17.2110758102307,8.88178419700125E-16)) ;
#48391=CARTESIAN_POINT('Ctrl Pts',(-11.6973988559854,16.9962181384567,8.54966805149802E-15)) ;
#48392=CARTESIAN_POINT('Ctrl Pts',(-11.9873123492652,16.7735039907288,-5.06816677905142E-15)) ;
#48393=CARTESIAN_POINT('Ctrl Pts',(-12.2712874273964,16.5431754731543,-1.0325074129014E-14)) ;
#48394=CARTESIAN_POINT('Ctrl Pts',(-12.45058942981,16.3977459351616,-1.36442879859274E-14)) ;
#48395=CARTESIAN_POINT('Ctrl Pts',(-12.6275235917963,16.2492804225787,1.01350113779492E-14)) ;
#48396=CARTESIAN_POINT('Ctrl Pts',(-12.802008271987,16.0978363572816,-1.11022302462516E-15)) ;
#48397=CARTESIAN_POINT('Ctrl Pts',(-12.9038690872333,16.0094262118262,-7.6749755440494E-15)) ;
#48398=CARTESIAN_POINT('Ctrl Pts',(-13.0048967359161,15.9199994139826,-2.97934760950595E-14)) ;
#48399=CARTESIAN_POINT('Ctrl Pts',(-13.1050699521942,15.8295709857237,-2.56461518688411E-14)) ;
#48400=CARTESIAN_POINT('Ctrl Pts',(-13.1481766308034,15.7906576979317,-2.52283304015882E-14)) ;
#48401=CARTESIAN_POINT('Ctrl Pts',(-13.1911199874146,15.7515634969923,1.05548090712835E-14)) ;
#48402=CARTESIAN_POINT('Ctrl Pts',(-13.2338908622103,15.7122967829054,6.66133814775094E-15)) ;
#48403=CARTESIAN_POINT('Ctrl Pts',(-13.5479994724106,15.4239226720676,-2.37149819284577E-14)) ;
#48404=CARTESIAN_POINT('Ctrl Pts',(-13.8529315665021,15.1261364324721,-1.00319302306805E-14)) ;
#48405=CARTESIAN_POINT('Ctrl Pts',(-14.1482389299246,14.8193621077826,-9.76996261670138E-15)) ;
#48406=CARTESIAN_POINT('Ctrl Pts',(-14.4425915472528,14.5135796025483,-9.3945195395561E-15)) ;
#48407=CARTESIAN_POINT('Ctrl Pts',(-14.7273819262516,14.1988666297625,1.38838895804111E-14)) ;
#48408=CARTESIAN_POINT('Ctrl Pts',(-15.0021274209657,13.8756091472101,-5.10702591327572E-15)) ;
#48409=CARTESIAN_POINT('Ctrl Pts',(-15.2735129861793,13.5563048590604,-2.38656968809E-14)) ;
#48410=CARTESIAN_POINT('Ctrl Pts',(-15.5350981239967,13.2286633506192,-1.0903397624211E-15)) ;
#48411=CARTESIAN_POINT('Ctrl Pts',(-15.7863751831239,12.8930295683571,6.66133814775094E-16)) ;
#48412=CARTESIAN_POINT('Ctrl Pts',(-16.0074080429584,12.5977933259076,2.21119478985973E-15)) ;
#48413=CARTESIAN_POINT('Ctrl Pts',(-16.2204644323149,12.2963724144037,-5.1689895147707E-15)) ;
#48414=CARTESIAN_POINT('Ctrl Pts',(-16.4251684725406,11.9889877181628,4.66293670342566E-15)) ;
#48415=CARTESIAN_POINT('Origin',(0.,0.,-55.875)) ;
#48416=CARTESIAN_POINT('',(-4.10256677714363E-15,-33.5,-55.75)) ;
#48417=CARTESIAN_POINT('',(-4.10256677714363E-15,33.5,-55.75)) ;
#48418=CARTESIAN_POINT('Origin',(0.,0.,-55.75)) ;
#48419=CARTESIAN_POINT('',(-4.07195060716495E-15,33.25,-56.)) ;
#48420=CARTESIAN_POINT('',(-4.08725869215429E-15,33.375,-55.875)) ;
#48421=CARTESIAN_POINT('Origin',(0.,0.,-56.)) ;
#48422=CARTESIAN_POINT('Origin',(0.,0.,-55.75)) ;
#48423=CARTESIAN_POINT('Origin',(0.,0.,-49.935)) ;
#48424=CARTESIAN_POINT('',(-4.10256677714363E-15,-33.5,-44.12)) ;
#48425=CARTESIAN_POINT('',(-4.10256677714363E-15,-33.5,-49.935)) ;
#48426=CARTESIAN_POINT('',(-4.10256677714363E-15,33.5,-44.12)) ;
#48427=CARTESIAN_POINT('Origin',(0.,0.,-44.12)) ;
#48428=CARTESIAN_POINT('Origin',(0.,0.,-44.12)) ;
#48429=CARTESIAN_POINT('',(27.103076092507,-19.6894201622032,-49.935)) ;
#48430=CARTESIAN_POINT('Ctrl Pts',(27.103076092507,-19.6894201622032,-49.935)) ;
#48431=CARTESIAN_POINT('Ctrl Pts',(27.103076092507,-19.6894201622032,-49.4951866852561)) ;
#48432=CARTESIAN_POINT('Ctrl Pts',(27.1553769624387,-19.6180456661006,-49.0262784098868)) ;
#48433=CARTESIAN_POINT('Ctrl Pts',(27.3640256598749,-19.3259492202238,-48.1640465487623)) ;
#48434=CARTESIAN_POINT('Ctrl Pts',(27.5199265959608,-19.1049894709151,-47.7706954545604)) ;
#48435=CARTESIAN_POINT('Ctrl Pts',(27.8703439079723,-18.590075637148,-47.1495583377523)) ;
#48436=CARTESIAN_POINT('Ctrl Pts',(28.088216344668,-18.2616609897394,-46.8802501289145)) ;
#48437=CARTESIAN_POINT('Ctrl Pts',(28.5492221416872,-17.5322010777203,-46.5229621057665)) ;
#48438=CARTESIAN_POINT('Ctrl Pts',(28.7919452620208,-17.130887957438,-46.435)) ;
#48439=CARTESIAN_POINT('Ctrl Pts',(29.2317567915366,-16.369112042562,-46.435)) ;
#48440=CARTESIAN_POINT('Ctrl Pts',(29.4579425884063,-15.9582510941262,-46.5229621057665)) ;
#48441=CARTESIAN_POINT('Ctrl Pts',(29.8591705047475,-15.1942784066061,-46.8802501289145)) ;
#48442=CARTESIAN_POINT('Ctrl Pts',(30.0346497140305,-14.841388017939,-47.1495583377523)) ;
#48443=CARTESIAN_POINT('Ctrl Pts',(30.3053695188271,-14.2804608069275,-47.7706954545604)) ;
#48444=CARTESIAN_POINT('Ctrl Pts',(30.4187758068994,-14.034966761149,-48.1640465487623)) ;
#48445=CARTESIAN_POINT('Ctrl Pts',(30.5674144006656,-13.7082234657643,-49.0262784098868)) ;
#48446=CARTESIAN_POINT('Ctrl Pts',(30.603076092507,-13.6272423357122,-49.4951866852561)) ;
#48447=CARTESIAN_POINT('Ctrl Pts',(30.603076092507,-13.6272423357122,-50.3748133147439)) ;
#48448=CARTESIAN_POINT('Ctrl Pts',(30.5674144006656,-13.7082234657643,-50.8437215901132)) ;
#48449=CARTESIAN_POINT('Ctrl Pts',(30.4187758068994,-14.0349667611491,-51.7059534512376)) ;
#48450=CARTESIAN_POINT('Ctrl Pts',(30.3053695188271,-14.2804608069275,-52.0993045454395)) ;
#48451=CARTESIAN_POINT('Ctrl Pts',(30.0346497140305,-14.841388017939,-52.7204416622477)) ;
#48452=CARTESIAN_POINT('Ctrl Pts',(29.8591705047475,-15.1942784066061,-52.9897498710854)) ;
#48453=CARTESIAN_POINT('Ctrl Pts',(29.4579425884063,-15.9582510941262,-53.3470378942334)) ;
#48454=CARTESIAN_POINT('Ctrl Pts',(29.2317567915366,-16.369112042562,-53.435)) ;
#48455=CARTESIAN_POINT('Ctrl Pts',(28.7919452620208,-17.130887957438,-53.435)) ;
#48456=CARTESIAN_POINT('Ctrl Pts',(28.5492221416872,-17.5322010777204,-53.3470378942334)) ;
#48457=CARTESIAN_POINT('Ctrl Pts',(28.088216344668,-18.2616609897394,-52.9897498710854)) ;
#48458=CARTESIAN_POINT('Ctrl Pts',(27.8703439079723,-18.590075637148,-52.7204416622477)) ;
#48459=CARTESIAN_POINT('Ctrl Pts',(27.5199265959608,-19.1049894709151,-52.0993045454395)) ;
#48460=CARTESIAN_POINT('Ctrl Pts',(27.3640256598749,-19.3259492202238,-51.7059534512376)) ;
#48461=CARTESIAN_POINT('Ctrl Pts',(27.1553769624387,-19.6180456661006,-50.8437215901132)) ;
#48462=CARTESIAN_POINT('Ctrl Pts',(27.103076092507,-19.6894201622032,-50.3748133147439)) ;
#48463=CARTESIAN_POINT('Ctrl Pts',(27.103076092507,-19.6894201622032,-49.935)) ;
#48464=CARTESIAN_POINT('',(-30.603076092507,-13.6272423357121,-49.935)) ;
#48465=CARTESIAN_POINT('Ctrl Pts',(-30.603076092507,-13.6272423357121,-49.935)) ;
#48466=CARTESIAN_POINT('Ctrl Pts',(-30.603076092507,-13.6272423357121,-49.4951866852561)) ;
#48467=CARTESIAN_POINT('Ctrl Pts',(-30.5674144006657,-13.7082234657643,
-49.0262784098868)) ;
#48468=CARTESIAN_POINT('Ctrl Pts',(-30.4187758068994,-14.034966761149,-48.1640465487624)) ;
#48469=CARTESIAN_POINT('Ctrl Pts',(-30.3053695188271,-14.2804608069275,
-47.7706954545604)) ;
#48470=CARTESIAN_POINT('Ctrl Pts',(-30.0346497140305,-14.8413880179389,
-47.1495583377523)) ;
#48471=CARTESIAN_POINT('Ctrl Pts',(-29.8591705047475,-15.1942784066061,
-46.8802501289145)) ;
#48472=CARTESIAN_POINT('Ctrl Pts',(-29.4579425884064,-15.9582510941262,
-46.5229621057665)) ;
#48473=CARTESIAN_POINT('Ctrl Pts',(-29.2317567915366,-16.369112042562,-46.435)) ;
#48474=CARTESIAN_POINT('Ctrl Pts',(-28.7919452620208,-17.130887957438,-46.435)) ;
#48475=CARTESIAN_POINT('Ctrl Pts',(-28.5492221416873,-17.5322010777203,
-46.5229621057665)) ;
#48476=CARTESIAN_POINT('Ctrl Pts',(-28.088216344668,-18.2616609897393,-46.8802501289145)) ;
#48477=CARTESIAN_POINT('Ctrl Pts',(-27.8703439079724,-18.5900756371479,
-47.1495583377523)) ;
#48478=CARTESIAN_POINT('Ctrl Pts',(-27.5199265959608,-19.1049894709151,
-47.7706954545604)) ;
#48479=CARTESIAN_POINT('Ctrl Pts',(-27.364025659875,-19.3259492202238,-48.1640465487624)) ;
#48480=CARTESIAN_POINT('Ctrl Pts',(-27.1553769624387,-19.6180456661006,
-49.0262784098868)) ;
#48481=CARTESIAN_POINT('Ctrl Pts',(-27.103076092507,-19.6894201622032,-49.4951866852561)) ;
#48482=CARTESIAN_POINT('Ctrl Pts',(-27.103076092507,-19.6894201622032,-50.3748133147439)) ;
#48483=CARTESIAN_POINT('Ctrl Pts',(-27.1553769624387,-19.6180456661006,
-50.8437215901132)) ;
#48484=CARTESIAN_POINT('Ctrl Pts',(-27.364025659875,-19.3259492202238,-51.7059534512376)) ;
#48485=CARTESIAN_POINT('Ctrl Pts',(-27.5199265959608,-19.1049894709151,
-52.0993045454395)) ;
#48486=CARTESIAN_POINT('Ctrl Pts',(-27.8703439079724,-18.5900756371479,
-52.7204416622477)) ;
#48487=CARTESIAN_POINT('Ctrl Pts',(-28.088216344668,-18.2616609897393,-52.9897498710855)) ;
#48488=CARTESIAN_POINT('Ctrl Pts',(-28.5492221416873,-17.5322010777203,
-53.3470378942334)) ;
#48489=CARTESIAN_POINT('Ctrl Pts',(-28.7919452620208,-17.130887957438,-53.435)) ;
#48490=CARTESIAN_POINT('Ctrl Pts',(-29.2317567915366,-16.369112042562,-53.435)) ;
#48491=CARTESIAN_POINT('Ctrl Pts',(-29.4579425884064,-15.9582510941262,
-53.3470378942334)) ;
#48492=CARTESIAN_POINT('Ctrl Pts',(-29.8591705047475,-15.1942784066061,
-52.9897498710855)) ;
#48493=CARTESIAN_POINT('Ctrl Pts',(-30.0346497140305,-14.8413880179389,
-52.7204416622477)) ;
#48494=CARTESIAN_POINT('Ctrl Pts',(-30.3053695188271,-14.2804608069275,
-52.0993045454395)) ;
#48495=CARTESIAN_POINT('Ctrl Pts',(-30.4187758068994,-14.034966761149,-51.7059534512376)) ;
#48496=CARTESIAN_POINT('Ctrl Pts',(-30.5674144006656,-13.7082234657643,
-50.8437215901132)) ;
#48497=CARTESIAN_POINT('Ctrl Pts',(-30.603076092507,-13.6272423357121,-50.3748133147439)) ;
#48498=CARTESIAN_POINT('Ctrl Pts',(-30.603076092507,-13.6272423357121,-49.935)) ;
#48499=CARTESIAN_POINT('',(3.5,33.3166624979154,-49.935)) ;
#48500=CARTESIAN_POINT('Ctrl Pts',(3.5,33.3166624979154,-49.935)) ;
#48501=CARTESIAN_POINT('Ctrl Pts',(3.5,33.3166624979154,-49.4951866852561)) ;
#48502=CARTESIAN_POINT('Ctrl Pts',(3.41203743822697,33.3262691318649,-49.0262784098868)) ;
#48503=CARTESIAN_POINT('Ctrl Pts',(3.05475014702442,33.3609159813728,-48.1640465487623)) ;
#48504=CARTESIAN_POINT('Ctrl Pts',(2.7854429228663,33.3854502778426,-47.7706954545604)) ;
#48505=CARTESIAN_POINT('Ctrl Pts',(2.16430580605813,33.4314636550869,-47.1495583377523)) ;
#48506=CARTESIAN_POINT('Ctrl Pts',(1.77095416007957,33.4559393963454,-46.8802501289145)) ;
#48507=CARTESIAN_POINT('Ctrl Pts',(0.908720446719096,33.4904521718465,-46.5229621057665)) ;
#48508=CARTESIAN_POINT('Ctrl Pts',(0.439811529515813,33.5,-46.435)) ;
#48509=CARTESIAN_POINT('Ctrl Pts',(-0.439811529515812,33.5,-46.435)) ;
#48510=CARTESIAN_POINT('Ctrl Pts',(-0.908720446719095,33.4904521718465,
-46.5229621057665)) ;
#48511=CARTESIAN_POINT('Ctrl Pts',(-1.77095416007956,33.4559393963454,-46.8802501289145)) ;
#48512=CARTESIAN_POINT('Ctrl Pts',(-2.16430580605813,33.4314636550869,-47.1495583377523)) ;
#48513=CARTESIAN_POINT('Ctrl Pts',(-2.7854429228663,33.3854502778426,-47.7706954545604)) ;
#48514=CARTESIAN_POINT('Ctrl Pts',(-3.05475014702442,33.3609159813728,-48.1640465487623)) ;
#48515=CARTESIAN_POINT('Ctrl Pts',(-3.41203743822697,33.3262691318649,-49.0262784098868)) ;
#48516=CARTESIAN_POINT('Ctrl Pts',(-3.5,33.3166624979154,-49.4951866852561)) ;
#48517=CARTESIAN_POINT('Ctrl Pts',(-3.5,33.3166624979154,-50.3748133147439)) ;
#48518=CARTESIAN_POINT('Ctrl Pts',(-3.41203743822697,33.3262691318649,-50.8437215901132)) ;
#48519=CARTESIAN_POINT('Ctrl Pts',(-3.05475014702442,33.3609159813728,-51.7059534512376)) ;
#48520=CARTESIAN_POINT('Ctrl Pts',(-2.7854429228663,33.3854502778426,-52.0993045454395)) ;
#48521=CARTESIAN_POINT('Ctrl Pts',(-2.16430580605813,33.4314636550869,-52.7204416622477)) ;
#48522=CARTESIAN_POINT('Ctrl Pts',(-1.77095416007956,33.4559393963454,-52.9897498710854)) ;
#48523=CARTESIAN_POINT('Ctrl Pts',(-0.908720446719096,33.4904521718465,
-53.3470378942334)) ;
#48524=CARTESIAN_POINT('Ctrl Pts',(-0.439811529515812,33.5,-53.435)) ;
#48525=CARTESIAN_POINT('Ctrl Pts',(0.439811529515812,33.5,-53.435)) ;
#48526=CARTESIAN_POINT('Ctrl Pts',(0.908720446719096,33.4904521718465,-53.3470378942334)) ;
#48527=CARTESIAN_POINT('Ctrl Pts',(1.77095416007957,33.4559393963454,-52.9897498710854)) ;
#48528=CARTESIAN_POINT('Ctrl Pts',(2.16430580605813,33.4314636550869,-52.7204416622477)) ;
#48529=CARTESIAN_POINT('Ctrl Pts',(2.7854429228663,33.3854502778426,-52.0993045454395)) ;
#48530=CARTESIAN_POINT('Ctrl Pts',(3.05475014702442,33.3609159813728,-51.7059534512376)) ;
#48531=CARTESIAN_POINT('Ctrl Pts',(3.41203743822697,33.3262691318649,-50.8437215901132)) ;
#48532=CARTESIAN_POINT('Ctrl Pts',(3.5,33.3166624979154,-50.3748133147439)) ;
#48533=CARTESIAN_POINT('Ctrl Pts',(3.5,33.3166624979154,-49.935)) ;
#48534=CARTESIAN_POINT('Origin',(0.,22.5,-56.)) ;
#48535=CARTESIAN_POINT('',(-2.75545529808154E-15,-22.5,-56.)) ;
#48536=CARTESIAN_POINT('Origin',(0.,0.,-56.)) ;
#48537=CARTESIAN_POINT('Origin',(0.,0.,-43.995)) ;
#48538=CARTESIAN_POINT('',(4.07195060716495E-15,33.25,-43.87)) ;
#48539=CARTESIAN_POINT('',(4.08725869215429E-15,33.375,-43.995)) ;
#48540=CARTESIAN_POINT('Origin',(0.,0.,-43.87)) ;
#48541=CARTESIAN_POINT('Origin',(0.,33.5,-43.87)) ;
#48542=CARTESIAN_POINT('',(-2.45725380248917E-15,-20.065,-43.87)) ;
#48543=CARTESIAN_POINT('Origin',(0.,0.,-43.87)) ;
#48544=CARTESIAN_POINT('Ctrl Pts',(27.103076092507,-19.6894201622032,-49.935)) ;
#48545=CARTESIAN_POINT('Ctrl Pts',(18.4427076638945,-14.6893541186624,-49.935)) ;
#48546=CARTESIAN_POINT('Ctrl Pts',(27.103076092507,-19.6894201622032,-49.4951866852561)) ;
#48547=CARTESIAN_POINT('Ctrl Pts',(18.4427076638945,-14.6893541186624,-49.4951866852561)) ;
#48548=CARTESIAN_POINT('Ctrl Pts',(27.1553769624387,-19.6180456661006,-49.0262784098868)) ;
#48549=CARTESIAN_POINT('Ctrl Pts',(18.4950085338262,-14.6179796225598,-49.0262784098868)) ;
#48550=CARTESIAN_POINT('Ctrl Pts',(27.3640256598749,-19.3259492202238,-48.1640465487623)) ;
#48551=CARTESIAN_POINT('Ctrl Pts',(18.7036572312625,-14.325883176683,-48.1640465487623)) ;
#48552=CARTESIAN_POINT('Ctrl Pts',(27.5199265959608,-19.1049894709151,-47.7706954545604)) ;
#48553=CARTESIAN_POINT('Ctrl Pts',(18.8595581673483,-14.1049234273743,-47.7706954545604)) ;
#48554=CARTESIAN_POINT('Ctrl Pts',(27.8703439079723,-18.590075637148,-47.1495583377523)) ;
#48555=CARTESIAN_POINT('Ctrl Pts',(19.2099754793599,-13.5900095936072,-47.1495583377523)) ;
#48556=CARTESIAN_POINT('Ctrl Pts',(28.088216344668,-18.2616609897394,-46.8802501289145)) ;
#48557=CARTESIAN_POINT('Ctrl Pts',(19.4278479160555,-13.2615949461985,-46.8802501289145)) ;
#48558=CARTESIAN_POINT('Ctrl Pts',(28.5492221416872,-17.5322010777203,-46.5229621057665)) ;
#48559=CARTESIAN_POINT('Ctrl Pts',(19.8888537130748,-12.5321350341795,-46.5229621057665)) ;
#48560=CARTESIAN_POINT('Ctrl Pts',(28.7919452620208,-17.130887957438,-46.435)) ;
#48561=CARTESIAN_POINT('Ctrl Pts',(20.1315768334083,-12.1308219138972,-46.435)) ;
#48562=CARTESIAN_POINT('Ctrl Pts',(29.2317567915366,-16.369112042562,-46.435)) ;
#48563=CARTESIAN_POINT('Ctrl Pts',(20.5713883629241,-11.3690459990212,-46.435)) ;
#48564=CARTESIAN_POINT('Ctrl Pts',(29.4579425884063,-15.9582510941262,-46.5229621057665)) ;
#48565=CARTESIAN_POINT('Ctrl Pts',(20.7975741597939,-10.9581850505854,-46.5229621057665)) ;
#48566=CARTESIAN_POINT('Ctrl Pts',(29.8591705047475,-15.1942784066061,-46.8802501289145)) ;
#48567=CARTESIAN_POINT('Ctrl Pts',(21.198802076135,-10.1942123630653,-46.8802501289145)) ;
#48568=CARTESIAN_POINT('Ctrl Pts',(30.0346497140305,-14.841388017939,-47.1495583377523)) ;
#48569=CARTESIAN_POINT('Ctrl Pts',(21.374281285418,-9.84132197439817,-47.1495583377523)) ;
#48570=CARTESIAN_POINT('Ctrl Pts',(30.3053695188271,-14.2804608069275,-47.7706954545604)) ;
#48571=CARTESIAN_POINT('Ctrl Pts',(21.6450010902146,-9.28039476338673,-47.7706954545604)) ;
#48572=CARTESIAN_POINT('Ctrl Pts',(30.4187758068994,-14.034966761149,-48.1640465487623)) ;
#48573=CARTESIAN_POINT('Ctrl Pts',(21.7584073782869,-9.03490071760825,-48.1640465487623)) ;
#48574=CARTESIAN_POINT('Ctrl Pts',(30.5674144006656,-13.7082234657643,-49.0262784098868)) ;
#48575=CARTESIAN_POINT('Ctrl Pts',(21.9070459720532,-8.70815742222352,-49.0262784098868)) ;
#48576=CARTESIAN_POINT('Ctrl Pts',(30.603076092507,-13.6272423357122,-49.4951866852561)) ;
#48577=CARTESIAN_POINT('Ctrl Pts',(21.9427076638945,-8.62717629217136,-49.4951866852561)) ;
#48578=CARTESIAN_POINT('Ctrl Pts',(30.603076092507,-13.6272423357122,-50.3748133147439)) ;
#48579=CARTESIAN_POINT('Ctrl Pts',(21.9427076638945,-8.62717629217136,-50.3748133147439)) ;
#48580=CARTESIAN_POINT('Ctrl Pts',(30.5674144006656,-13.7082234657643,-50.8437215901132)) ;
#48581=CARTESIAN_POINT('Ctrl Pts',(21.9070459720532,-8.70815742222352,-50.8437215901132)) ;
#48582=CARTESIAN_POINT('Ctrl Pts',(30.4187758068994,-14.0349667611491,-51.7059534512376)) ;
#48583=CARTESIAN_POINT('Ctrl Pts',(21.7584073782869,-9.03490071760825,-51.7059534512376)) ;
#48584=CARTESIAN_POINT('Ctrl Pts',(30.3053695188271,-14.2804608069275,-52.0993045454395)) ;
#48585=CARTESIAN_POINT('Ctrl Pts',(21.6450010902146,-9.28039476338673,-52.0993045454395)) ;
#48586=CARTESIAN_POINT('Ctrl Pts',(30.0346497140305,-14.841388017939,-52.7204416622477)) ;
#48587=CARTESIAN_POINT('Ctrl Pts',(21.374281285418,-9.84132197439817,-52.7204416622477)) ;
#48588=CARTESIAN_POINT('Ctrl Pts',(29.8591705047475,-15.1942784066061,-52.9897498710854)) ;
#48589=CARTESIAN_POINT('Ctrl Pts',(21.198802076135,-10.1942123630653,-52.9897498710854)) ;
#48590=CARTESIAN_POINT('Ctrl Pts',(29.4579425884063,-15.9582510941262,-53.3470378942334)) ;
#48591=CARTESIAN_POINT('Ctrl Pts',(20.7975741597939,-10.9581850505854,-53.3470378942334)) ;
#48592=CARTESIAN_POINT('Ctrl Pts',(29.2317567915366,-16.369112042562,-53.435)) ;
#48593=CARTESIAN_POINT('Ctrl Pts',(20.5713883629241,-11.3690459990212,-53.435)) ;
#48594=CARTESIAN_POINT('Ctrl Pts',(28.7919452620208,-17.130887957438,-53.435)) ;
#48595=CARTESIAN_POINT('Ctrl Pts',(20.1315768334083,-12.1308219138972,-53.435)) ;
#48596=CARTESIAN_POINT('Ctrl Pts',(28.5492221416872,-17.5322010777204,-53.3470378942334)) ;
#48597=CARTESIAN_POINT('Ctrl Pts',(19.8888537130748,-12.5321350341795,-53.3470378942334)) ;
#48598=CARTESIAN_POINT('Ctrl Pts',(28.088216344668,-18.2616609897394,-52.9897498710854)) ;
#48599=CARTESIAN_POINT('Ctrl Pts',(19.4278479160555,-13.2615949461986,-52.9897498710854)) ;
#48600=CARTESIAN_POINT('Ctrl Pts',(27.8703439079723,-18.590075637148,-52.7204416622477)) ;
#48601=CARTESIAN_POINT('Ctrl Pts',(19.2099754793599,-13.5900095936072,-52.7204416622477)) ;
#48602=CARTESIAN_POINT('Ctrl Pts',(27.5199265959608,-19.1049894709151,-52.0993045454395)) ;
#48603=CARTESIAN_POINT('Ctrl Pts',(18.8595581673483,-14.1049234273743,-52.0993045454395)) ;
#48604=CARTESIAN_POINT('Ctrl Pts',(27.3640256598749,-19.3259492202238,-51.7059534512376)) ;
#48605=CARTESIAN_POINT('Ctrl Pts',(18.7036572312625,-14.325883176683,-51.7059534512376)) ;
#48606=CARTESIAN_POINT('Ctrl Pts',(27.1553769624387,-19.6180456661006,-50.8437215901132)) ;
#48607=CARTESIAN_POINT('Ctrl Pts',(18.4950085338262,-14.6179796225598,-50.8437215901132)) ;
#48608=CARTESIAN_POINT('Ctrl Pts',(27.103076092507,-19.6894201622032,-50.3748133147439)) ;
#48609=CARTESIAN_POINT('Ctrl Pts',(18.4427076638945,-14.6893541186624,-50.3748133147439)) ;
#48610=CARTESIAN_POINT('Ctrl Pts',(27.103076092507,-19.6894201622032,-49.935)) ;
#48611=CARTESIAN_POINT('Ctrl Pts',(18.4427076638945,-14.6893541186624,-49.935)) ;
#48612=CARTESIAN_POINT('',(18.4427987905013,-14.6894573115498,-49.9350000240614)) ;
#48613=CARTESIAN_POINT('Ctrl Pts',(27.103076092507,-19.6894201622032,-49.935)) ;
#48614=CARTESIAN_POINT('Ctrl Pts',(18.4428206926806,-14.6894193758625,-49.935)) ;
#48615=CARTESIAN_POINT('Ctrl Pts',(18.4427987905013,-14.6894573115498,-49.9350000240614)) ;
#48616=CARTESIAN_POINT('Ctrl Pts',(18.4427531120374,-14.6895275477814,-49.7823947044338)) ;
#48617=CARTESIAN_POINT('Ctrl Pts',(18.44886735586,-14.681117357845,-49.6112134273951)) ;
#48618=CARTESIAN_POINT('Ctrl Pts',(18.4853437963175,-14.6307823444917,-49.1998503646376)) ;
#48619=CARTESIAN_POINT('Ctrl Pts',(18.5175132400749,-14.5863573189043,-48.9745962929381)) ;
#48620=CARTESIAN_POINT('Ctrl Pts',(18.6657603536904,-14.3796102913098,-48.2662983684852)) ;
#48621=CARTESIAN_POINT('Ctrl Pts',(18.819056053797,-14.1621995813133,-47.883172642928)) ;
#48622=CARTESIAN_POINT('Ctrl Pts',(19.1522667831666,-13.6773365162311,-47.2139532467364)) ;
#48623=CARTESIAN_POINT('Ctrl Pts',(19.3750593745531,-13.3405007077791,-46.9533770888002)) ;
#48624=CARTESIAN_POINT('Ctrl Pts',(19.7974436197774,-12.6811571505934,-46.5664922879644)) ;
#48625=CARTESIAN_POINT('Ctrl Pts',(20.0358995829733,-12.2890367087697,-46.4734326225838)) ;
#48626=CARTESIAN_POINT('Ctrl Pts',(20.4843327090169,-11.5262783305788,-46.4045524997322)) ;
#48627=CARTESIAN_POINT('Ctrl Pts',(20.7104180554908,-11.1164311593209,-46.4925278051967)) ;
#48628=CARTESIAN_POINT('Ctrl Pts',(21.108737346578,-10.3719551438664,-46.7651000997357)) ;
#48629=CARTESIAN_POINT('Ctrl Pts',(21.285707958859,-10.0190112984326,-47.0172803610138)) ;
#48630=CARTESIAN_POINT('Ctrl Pts',(21.5947015506035,-9.38960342665918,-47.6023005356928)) ;
#48631=CARTESIAN_POINT('Ctrl Pts',(21.7078493371503,-9.14418273779913,-47.9944593073979)) ;
#48632=CARTESIAN_POINT('Ctrl Pts',(21.8061586042231,-8.93024469048519,-48.4438880038744)) ;
#48633=CARTESIAN_POINT('Ctrl Pts',(21.8303892027021,-8.87707989392543,-48.5725202466068)) ;
#48634=CARTESIAN_POINT('Ctrl Pts',(21.8812156221636,-8.76494580189594,-48.9021343175402)) ;
#48635=CARTESIAN_POINT('Ctrl Pts',(21.9045461994582,-8.71293077313088,-49.1073011631895)) ;
#48636=CARTESIAN_POINT('Ctrl Pts',(21.9350469301527,-8.64473773197279,-49.5238351190534)) ;
#48637=CARTESIAN_POINT('Ctrl Pts',(21.9428220546626,-8.62724233571215,-49.7302427331702)) ;
#48638=CARTESIAN_POINT('Ctrl Pts',(21.9428220546626,-8.62724233571215,-49.9349999999999)) ;
#48639=CARTESIAN_POINT('Ctrl Pts',(21.9428220546626,-8.62724233571214,-50.1455828409762)) ;
#48640=CARTESIAN_POINT('Ctrl Pts',(21.9346003886721,-8.64575634274508,-50.3651730635469)) ;
#48641=CARTESIAN_POINT('Ctrl Pts',(21.8828966189749,-8.76128851199987,-51.0288729348249)) ;
#48642=CARTESIAN_POINT('Ctrl Pts',(21.8146962770843,-8.91397276739595,-51.4570912893389)) ;
#48643=CARTESIAN_POINT('Ctrl Pts',(21.6503326879261,-9.26650739525063,-52.0447545851038)) ;
#48644=CARTESIAN_POINT('Ctrl Pts',(21.5887973035584,-9.39696090923297,-52.2259765012846)) ;
#48645=CARTESIAN_POINT('Ctrl Pts',(21.4513830427457,-9.68202705953242,-52.5458841412737)) ;
#48646=CARTESIAN_POINT('Ctrl Pts',(21.3762106229735,-9.83562627323664,-52.6891786697716)) ;
#48647=CARTESIAN_POINT('Ctrl Pts',(21.2102533734648,-10.1669521283806,-52.9435506339985)) ;
#48648=CARTESIAN_POINT('Ctrl Pts',(21.1181821598937,-10.347396276298,-53.0578107060786)) ;
#48649=CARTESIAN_POINT('Ctrl Pts',(20.9269456889309,-10.712576459322,-53.2347269698551)) ;
#48650=CARTESIAN_POINT('Ctrl Pts',(20.8290550037948,-10.8958458805748,-53.3020383948391)) ;
#48651=CARTESIAN_POINT('Ctrl Pts',(20.6215184026939,-11.2749481451676,-53.3980021942758)) ;
#48652=CARTESIAN_POINT('Ctrl Pts',(20.5100659904938,-11.4741500863567,-53.4280956303302)) ;
#48653=CARTESIAN_POINT('Ctrl Pts',(20.3007086380488,-11.8388564562127,-53.4385899044817)) ;
#48654=CARTESIAN_POINT('Ctrl Pts',(20.1905268829027,-12.0278357833663,-53.4290562483249)) ;
#48655=CARTESIAN_POINT('Ctrl Pts',(19.9467874918082,-12.4337355258641,-53.3497426101656)) ;
#48656=CARTESIAN_POINT('Ctrl Pts',(19.8292512709116,-12.6251940105125,-53.2913599998512)) ;
#48657=CARTESIAN_POINT('Ctrl Pts',(19.6045297561846,-12.983107603713,-53.1317914335173)) ;
#48658=CARTESIAN_POINT('Ctrl Pts',(19.4976150092651,-13.1499610391986,-53.0347656954103)) ;
#48659=CARTESIAN_POINT('Ctrl Pts',(19.2900755252539,-13.4679315770041,-52.8014456739523)) ;
#48660=CARTESIAN_POINT('Ctrl Pts',(19.1872844094319,-13.6224261317564,-52.6636415879439)) ;
#48661=CARTESIAN_POINT('Ctrl Pts',(19.0121283157254,-13.8814349031294,-52.3760206544823)) ;
#48662=CARTESIAN_POINT('Ctrl Pts',(18.9262394436352,-14.0068222128443,-52.2154232168395)) ;
#48663=CARTESIAN_POINT('Ctrl Pts',(18.7059260228408,-14.3234467106669,-51.690363352432)) ;
#48664=CARTESIAN_POINT('Ctrl Pts',(18.5760427442282,-14.5051400890156,-51.2863619910567)) ;
#48665=CARTESIAN_POINT('Ctrl Pts',(18.4709264873325,-14.6507434167168,-50.5442029076166)) ;
#48666=CARTESIAN_POINT('Ctrl Pts',(18.4508136331523,-14.678417533721,-50.3167637435239)) ;
#48667=CARTESIAN_POINT('Ctrl Pts',(18.4435200648678,-14.6884594034969,-50.0351173441296)) ;
#48668=CARTESIAN_POINT('Ctrl Pts',(18.4428140859908,-14.6894337928618,-49.9861001018761)) ;
#48669=CARTESIAN_POINT('Ctrl Pts',(18.4427987905013,-14.6894573115498,-49.9350000240614)) ;
#48670=CARTESIAN_POINT('Origin',(-8.66025403784438,5.,-49.935)) ;
#48671=CARTESIAN_POINT('Ctrl Pts',(-30.603076092507,-13.6272423357121,-49.935)) ;
#48672=CARTESIAN_POINT('Ctrl Pts',(-21.9427076638945,-8.62717629217139,
-49.935)) ;
#48673=CARTESIAN_POINT('Ctrl Pts',(-30.603076092507,-13.6272423357121,-49.4951866852561)) ;
#48674=CARTESIAN_POINT('Ctrl Pts',(-21.9427076638945,-8.62717629217139,
-49.4951866852561)) ;
#48675=CARTESIAN_POINT('Ctrl Pts',(-30.5674144006657,-13.7082234657643,
-49.0262784098868)) ;
#48676=CARTESIAN_POINT('Ctrl Pts',(-21.9070459720532,-8.70815742222356,
-49.0262784098868)) ;
#48677=CARTESIAN_POINT('Ctrl Pts',(-30.4187758068994,-14.034966761149,-48.1640465487624)) ;
#48678=CARTESIAN_POINT('Ctrl Pts',(-21.758407378287,-9.03490071760828,-48.1640465487624)) ;
#48679=CARTESIAN_POINT('Ctrl Pts',(-30.3053695188271,-14.2804608069275,
-47.7706954545604)) ;
#48680=CARTESIAN_POINT('Ctrl Pts',(-21.6450010902146,-9.28039476338676,
-47.7706954545604)) ;
#48681=CARTESIAN_POINT('Ctrl Pts',(-30.0346497140305,-14.8413880179389,
-47.1495583377523)) ;
#48682=CARTESIAN_POINT('Ctrl Pts',(-21.374281285418,-9.8413219743982,-47.1495583377523)) ;
#48683=CARTESIAN_POINT('Ctrl Pts',(-29.8591705047475,-15.1942784066061,
-46.8802501289145)) ;
#48684=CARTESIAN_POINT('Ctrl Pts',(-21.198802076135,-10.1942123630653,-46.8802501289145)) ;
#48685=CARTESIAN_POINT('Ctrl Pts',(-29.4579425884064,-15.9582510941262,
-46.5229621057665)) ;
#48686=CARTESIAN_POINT('Ctrl Pts',(-20.797574159794,-10.9581850505854,-46.5229621057665)) ;
#48687=CARTESIAN_POINT('Ctrl Pts',(-29.2317567915366,-16.369112042562,-46.435)) ;
#48688=CARTESIAN_POINT('Ctrl Pts',(-20.5713883629241,-11.3690459990212,
-46.435)) ;
#48689=CARTESIAN_POINT('Ctrl Pts',(-28.7919452620208,-17.130887957438,-46.435)) ;
#48690=CARTESIAN_POINT('Ctrl Pts',(-20.1315768334083,-12.1308219138972,
-46.435)) ;
#48691=CARTESIAN_POINT('Ctrl Pts',(-28.5492221416873,-17.5322010777203,
-46.5229621057665)) ;
#48692=CARTESIAN_POINT('Ctrl Pts',(-19.8888537130748,-12.5321350341795,
-46.5229621057665)) ;
#48693=CARTESIAN_POINT('Ctrl Pts',(-28.088216344668,-18.2616609897393,-46.8802501289145)) ;
#48694=CARTESIAN_POINT('Ctrl Pts',(-19.4278479160555,-13.2615949461985,
-46.8802501289145)) ;
#48695=CARTESIAN_POINT('Ctrl Pts',(-27.8703439079724,-18.5900756371479,
-47.1495583377523)) ;
#48696=CARTESIAN_POINT('Ctrl Pts',(-19.2099754793599,-13.5900095936071,
-47.1495583377523)) ;
#48697=CARTESIAN_POINT('Ctrl Pts',(-27.5199265959608,-19.1049894709151,
-47.7706954545604)) ;
#48698=CARTESIAN_POINT('Ctrl Pts',(-18.8595581673484,-14.1049234273743,
-47.7706954545604)) ;
#48699=CARTESIAN_POINT('Ctrl Pts',(-27.364025659875,-19.3259492202238,-48.1640465487624)) ;
#48700=CARTESIAN_POINT('Ctrl Pts',(-18.7036572312625,-14.325883176683,-48.1640465487624)) ;
#48701=CARTESIAN_POINT('Ctrl Pts',(-27.1553769624387,-19.6180456661006,
-49.0262784098868)) ;
#48702=CARTESIAN_POINT('Ctrl Pts',(-18.4950085338262,-14.6179796225598,
-49.0262784098868)) ;
#48703=CARTESIAN_POINT('Ctrl Pts',(-27.103076092507,-19.6894201622032,-49.4951866852561)) ;
#48704=CARTESIAN_POINT('Ctrl Pts',(-18.4427076638945,-14.6893541186624,
-49.4951866852561)) ;
#48705=CARTESIAN_POINT('Ctrl Pts',(-27.103076092507,-19.6894201622032,-50.3748133147439)) ;
#48706=CARTESIAN_POINT('Ctrl Pts',(-18.4427076638945,-14.6893541186624,
-50.3748133147439)) ;
#48707=CARTESIAN_POINT('Ctrl Pts',(-27.1553769624387,-19.6180456661006,
-50.8437215901132)) ;
#48708=CARTESIAN_POINT('Ctrl Pts',(-18.4950085338262,-14.6179796225598,
-50.8437215901132)) ;
#48709=CARTESIAN_POINT('Ctrl Pts',(-27.364025659875,-19.3259492202238,-51.7059534512376)) ;
#48710=CARTESIAN_POINT('Ctrl Pts',(-18.7036572312625,-14.325883176683,-51.7059534512376)) ;
#48711=CARTESIAN_POINT('Ctrl Pts',(-27.5199265959608,-19.1049894709151,
-52.0993045454395)) ;
#48712=CARTESIAN_POINT('Ctrl Pts',(-18.8595581673484,-14.1049234273743,
-52.0993045454395)) ;
#48713=CARTESIAN_POINT('Ctrl Pts',(-27.8703439079724,-18.5900756371479,
-52.7204416622477)) ;
#48714=CARTESIAN_POINT('Ctrl Pts',(-19.2099754793599,-13.5900095936072,
-52.7204416622477)) ;
#48715=CARTESIAN_POINT('Ctrl Pts',(-28.088216344668,-18.2616609897393,-52.9897498710855)) ;
#48716=CARTESIAN_POINT('Ctrl Pts',(-19.4278479160555,-13.2615949461985,
-52.9897498710855)) ;
#48717=CARTESIAN_POINT('Ctrl Pts',(-28.5492221416873,-17.5322010777203,
-53.3470378942334)) ;
#48718=CARTESIAN_POINT('Ctrl Pts',(-19.8888537130748,-12.5321350341795,
-53.3470378942334)) ;
#48719=CARTESIAN_POINT('Ctrl Pts',(-28.7919452620208,-17.130887957438,-53.435)) ;
#48720=CARTESIAN_POINT('Ctrl Pts',(-20.1315768334083,-12.1308219138972,
-53.435)) ;
#48721=CARTESIAN_POINT('Ctrl Pts',(-29.2317567915366,-16.369112042562,-53.435)) ;
#48722=CARTESIAN_POINT('Ctrl Pts',(-20.5713883629241,-11.3690459990212,
-53.435)) ;
#48723=CARTESIAN_POINT('Ctrl Pts',(-29.4579425884064,-15.9582510941262,
-53.3470378942334)) ;
#48724=CARTESIAN_POINT('Ctrl Pts',(-20.797574159794,-10.9581850505854,-53.3470378942334)) ;
#48725=CARTESIAN_POINT('Ctrl Pts',(-29.8591705047475,-15.1942784066061,
-52.9897498710855)) ;
#48726=CARTESIAN_POINT('Ctrl Pts',(-21.198802076135,-10.1942123630653,-52.9897498710855)) ;
#48727=CARTESIAN_POINT('Ctrl Pts',(-30.0346497140305,-14.8413880179389,
-52.7204416622477)) ;
#48728=CARTESIAN_POINT('Ctrl Pts',(-21.374281285418,-9.8413219743982,-52.7204416622477)) ;
#48729=CARTESIAN_POINT('Ctrl Pts',(-30.3053695188271,-14.2804608069275,
-52.0993045454395)) ;
#48730=CARTESIAN_POINT('Ctrl Pts',(-21.6450010902146,-9.28039476338676,
-52.0993045454395)) ;
#48731=CARTESIAN_POINT('Ctrl Pts',(-30.4187758068994,-14.034966761149,-51.7059534512376)) ;
#48732=CARTESIAN_POINT('Ctrl Pts',(-21.758407378287,-9.03490071760827,-51.7059534512376)) ;
#48733=CARTESIAN_POINT('Ctrl Pts',(-30.5674144006656,-13.7082234657643,
-50.8437215901132)) ;
#48734=CARTESIAN_POINT('Ctrl Pts',(-21.9070459720532,-8.70815742222355,
-50.8437215901132)) ;
#48735=CARTESIAN_POINT('Ctrl Pts',(-30.603076092507,-13.6272423357121,-50.3748133147439)) ;
#48736=CARTESIAN_POINT('Ctrl Pts',(-21.9427076638945,-8.62717629217139,
-50.3748133147439)) ;
#48737=CARTESIAN_POINT('Ctrl Pts',(-30.603076092507,-13.6272423357121,-49.935)) ;
#48738=CARTESIAN_POINT('Ctrl Pts',(-21.9427076638945,-8.62717629217139,
-49.935)) ;
#48739=CARTESIAN_POINT('',(-21.9428425948598,-8.62720361368415,-49.9350000240614)) ;
#48740=CARTESIAN_POINT('Ctrl Pts',(-30.603076092507,-13.6272423357121,-49.935)) ;
#48741=CARTESIAN_POINT('Ctrl Pts',(-21.9428206926805,-8.62724154937146,
-49.935)) ;
#48742=CARTESIAN_POINT('Ctrl Pts',(-21.9428425948598,-8.62720361368415,
-49.9350000240614)) ;
#48743=CARTESIAN_POINT('Ctrl Pts',(-21.9428805819887,-8.62712893685822,
-49.7823947044339)) ;
#48744=CARTESIAN_POINT('Ctrl Pts',(-21.9386542657645,-8.6366291223017,-49.6112134273954)) ;
#48745=CARTESIAN_POINT('Ctrl Pts',(-21.9133010857295,-8.69338615305404,
-49.1998503646382)) ;
#48746=CARTESIAN_POINT('Ctrl Pts',(-21.8909126068857,-8.74345822136723,
-48.9745962929387)) ;
#48747=CARTESIAN_POINT('Ctrl Pts',(-21.7859879856397,-8.97521750159318,
-48.2662983684853)) ;
#48748=CARTESIAN_POINT('Ctrl Pts',(-21.6743526377812,-9.21668082717488,
-47.883172642928)) ;
#48749=CARTESIAN_POINT('Ctrl Pts',(-21.4210542707481,-9.74768131616324,
-47.2139532467367)) ;
#48750=CARTESIAN_POINT('Ctrl Pts',(-21.2407421994177,-10.109043264305,-46.9533770888004)) ;
#48751=CARTESIAN_POINT('Ctrl Pts',(-20.8809260516853,-10.8045105294205,
-46.5664922879644)) ;
#48752=CARTESIAN_POINT('Ctrl Pts',(-20.6605677693207,-11.207079672144,-46.4734326225838)) ;
#48753=CARTESIAN_POINT('Ctrl Pts',(-20.22421619988,-11.9768133402915,-46.4045524997322)) ;
#48754=CARTESIAN_POINT('Ctrl Pts',(-19.9823208111384,-12.3775325793903,
-46.4925278051966)) ;
#48755=CARTESIAN_POINT('Ctrl Pts',(-19.53674531479,-13.0947252120165,-46.7651000997356)) ;
#48756=CARTESIAN_POINT('Ctrl Pts',(-19.3195722846755,-13.4244581806921,
-47.0172803610137)) ;
#48757=CARTESIAN_POINT('Ctrl Pts',(-18.92898587425,-14.0067584166363,-47.6023005356929)) ;
#48758=CARTESIAN_POINT('Ctrl Pts',(-18.7730192163563,-14.2274576185978,
-47.994459307398)) ;
#48759=CARTESIAN_POINT('Ctrl Pts',(-18.6368980660828,-14.4195649649672,
-48.4438880038746)) ;
#48760=CARTESIAN_POINT('Ctrl Pts',(-18.6029713009145,-14.4671316770788,
-48.5725202466069)) ;
#48761=CARTESIAN_POINT('Ctrl Pts',(-18.5312735383174,-14.5672156935307,
-48.9021343175404)) ;
#48762=CARTESIAN_POINT('Ctrl Pts',(-18.4978924906756,-14.6134280805353,
-49.1073011631897)) ;
#48763=CARTESIAN_POINT('Ctrl Pts',(-18.4540859500186,-14.6739390087297,
-49.5238351190534)) ;
#48764=CARTESIAN_POINT('Ctrl Pts',(-18.4428220546626,-14.6894201622032,
-49.7302427331703)) ;
#48765=CARTESIAN_POINT('Ctrl Pts',(-18.4428220546626,-14.6894201622032,
-49.935)) ;
#48766=CARTESIAN_POINT('Ctrl Pts',(-18.4428220546626,-14.6894201622032,
-50.1455828409762)) ;
#48767=CARTESIAN_POINT('Ctrl Pts',(-18.4547448220837,-14.6730429870775,
-50.3651730635468)) ;
#48768=CARTESIAN_POINT('Ctrl Pts',(-18.5289467307641,-14.570500124421,-51.0288729348248)) ;
#48769=CARTESIAN_POINT('Ctrl Pts',(-18.6270750037497,-14.4350947680988,
-51.4570912893389)) ;
#48770=CARTESIAN_POINT('Ctrl Pts',(-18.8501971526065,-14.1164844105032,
-52.0447545851039)) ;
#48771=CARTESIAN_POINT('Ctrl Pts',(-18.9324055175443,-13.997966447418,-52.2259765012847)) ;
#48772=CARTESIAN_POINT('Ctrl Pts',(-19.1105729150563,-13.7364291315622,
-52.5458841412738)) ;
#48773=CARTESIAN_POINT('Ctrl Pts',(-19.2060075262394,-13.5945282995234,
-52.6891786697718)) ;
#48774=CARTESIAN_POINT('Ctrl Pts',(-19.4099655089703,-13.2851421779347,
-52.9435506339987)) ;
#48775=CARTESIAN_POINT('Ctrl Pts',(-19.5201991182455,-13.1151840940661,
-53.0578107060788)) ;
#48776=CARTESIAN_POINT('Ctrl Pts',(-19.7408361982214,-12.7669783605705,
-53.234726969855)) ;
#48777=CARTESIAN_POINT('Ctrl Pts',(-19.850606830195,-12.5905678298225,-53.302038394839)) ;
#48778=CARTESIAN_POINT('Ctrl Pts',(-20.075150721414,-12.2212847287579,-53.3980021942757)) ;
#48779=CARTESIAN_POINT('Ctrl Pts',(-20.1919384568669,-12.025163137885,-53.4280956303302)) ;
#48780=CARTESIAN_POINT('Ctrl Pts',(-20.4031047618617,-11.6615011672705,
-53.4385899044817)) ;
#48781=CARTESIAN_POINT('Ctrl Pts',(-20.5116747823938,-11.4715913047036,
-53.4290562483249)) ;
#48782=CARTESIAN_POINT('Ctrl Pts',(-20.7413245752393,-11.0575569288639,
-53.3497426101657)) ;
#48783=CARTESIAN_POINT('Ctrl Pts',(-20.8483643762666,-10.8600383333785,
-53.2913599998514)) ;
#48784=CARTESIAN_POINT('Ctrl Pts',(-21.0459658829745,-10.4864669962478,
-53.1317914335176)) ;
#48785=CARTESIAN_POINT('Ctrl Pts',(-21.1370078233539,-10.3104493916336,
-53.0347656954107)) ;
#48786=CARTESIAN_POINT('Ctrl Pts',(-21.3086086447428,-9.97172965728879,
-52.8014456739528)) ;
#48787=CARTESIAN_POINT('Ctrl Pts',(-21.3910092959937,-9.80546266232745,
-52.6636415879444)) ;
#48788=CARTESIAN_POINT('Ctrl Pts',(-21.5277394249525,-9.52426864986341,
-52.3760206544828)) ;
#48789=CARTESIAN_POINT('Ctrl Pts',(-21.5933835844328,-9.38719304987331,
-52.2154232168399)) ;
#48790=CARTESIAN_POINT('Ctrl Pts',(-21.7574317326105,-9.03808378175918,
-51.6903633524324)) ;
#48791=CARTESIAN_POINT('Ctrl Pts',(-21.8498411746536,-8.83475487377964,
-51.2863619910574)) ;
#48792=CARTESIAN_POINT('Ctrl Pts',(-21.9233792268706,-8.67091986110646,
-50.5442029076174)) ;
#48793=CARTESIAN_POINT('Ctrl Pts',(-21.9372892881334,-8.63966455994172,
-50.3167637435247)) ;
#48794=CARTESIAN_POINT('Ctrl Pts',(-21.9423390183187,-8.62832720963509,
-50.0351173441301)) ;
#48795=CARTESIAN_POINT('Ctrl Pts',(-21.9428298748233,-8.62722861931059,
-49.9861001018763)) ;
#48796=CARTESIAN_POINT('Ctrl Pts',(-21.9428425948598,-8.62720361368415,
-49.9350000240614)) ;
#48797=CARTESIAN_POINT('Origin',(8.66025403784439,5.,-49.935)) ;
#48798=CARTESIAN_POINT('Ctrl Pts',(3.5,33.3166624979154,-49.935)) ;
#48799=CARTESIAN_POINT('Ctrl Pts',(3.5,23.3165304108338,-49.935)) ;
#48800=CARTESIAN_POINT('Ctrl Pts',(3.5,33.3166624979154,-49.4951866852561)) ;
#48801=CARTESIAN_POINT('Ctrl Pts',(3.5,23.3165304108338,-49.4951866852561)) ;
#48802=CARTESIAN_POINT('Ctrl Pts',(3.41203743822697,33.3262691318649,-49.0262784098868)) ;
#48803=CARTESIAN_POINT('Ctrl Pts',(3.41203743822697,23.3261370447833,-49.0262784098868)) ;
#48804=CARTESIAN_POINT('Ctrl Pts',(3.05475014702442,33.3609159813728,-48.1640465487623)) ;
#48805=CARTESIAN_POINT('Ctrl Pts',(3.05475014702442,23.3607838942912,-48.1640465487623)) ;
#48806=CARTESIAN_POINT('Ctrl Pts',(2.7854429228663,33.3854502778426,-47.7706954545604)) ;
#48807=CARTESIAN_POINT('Ctrl Pts',(2.7854429228663,23.385318190761,-47.7706954545604)) ;
#48808=CARTESIAN_POINT('Ctrl Pts',(2.16430580605813,33.4314636550869,-47.1495583377523)) ;
#48809=CARTESIAN_POINT('Ctrl Pts',(2.16430580605813,23.4313315680053,-47.1495583377523)) ;
#48810=CARTESIAN_POINT('Ctrl Pts',(1.77095416007957,33.4559393963454,-46.8802501289145)) ;
#48811=CARTESIAN_POINT('Ctrl Pts',(1.77095416007957,23.4558073092638,-46.8802501289145)) ;
#48812=CARTESIAN_POINT('Ctrl Pts',(0.908720446719096,33.4904521718465,-46.5229621057665)) ;
#48813=CARTESIAN_POINT('Ctrl Pts',(0.908720446719096,23.4903200847649,-46.5229621057665)) ;
#48814=CARTESIAN_POINT('Ctrl Pts',(0.439811529515813,33.5,-46.435)) ;
#48815=CARTESIAN_POINT('Ctrl Pts',(0.439811529515813,23.4998679129184,-46.435)) ;
#48816=CARTESIAN_POINT('Ctrl Pts',(-0.439811529515812,33.5,-46.435)) ;
#48817=CARTESIAN_POINT('Ctrl Pts',(-0.439811529515812,23.4998679129184,
-46.435)) ;
#48818=CARTESIAN_POINT('Ctrl Pts',(-0.908720446719095,33.4904521718465,
-46.5229621057665)) ;
#48819=CARTESIAN_POINT('Ctrl Pts',(-0.908720446719095,23.4903200847649,
-46.5229621057665)) ;
#48820=CARTESIAN_POINT('Ctrl Pts',(-1.77095416007956,33.4559393963454,-46.8802501289145)) ;
#48821=CARTESIAN_POINT('Ctrl Pts',(-1.77095416007956,23.4558073092638,-46.8802501289145)) ;
#48822=CARTESIAN_POINT('Ctrl Pts',(-2.16430580605813,33.4314636550869,-47.1495583377523)) ;
#48823=CARTESIAN_POINT('Ctrl Pts',(-2.16430580605813,23.4313315680053,-47.1495583377523)) ;
#48824=CARTESIAN_POINT('Ctrl Pts',(-2.7854429228663,33.3854502778426,-47.7706954545604)) ;
#48825=CARTESIAN_POINT('Ctrl Pts',(-2.7854429228663,23.385318190761,-47.7706954545604)) ;
#48826=CARTESIAN_POINT('Ctrl Pts',(-3.05475014702442,33.3609159813728,-48.1640465487623)) ;
#48827=CARTESIAN_POINT('Ctrl Pts',(-3.05475014702442,23.3607838942912,-48.1640465487623)) ;
#48828=CARTESIAN_POINT('Ctrl Pts',(-3.41203743822697,33.3262691318649,-49.0262784098868)) ;
#48829=CARTESIAN_POINT('Ctrl Pts',(-3.41203743822697,23.3261370447833,-49.0262784098868)) ;
#48830=CARTESIAN_POINT('Ctrl Pts',(-3.5,33.3166624979154,-49.4951866852561)) ;
#48831=CARTESIAN_POINT('Ctrl Pts',(-3.5,23.3165304108338,-49.4951866852561)) ;
#48832=CARTESIAN_POINT('Ctrl Pts',(-3.5,33.3166624979154,-50.3748133147439)) ;
#48833=CARTESIAN_POINT('Ctrl Pts',(-3.5,23.3165304108338,-50.3748133147439)) ;
#48834=CARTESIAN_POINT('Ctrl Pts',(-3.41203743822697,33.3262691318649,-50.8437215901132)) ;
#48835=CARTESIAN_POINT('Ctrl Pts',(-3.41203743822697,23.3261370447833,-50.8437215901132)) ;
#48836=CARTESIAN_POINT('Ctrl Pts',(-3.05475014702442,33.3609159813728,-51.7059534512376)) ;
#48837=CARTESIAN_POINT('Ctrl Pts',(-3.05475014702442,23.3607838942912,-51.7059534512376)) ;
#48838=CARTESIAN_POINT('Ctrl Pts',(-2.7854429228663,33.3854502778426,-52.0993045454395)) ;
#48839=CARTESIAN_POINT('Ctrl Pts',(-2.7854429228663,23.385318190761,-52.0993045454395)) ;
#48840=CARTESIAN_POINT('Ctrl Pts',(-2.16430580605813,33.4314636550869,-52.7204416622477)) ;
#48841=CARTESIAN_POINT('Ctrl Pts',(-2.16430580605813,23.4313315680053,-52.7204416622477)) ;
#48842=CARTESIAN_POINT('Ctrl Pts',(-1.77095416007956,33.4559393963454,-52.9897498710854)) ;
#48843=CARTESIAN_POINT('Ctrl Pts',(-1.77095416007956,23.4558073092638,-52.9897498710854)) ;
#48844=CARTESIAN_POINT('Ctrl Pts',(-0.908720446719096,33.4904521718465,
-53.3470378942334)) ;
#48845=CARTESIAN_POINT('Ctrl Pts',(-0.908720446719096,23.4903200847649,
-53.3470378942334)) ;
#48846=CARTESIAN_POINT('Ctrl Pts',(-0.439811529515812,33.5,-53.435)) ;
#48847=CARTESIAN_POINT('Ctrl Pts',(-0.439811529515812,23.4998679129184,
-53.435)) ;
#48848=CARTESIAN_POINT('Ctrl Pts',(0.439811529515812,33.5,-53.435)) ;
#48849=CARTESIAN_POINT('Ctrl Pts',(0.439811529515812,23.4998679129184,-53.435)) ;
#48850=CARTESIAN_POINT('Ctrl Pts',(0.908720446719096,33.4904521718465,-53.3470378942334)) ;
#48851=CARTESIAN_POINT('Ctrl Pts',(0.908720446719096,23.4903200847649,-53.3470378942334)) ;
#48852=CARTESIAN_POINT('Ctrl Pts',(1.77095416007957,33.4559393963454,-52.9897498710854)) ;
#48853=CARTESIAN_POINT('Ctrl Pts',(1.77095416007957,23.4558073092638,-52.9897498710854)) ;
#48854=CARTESIAN_POINT('Ctrl Pts',(2.16430580605813,33.4314636550869,-52.7204416622477)) ;
#48855=CARTESIAN_POINT('Ctrl Pts',(2.16430580605813,23.4313315680053,-52.7204416622477)) ;
#48856=CARTESIAN_POINT('Ctrl Pts',(2.7854429228663,33.3854502778426,-52.0993045454395)) ;
#48857=CARTESIAN_POINT('Ctrl Pts',(2.7854429228663,23.385318190761,-52.0993045454395)) ;
#48858=CARTESIAN_POINT('Ctrl Pts',(3.05475014702442,33.3609159813728,-51.7059534512376)) ;
#48859=CARTESIAN_POINT('Ctrl Pts',(3.05475014702442,23.3607838942912,-51.7059534512376)) ;
#48860=CARTESIAN_POINT('Ctrl Pts',(3.41203743822697,33.3262691318649,-50.8437215901132)) ;
#48861=CARTESIAN_POINT('Ctrl Pts',(3.41203743822697,23.3261370447833,-50.8437215901132)) ;
#48862=CARTESIAN_POINT('Ctrl Pts',(3.5,33.3166624979154,-50.3748133147439)) ;
#48863=CARTESIAN_POINT('Ctrl Pts',(3.5,23.3165304108338,-50.3748133147439)) ;
#48864=CARTESIAN_POINT('Ctrl Pts',(3.5,33.3166624979154,-49.935)) ;
#48865=CARTESIAN_POINT('Ctrl Pts',(3.5,23.3165304108338,-49.935)) ;
#48866=CARTESIAN_POINT('',(3.50004380435856,23.3166609252339,-49.9350000240614)) ;
#48867=CARTESIAN_POINT('Ctrl Pts',(3.5,33.3166624979154,-49.935)) ;
#48868=CARTESIAN_POINT('Ctrl Pts',(3.5,23.3166609252339,-49.935)) ;
#48869=CARTESIAN_POINT('Ctrl Pts',(3.50004380435856,23.3166609252339,-49.9350000240614)) ;
#48870=CARTESIAN_POINT('Ctrl Pts',(3.50012746995133,23.3166564846396,-49.7823947044339)) ;
#48871=CARTESIAN_POINT('Ctrl Pts',(3.4897869099045,23.3177464801467,-49.6112134273953)) ;
#48872=CARTESIAN_POINT('Ctrl Pts',(3.42795728941205,23.3241684975459,-49.199850364638)) ;
#48873=CARTESIAN_POINT('Ctrl Pts',(3.37339936681084,23.3298155402716,-48.9745962929384)) ;
#48874=CARTESIAN_POINT('Ctrl Pts',(3.12022763194928,23.3548277929032,-48.266298368485)) ;
#48875=CARTESIAN_POINT('Ctrl Pts',(2.85529658398398,23.3788804084882,-47.8831726429277)) ;
#48876=CARTESIAN_POINT('Ctrl Pts',(2.26878748758131,23.4250178323947,-47.2139532467363)) ;
#48877=CARTESIAN_POINT('Ctrl Pts',(1.86568282486425,23.4495439720844,-46.9533770888)) ;
#48878=CARTESIAN_POINT('Ctrl Pts',(1.08348243190786,23.4856676800141,-46.5664922879645)) ;
#48879=CARTESIAN_POINT('Ctrl Pts',(0.624668186347566,23.4961163809137,-46.4734326225838)) ;
#48880=CARTESIAN_POINT('Ctrl Pts',(-0.260116509136987,23.5030916708706,
-46.4045524997322)) ;
#48881=CARTESIAN_POINT('Ctrl Pts',(-0.728097244352491,23.4939637387114,
-46.4925278051967)) ;
#48882=CARTESIAN_POINT('Ctrl Pts',(-1.57199203178796,23.466680355883,-46.7651000997356)) ;
#48883=CARTESIAN_POINT('Ctrl Pts',(-1.96613567418351,23.4434694791248,-47.0172803610138)) ;
#48884=CARTESIAN_POINT('Ctrl Pts',(-2.66571567635337,23.3963618432954,-47.6023005356928)) ;
#48885=CARTESIAN_POINT('Ctrl Pts',(-2.9348301207939,23.3716403563969,-47.9944593073978)) ;
#48886=CARTESIAN_POINT('Ctrl Pts',(-3.16926053814024,23.3498096554524,-48.4438880038744)) ;
#48887=CARTESIAN_POINT('Ctrl Pts',(-3.22741790178752,23.3442115710042,-48.5725202466068)) ;
#48888=CARTESIAN_POINT('Ctrl Pts',(-3.34994208384615,23.3321614954266,-48.9021343175402)) ;
#48889=CARTESIAN_POINT('Ctrl Pts',(-3.40665370878256,23.3263588536661,-49.1073011631896)) ;
#48890=CARTESIAN_POINT('Ctrl Pts',(-3.48096098013405,23.3186767407025,-49.5238351190535)) ;
#48891=CARTESIAN_POINT('Ctrl Pts',(-3.5,23.3166624979154,-49.7302427331703)) ;
#48892=CARTESIAN_POINT('Ctrl Pts',(-3.5,23.3166624979154,-49.935)) ;
#48893=CARTESIAN_POINT('Ctrl Pts',(-3.5,23.3166624979154,-50.1455828409761)) ;
#48894=CARTESIAN_POINT('Ctrl Pts',(-3.47985556658837,23.3187993298226,-50.3651730635468)) ;
#48895=CARTESIAN_POINT('Ctrl Pts',(-3.35394988821085,23.3317886364208,-51.0288729348247)) ;
#48896=CARTESIAN_POINT('Ctrl Pts',(-3.18762127333464,23.3490675354948,-51.4570912893388)) ;
#48897=CARTESIAN_POINT('Ctrl Pts',(-2.80013553531963,23.3829918057539,-52.0447545851038)) ;
#48898=CARTESIAN_POINT('Ctrl Pts',(-2.65639178601418,23.3949273566511,-52.2259765012846)) ;
#48899=CARTESIAN_POINT('Ctrl Pts',(-2.34081012768953,23.4184561910947,-52.5458841412736)) ;
#48900=CARTESIAN_POINT('Ctrl Pts',(-2.17020309673431,23.4301545727601,-52.6891786697715)) ;
#48901=CARTESIAN_POINT('Ctrl Pts',(-1.8002878644947,23.4520943063154,-52.9435506339984)) ;
#48902=CARTESIAN_POINT('Ctrl Pts',(-1.59798304164838,23.4625803703643,-53.0578107060785)) ;
#48903=CARTESIAN_POINT('Ctrl Pts',(-1.18610949070958,23.4795548198924,-53.234726969855)) ;
#48904=CARTESIAN_POINT('Ctrl Pts',(-0.978448173599702,23.4864137103971,
-53.3020383948391)) ;
#48905=CARTESIAN_POINT('Ctrl Pts',(-0.546367681279802,23.496232873925,-53.3980021942758)) ;
#48906=CARTESIAN_POINT('Ctrl Pts',(-0.318127533626824,23.4993132242412,
-53.4280956303302)) ;
#48907=CARTESIAN_POINT('Ctrl Pts',(0.102396123813041,23.5003576234828,-53.4385899044817)) ;
#48908=CARTESIAN_POINT('Ctrl Pts',(0.321147899491233,23.4994270880695,-53.4290562483249)) ;
#48909=CARTESIAN_POINT('Ctrl Pts',(0.794537083431156,23.4912924547276,-53.3497426101656)) ;
#48910=CARTESIAN_POINT('Ctrl Pts',(1.01911310535502,23.4852323438906,-53.2913599998513)) ;
#48911=CARTESIAN_POINT('Ctrl Pts',(1.44143612678983,23.4695745999603,-53.1317914335174)) ;
#48912=CARTESIAN_POINT('Ctrl Pts',(1.63939281408875,23.4604104308317,-53.0347656954105)) ;
#48913=CARTESIAN_POINT('Ctrl Pts',(2.01853311948898,23.4396612342924,-52.8014456739525)) ;
#48914=CARTESIAN_POINT('Ctrl Pts',(2.20372488656182,23.4278887940833,-52.6636415879441)) ;
#48915=CARTESIAN_POINT('Ctrl Pts',(2.51561110922712,23.4057035529924,-52.3760206544825)) ;
#48916=CARTESIAN_POINT('Ctrl Pts',(2.66714414079755,23.3940152627173,-52.2154232168398)) ;
#48917=CARTESIAN_POINT('Ctrl Pts',(3.0515057097697,23.3615304924259,-51.6903633524322)) ;
#48918=CARTESIAN_POINT('Ctrl Pts',(3.27379843042537,23.339894962795,-51.2863619910571)) ;
#48919=CARTESIAN_POINT('Ctrl Pts',(3.45245273953815,23.3216632778232,-50.5442029076169)) ;
#48920=CARTESIAN_POINT('Ctrl Pts',(3.48647565498117,23.3180820936627,-50.3167637435242)) ;
#48921=CARTESIAN_POINT('Ctrl Pts',(3.49881895345089,23.316786613132,-50.0351173441297)) ;
#48922=CARTESIAN_POINT('Ctrl Pts',(3.50001578883256,23.3166624121724,-49.9861001018762)) ;
#48923=CARTESIAN_POINT('Ctrl Pts',(3.50004380435856,23.3166609252339,-49.9350000240614)) ;
#48924=CARTESIAN_POINT('Origin',(0.,-10.,-49.935)) ;
#48925=CARTESIAN_POINT('Ctrl Pts',(16.7609414886787,-7.98064845424476,-317.752799113276)) ;
#48926=CARTESIAN_POINT('Ctrl Pts',(15.4331208186407,-10.7693750356367,-317.792519869162)) ;
#48927=CARTESIAN_POINT('Ctrl Pts',(11.3606506581665,-15.6667943575778,-317.87193861083)) ;
#48928=CARTESIAN_POINT('Ctrl Pts',(2.47769983667288,-19.1925023884035,-317.991055338281)) ;
#48929=CARTESIAN_POINT('Ctrl Pts',(-7.00582195046985,-18.0388785509995,
-318.110149295626)) ;
#48930=CARTESIAN_POINT('Ctrl Pts',(-14.7825411735154,-12.4887043542397,
-318.229243252972)) ;
#48931=CARTESIAN_POINT('Ctrl Pts',(-18.9557365910499,-3.89435973286506,
-318.348337210317)) ;
#48932=CARTESIAN_POINT('Ctrl Pts',(-18.5088006439409,5.64913768061575,-318.467431167663)) ;
#48933=CARTESIAN_POINT('Ctrl Pts',(-13.5503917473811,13.8157328865779,-318.586525125009)) ;
#48934=CARTESIAN_POINT('Ctrl Pts',(-5.2892196625952,18.6148302662477,-318.705619082354)) ;
#48935=CARTESIAN_POINT('Ctrl Pts',(4.26118141986884,18.8767092069171,-318.8247130397)) ;
#48936=CARTESIAN_POINT('Ctrl Pts',(12.7729410982788,14.5375272811165,-318.943806997045)) ;
#48937=CARTESIAN_POINT('Ctrl Pts',(18.1713965148236,6.65493323331481,-319.062900954391)) ;
#48938=CARTESIAN_POINT('Ctrl Pts',(19.140707108569,-2.84975204642665,-319.181994911737)) ;
#48939=CARTESIAN_POINT('Ctrl Pts',(15.4446141670581,-11.659831090839,-319.301088869082)) ;
#48940=CARTESIAN_POINT('Ctrl Pts',(7.9840110955058,-17.6279134214656,-319.420182826427)) ;
#48941=CARTESIAN_POINT('Ctrl Pts',(-1.42263490016496,-19.2993231591151,
-319.539276783773)) ;
#48942=CARTESIAN_POINT('Ctrl Pts',(-10.4825243720861,-16.2666667828338,
-319.658370741119)) ;
#48943=CARTESIAN_POINT('Ctrl Pts',(-16.9873766041342,-9.26913160922992,
-319.777464698464)) ;
#48944=CARTESIAN_POINT('Ctrl Pts',(-19.351682444702,-0.0123147099169769,
-319.89655865581)) ;
#48945=CARTESIAN_POINT('Ctrl Pts',(-16.9991599245348,9.24750381339812,-320.015652613156)) ;
#48946=CARTESIAN_POINT('Ctrl Pts',(-10.5032188933883,16.2533122115955,-320.134746570501)) ;
#48947=CARTESIAN_POINT('Ctrl Pts',(-1.44719654578774,19.2974969134576,-320.253840527847)) ;
#48948=CARTESIAN_POINT('Ctrl Pts',(7.96156917065858,17.638060587787,-320.372934485192)) ;
#48949=CARTESIAN_POINT('Ctrl Pts',(15.4297617489728,11.6794784702161,-320.492028442538)) ;
#48950=CARTESIAN_POINT('Ctrl Pts',(19.1370649157766,2.87411053553889,-320.611122399883)) ;
#48951=CARTESIAN_POINT('Ctrl Pts',(18.1798511593771,-6.63180041816628,-320.730216357229)) ;
#48952=CARTESIAN_POINT('Ctrl Pts',(12.7914341974471,-14.5212594541618,-320.849310314575)) ;
#48953=CARTESIAN_POINT('Ctrl Pts',(4.28520049872143,-18.8712697412915,-320.96840427192)) ;
#48954=CARTESIAN_POINT('Ctrl Pts',(-5.26551887922155,-18.6215486975565,
-321.087498229266)) ;
#48955=CARTESIAN_POINT('Ctrl Pts',(-13.5328072801144,-13.8329639659074,
-321.206592186611)) ;
#48956=CARTESIAN_POINT('Ctrl Pts',(-18.5015747815521,-5.67269738003963,
-321.325686143957)) ;
#48957=CARTESIAN_POINT('Ctrl Pts',(-18.9607213428039,3.87024690728918,-321.444780101302)) ;
#48958=CARTESIAN_POINT('Ctrl Pts',(-14.7983334120984,12.4698473602217,-321.563874058648)) ;
#48959=CARTESIAN_POINT('Ctrl Pts',(-7.0289620206353,18.0300154707455,-321.682968015994)) ;
#48960=CARTESIAN_POINT('Ctrl Pts',(2.45366646868374,19.1955017080385,-321.802061973339)) ;
#48961=CARTESIAN_POINT('Ctrl Pts',(11.3382320461671,15.6822274894264,-321.921155930684)) ;
#48962=CARTESIAN_POINT('Ctrl Pts',(17.4591880788544,8.34652721735456,-322.04024988803)) ;
#48963=CARTESIAN_POINT('Ctrl Pts',(19.324597160073,-1.02357684799465,-322.159343845376)) ;
#48964=CARTESIAN_POINT('Ctrl Pts',(16.479779731245,-10.1441916865021,-322.278437802722)) ;
#48965=CARTESIAN_POINT('Ctrl Pts',(9.61813883505806,-16.7922354173708,-322.397531760066)) ;
#48966=CARTESIAN_POINT('Ctrl Pts',(0.412148292514622,-19.347296936467,-322.516625717413)) ;
#48967=CARTESIAN_POINT('Ctrl Pts',(-8.89430032412952,-17.1865990442275,
-322.635719674758)) ;
#48968=CARTESIAN_POINT('Ctrl Pts',(-16.0328295358823,-10.8367957458002,
-322.754813632104)) ;
#48969=CARTESIAN_POINT('Ctrl Pts',(-19.2634760587788,-1.84560426302867,
-322.873907589449)) ;
#48970=CARTESIAN_POINT('Ctrl Pts',(-17.7987938844656,7.5954395015143,-322.993001546795)) ;
#48971=CARTESIAN_POINT('Ctrl Pts',(-11.9957883750258,15.1851515048236,-323.11209550414)) ;
#48972=CARTESIAN_POINT('Ctrl Pts',(-3.26889886712957,19.0735960206599,-323.231189461486)) ;
#48973=CARTESIAN_POINT('Ctrl Pts',(6.25476037288962,18.3129936831907,-323.350283418831)) ;
#48974=CARTESIAN_POINT('Ctrl Pts',(14.2538683957045,13.0887356425588,-323.469377376177)) ;
#48975=CARTESIAN_POINT('Ctrl Pts',(18.7787022470048,4.6741958539612,-323.588471333522)) ;
#48976=CARTESIAN_POINT('Ctrl Pts',(18.7263674041569,-4.87964433205772,-323.707565290868)) ;
#48977=CARTESIAN_POINT('Ctrl Pts',(14.109620094995,-13.2441075855554,-323.826659248214)) ;
#48978=CARTESIAN_POINT('Ctrl Pts',(6.05375806237365,-18.3804183381417,-323.94575320556)) ;
#48979=CARTESIAN_POINT('Ctrl Pts',(-3.47766237255771,-19.0366391305122,
-324.064847162905)) ;
#48980=CARTESIAN_POINT('Ctrl Pts',(-12.1614285270647,-15.0528210360699,
-324.18394112025)) ;
#48981=CARTESIAN_POINT('Ctrl Pts',(-17.880937130756,-7.39999001950697,-324.303035077596)) ;
#48982=CARTESIAN_POINT('Ctrl Pts',(-19.2421005953424,2.0565334039527,-324.422129034941)) ;
#48983=CARTESIAN_POINT('Ctrl Pts',(-15.9131454725967,11.0117921398302,-324.541222992288)) ;
#48984=CARTESIAN_POINT('Ctrl Pts',(-8.70547975928213,17.2830086247616,-324.660316949633)) ;
#48985=CARTESIAN_POINT('Ctrl Pts',(0.624081753732046,19.3416205868979,-324.779410906979)) ;
#48986=CARTESIAN_POINT('Ctrl Pts',(9.80152799124969,16.6858567055935,-324.898504864324)) ;
#48987=CARTESIAN_POINT('Ctrl Pts',(16.5899248425925,9.96303963055379,-325.01759882167)) ;
#48988=CARTESIAN_POINT('Ctrl Pts',(19.3346511767194,0.81180591118477,-325.136692779015)) ;
#48989=CARTESIAN_POINT('Ctrl Pts',(17.366700409186,-8.53729944774287,-325.255786736361)) ;
#48990=CARTESIAN_POINT('Ctrl Pts',(11.1657458702521,-15.8055017042738,-325.374880693706)) ;
#48991=CARTESIAN_POINT('Ctrl Pts',(2.24322400617006,-19.2212307363757,-325.493974651052)) ;
#48992=CARTESIAN_POINT('Ctrl Pts',(-7.22606698817188,-17.9519280537023,
-325.613068608397)) ;
#48993=CARTESIAN_POINT('Ctrl Pts',(-14.9340580180631,-12.3069767236302,
-325.732162565743)) ;
#48994=CARTESIAN_POINT('Ctrl Pts',(-19.0019837262,-3.66229155476228,-325.851256523089)) ;
#48995=CARTESIAN_POINT('Ctrl Pts',(-18.438317544,5.87504988144573,-325.970350480434)) ;
#48996=CARTESIAN_POINT('Ctrl Pts',(-13.3804489017432,13.9803917023341,-326.08944443778)) ;
#48997=CARTESIAN_POINT('Ctrl Pts',(-5.0611955790579,18.6781172571911,-326.208538395126)) ;
#48998=CARTESIAN_POINT('Ctrl Pts',(4.49168643930156,18.8231909593949,-326.327632352471)) ;
#48999=CARTESIAN_POINT('Ctrl Pts',(12.9497533696173,14.3802521754293,-326.446726309816)) ;
#49000=CARTESIAN_POINT('Ctrl Pts',(18.2514144450072,6.43223411572022,-326.565820267162)) ;
#49001=CARTESIAN_POINT('Ctrl Pts',(19.1044292975231,-3.08359306309894,-326.684914224507)) ;
#49002=CARTESIAN_POINT('Ctrl Pts',(15.300881915333,-11.8478174182373,-326.804008181853)) ;
#49003=CARTESIAN_POINT('Ctrl Pts',(7.76785862077557,-17.7242245926442,-326.923102139199)) ;
#49004=CARTESIAN_POINT('Ctrl Pts',(-1.6585223101039,-19.2804841409582,-327.042196096544)) ;
#49005=CARTESIAN_POINT('Ctrl Pts',(-10.6806507907074,-16.1372693988114,
-327.16129005389)) ;
#49006=CARTESIAN_POINT('Ctrl Pts',(-17.0994502558485,-9.06071552972577,
-327.280384011235)) ;
#49007=CARTESIAN_POINT('Ctrl Pts',(-19.3503861823524,0.22432021013761,-327.399477968581)) ;
#49008=CARTESIAN_POINT('Ctrl Pts',(-16.8848097168634,9.45467957088808,-327.518571925927)) ;
#49009=CARTESIAN_POINT('Ctrl Pts',(-10.30368674416,16.3805312624797,-327.637665883272)) ;
#49010=CARTESIAN_POINT('Ctrl Pts',(-1.21111693240772,19.3137505611646,-327.756759840617)) ;
#49011=CARTESIAN_POINT('Ctrl Pts',(8.176653603817,17.5393871274351,-327.875853797964)) ;
#49012=CARTESIAN_POINT('Ctrl Pts',(15.5714257738071,11.4899288219582,-327.994947755309)) ;
#49013=CARTESIAN_POINT('Ctrl Pts',(19.1707789825913,2.63988601335093,-328.114041712654)) ;
#49014=CARTESIAN_POINT('Ctrl Pts',(18.0973977155121,-6.85360933300335,-328.23313567)) ;
#49015=CARTESIAN_POINT('Ctrl Pts',(12.6129106553152,-14.6765884920131,-328.352229627345)) ;
#49016=CARTESIAN_POINT('Ctrl Pts',(4.05412064094016,-18.9222586070362,-328.471323584691)) ;
#49017=CARTESIAN_POINT('Ctrl Pts',(-5.49283105979263,-18.5557692352387,
-328.590417542037)) ;
#49018=CARTESIAN_POINT('Ctrl Pts',(-13.7009461338816,-13.6664494291431,
-328.709511499382)) ;
#49019=CARTESIAN_POINT('Ctrl Pts',(-18.5695577162308,-5.4460344459454,-328.828605456728)) ;
#49020=CARTESIAN_POINT('Ctrl Pts',(-18.911978024821,4.10181083809812,-328.947699414073)) ;
#49021=CARTESIAN_POINT('Ctrl Pts',(-14.6447446618728,12.6498703057146,-329.066793371419)) ;
#49022=CARTESIAN_POINT('Ctrl Pts',(-6.80796395116725,18.1146181798696,-329.185887328764)) ;
#49023=CARTESIAN_POINT('Ctrl Pts',(2.68820722530604,19.1640629010829,-329.30498128611)) ;
#49024=CARTESIAN_POINT('Ctrl Pts',(11.5291479288101,15.5424101412383,-329.424075243456)) ;
#49025=CARTESIAN_POINT('Ctrl Pts',(17.5599447642324,8.13241076434041,-329.543169200801)) ;
#49026=CARTESIAN_POINT('Ctrl Pts',(19.3106359571767,-1.25980311646076,-329.662263158147)) ;
#49027=CARTESIAN_POINT('Ctrl Pts',(16.3545035792121,-10.3449493783388,-329.781357115492)) ;
#49028=CARTESIAN_POINT('Ctrl Pts',(9.41208286212398,-16.9085913416631,-329.900451072838)) ;
#49029=CARTESIAN_POINT('Ctrl Pts',(0.175537106117643,-19.3508902039991,
-330.019545030184)) ;
#49030=CARTESIAN_POINT('Ctrl Pts',(-9.10379451103152,-17.0765538228228,
-330.138638987529)) ;
#49031=CARTESIAN_POINT('Ctrl Pts',(-16.1641440768252,-10.6399347378867,
-330.257732944874)) ;
#49032=CARTESIAN_POINT('Ctrl Pts',(-19.2846040132411,-1.60991087186129,
-330.376826902221)) ;
#49033=CARTESIAN_POINT('Ctrl Pts',(-17.7045854710373,7.81251676872362,-330.495920859566)) ;
#49034=CARTESIAN_POINT('Ctrl Pts',(-11.80920619224,15.330701682311,-330.615014816912)) ;
#49035=CARTESIAN_POINT('Ctrl Pts',(-3.03542093123559,19.1121423376101,-330.734108774257)) ;
#49036=CARTESIAN_POINT('Ctrl Pts',(6.47822555538839,18.2351407621758,-330.853202731602)) ;
#49037=CARTESIAN_POINT('Ctrl Pts',(14.4128528523085,12.9134595527517,-330.972296688948)) ;
#49038=CARTESIAN_POINT('Ctrl Pts',(18.8344547015049,4.44421883572467,-331.091390646294)) ;
#49039=CARTESIAN_POINT('Ctrl Pts',(18.6652986113538,-5.10826709480303,-331.210484603639)) ;
#49040=CARTESIAN_POINT('Ctrl Pts',(13.9466151179208,-13.4156509985701,-331.329578560985)) ;
#49041=CARTESIAN_POINT('Ctrl Pts',(5.82854814913269,-18.4530699732075,-331.44867251833)) ;
#49042=CARTESIAN_POINT('Ctrl Pts',(-3.71018398435288,-18.9926906931352,
-331.567766475676)) ;
#49043=CARTESIAN_POINT('Ctrl Pts',(-12.3445864277812,-14.9029846302641,
-331.686860433021)) ;
#49044=CARTESIAN_POINT('Ctrl Pts',(-17.9700879473739,-7.18078715229037,
-331.805954390367)) ;
#49045=CARTESIAN_POINT('Ctrl Pts',(-19.2155144808514,2.2916736676591,-331.925048347713)) ;
#49046=CARTESIAN_POINT('Ctrl Pts',(-15.7773025942279,11.20555611351,-332.044142305059)) ;
#49047=CARTESIAN_POINT('Ctrl Pts',(-8.49349080604967,17.3881677841687,-332.163236262404)) ;
#49048=CARTESIAN_POINT('Ctrl Pts',(0.860546054667159,19.3325431707949,-332.282330219749)) ;
#49049=CARTESIAN_POINT('Ctrl Pts',(10.0048312291659,16.5647552664916,-332.401424177095)) ;
#49050=CARTESIAN_POINT('Ctrl Pts',(16.710513368693,9.75943174153013,-332.520518134441)) ;
#49051=CARTESIAN_POINT('Ctrl Pts',(19.3431324366477,0.57531947747291,-332.639612091786)) ;
#49052=CARTESIAN_POINT('Ctrl Pts',(17.2610071590549,-8.74902262072224,-332.758706049132)) ;
#49053=CARTESIAN_POINT('Ctrl Pts',(10.9716400519316,-15.9408556713152,-332.877800006477)) ;
#49054=CARTESIAN_POINT('Ctrl Pts',(2.00801746598928,-19.2472239769566,-332.996893963823)) ;
#49055=CARTESIAN_POINT('Ctrl Pts',(-7.44504440929992,-17.8622249091877,
-333.115987921168)) ;
#49056=CARTESIAN_POINT('Ctrl Pts',(-15.0834322060208,-12.1234416668381,
-333.235081878514)) ;
#49057=CARTESIAN_POINT('Ctrl Pts',(-19.0453458361247,-3.42965988769476,
-333.35417583586)) ;
#49058=CARTESIAN_POINT('Ctrl Pts',(-18.3650983848235,6.10007592400356,-333.473269793205)) ;
#49059=CARTESIAN_POINT('Ctrl Pts',(-13.2084950977309,14.1429636998782,-333.592363750551)) ;
#49060=CARTESIAN_POINT('Ctrl Pts',(-4.83241958817477,18.7386094971499,-333.711457707896)) ;
#49061=CARTESIAN_POINT('Ctrl Pts',(4.7215221745996,18.7668589091946,-333.830551665242)) ;
#49062=CARTESIAN_POINT('Ctrl Pts',(13.1246281020728,14.2208263524006,-333.949645622587)) ;
#49063=CARTESIAN_POINT('Ctrl Pts',(18.3287037621201,6.2085733758486,-334.068739579933)) ;
#49064=CARTESIAN_POINT('Ctrl Pts',(19.0652945043705,-3.31697308166238,-334.187833537278)) ;
#49065=CARTESIAN_POINT('Ctrl Pts',(15.1548618260305,-12.0340320756082,-334.306927494624)) ;
#49066=CARTESIAN_POINT('Ctrl Pts',(7.55054454364082,-17.8178854541545,-334.42602145197)) ;
#49067=CARTESIAN_POINT('Ctrl Pts',(-1.89416168865372,-19.2587620697709,
-334.545115409315)) ;
#49068=CARTESIAN_POINT('Ctrl Pts',(-10.8771801286315,-16.0054589878645,
-334.664209366661)) ;
#49069=CARTESIAN_POINT('Ctrl Pts',(-17.2089669919832,-8.85094458414816,
-334.783303324007)) ;
#49070=CARTESIAN_POINT('Ctrl Pts',(-19.3461964286075,0.460921585997261,
-334.902397281352)) ;
#49071=CARTESIAN_POINT('Ctrl Pts',(-16.7679346944988,9.66044155535967,-335.021491238698)) ;
#49072=CARTESIAN_POINT('Ctrl Pts',(-10.1026138686454,16.5053009055333,-335.140585196043)) ;
#49073=CARTESIAN_POINT('Ctrl Pts',(-0.974856218396629,19.3271161925352,
-335.259679153389)) ;
#49074=CARTESIAN_POINT('Ctrl Pts',(8.39051536853628,17.4380909737272,-335.378773110734)) ;
#49075=CARTESIAN_POINT('Ctrl Pts',(15.7107613779483,11.2986610663483,-335.49786706808)) ;
#49076=CARTESIAN_POINT('Ctrl Pts',(19.2016264118602,2.4052667439143,-335.616961025425)) ;
#49077=CARTESIAN_POINT('Ctrl Pts',(18.0122381377377,-7.07439341485539,-335.736054982772)) ;
#49078=CARTESIAN_POINT('Ctrl Pts',(12.4325010853337,-14.8297229190515,-335.855148940116)) ;
#49079=CARTESIAN_POINT('Ctrl Pts',(3.82243456137157,-18.9704179897003,-335.974242897462)) ;
#49080=CARTESIAN_POINT('Ctrl Pts',(-5.71932188314611,-18.4872151129394,
-336.093336854808)) ;
#49081=CARTESIAN_POINT('Ctrl Pts',(-13.86703627375,-13.4978912961108,-336.212430812153)) ;
#49082=CARTESIAN_POINT('Ctrl Pts',(-18.6347638921671,-5.21855721929272,
-336.331524769499)) ;
#49083=CARTESIAN_POINT('Ctrl Pts',(-18.8604068147111,4.3327615466108,-336.450618726845)) ;
#49084=CARTESIAN_POINT('Ctrl Pts',(-14.4889659622868,12.8280014299124,-336.56971268419)) ;
#49085=CARTESIAN_POINT('Ctrl Pts',(-6.585948076489,18.1965127310871,-336.688806641536)) ;
#49086=CARTESIAN_POINT('Ctrl Pts',(2.92234642591305,19.1297573198475,-336.807900598881)) ;
#49087=CARTESIAN_POINT('Ctrl Pts',(11.7183389770801,15.4002710753346,-336.926994556227)) ;
#49088=CARTESIAN_POINT('Ctrl Pts',(17.6580774691844,7.91707335905638,-337.046088513572)) ;
#49089=CARTESIAN_POINT('Ctrl Pts',(19.2937835006079,-1.49583085020681,-337.165182470918)) ;
#49090=CARTESIAN_POINT('Ctrl Pts',(16.2267895858379,-10.544181217555,-337.284276428263)) ;
#49091=CARTESIAN_POINT('Ctrl Pts',(9.20460358311207,-17.0223752841955,-337.403370385609)) ;
#49092=CARTESIAN_POINT('Ctrl Pts',(-0.0610673351825857,-19.3516803088222,
-337.522464342955)) ;
#49093=CARTESIAN_POINT('Ctrl Pts',(-9.31199539433652,-16.9637679291851,
-337.6415583003)) ;
#49094=CARTESIAN_POINT('Ctrl Pts',(-16.2928939482416,-10.4418748891603,
-337.760652257646)) ;
#49095=CARTESIAN_POINT('Ctrl Pts',(-19.3035682799848,-1.37177778166763,
-337.879764674221)) ;
#49096=CARTESIAN_POINT('Ctrl Pts',(-18.1711237806586,4.89578622149652,-337.959179105016)) ;
#49097=CARTESIAN_POINT('Ctrl Pts',(-16.8891883469502,7.70553220148658,-337.998895550028)) ;
#49098=CARTESIAN_POINT('Ctrl Pts',(17.0212170400392,-8.10457751145466,-317.919234059516)) ;
#49099=CARTESIAN_POINT('Ctrl Pts',(15.6727770475582,-10.9366093778782,-317.958954815403)) ;
#49100=CARTESIAN_POINT('Ctrl Pts',(11.5370667393196,-15.9100792316539,-318.038373557071)) ;
#49101=CARTESIAN_POINT('Ctrl Pts',(2.51617528219197,-19.4905369077951,-318.157490284521)) ;
#49102=CARTESIAN_POINT('Ctrl Pts',(-7.11461322404616,-18.318998797464,-318.276584241867)) ;
#49103=CARTESIAN_POINT('Ctrl Pts',(-15.0120947494314,-12.6826376373893,
-318.395678199212)) ;
#49104=CARTESIAN_POINT('Ctrl Pts',(-19.2500944465446,-3.95483405809031,
-318.514772156558)) ;
#49105=CARTESIAN_POINT('Ctrl Pts',(-18.7962181673464,5.7368614177057,-318.633866113904)) ;
#49106=CARTESIAN_POINT('Ctrl Pts',(-13.7608116504385,14.0302731913054,-318.752960071249)) ;
#49107=CARTESIAN_POINT('Ctrl Pts',(-5.37135434249244,18.9038942913386,-318.872054028595)) ;
#49108=CARTESIAN_POINT('Ctrl Pts',(4.3273520072581,19.1698398702525,-318.99114798594)) ;
#49109=CARTESIAN_POINT('Ctrl Pts',(12.9712882071864,14.7632761109818,-319.110241943286)) ;
#49110=CARTESIAN_POINT('Ctrl Pts',(18.4535745923546,6.75827566295925,-319.229335900631)) ;
#49111=CARTESIAN_POINT('Ctrl Pts',(19.4379373148482,-2.89400497730318,-319.348429857977)) ;
#49112=CARTESIAN_POINT('Ctrl Pts',(15.6844488726799,-11.8408930537357,-319.467523815322)) ;
#49113=CARTESIAN_POINT('Ctrl Pts',(8.1079923701469,-17.9016519157027,-319.586617772668)) ;
#49114=CARTESIAN_POINT('Ctrl Pts',(-1.44472656388653,-19.5990164656943,
-319.705711730014)) ;
#49115=CARTESIAN_POINT('Ctrl Pts',(-10.6453042978102,-16.5192668929505,
-319.824805687359)) ;
#49116=CARTESIAN_POINT('Ctrl Pts',(-17.2511683973814,-9.41306912860228,
-319.943899644705)) ;
#49117=CARTESIAN_POINT('Ctrl Pts',(-19.652188822667,-0.0125059412935629,
-320.06299360205)) ;
#49118=CARTESIAN_POINT('Ctrl Pts',(-17.2631346973726,9.39110548132147,-320.182087559396)) ;
#49119=CARTESIAN_POINT('Ctrl Pts',(-10.6663201780257,16.505704942646,-320.301181516741)) ;
#49120=CARTESIAN_POINT('Ctrl Pts',(-1.46966961981743,19.5971618608248,-320.420275474087)) ;
#49121=CARTESIAN_POINT('Ctrl Pts',(8.08520195148935,17.9119566542768,-320.539369431433)) ;
#49122=CARTESIAN_POINT('Ctrl Pts',(15.6693658159213,11.8608455312784,-320.658463388778)) ;
#49123=CARTESIAN_POINT('Ctrl Pts',(19.434238563554,2.918741721968,-320.777557346124)) ;
#49124=CARTESIAN_POINT('Ctrl Pts',(18.4621605265063,-6.73478362537551,-320.896651303469)) ;
#49125=CARTESIAN_POINT('Ctrl Pts',(12.9900684800548,-14.7467556659011,-321.015745260815)) ;
#49126=CARTESIAN_POINT('Ctrl Pts',(4.35174407106482,-19.1643159368233,-321.134839218161)) ;
#49127=CARTESIAN_POINT('Ctrl Pts',(-5.34728551687813,-18.9107170511193,
-321.253933175506)) ;
#49128=CARTESIAN_POINT('Ctrl Pts',(-13.7429541193398,-14.0477718468136,
-321.373027132851)) ;
#49129=CARTESIAN_POINT('Ctrl Pts',(-18.7888800967433,-5.7607869685206,-321.492121090197)) ;
#49130=CARTESIAN_POINT('Ctrl Pts',(-19.2551566049893,3.93034679179602,-321.611215047543)) ;
#49131=CARTESIAN_POINT('Ctrl Pts',(-15.0281322208737,12.6634878188591,-321.730309004888)) ;
#49132=CARTESIAN_POINT('Ctrl Pts',(-7.13811262930777,18.3099980851382,-321.849402962234)) ;
#49133=CARTESIAN_POINT('Ctrl Pts',(2.49176870735705,19.4935828029504,-321.968496919579)) ;
#49134=CARTESIAN_POINT('Ctrl Pts',(11.5142999955279,15.9257520199028,-322.087590876925)) ;
#49135=CARTESIAN_POINT('Ctrl Pts',(17.7303064886763,8.47613789435082,-322.206684834271)) ;
#49136=CARTESIAN_POINT('Ctrl Pts',(19.6246829389091,-1.03947166086367,-322.325778791616)) ;
#49137=CARTESIAN_POINT('Ctrl Pts',(16.7356892073772,-10.3017177470814,-322.444872748962)) ;
#49138=CARTESIAN_POINT('Ctrl Pts',(9.76749598125699,-17.0529969226109,-322.563966706307)) ;
#49139=CARTESIAN_POINT('Ctrl Pts',(0.418548417719366,-19.6477352132116,
-322.683060663653)) ;
#49140=CARTESIAN_POINT('Ctrl Pts',(-9.03241720273038,-17.4534845020206,
-322.802154620998)) ;
#49141=CARTESIAN_POINT('Ctrl Pts',(-16.2817984586686,-11.0050770436988,
-322.921248578344)) ;
#49142=CARTESIAN_POINT('Ctrl Pts',(-19.5626127066636,-1.874264089058,-323.04034253569)) ;
#49143=CARTESIAN_POINT('Ctrl Pts',(-18.0751859293253,7.71338676631542,-323.159436493035)) ;
#49144=CARTESIAN_POINT('Ctrl Pts',(-12.1820673161834,15.4209570938522,-323.278530450381)) ;
#49145=CARTESIAN_POINT('Ctrl Pts',(-3.31966060122183,19.3697840793114,-323.397624407726)) ;
#49146=CARTESIAN_POINT('Ctrl Pts',(6.35188864016391,18.5973705799881,-323.516718365072)) ;
#49147=CARTESIAN_POINT('Ctrl Pts',(14.4752123732022,13.2919866286851,-323.635812322417)) ;
#49148=CARTESIAN_POINT('Ctrl Pts',(19.070310990134,4.74678001660378,-323.754906279763)) ;
#49149=CARTESIAN_POINT('Ctrl Pts',(19.0171634554639,-4.95541884149247,-323.874000237108)) ;
#49150=CARTESIAN_POINT('Ctrl Pts',(14.3287240846003,-13.4497712952244,-323.993094194454)) ;
#49151=CARTESIAN_POINT('Ctrl Pts',(6.14776502603686,-18.6658422518537,-324.1121881518)) ;
#49152=CARTESIAN_POINT('Ctrl Pts',(-3.53166593149108,-19.3322532968818,
-324.231282109145)) ;
#49153=CARTESIAN_POINT('Ctrl Pts',(-12.3502796436532,-15.2865717055856,
-324.350376066491)) ;
#49154=CARTESIAN_POINT('Ctrl Pts',(-18.1586047530488,-7.51490220887834,
-324.469470023836)) ;
#49155=CARTESIAN_POINT('Ctrl Pts',(-19.5409053101712,2.08846868431664,-324.588563981182)) ;
#49156=CARTESIAN_POINT('Ctrl Pts',(-16.160255858046,11.1827909033899,-324.707657938528)) ;
#49157=CARTESIAN_POINT('Ctrl Pts',(-8.84066450088723,17.5513911975433,-324.826751895873)) ;
#49158=CARTESIAN_POINT('Ctrl Pts',(0.633772929055101,19.6419707173401,-324.945845853219)) ;
#49159=CARTESIAN_POINT('Ctrl Pts',(9.953732931755,16.9449662882446,-325.064939810564)) ;
#49160=CARTESIAN_POINT('Ctrl Pts',(16.8475447285846,10.1177526360744,-325.18403376791)) ;
#49161=CARTESIAN_POINT('Ctrl Pts',(19.6348930813154,0.82441219772747,-325.303127725255)) ;
#49162=CARTESIAN_POINT('Ctrl Pts',(17.6363826061774,-8.66987256855422,-325.422221682601)) ;
#49163=CARTESIAN_POINT('Ctrl Pts',(11.3391353343638,-16.0509405224563,-325.541315639947)) ;
#49164=CARTESIAN_POINT('Ctrl Pts',(2.27805834798945,-19.5197113695261,-325.660409597292)) ;
#49165=CARTESIAN_POINT('Ctrl Pts',(-7.33827837980427,-18.2306980723983,
-325.779503554638)) ;
#49166=CARTESIAN_POINT('Ctrl Pts',(-15.1659644528732,-12.4980880137978,
-325.898597511983)) ;
#49167=CARTESIAN_POINT('Ctrl Pts',(-19.2970597393595,-3.71916216398806,
-326.017691469329)) ;
#49168=CARTESIAN_POINT('Ctrl Pts',(-18.7246405568311,5.96628174024054,-326.136785426674)) ;
#49169=CARTESIAN_POINT('Ctrl Pts',(-13.5882298141522,14.1974889436208,-326.25587938402)) ;
#49170=CARTESIAN_POINT('Ctrl Pts',(-5.13978934246745,18.9681640466733,-326.374973341366)) ;
#49171=CARTESIAN_POINT('Ctrl Pts',(4.56143646887577,19.1154905541777,-326.494067298711)) ;
#49172=CARTESIAN_POINT('Ctrl Pts',(13.1508461423911,14.6035587281184,-326.613161256057)) ;
#49173=CARTESIAN_POINT('Ctrl Pts',(18.5348350965852,6.53211831864999,-326.732255213402)) ;
#49174=CARTESIAN_POINT('Ctrl Pts',(19.4010961567326,-3.13147723984469,-326.851349170748)) ;
#49175=CARTESIAN_POINT('Ctrl Pts',(15.5384846466298,-12.0317985635109,-326.970443128093)) ;
#49176=CARTESIAN_POINT('Ctrl Pts',(7.88848332952349,-17.9994586737014,-327.089537085439)) ;
#49177=CARTESIAN_POINT('Ctrl Pts',(-1.68427699751195,-19.5798849021668,
-327.208631042785)) ;
#49178=CARTESIAN_POINT('Ctrl Pts',(-10.8465073611941,-16.3878601363941,
-327.32772500013)) ;
#49179=CARTESIAN_POINT('Ctrl Pts',(-17.3649824066712,-9.20141661932822,
-327.446818957476)) ;
#49180=CARTESIAN_POINT('Ctrl Pts',(-19.6508724310546,0.227803610304238,
-327.565912914822)) ;
#49181=CARTESIAN_POINT('Ctrl Pts',(-17.1470087801823,9.60149840799883,-327.685006872167)) ;
#49182=CARTESIAN_POINT('Ctrl Pts',(-10.4636895548728,16.634899539393,-327.804100829513)) ;
#49183=CARTESIAN_POINT('Ctrl Pts',(-1.22992399808227,19.6136679064725,-327.923194786858)) ;
#49184=CARTESIAN_POINT('Ctrl Pts',(8.30362636524895,17.8117509238366,-328.042288744204)) ;
#49185=CARTESIAN_POINT('Ctrl Pts',(15.8132296982158,11.6683524243107,-328.161382701549)) ;
#49186=CARTESIAN_POINT('Ctrl Pts',(19.4684761658357,2.68087999857057,-328.280476658895)) ;
#49187=CARTESIAN_POINT('Ctrl Pts',(18.3784266882447,-6.96003694323999,-328.39957061624)) ;
#49188=CARTESIAN_POINT('Ctrl Pts',(12.808772700254,-14.9044967610342,-328.518664573586)) ;
#49189=CARTESIAN_POINT('Ctrl Pts',(4.11707584460909,-19.2160965931217,-328.637758530931)) ;
#49190=CARTESIAN_POINT('Ctrl Pts',(-5.57812755901271,-18.8439161195818,
-328.756852488277)) ;
#49191=CARTESIAN_POINT('Ctrl Pts',(-13.9137039501156,-13.8786715565644,
-328.875946445623)) ;
#49192=CARTESIAN_POINT('Ctrl Pts',(-18.8579187176923,-5.53060425481351,
-328.995040402968)) ;
#49193=CARTESIAN_POINT('Ctrl Pts',(-19.2056563668791,4.16550660830191,-329.114134360314)) ;
#49194=CARTESIAN_POINT('Ctrl Pts',(-14.8721584377622,12.8463062857986,-329.23322831766)) ;
#49195=CARTESIAN_POINT('Ctrl Pts',(-6.91368274818291,18.395914563944,-329.352322275005)) ;
#49196=CARTESIAN_POINT('Ctrl Pts',(2.72995157589699,19.4616557923449,-329.471416232351)) ;
#49197=CARTESIAN_POINT('Ctrl Pts',(11.7081805527181,15.7837634907333,-329.590510189696)) ;
#49198=CARTESIAN_POINT('Ctrl Pts',(17.8326277939093,8.25869649220413,-329.709604147042)) ;
#49199=CARTESIAN_POINT('Ctrl Pts',(19.6105049367488,-1.27936621504706,-329.828698104387)) ;
#49200=CARTESIAN_POINT('Ctrl Pts',(16.6084676801657,-10.5055929439203,-329.947792061733)) ;
#49201=CARTESIAN_POINT('Ctrl Pts',(9.55824022792855,-17.1711597025844,-330.066886019078)) ;
#49202=CARTESIAN_POINT('Ctrl Pts',(0.178262968331908,-19.6513842794997,
-330.185979976424)) ;
#49203=CARTESIAN_POINT('Ctrl Pts',(-9.24516456100345,-17.3417304219163,
-330.305073933769)) ;
#49204=CARTESIAN_POINT('Ctrl Pts',(-16.4151521430909,-10.8051590412002,
-330.424167891115)) ;
#49205=CARTESIAN_POINT('Ctrl Pts',(-19.5840687506908,-1.63491068706249,
-330.54326184846)) ;
#49206=CARTESIAN_POINT('Ctrl Pts',(-17.9795145821613,7.93383496023844,-330.662355805807)) ;
#49207=CARTESIAN_POINT('Ctrl Pts',(-11.9925877555544,15.5687674756795,-330.781449763152)) ;
#49208=CARTESIAN_POINT('Ctrl Pts',(-3.08255705762935,19.408928970268,-330.900543720498)) ;
#49209=CARTESIAN_POINT('Ctrl Pts',(6.57882394536576,18.5183087046937,-331.019637677843)) ;
#49210=CARTESIAN_POINT('Ctrl Pts',(14.6366656509717,13.1139887299065,-331.138731635189)) ;
#49211=CARTESIAN_POINT('Ctrl Pts',(19.1269292075056,4.51323175535192,-331.257825592534)) ;
#49212=CARTESIAN_POINT('Ctrl Pts',(18.9551463439922,-5.18759181743238,-331.37691954988)) ;
#49213=CARTESIAN_POINT('Ctrl Pts',(14.1631878529239,-13.6239785536106,-331.496013507225)) ;
#49214=CARTESIAN_POINT('Ctrl Pts',(5.91905789670097,-18.739622072015,-331.615107464571)) ;
#49215=CARTESIAN_POINT('Ctrl Pts',(-3.76779830051932,-19.287622397617,-331.734201421916)) ;
#49216=CARTESIAN_POINT('Ctrl Pts',(-12.5362817475804,-15.1344085359069,
-331.853295379262)) ;
#49217=CARTESIAN_POINT('Ctrl Pts',(-18.2491399655233,-7.29229540715344,
-331.972389336607)) ;
#49218=CARTESIAN_POINT('Ctrl Pts',(-19.5139063480122,2.32726036950342,-332.091483293954)) ;
#49219=CARTESIAN_POINT('Ctrl Pts',(-16.0223035170261,11.3795637787544,-332.210577251299)) ;
#49220=CARTESIAN_POINT('Ctrl Pts',(-8.62538363581782,17.6581833414827,-332.329671208644)) ;
#49221=CARTESIAN_POINT('Ctrl Pts',(0.873909212041135,19.6327523408094,-332.44876516599)) ;
#49222=CARTESIAN_POINT('Ctrl Pts',(10.1601932036826,16.8219843018086,-332.567859123336)) ;
#49223=CARTESIAN_POINT('Ctrl Pts',(16.9700058371495,9.91098298220524,-332.686953080681)) ;
#49224=CARTESIAN_POINT('Ctrl Pts',(19.6435060441439,0.584253438271538,-332.806047038027)) ;
#49225=CARTESIAN_POINT('Ctrl Pts',(17.5290480777822,-8.88488352614997,-332.925140995372)) ;
#49226=CARTESIAN_POINT('Ctrl Pts',(11.1420153059574,-16.1883963599938,-333.044234952718)) ;
#49227=CARTESIAN_POINT('Ctrl Pts',(2.03919935714112,-19.5461082512168,-333.163328910063)) ;
#49228=CARTESIAN_POINT('Ctrl Pts',(-7.56065623455701,-18.1396019550955,
-333.282422867409)) ;
#49229=CARTESIAN_POINT('Ctrl Pts',(-15.317658227064,-12.3117028970533,-333.401516824754)) ;
#49230=CARTESIAN_POINT('Ctrl Pts',(-19.3410952062716,-3.4829180306727,-333.5206107821)) ;
#49231=CARTESIAN_POINT('Ctrl Pts',(-18.6502843996501,6.19480214362151,-333.639704739446)) ;
#49232=CARTESIAN_POINT('Ctrl Pts',(-13.4136057919318,14.3625854721601,-333.758798696791)) ;
#49233=CARTESIAN_POINT('Ctrl Pts',(-4.9074607589567,19.0295956521874,-333.877892654137)) ;
#49234=CARTESIAN_POINT('Ctrl Pts',(4.79484125324946,19.0582837407409,-333.996986611482)) ;
#49235=CARTESIAN_POINT('Ctrl Pts',(13.3284364512622,14.4416572300797,-334.116080568828)) ;
#49236=CARTESIAN_POINT('Ctrl Pts',(18.6133246159446,6.30498441932446,-334.235174526174)) ;
#49237=CARTESIAN_POINT('Ctrl Pts',(19.3613536513061,-3.36848134557823,-334.354268483519)) ;
#49238=CARTESIAN_POINT('Ctrl Pts',(15.3901970558699,-12.2209048915347,-334.473362440865)) ;
#49239=CARTESIAN_POINT('Ctrl Pts',(7.66779464832591,-18.0945739661805,-334.59245639821)) ;
#49240=CARTESIAN_POINT('Ctrl Pts',(-1.92357554814441,-19.5578255155574,
-334.711550355556)) ;
#49241=CARTESIAN_POINT('Ctrl Pts',(-11.0460885433012,-16.2540028817536,
-334.830644312901)) ;
#49242=CARTESIAN_POINT('Ctrl Pts',(-17.4761997948187,-8.98838820467845,
-334.949738270247)) ;
#49243=CARTESIAN_POINT('Ctrl Pts',(-19.6466176159009,0.468079096809521,
-335.068832227593)) ;
#49244=CARTESIAN_POINT('Ctrl Pts',(-17.0283188412208,9.81045560760757,-335.187926184938)) ;
#49245=CARTESIAN_POINT('Ctrl Pts',(-10.2594942799648,16.7616066922016,-335.307020142284)) ;
#49246=CARTESIAN_POINT('Ctrl Pts',(-0.989994463459544,19.6272410886586,
-335.426114099629)) ;
#49247=CARTESIAN_POINT('Ctrl Pts',(8.52080912412389,17.7088817730344,-335.545208056975)) ;
#49248=CARTESIAN_POINT('Ctrl Pts',(15.9547290024818,11.4741145300255,-335.66430201432)) ;
#49249=CARTESIAN_POINT('Ctrl Pts',(19.4998026154309,2.44261739801477,-335.783395971666)) ;
#49250=CARTESIAN_POINT('Ctrl Pts',(18.2919446933451,-7.18424951380041,-335.902489929011)) ;
#49251=CARTESIAN_POINT('Ctrl Pts',(12.6255616050522,-15.0600091659121,-336.021583886357)) ;
#49252=CARTESIAN_POINT('Ctrl Pts',(3.8817919825327,-19.2650038281594,-336.140677843703)) ;
#49253=CARTESIAN_POINT('Ctrl Pts',(-5.80813548932383,-18.7742974412137,
-336.259771801048)) ;
#49254=CARTESIAN_POINT('Ctrl Pts',(-14.0823732531388,-13.7074959356636,
-336.378865758394)) ;
#49255=CARTESIAN_POINT('Ctrl Pts',(-18.9241374604587,-5.29959460364702,
-336.49795971574)) ;
#49256=CARTESIAN_POINT('Ctrl Pts',(-19.1532843231671,4.40004367996941,-336.617053673085)) ;
#49257=CARTESIAN_POINT('Ctrl Pts',(-14.7139606982344,13.0272035539266,-336.736147630431)) ;
#49258=CARTESIAN_POINT('Ctrl Pts',(-6.68821925666094,18.4790808306846,-336.855241587776)) ;
#49259=CARTESIAN_POINT('Ctrl Pts',(2.96772665278063,19.4268174901953,-336.974335545122)) ;
#49260=CARTESIAN_POINT('Ctrl Pts',(11.9003094911082,15.6394171906014,-337.093429502467)) ;
#49261=CARTESIAN_POINT('Ctrl Pts',(17.932284371724,8.0400151779919,-337.212523459813)) ;
#49262=CARTESIAN_POINT('Ctrl Pts',(19.5933907835188,-1.51905915152522,-337.331617417158)) ;
#49263=CARTESIAN_POINT('Ctrl Pts',(16.4787704551177,-10.7079185936385,-337.450711374504)) ;
#49264=CARTESIAN_POINT('Ctrl Pts',(9.34753906643606,-17.2867105612771,-337.569805331849)) ;
#49265=CARTESIAN_POINT('Ctrl Pts',(-0.0620156312162582,-19.6521866536198,
-337.688899289195)) ;
#49266=CARTESIAN_POINT('Ctrl Pts',(-9.45659853236213,-17.2271931105152,
-337.807993246541)) ;
#49267=CARTESIAN_POINT('Ctrl Pts',(-16.5459013320153,-10.6040235814547,
-337.927087203886)) ;
#49268=CARTESIAN_POINT('Ctrl Pts',(-19.603327507752,-1.39307970069821,-338.046199620463)) ;
#49269=CARTESIAN_POINT('Ctrl Pts',(-18.4532976229839,4.97181139341203,-338.125614051257)) ;
#49270=CARTESIAN_POINT('Ctrl Pts',(-17.1514554046811,7.82518906226747,-338.165330496269)) ;
#49271=CARTESIAN_POINT('Ctrl Pts',(17.2814925913997,-8.22850656866457,-318.085669005756)) ;
#49272=CARTESIAN_POINT('Ctrl Pts',(15.9124332764758,-11.1038437201197,-318.125389761643)) ;
#49273=CARTESIAN_POINT('Ctrl Pts',(11.7134828204727,-16.15336410573,-318.204808503311)) ;
#49274=CARTESIAN_POINT('Ctrl Pts',(2.55465072771105,-19.7885714271867,-318.323925230762)) ;
#49275=CARTESIAN_POINT('Ctrl Pts',(-7.22340449762248,-18.5991190439285,
-318.443019188107)) ;
#49276=CARTESIAN_POINT('Ctrl Pts',(-15.2416483253474,-12.8765709205389,
-318.562113145453)) ;
#49277=CARTESIAN_POINT('Ctrl Pts',(-19.5444523020393,-4.01530838331557,
-318.681207102798)) ;
#49278=CARTESIAN_POINT('Ctrl Pts',(-19.083635690752,5.82458515479567,-318.800301060144)) ;
#49279=CARTESIAN_POINT('Ctrl Pts',(-13.9712315534961,14.2448134960331,-318.919395017489)) ;
#49280=CARTESIAN_POINT('Ctrl Pts',(-5.45348902238969,19.1929583164294,-319.038488974835)) ;
#49281=CARTESIAN_POINT('Ctrl Pts',(4.39352259464737,19.4629705335878,-319.157582932181)) ;
#49282=CARTESIAN_POINT('Ctrl Pts',(13.1696353160941,14.9890249408472,-319.276676889526)) ;
#49283=CARTESIAN_POINT('Ctrl Pts',(18.7357526698857,6.8616180926037,-319.395770846872)) ;
#49284=CARTESIAN_POINT('Ctrl Pts',(19.7351675211273,-2.93825790817971,-319.514864804217)) ;
#49285=CARTESIAN_POINT('Ctrl Pts',(15.9242835783017,-12.0219550166326,-319.633958761563)) ;
#49286=CARTESIAN_POINT('Ctrl Pts',(8.231973644788,-18.1753904099397,-319.753052718909)) ;
#49287=CARTESIAN_POINT('Ctrl Pts',(-1.46681822760808,-19.8987097722735,
-319.872146676254)) ;
#49288=CARTESIAN_POINT('Ctrl Pts',(-10.8080842235345,-16.7718670030672,
-319.991240633599)) ;
#49289=CARTESIAN_POINT('Ctrl Pts',(-17.5149601906285,-9.5570066479746,-320.110334590946)) ;
#49290=CARTESIAN_POINT('Ctrl Pts',(-19.9526952006321,-0.0126971726701712,
-320.229428548291)) ;
#49291=CARTESIAN_POINT('Ctrl Pts',(-17.5271094702105,9.53470714924482,-320.348522505636)) ;
#49292=CARTESIAN_POINT('Ctrl Pts',(-10.8294214626632,16.7580976736966,-320.467616462982)) ;
#49293=CARTESIAN_POINT('Ctrl Pts',(-1.4921426938471,19.8968268081918,-320.586710420328)) ;
#49294=CARTESIAN_POINT('Ctrl Pts',(8.20883473232013,18.1858527207668,-320.705804377673)) ;
#49295=CARTESIAN_POINT('Ctrl Pts',(15.9089698828699,12.0422125923406,-320.824898335019)) ;
#49296=CARTESIAN_POINT('Ctrl Pts',(19.7314122113315,2.96337290839712,-320.943992292364)) ;
#49297=CARTESIAN_POINT('Ctrl Pts',(18.7444698936355,-6.83776683258475,-321.06308624971)) ;
#49298=CARTESIAN_POINT('Ctrl Pts',(13.1887027626624,-14.9722518776403,-321.182180207055)) ;
#49299=CARTESIAN_POINT('Ctrl Pts',(4.41828764340822,-19.4573621323549,-321.301274164401)) ;
#49300=CARTESIAN_POINT('Ctrl Pts',(-5.42905215453471,-19.199885404682,-321.420368121746)) ;
#49301=CARTESIAN_POINT('Ctrl Pts',(-13.9531009585651,-14.2625797277198,
-321.539462079092)) ;
#49302=CARTESIAN_POINT('Ctrl Pts',(-19.0761854119345,-5.84887655700157,
-321.658556036438)) ;
#49303=CARTESIAN_POINT('Ctrl Pts',(-19.5495918671744,3.99044667630287,-321.777649993783)) ;
#49304=CARTESIAN_POINT('Ctrl Pts',(-15.2579310296489,12.8571282774965,-321.896743951129)) ;
#49305=CARTESIAN_POINT('Ctrl Pts',(-7.24726323798025,18.5899806995311,-322.015837908475)) ;
#49306=CARTESIAN_POINT('Ctrl Pts',(2.52987094603034,19.7916638978624,-322.13493186582)) ;
#49307=CARTESIAN_POINT('Ctrl Pts',(11.6903679448888,16.169276550379,-322.254025823166)) ;
#49308=CARTESIAN_POINT('Ctrl Pts',(18.0014248984984,8.60574857134709,-322.373119780511)) ;
#49309=CARTESIAN_POINT('Ctrl Pts',(19.9247687177452,-1.0553664737327,-322.492213737857)) ;
#49310=CARTESIAN_POINT('Ctrl Pts',(16.9915986835093,-10.4592438076606,-322.611307695202)) ;
#49311=CARTESIAN_POINT('Ctrl Pts',(9.91685312745595,-17.3137584278511,-322.730401652548)) ;
#49312=CARTESIAN_POINT('Ctrl Pts',(0.424948542924112,-19.9481734899561,
-322.849495609893)) ;
#49313=CARTESIAN_POINT('Ctrl Pts',(-9.17053408133125,-17.7203699598135,
-322.968589567239)) ;
#49314=CARTESIAN_POINT('Ctrl Pts',(-16.5307673814548,-11.1733583415976,
-323.087683524584)) ;
#49315=CARTESIAN_POINT('Ctrl Pts',(-19.8617493545485,-1.90292391508733,
-323.20677748193)) ;
#49316=CARTESIAN_POINT('Ctrl Pts',(-18.3515779741851,7.83133403111656,-323.325871439276)) ;
#49317=CARTESIAN_POINT('Ctrl Pts',(-12.3683462573407,15.6567626828807,-323.444965396621)) ;
#49318=CARTESIAN_POINT('Ctrl Pts',(-3.37042233531407,19.665972137963,-323.564059353967)) ;
#49319=CARTESIAN_POINT('Ctrl Pts',(6.44901690743819,18.8817474767855,-323.683153311313)) ;
#49320=CARTESIAN_POINT('Ctrl Pts',(14.6965563507,13.4952376148113,-323.802247268658)) ;
#49321=CARTESIAN_POINT('Ctrl Pts',(19.3619197332629,4.81936417924636,-323.921341226004)) ;
#49322=CARTESIAN_POINT('Ctrl Pts',(19.3079595067709,-5.0311933509272,-324.040435183349)) ;
#49323=CARTESIAN_POINT('Ctrl Pts',(14.5478280742058,-13.6554350048934,-324.159529140695)) ;
#49324=CARTESIAN_POINT('Ctrl Pts',(6.24177198970008,-18.9512661655657,-324.27862309804)) ;
#49325=CARTESIAN_POINT('Ctrl Pts',(-3.58566949042444,-19.6278674632513,
-324.397717055386)) ;
#49326=CARTESIAN_POINT('Ctrl Pts',(-12.5391307602418,-15.5203223751015,
-324.516811012731)) ;
#49327=CARTESIAN_POINT('Ctrl Pts',(-18.4362723753415,-7.62981439824971,
-324.635904970077)) ;
#49328=CARTESIAN_POINT('Ctrl Pts',(-19.8397100249999,2.12040396468059,-324.754998927422)) ;
#49329=CARTESIAN_POINT('Ctrl Pts',(-16.4073662434953,11.3537896669496,-324.874092884768)) ;
#49330=CARTESIAN_POINT('Ctrl Pts',(-8.97584924249228,17.8197737703252,-324.993186842114)) ;
#49331=CARTESIAN_POINT('Ctrl Pts',(0.643464104378149,19.9423208477824,-325.112280799459)) ;
#49332=CARTESIAN_POINT('Ctrl Pts',(10.1059378722603,17.2040758708956,-325.231374756805)) ;
#49333=CARTESIAN_POINT('Ctrl Pts',(17.1051646145768,10.272465641595,-325.350468714151)) ;
#49334=CARTESIAN_POINT('Ctrl Pts',(19.9351349859114,0.837018484270181,-325.469562671496)) ;
#49335=CARTESIAN_POINT('Ctrl Pts',(17.906064803169,-8.80244568936556,-325.588656628842)) ;
#49336=CARTESIAN_POINT('Ctrl Pts',(11.5125247984757,-16.2963793406389,-325.707750586187)) ;
#49337=CARTESIAN_POINT('Ctrl Pts',(2.31289268980884,-19.8181920026764,-325.826844543533)) ;
#49338=CARTESIAN_POINT('Ctrl Pts',(-7.45048977143667,-18.5094680910942,
-325.945938500878)) ;
#49339=CARTESIAN_POINT('Ctrl Pts',(-15.3978708876834,-12.6891993039652,
-326.065032458224)) ;
#49340=CARTESIAN_POINT('Ctrl Pts',(-19.592135752519,-3.77603277321385,-326.184126415569)) ;
#49341=CARTESIAN_POINT('Ctrl Pts',(-19.0109635696622,6.05751359903536,-326.303220372915)) ;
#49342=CARTESIAN_POINT('Ctrl Pts',(-13.7960107265613,14.4145861849075,-326.42231433026)) ;
#49343=CARTESIAN_POINT('Ctrl Pts',(-5.21838310587703,19.2582108361555,-326.541408287606)) ;
#49344=CARTESIAN_POINT('Ctrl Pts',(4.63118649845001,19.4077901489607,-326.660502244952)) ;
#49345=CARTESIAN_POINT('Ctrl Pts',(13.351938915165,14.8268652808078,-326.779596202297)) ;
#49346=CARTESIAN_POINT('Ctrl Pts',(18.8182557481633,6.63200252157975,-326.898690159643)) ;
#49347=CARTESIAN_POINT('Ctrl Pts',(19.6977630159421,-3.17936141659043,-327.017784116988)) ;
#49348=CARTESIAN_POINT('Ctrl Pts',(15.7760873779264,-12.2157797087843,-327.136878074334)) ;
#49349=CARTESIAN_POINT('Ctrl Pts',(8.00910803827142,-18.2746927547583,-327.25597203168)) ;
#49350=CARTESIAN_POINT('Ctrl Pts',(-1.71003168492,-19.8792856633756,-327.375065989025)) ;
#49351=CARTESIAN_POINT('Ctrl Pts',(-11.0123639316808,-16.6384508739767,
-327.494159946371)) ;
#49352=CARTESIAN_POINT('Ctrl Pts',(-17.6305145574939,-9.34211770893069,
-327.613253903716)) ;
#49353=CARTESIAN_POINT('Ctrl Pts',(-19.9513586797568,0.231287010470866,
-327.732347861062)) ;
#49354=CARTESIAN_POINT('Ctrl Pts',(-17.409207843501,9.74831724510958,-327.851441818407)) ;
#49355=CARTESIAN_POINT('Ctrl Pts',(-10.6236923655856,16.8892678163062,-327.970535775753)) ;
#49356=CARTESIAN_POINT('Ctrl Pts',(-1.2487310637568,19.9135852517806,-328.089629733099)) ;
#49357=CARTESIAN_POINT('Ctrl Pts',(8.43059912668088,18.084114720238,-328.208723690444)) ;
#49358=CARTESIAN_POINT('Ctrl Pts',(16.0550336226244,11.8467760266631,-328.32781764779)) ;
#49359=CARTESIAN_POINT('Ctrl Pts',(19.7661733490801,2.7218739837902,-328.446911605136)) ;
#49360=CARTESIAN_POINT('Ctrl Pts',(18.6594556609773,-7.06646455347665,-328.566005562481)) ;
#49361=CARTESIAN_POINT('Ctrl Pts',(13.0046347451928,-15.1324050300553,-328.685099519827)) ;
#49362=CARTESIAN_POINT('Ctrl Pts',(4.18003104827804,-19.5099345792074,-328.804193477172)) ;
#49363=CARTESIAN_POINT('Ctrl Pts',(-5.66342405823282,-19.1320630039249,
-328.923287434518)) ;
#49364=CARTESIAN_POINT('Ctrl Pts',(-14.1264617663495,-14.0908936839856,
-329.042381391863)) ;
#49365=CARTESIAN_POINT('Ctrl Pts',(-19.1462797191538,-5.61517406368159,
-329.161475349209)) ;
#49366=CARTESIAN_POINT('Ctrl Pts',(-19.4993347089371,4.22920237850569,-329.280569306554)) ;
#49367=CARTESIAN_POINT('Ctrl Pts',(-15.0995722136517,13.0427422658826,-329.3996632639)) ;
#49368=CARTESIAN_POINT('Ctrl Pts',(-7.01940154519854,18.6772109480185,-329.518757221246)) ;
#49369=CARTESIAN_POINT('Ctrl Pts',(2.77169592648789,19.7592486836067,-329.637851178591)) ;
#49370=CARTESIAN_POINT('Ctrl Pts',(11.8872131766261,16.0251168402282,-329.756945135937)) ;
#49371=CARTESIAN_POINT('Ctrl Pts',(18.1053108235861,8.38498222006786,-329.876039093282)) ;
#49372=CARTESIAN_POINT('Ctrl Pts',(19.9103739163207,-1.29892931363334,-329.995133050628)) ;
#49373=CARTESIAN_POINT('Ctrl Pts',(16.8624317811191,-10.6662365095016,-330.114227007973)) ;
#49374=CARTESIAN_POINT('Ctrl Pts',(9.70439759373315,-17.4337280635058,-330.233320965319)) ;
#49375=CARTESIAN_POINT('Ctrl Pts',(0.180988830546168,-19.9518783550005,
-330.352414922664)) ;
#49376=CARTESIAN_POINT('Ctrl Pts',(-9.38653461097536,-17.6069070210097,
-330.47150888001)) ;
#49377=CARTESIAN_POINT('Ctrl Pts',(-16.6661602093566,-10.9703833445135,
-330.590602837355)) ;
#49378=CARTESIAN_POINT('Ctrl Pts',(-19.8835334881402,-1.65991050226371,
-330.709696794702)) ;
#49379=CARTESIAN_POINT('Ctrl Pts',(-18.2544436932851,8.05515315175324,-330.828790752047)) ;
#49380=CARTESIAN_POINT('Ctrl Pts',(-12.1759693188687,15.8068332690481,-330.947884709393)) ;
#49381=CARTESIAN_POINT('Ctrl Pts',(-3.12969318402311,19.7057156029259,-331.066978666738)) ;
#49382=CARTESIAN_POINT('Ctrl Pts',(6.67942233534311,18.8014766472115,-331.186072624084)) ;
#49383=CARTESIAN_POINT('Ctrl Pts',(14.860478449635,13.3145179070613,-331.305166581429)) ;
#49384=CARTESIAN_POINT('Ctrl Pts',(19.4194037135064,4.58224467497918,-331.424260538775)) ;
#49385=CARTESIAN_POINT('Ctrl Pts',(19.2449940766305,-5.26691654006172,-331.54335449612)) ;
#49386=CARTESIAN_POINT('Ctrl Pts',(14.3797605879269,-13.8323061086509,-331.662448453466)) ;
#49387=CARTESIAN_POINT('Ctrl Pts',(6.00956764426923,-19.0261741708225,-331.781542410811)) ;
#49388=CARTESIAN_POINT('Ctrl Pts',(-3.82541261668574,-19.5825541020987,
-331.900636368157)) ;
#49389=CARTESIAN_POINT('Ctrl Pts',(-12.7279770673796,-15.3658324415495,
-332.019730325502)) ;
#49390=CARTESIAN_POINT('Ctrl Pts',(-18.5281919836726,-7.40380366201654,
-332.138824282848)) ;
#49391=CARTESIAN_POINT('Ctrl Pts',(-19.8122982151729,2.36284707134774,-332.257918240194)) ;
#49392=CARTESIAN_POINT('Ctrl Pts',(-16.2673044398244,11.553571443999,-332.377012197539)) ;
#49393=CARTESIAN_POINT('Ctrl Pts',(-8.75727646558595,17.9281988987967,-332.496106154885)) ;
#49394=CARTESIAN_POINT('Ctrl Pts',(0.887272369415106,19.9329615108239,-332.615200112231)) ;
#49395=CARTESIAN_POINT('Ctrl Pts',(10.3155551781992,17.0792133371256,-332.734294069576)) ;
#49396=CARTESIAN_POINT('Ctrl Pts',(17.229498305606,10.0625342228804,-332.853388026922)) ;
#49397=CARTESIAN_POINT('Ctrl Pts',(19.9438796516401,0.593187399070185,-332.972481984267)) ;
#49398=CARTESIAN_POINT('Ctrl Pts',(17.7970889965095,-9.02074443157773,-333.091575941613)) ;
#49399=CARTESIAN_POINT('Ctrl Pts',(11.3123905599832,-16.4359370486724,-333.210669898958)) ;
#49400=CARTESIAN_POINT('Ctrl Pts',(2.07038124829295,-19.8449925254769,-333.329763856304)) ;
#49401=CARTESIAN_POINT('Ctrl Pts',(-7.67626805981411,-18.4169790010034,
-333.448857813649)) ;
#49402=CARTESIAN_POINT('Ctrl Pts',(-15.5518842481071,-12.4999641272684,
-333.567951770995)) ;
#49403=CARTESIAN_POINT('Ctrl Pts',(-19.6368445764187,-3.53617617365065,
-333.68704572834)) ;
#49404=CARTESIAN_POINT('Ctrl Pts',(-18.9354704144768,6.28952836323949,-333.806139685686)) ;
#49405=CARTESIAN_POINT('Ctrl Pts',(-13.6187164861328,14.582207244442,-333.925233643031)) ;
#49406=CARTESIAN_POINT('Ctrl Pts',(-4.98250192973862,19.320581807225,-334.044327600378)) ;
#49407=CARTESIAN_POINT('Ctrl Pts',(4.86816033189934,19.3497085722871,-334.163421557723)) ;
#49408=CARTESIAN_POINT('Ctrl Pts',(13.5322448004516,14.6624881077588,-334.282515515069)) ;
#49409=CARTESIAN_POINT('Ctrl Pts',(18.8979454697689,6.40139546280031,-334.401609472414)) ;
#49410=CARTESIAN_POINT('Ctrl Pts',(19.6574127982416,-3.41998960949409,-334.52070342976)) ;
#49411=CARTESIAN_POINT('Ctrl Pts',(15.6255322857092,-12.4077777074612,-334.639797387105)) ;
#49412=CARTESIAN_POINT('Ctrl Pts',(7.785044753011,-18.3712624782065,-334.758891344451)) ;
#49413=CARTESIAN_POINT('Ctrl Pts',(-1.95298940763513,-19.8568889613439,
-334.877985301796)) ;
#49414=CARTESIAN_POINT('Ctrl Pts',(-11.214996957971,-16.5025467756427,-334.997079259142)) ;
#49415=CARTESIAN_POINT('Ctrl Pts',(-17.7434325976543,-9.12583182520876,
-335.116173216487)) ;
#49416=CARTESIAN_POINT('Ctrl Pts',(-19.9470388031943,0.475236607621789,
-335.235267173833)) ;
#49417=CARTESIAN_POINT('Ctrl Pts',(-17.2887029879428,9.96046965985546,-335.354361131178)) ;
#49418=CARTESIAN_POINT('Ctrl Pts',(-10.4163746912842,17.0179124788699,-335.473455088524)) ;
#49419=CARTESIAN_POINT('Ctrl Pts',(-1.00513270852244,19.927365984782,-335.592549045869)) ;
#49420=CARTESIAN_POINT('Ctrl Pts',(8.65110287971146,17.9796725723416,-335.711643003215)) ;
#49421=CARTESIAN_POINT('Ctrl Pts',(16.1986966270153,11.6495679937027,-335.830736960561)) ;
#49422=CARTESIAN_POINT('Ctrl Pts',(19.7979788190015,2.47996805211521,-335.949830917907)) ;
#49423=CARTESIAN_POINT('Ctrl Pts',(18.5716512489525,-7.29410561274543,-336.068924875252)) ;
#49424=CARTESIAN_POINT('Ctrl Pts',(12.8186221247707,-15.2902954127728,-336.188018832597)) ;
#49425=CARTESIAN_POINT('Ctrl Pts',(3.94114940369384,-19.5595896666186,-336.307112789943)) ;
#49426=CARTESIAN_POINT('Ctrl Pts',(-5.89694909550156,-19.0613797694881,
-336.426206747289)) ;
#49427=CARTESIAN_POINT('Ctrl Pts',(-14.2977102325278,-13.9171005752164,
-336.545300704634)) ;
#49428=CARTESIAN_POINT('Ctrl Pts',(-19.2135110287503,-5.3806319880013,-336.66439466198)) ;
#49429=CARTESIAN_POINT('Ctrl Pts',(-19.4461618316232,4.46732581332802,-336.783488619325)) ;
#49430=CARTESIAN_POINT('Ctrl Pts',(-14.9389554341818,13.2264056779408,-336.902582576671)) ;
#49431=CARTESIAN_POINT('Ctrl Pts',(-6.79049043683288,18.7616489302821,-337.021676534017)) ;
#49432=CARTESIAN_POINT('Ctrl Pts',(3.0131068796482,19.723877660543,-337.140770491362)) ;
#49433=CARTESIAN_POINT('Ctrl Pts',(12.0822800051361,15.8785633058685,-337.259864448708)) ;
#49434=CARTESIAN_POINT('Ctrl Pts',(18.2064912742636,8.16295699692743,-337.378958406053)) ;
#49435=CARTESIAN_POINT('Ctrl Pts',(19.8929980664296,-1.54228745284361,-337.498052363399)) ;
#49436=CARTESIAN_POINT('Ctrl Pts',(16.7307513243974,-10.8716559697218,-337.617146320744)) ;
#49437=CARTESIAN_POINT('Ctrl Pts',(9.49047454976006,-17.5510458383587,-337.73624027809)) ;
#49438=CARTESIAN_POINT('Ctrl Pts',(-0.0629639272499312,-19.9526929984175,
-337.855334235436)) ;
#49439=CARTESIAN_POINT('Ctrl Pts',(-9.60120167038777,-17.4906182918455,
-337.974428192781)) ;
#49440=CARTESIAN_POINT('Ctrl Pts',(-16.7989087157891,-10.7661722737493,
-338.093522150127)) ;
#49441=CARTESIAN_POINT('Ctrl Pts',(-19.9030867355192,-1.41438161972877,
-338.212634566703)) ;
#49442=CARTESIAN_POINT('Ctrl Pts',(-18.7354714653092,5.04783656532755,-338.292048997497)) ;
#49443=CARTESIAN_POINT('Ctrl Pts',(-17.4137224624119,7.94484592304836,-338.33176544251)) ;
#49444=CARTESIAN_POINT('Ctrl Pts',(17.5417681427602,-8.35243562587447,-318.252103951997)) ;
#49445=CARTESIAN_POINT('Ctrl Pts',(16.1520895053933,-11.2710780623612,-318.291824707884)) ;
#49446=CARTESIAN_POINT('Ctrl Pts',(11.8898989016257,-16.396648979806,-318.371243449552)) ;
#49447=CARTESIAN_POINT('Ctrl Pts',(2.59312617323014,-20.0866059465783,-318.490360177002)) ;
#49448=CARTESIAN_POINT('Ctrl Pts',(-7.3321957711988,-18.8792392903931,-318.609454134348)) ;
#49449=CARTESIAN_POINT('Ctrl Pts',(-15.4712019012634,-13.0705042036884,
-318.728548091693)) ;
#49450=CARTESIAN_POINT('Ctrl Pts',(-19.8388101575339,-4.07578270854084,
-318.847642049039)) ;
#49451=CARTESIAN_POINT('Ctrl Pts',(-19.3710532141577,5.91230889188563,-318.966736006384)) ;
#49452=CARTESIAN_POINT('Ctrl Pts',(-14.1816514565534,14.4593538007606,-319.08582996373)) ;
#49453=CARTESIAN_POINT('Ctrl Pts',(-5.53562370228694,19.4820223415202,-319.204923921076)) ;
#49454=CARTESIAN_POINT('Ctrl Pts',(4.45969318203664,19.7561011969232,-319.324017878421)) ;
#49455=CARTESIAN_POINT('Ctrl Pts',(13.3679824250016,15.2147737707125,-319.443111835767)) ;
#49456=CARTESIAN_POINT('Ctrl Pts',(19.0179307474167,6.96496052224815,-319.562205793112)) ;
#49457=CARTESIAN_POINT('Ctrl Pts',(20.0323977274064,-2.98251083905622,-319.681299750458)) ;
#49458=CARTESIAN_POINT('Ctrl Pts',(16.1641182839235,-12.2030169795293,-319.800393707803)) ;
#49459=CARTESIAN_POINT('Ctrl Pts',(8.35595491942909,-18.4491289041768,-319.91948766515)) ;
#49460=CARTESIAN_POINT('Ctrl Pts',(-1.48890989132965,-20.1984030788527,
-320.038581622495)) ;
#49461=CARTESIAN_POINT('Ctrl Pts',(-10.9708641492585,-17.0244671131838,
-320.15767557984)) ;
#49462=CARTESIAN_POINT('Ctrl Pts',(-17.7787519838756,-9.70094416734697,
-320.276769537186)) ;
#49463=CARTESIAN_POINT('Ctrl Pts',(-20.2532015785971,-0.0128884040467512,
-320.395863494531)) ;
#49464=CARTESIAN_POINT('Ctrl Pts',(-17.7910842430484,9.67830881716817,-320.514957451877)) ;
#49465=CARTESIAN_POINT('Ctrl Pts',(-10.9925227473007,17.0104904047472,-320.634051409222)) ;
#49466=CARTESIAN_POINT('Ctrl Pts',(-1.51461576787678,20.1964917555588,-320.753145366568)) ;
#49467=CARTESIAN_POINT('Ctrl Pts',(8.3324675131509,18.4597487872566,-320.872239323914)) ;
#49468=CARTESIAN_POINT('Ctrl Pts',(16.1485739498185,12.2235796534028,-320.991333281259)) ;
#49469=CARTESIAN_POINT('Ctrl Pts',(20.0285858591089,3.00800409482623,-321.110427238605)) ;
#49470=CARTESIAN_POINT('Ctrl Pts',(19.0267792607647,-6.94075003979398,-321.229521195951)) ;
#49471=CARTESIAN_POINT('Ctrl Pts',(13.3873370452701,-15.1977480893796,-321.348615153296)) ;
#49472=CARTESIAN_POINT('Ctrl Pts',(4.4848312157516,-19.7504083278867,-321.467709110641)) ;
#49473=CARTESIAN_POINT('Ctrl Pts',(-5.51081879219129,-19.4890537582448,
-321.586803067987)) ;
#49474=CARTESIAN_POINT('Ctrl Pts',(-14.1632477977904,-14.4773876086261,
-321.705897025332)) ;
#49475=CARTESIAN_POINT('Ctrl Pts',(-19.3634907271257,-5.93696614548253,
-321.824990982678)) ;
#49476=CARTESIAN_POINT('Ctrl Pts',(-19.8440271293597,4.05054656080969,-321.944084940023)) ;
#49477=CARTESIAN_POINT('Ctrl Pts',(-15.4877298384242,13.0507687361339,-322.06317889737)) ;
#49478=CARTESIAN_POINT('Ctrl Pts',(-7.35641384665271,18.869963313924,-322.182272854715)) ;
#49479=CARTESIAN_POINT('Ctrl Pts',(2.56797318470365,20.0897449927744,-322.301366812061)) ;
#49480=CARTESIAN_POINT('Ctrl Pts',(11.8664358942496,16.4128010808553,-322.420460769406)) ;
#49481=CARTESIAN_POINT('Ctrl Pts',(18.2725433083203,8.73535924834337,-322.539554726752)) ;
#49482=CARTESIAN_POINT('Ctrl Pts',(20.2248544965814,-1.07126128660173,-322.658648684097)) ;
#49483=CARTESIAN_POINT('Ctrl Pts',(17.2475081596413,-10.6167698682398,-322.777742641443)) ;
#49484=CARTESIAN_POINT('Ctrl Pts',(10.0662102736548,-17.5745199330913,-322.896836598788)) ;
#49485=CARTESIAN_POINT('Ctrl Pts',(0.431348668128854,-20.2486117667006,
-323.015930556134)) ;
#49486=CARTESIAN_POINT('Ctrl Pts',(-9.30865095993212,-17.9872554176065,
-323.135024513479)) ;
#49487=CARTESIAN_POINT('Ctrl Pts',(-16.779736304241,-11.3416396394963,-323.254118470825)) ;
#49488=CARTESIAN_POINT('Ctrl Pts',(-20.1608860024333,-1.93158374111668,
-323.37321242817)) ;
#49489=CARTESIAN_POINT('Ctrl Pts',(-18.6279700190449,7.94928129591769,-323.492306385517)) ;
#49490=CARTESIAN_POINT('Ctrl Pts',(-12.5546251984983,15.8925682719091,-323.611400342862)) ;
#49491=CARTESIAN_POINT('Ctrl Pts',(-3.42118406940633,19.9621601966145,-323.730494300208)) ;
#49492=CARTESIAN_POINT('Ctrl Pts',(6.54614517471249,19.1661243735829,-323.849588257553)) ;
#49493=CARTESIAN_POINT('Ctrl Pts',(14.9179003281977,13.6984886009376,-323.968682214899)) ;
#49494=CARTESIAN_POINT('Ctrl Pts',(19.653528476392,4.89194834188894,-324.087776172244)) ;
#49495=CARTESIAN_POINT('Ctrl Pts',(19.5987555580779,-5.10696786036194,-324.20687012959)) ;
#49496=CARTESIAN_POINT('Ctrl Pts',(14.7669320638112,-13.8610987145625,-324.325964086935)) ;
#49497=CARTESIAN_POINT('Ctrl Pts',(6.33577895336331,-19.2366900792777,-324.445058044282)) ;
#49498=CARTESIAN_POINT('Ctrl Pts',(-3.63967304935781,-19.9234816296209,
-324.564152001626)) ;
#49499=CARTESIAN_POINT('Ctrl Pts',(-12.7279818768303,-15.7540730446173,
-324.683245958972)) ;
#49500=CARTESIAN_POINT('Ctrl Pts',(-18.7139399976343,-7.74472658762109,
-324.802339916318)) ;
#49501=CARTESIAN_POINT('Ctrl Pts',(-20.1385147398288,2.15233924504454,-324.921433873664)) ;
#49502=CARTESIAN_POINT('Ctrl Pts',(-16.6544766289445,11.5247884305093,-325.040527831009)) ;
#49503=CARTESIAN_POINT('Ctrl Pts',(-9.11103398409737,18.0881563431071,-325.159621788354)) ;
#49504=CARTESIAN_POINT('Ctrl Pts',(0.653155279701203,20.2426709782248,-325.2787157457)) ;
#49505=CARTESIAN_POINT('Ctrl Pts',(10.2581428127656,17.4631854535467,-325.397809703047)) ;
#49506=CARTESIAN_POINT('Ctrl Pts',(17.3627845005688,10.4271786471158,-325.516903660391)) ;
#49507=CARTESIAN_POINT('Ctrl Pts',(20.2353768905073,0.849624770812879,-325.635997617737)) ;
#49508=CARTESIAN_POINT('Ctrl Pts',(18.1757470001605,-8.9350188101769,-325.755091575082)) ;
#49509=CARTESIAN_POINT('Ctrl Pts',(11.6859142625875,-16.5418181588214,-325.874185532428)) ;
#49510=CARTESIAN_POINT('Ctrl Pts',(2.34772703162821,-20.1166726358267,-325.993279489773)) ;
#49511=CARTESIAN_POINT('Ctrl Pts',(-7.56270116306905,-18.7882381097902,
-326.112373447119)) ;
#49512=CARTESIAN_POINT('Ctrl Pts',(-15.6297773224935,-12.8803105941328,
-326.231467404464)) ;
#49513=CARTESIAN_POINT('Ctrl Pts',(-19.8872117656786,-3.83290338243963,
-326.35056136181)) ;
#49514=CARTESIAN_POINT('Ctrl Pts',(-19.2972865824933,6.14874545783015,-326.469655319156)) ;
#49515=CARTESIAN_POINT('Ctrl Pts',(-14.0037916389702,14.6316834261942,-326.588749276501)) ;
#49516=CARTESIAN_POINT('Ctrl Pts',(-5.2969768692866,19.5482576256378,-326.707843233846)) ;
#49517=CARTESIAN_POINT('Ctrl Pts',(4.70093652802422,19.7000897437435,-326.826937191194)) ;
#49518=CARTESIAN_POINT('Ctrl Pts',(13.5530316879388,15.050171833497,-326.946031148539)) ;
#49519=CARTESIAN_POINT('Ctrl Pts',(19.1016763997412,6.73188672450952,-327.065125105884)) ;
#49520=CARTESIAN_POINT('Ctrl Pts',(19.9944298751515,-3.22724559333618,-327.184219063229)) ;
#49521=CARTESIAN_POINT('Ctrl Pts',(16.0136901092232,-12.3997608540579,-327.303313020575)) ;
#49522=CARTESIAN_POINT('Ctrl Pts',(8.12973274701934,-18.5499268358154,-327.422406977921)) ;
#49523=CARTESIAN_POINT('Ctrl Pts',(-1.73578637232805,-20.1786864245842,
-327.541500935266)) ;
#49524=CARTESIAN_POINT('Ctrl Pts',(-11.1782205021675,-16.8890416115595,
-327.660594892611)) ;
#49525=CARTESIAN_POINT('Ctrl Pts',(-17.8960467083165,-9.48281879853313,
-327.779688849957)) ;
#49526=CARTESIAN_POINT('Ctrl Pts',(-20.251844928459,0.234770410637488,-327.898782807302)) ;
#49527=CARTESIAN_POINT('Ctrl Pts',(-17.6714069068199,9.89513608222032,-328.017876764648)) ;
#49528=CARTESIAN_POINT('Ctrl Pts',(-10.7836951762985,17.1436360932194,-328.136970721993)) ;
#49529=CARTESIAN_POINT('Ctrl Pts',(-1.26753812943136,20.2135025970884,-328.256064679339)) ;
#49530=CARTESIAN_POINT('Ctrl Pts',(8.55757188811282,18.3564785166393,-328.375158636686)) ;
#49531=CARTESIAN_POINT('Ctrl Pts',(16.2968375470331,12.0251996290154,-328.494252594031)) ;
#49532=CARTESIAN_POINT('Ctrl Pts',(20.0638705323245,2.76286796900985,-328.613346551376)) ;
#49533=CARTESIAN_POINT('Ctrl Pts',(18.94048463371,-7.17289216371329,-328.732440508722)) ;
#49534=CARTESIAN_POINT('Ctrl Pts',(13.2004967901317,-15.3603132990765,-328.851534466067)) ;
#49535=CARTESIAN_POINT('Ctrl Pts',(4.24298625194697,-19.8037725652929,-328.970628423413)) ;
#49536=CARTESIAN_POINT('Ctrl Pts',(-5.7487205574529,-19.420209888268,-329.089722380758)) ;
#49537=CARTESIAN_POINT('Ctrl Pts',(-14.3392195825834,-14.3031158114068,
-329.208816338104)) ;
#49538=CARTESIAN_POINT('Ctrl Pts',(-19.4346407206152,-5.6997438725497,-329.327910295449)) ;
#49539=CARTESIAN_POINT('Ctrl Pts',(-19.7930130509952,4.29289814870947,-329.447004252795)) ;
#49540=CARTESIAN_POINT('Ctrl Pts',(-15.3269859895412,13.2391782459665,-329.56609821014)) ;
#49541=CARTESIAN_POINT('Ctrl Pts',(-7.12512034221418,18.9585073320931,-329.685192167486)) ;
#49542=CARTESIAN_POINT('Ctrl Pts',(2.81344027707881,20.0568415748685,-329.804286124832)) ;
#49543=CARTESIAN_POINT('Ctrl Pts',(12.0662458005342,16.2664701897232,-329.923380082177)) ;
#49544=CARTESIAN_POINT('Ctrl Pts',(18.377993853263,8.51126794793155,-330.042474039523)) ;
#49545=CARTESIAN_POINT('Ctrl Pts',(20.2102428958927,-1.31849241221963,-330.161567996868)) ;
#49546=CARTESIAN_POINT('Ctrl Pts',(17.1163958820726,-10.826880075083,-330.280661954214)) ;
#49547=CARTESIAN_POINT('Ctrl Pts',(9.85055495953772,-17.696296424427,-330.399755911559)) ;
#49548=CARTESIAN_POINT('Ctrl Pts',(0.183714692760428,-20.2523724305013,
-330.518849868905)) ;
#49549=CARTESIAN_POINT('Ctrl Pts',(-9.52790466094728,-17.8720836201031,
-330.63794382625)) ;
#49550=CARTESIAN_POINT('Ctrl Pts',(-16.9171682756223,-11.1356076478269,
-330.757037783596)) ;
#49551=CARTESIAN_POINT('Ctrl Pts',(-20.1829982255898,-1.68491031746492,
-330.876131740941)) ;
#49552=CARTESIAN_POINT('Ctrl Pts',(-18.5293728044092,8.17647134326807,-330.995225698287)) ;
#49553=CARTESIAN_POINT('Ctrl Pts',(-12.3593508821832,16.0448990624167,-331.114319655634)) ;
#49554=CARTESIAN_POINT('Ctrl Pts',(-3.17682931041687,20.0025022355838,-331.233413612979)) ;
#49555=CARTESIAN_POINT('Ctrl Pts',(6.78002072532046,19.0846445897294,-331.352507570324)) ;
#49556=CARTESIAN_POINT('Ctrl Pts',(15.0842912482982,13.515047084216,-331.47160152767)) ;
#49557=CARTESIAN_POINT('Ctrl Pts',(19.711878219507,4.65125759460642,-331.590695485015)) ;
#49558=CARTESIAN_POINT('Ctrl Pts',(19.5348418092689,-5.34624126269106,-331.709789442361)) ;
#49559=CARTESIAN_POINT('Ctrl Pts',(14.5963333229299,-14.0406336636914,-331.828883399706)) ;
#49560=CARTESIAN_POINT('Ctrl Pts',(6.10007739183751,-19.3127262696298,-331.947977357052)) ;
#49561=CARTESIAN_POINT('Ctrl Pts',(-3.88302693285218,-19.8774858065804,
-332.067071314397)) ;
#49562=CARTESIAN_POINT('Ctrl Pts',(-12.9196723871788,-15.5972563471924,
-332.186165271743)) ;
#49563=CARTESIAN_POINT('Ctrl Pts',(-18.8072440018219,-7.51531191687963,
-332.305259229089)) ;
#49564=CARTESIAN_POINT('Ctrl Pts',(-20.1106900823336,2.39843377319207,-332.424353186434)) ;
#49565=CARTESIAN_POINT('Ctrl Pts',(-16.5123053626227,11.7275791092434,-332.543447143779)) ;
#49566=CARTESIAN_POINT('Ctrl Pts',(-8.8891692953541,18.1982144561107,-332.662541101126)) ;
#49567=CARTESIAN_POINT('Ctrl Pts',(0.900635526789087,20.2331706808385,-332.78163505847)) ;
#49568=CARTESIAN_POINT('Ctrl Pts',(10.4709171527158,17.3364423724425,-332.900729015817)) ;
#49569=CARTESIAN_POINT('Ctrl Pts',(17.4889907740626,10.2140854635555,-333.019822973162)) ;
#49570=CARTESIAN_POINT('Ctrl Pts',(20.2442532591362,0.602121359868808,-333.138916930508)) ;
#49571=CARTESIAN_POINT('Ctrl Pts',(18.0651299152368,-9.15660533700547,-333.258010887853)) ;
#49572=CARTESIAN_POINT('Ctrl Pts',(11.4827658140091,-16.6834777373511,-333.3771048452)) ;
#49573=CARTESIAN_POINT('Ctrl Pts',(2.10156313944477,-20.1438767997371,-333.496198802544)) ;
#49574=CARTESIAN_POINT('Ctrl Pts',(-7.79187988507116,-18.6943560469111,
-333.615292759891)) ;
#49575=CARTESIAN_POINT('Ctrl Pts',(-15.7861102691503,-12.6882253574836,
-333.734386717235)) ;
#49576=CARTESIAN_POINT('Ctrl Pts',(-19.9325939465657,-3.5894343166286,-333.853480674581)) ;
#49577=CARTESIAN_POINT('Ctrl Pts',(-19.2206564293034,6.38425458285745,-333.972574631926)) ;
#49578=CARTESIAN_POINT('Ctrl Pts',(-13.8238271803337,14.8018290167238,-334.091668589273)) ;
#49579=CARTESIAN_POINT('Ctrl Pts',(-5.05754310052052,19.6115679622625,-334.210762546618)) ;
#49580=CARTESIAN_POINT('Ctrl Pts',(4.9414794105492,19.6411334038334,-334.329856503964)) ;
#49581=CARTESIAN_POINT('Ctrl Pts',(13.7360531496411,14.8833189854379,-334.448950461308)) ;
#49582=CARTESIAN_POINT('Ctrl Pts',(19.1825663235932,6.49780650627617,-334.568044418655)) ;
#49583=CARTESIAN_POINT('Ctrl Pts',(19.9534719451772,-3.47149787340994,-334.687138376)) ;
#49584=CARTESIAN_POINT('Ctrl Pts',(15.8608675155485,-12.5946505233876,-334.806232333347)) ;
#49585=CARTESIAN_POINT('Ctrl Pts',(7.9022948576961,-18.6479509902325,-334.925326290692)) ;
#49586=CARTESIAN_POINT('Ctrl Pts',(-1.98240326712582,-20.1559524071304,
-335.044420248037)) ;
#49587=CARTESIAN_POINT('Ctrl Pts',(-11.3839053726409,-16.7510906695319,
-335.163514205383)) ;
#49588=CARTESIAN_POINT('Ctrl Pts',(-18.0106654004898,-9.26327544573905,
-335.282608162728)) ;
#49589=CARTESIAN_POINT('Ctrl Pts',(-20.2474599904878,0.482394118434052,
-335.401702120073)) ;
#49590=CARTESIAN_POINT('Ctrl Pts',(-17.5490871346648,10.1104837121034,-335.520796077419)) ;
#49591=CARTESIAN_POINT('Ctrl Pts',(-10.5732551026036,17.2742182655382,-335.639890034764)) ;
#49592=CARTESIAN_POINT('Ctrl Pts',(-1.02027095358536,20.2274908809053,-335.75898399211)) ;
#49593=CARTESIAN_POINT('Ctrl Pts',(8.78139663529907,18.2504633716488,-335.878077949457)) ;
#49594=CARTESIAN_POINT('Ctrl Pts',(16.4426642515488,11.8250214573798,-335.997171906802)) ;
#49595=CARTESIAN_POINT('Ctrl Pts',(20.0961550225722,2.51731870621567,-336.116265864147)) ;
#49596=CARTESIAN_POINT('Ctrl Pts',(18.8513578045599,-7.40396171169045,-336.235359821493)) ;
#49597=CARTESIAN_POINT('Ctrl Pts',(13.0116826444891,-15.5205816596335,-336.354453778838)) ;
#49598=CARTESIAN_POINT('Ctrl Pts',(4.00050682485498,-19.8541755050778,-336.473547736184)) ;
#49599=CARTESIAN_POINT('Ctrl Pts',(-5.9857627016793,-19.3484620977624,-336.592641693529)) ;
#49600=CARTESIAN_POINT('Ctrl Pts',(-14.5130472119166,-14.126705214769,-336.711735650875)) ;
#49601=CARTESIAN_POINT('Ctrl Pts',(-19.5028845970419,-5.46166937235563,
-336.83082960822)) ;
#49602=CARTESIAN_POINT('Ctrl Pts',(-19.7390393400793,4.53460794668666,-336.949923565566)) ;
#49603=CARTESIAN_POINT('Ctrl Pts',(-15.1639501701295,13.425607801955,-337.069017522911)) ;
#49604=CARTESIAN_POINT('Ctrl Pts',(-6.89276161700482,19.0442170298797,-337.188111480257)) ;
#49605=CARTESIAN_POINT('Ctrl Pts',(3.05848710651578,20.0209378308908,-337.307205437602)) ;
#49606=CARTESIAN_POINT('Ctrl Pts',(12.2642505191642,16.1177094211354,-337.426299394949)) ;
#49607=CARTESIAN_POINT('Ctrl Pts',(18.480698176803,8.28589881586294,-337.545393352293)) ;
#49608=CARTESIAN_POINT('Ctrl Pts',(20.1926053493404,-1.56551575416202,-337.66448730964)) ;
#49609=CARTESIAN_POINT('Ctrl Pts',(16.9827321936771,-11.0353933458052,-337.783581266985)) ;
#49610=CARTESIAN_POINT('Ctrl Pts',(9.63341003308405,-17.8153811154403,-337.902675224331)) ;
#49611=CARTESIAN_POINT('Ctrl Pts',(-0.0639122232836121,-20.2531993432151,
-338.021769181676)) ;
#49612=CARTESIAN_POINT('Ctrl Pts',(-9.74580480841337,-17.7540434731756,
-338.140863139021)) ;
#49613=CARTESIAN_POINT('Ctrl Pts',(-17.0519160995629,-10.9283209660436,
-338.259957096367)) ;
#49614=CARTESIAN_POINT('Ctrl Pts',(-20.2028459632864,-1.43568353875935,
-338.379069512944)) ;
#49615=CARTESIAN_POINT('Ctrl Pts',(-19.0176453076346,5.12386173724306,-338.458483943739)) ;
#49616=CARTESIAN_POINT('Ctrl Pts',(-17.6759895201426,8.06450278382925,-338.49820038875)) ;
#49617=CARTESIAN_POINT('Ctrl Pts',(1.53122046431516,-19.3652704049865,-338.)) ;
#49618=CARTESIAN_POINT('Ctrl Pts',(1.12192133411244,-19.3892945386684,-338.)) ;
#49619=CARTESIAN_POINT('Ctrl Pts',(0.712537519554564,-19.4002678090365,
-338.)) ;
#49620=CARTESIAN_POINT('Ctrl Pts',(0.303666630142025,-19.3980968578391,
-338.)) ;
#49621=CARTESIAN_POINT('Ctrl Pts',(0.181986669634313,-19.3974507828487,
-338.)) ;
#49622=CARTESIAN_POINT('Ctrl Pts',(0.0603520673764698,-19.3956402363443,
-338.)) ;
#49623=CARTESIAN_POINT('Ctrl Pts',(-0.061221567909213,-19.3926618778456,
-338.)) ;
#49624=CARTESIAN_POINT('Ctrl Pts',(-0.466207908217332,-19.3827403639772,
-338.)) ;
#49625=CARTESIAN_POINT('Ctrl Pts',(-0.870517665367189,-19.3598637558529,
-338.)) ;
#49626=CARTESIAN_POINT('Ctrl Pts',(-1.2735764150429,-19.3242721999153,-338.)) ;
#49627=CARTESIAN_POINT('Ctrl Pts',(-1.68065183836914,-19.2883259570616,
-338.)) ;
#49628=CARTESIAN_POINT('Ctrl Pts',(-2.08645173638727,-19.2394100004437,
-338.)) ;
#49629=CARTESIAN_POINT('Ctrl Pts',(-2.49038044442016,-19.1777188116874,
-338.)) ;
#49630=CARTESIAN_POINT('Ctrl Pts',(-2.89439384831672,-19.1160146875086,
-338.)) ;
#49631=CARTESIAN_POINT('Ctrl Pts',(-3.29653581874664,-19.0415298124728,
-338.)) ;
#49632=CARTESIAN_POINT('Ctrl Pts',(-3.69619830300842,-18.9544080717603,
-338.)) ;
#49633=CARTESIAN_POINT('Ctrl Pts',(-4.09281102360135,-18.8679511438087,
-338.)) ;
#49634=CARTESIAN_POINT('Ctrl Pts',(-4.48698245887238,-18.7690492636138,
-338.)) ;
#49635=CARTESIAN_POINT('Ctrl Pts',(-4.87809877604152,-18.6577959732304,
-338.)) ;
#49636=CARTESIAN_POINT('Ctrl Pts',(-5.15629077763809,-18.578664077737,-338.)) ;
#49637=CARTESIAN_POINT('Ctrl Pts',(-5.4329367601865,-18.4932824403319,-338.)) ;
#49638=CARTESIAN_POINT('Ctrl Pts',(-5.70780760673927,-18.4016708993542,
-338.)) ;
#49639=CARTESIAN_POINT('Ctrl Pts',(-5.75904326826443,-18.3845945961951,
-338.)) ;
#49640=CARTESIAN_POINT('Ctrl Pts',(-5.81021723142297,-18.3673018061672,
-338.)) ;
#49641=CARTESIAN_POINT('Ctrl Pts',(-5.8613279811968,-18.3497926149073,-338.)) ;
#49642=CARTESIAN_POINT('Ctrl Pts',(-5.90598635521624,-18.3344938369492,
-338.)) ;
#49643=CARTESIAN_POINT('Ctrl Pts',(-5.95058793173612,-18.3190327470415,
-338.)) ;
#49644=CARTESIAN_POINT('Ctrl Pts',(-5.99512278417975,-18.3034128014496,
-338.)) ;
#49645=CARTESIAN_POINT('Ctrl Pts',(-6.01150522446275,-18.2976669010627,
-338.)) ;
#49646=CARTESIAN_POINT('Ctrl Pts',(-6.02787882113695,-18.2918994425318,
-338.)) ;
#49647=CARTESIAN_POINT('Ctrl Pts',(-6.04424329331104,-18.2861105298845,
-338.)) ;
#49648=CARTESIAN_POINT('Ctrl Pts',(-6.42829511386026,-18.1502526532877,
-338.)) ;
#49649=CARTESIAN_POINT('Ctrl Pts',(-6.80747072006426,-18.0025302201036,
-338.)) ;
#49650=CARTESIAN_POINT('Ctrl Pts',(-7.18119888215102,-17.8431638857732,
-338.)) ;
#49651=CARTESIAN_POINT('Ctrl Pts',(-7.55462919821985,-17.6839245598753,
-338.)) ;
#49652=CARTESIAN_POINT('Ctrl Pts',(-7.92262127604276,-17.5130596995448,
-338.)) ;
#49653=CARTESIAN_POINT('Ctrl Pts',(-8.28459074029327,-17.3307396766341,
-338.)) ;
#49654=CARTESIAN_POINT('Ctrl Pts',(-8.60540796776493,-17.1691475810581,
-338.)) ;
#49655=CARTESIAN_POINT('Ctrl Pts',(-8.92149419227665,-16.998556156645,-338.)) ;
#49656=CARTESIAN_POINT('Ctrl Pts',(-9.23242801516554,-16.819053016636,-338.)) ;
#49657=CARTESIAN_POINT('Ctrl Pts',(-9.58379862825655,-16.6162055818645,
-338.)) ;
#49658=CARTESIAN_POINT('Ctrl Pts',(-9.92859044196816,-16.4019782696566,
-338.)) ;
#49659=CARTESIAN_POINT('Ctrl Pts',(-10.2663642689513,-16.1768116880322,
-338.)) ;
#49660=CARTESIAN_POINT('Ctrl Pts',(-10.6170152476493,-15.9430609474202,
-338.)) ;
#49661=CARTESIAN_POINT('Ctrl Pts',(-10.9601036420671,-15.6975207646042,
-338.)) ;
#49662=CARTESIAN_POINT('Ctrl Pts',(-11.2950979866766,-15.4406404079358,
-338.)) ;
#49663=CARTESIAN_POINT('Ctrl Pts',(-11.6300923312865,-15.183760051267,-338.)) ;
#49664=CARTESIAN_POINT('Ctrl Pts',(-11.9569931202482,-14.9155390478906,
-338.)) ;
#49665=CARTESIAN_POINT('Ctrl Pts',(-12.2752207699239,-14.6363892224392,
-338.)) ;
#49666=CARTESIAN_POINT('Ctrl Pts',(-12.3029402979512,-14.6120736061868,
-338.)) ;
#49667=CARTESIAN_POINT('Ctrl Pts',(-12.3305931560439,-14.5876757429795,
-338.)) ;
#49668=CARTESIAN_POINT('Ctrl Pts',(-12.3581695198653,-14.5632043767021,
-338.)) ;
#49669=CARTESIAN_POINT('Ctrl Pts',(-12.6595416244126,-14.2957656670909,
-338.)) ;
#49670=CARTESIAN_POINT('Ctrl Pts',(-12.9520844173906,-14.0192854610996,
-338.)) ;
#49671=CARTESIAN_POINT('Ctrl Pts',(-13.2354196355927,-13.7342473807588,
-338.)) ;
#49672=CARTESIAN_POINT('Ctrl Pts',(-13.5205791579126,-13.4473740321199,
-338.)) ;
#49673=CARTESIAN_POINT('Ctrl Pts',(-13.7964125715532,-13.1518318817186,
-338.)) ;
#49674=CARTESIAN_POINT('Ctrl Pts',(-14.0625020156188,-12.8480723757908,
-338.)) ;
#49675=CARTESIAN_POINT('Ctrl Pts',(-14.328094515029,-12.544880166561,-338.)) ;
#49676=CARTESIAN_POINT('Ctrl Pts',(-14.5839797799945,-12.2335008504745,
-338.)) ;
#49677=CARTESIAN_POINT('Ctrl Pts',(-14.8297043966001,-11.9143480443392,
-338.)) ;
#49678=CARTESIAN_POINT('Ctrl Pts',(-15.0728958847685,-11.5984853239113,
-338.)) ;
#49679=CARTESIAN_POINT('Ctrl Pts',(-15.3061354351909,-11.275008127149,-338.)) ;
#49680=CARTESIAN_POINT('Ctrl Pts',(-15.5289414287006,-10.9442891626757,
-338.)) ;
#49681=CARTESIAN_POINT('Ctrl Pts',(-15.6845001549643,-10.7133877400778,
-338.)) ;
#49682=CARTESIAN_POINT('Ctrl Pts',(-15.8349721202972,-10.4789556881506,
-338.)) ;
#49683=CARTESIAN_POINT('Ctrl Pts',(-15.9801798449266,-10.2411132100054,
-338.)) ;
#49684=CARTESIAN_POINT('Ctrl Pts',(-16.1748344006451,-9.92227947004763,
-338.)) ;
#49685=CARTESIAN_POINT('Ctrl Pts',(-16.3600303833031,-9.59731728203679,
-338.)) ;
#49686=CARTESIAN_POINT('Ctrl Pts',(-16.5355799150942,-9.2666831201162,-338.)) ;
#49687=CARTESIAN_POINT('Ctrl Pts',(-16.5779666097208,-9.18685101169948,
-338.)) ;
#49688=CARTESIAN_POINT('Ctrl Pts',(-16.6197907574038,-9.10668819275675,
-338.)) ;
#49689=CARTESIAN_POINT('Ctrl Pts',(-16.661049385152,-9.02620102002121,-338.)) ;
#49690=CARTESIAN_POINT('Ctrl Pts',(-16.6936059345179,-8.96268982841101,
-338.)) ;
#49691=CARTESIAN_POINT('Ctrl Pts',(-16.7258103578028,-8.8989766759393,-338.)) ;
#49692=CARTESIAN_POINT('Ctrl Pts',(-16.7576611369262,-8.83506467784942,
-338.)) ;
#49693=CARTESIAN_POINT('Ctrl Pts',(-16.779604249934,-8.79103347248394,-338.)) ;
#49694=CARTESIAN_POINT('Ctrl Pts',(-16.8013802791104,-8.74690619927829,
-338.)) ;
#49695=CARTESIAN_POINT('Ctrl Pts',(-16.8229776736961,-8.7027068234737,-338.)) ;
#49696=CARTESIAN_POINT('Ctrl Pts',(-16.9064115593317,-8.53195818750261,
-338.)) ;
#49697=CARTESIAN_POINT('Ctrl Pts',(-16.9872118844882,-8.36007011454329,
-338.)) ;
#49698=CARTESIAN_POINT('Ctrl Pts',(-17.0653728977658,-8.18710624704896,
-338.)) ;
#49699=CARTESIAN_POINT('Ctrl Pts',(-17.2299870027546,-7.82282882728421,
-338.)) ;
#49700=CARTESIAN_POINT('Ctrl Pts',(-17.3828941511382,-7.45378725021279,
-338.)) ;
#49701=CARTESIAN_POINT('Ctrl Pts',(-17.5239885713209,-7.08059343174374,
-338.)) ;
#49702=CARTESIAN_POINT('Ctrl Pts',(-17.6659184550873,-6.70518981756066,
-338.)) ;
#49703=CARTESIAN_POINT('Ctrl Pts',(-17.7958954921236,-6.32558411687078,
-338.)) ;
#49704=CARTESIAN_POINT('Ctrl Pts',(-17.9137644956534,-5.9423765101345,-338.)) ;
#49705=CARTESIAN_POINT('Ctrl Pts',(-18.0314668555706,-5.55971068366358,
-338.)) ;
#49706=CARTESIAN_POINT('Ctrl Pts',(-18.1370955328315,-5.17345258238865,
-338.)) ;
#49707=CARTESIAN_POINT('Ctrl Pts',(-18.2304463747966,-4.7841853991055,-338.)) ;
#49708=CARTESIAN_POINT('Ctrl Pts',(-18.3232264444352,-4.39729830079178,
-338.)) ;
#49709=CARTESIAN_POINT('Ctrl Pts',(-18.4038784618712,-4.00743827161781,
-338.)) ;
#49710=CARTESIAN_POINT('Ctrl Pts',(-18.4721512104871,-3.61517165557224,
-338.)) ;
#49711=CARTESIAN_POINT('Ctrl Pts',(-18.5393817124124,-3.22889335244342,
-338.)) ;
#49712=CARTESIAN_POINT('Ctrl Pts',(-18.5946080455807,-2.84028088845193,
-338.)) ;
#49713=CARTESIAN_POINT('Ctrl Pts',(-18.6375401222669,-2.44987658596576,
-338.)) ;
#49714=CARTESIAN_POINT('Ctrl Pts',(-18.6620178572193,-2.22728746896645,
-338.)) ;
#49715=CARTESIAN_POINT('Ctrl Pts',(-18.6824981590813,-2.00411594415889,
-338.)) ;
#49716=CARTESIAN_POINT('Ctrl Pts',(-18.6989197228858,-1.78046367084787,
-338.)) ;
#49717=CARTESIAN_POINT('Ctrl Pts',(-18.7019205354198,-1.73959432655047,
-338.)) ;
#49718=CARTESIAN_POINT('Ctrl Pts',(-18.7047857659883,-1.69870898034511,
-338.)) ;
#49719=CARTESIAN_POINT('Ctrl Pts',(-18.7075141594755,-1.65782261116247,
-338.)) ;
#49720=CARTESIAN_POINT('Ctrl Pts',(-18.7147395803788,-1.54954599053089,
-338.)) ;
#49721=CARTESIAN_POINT('Ctrl Pts',(-18.721007273306,-1.44123695536378,-338.)) ;
#49722=CARTESIAN_POINT('Ctrl Pts',(-18.7263137442602,-1.33290715643541,
-338.)) ;
#49723=CARTESIAN_POINT('Ctrl Pts',(-18.7457439791969,-0.936245521609726,
-338.)) ;
#49724=CARTESIAN_POINT('Ctrl Pts',(-18.752290839866,-0.539305802993233,
-338.)) ;
#49725=CARTESIAN_POINT('Ctrl Pts',(-18.746150022536,-0.142677068484718,
-338.)) ;
#49726=CARTESIAN_POINT('Ctrl Pts',(-18.7399765659379,0.256059800969821,
-338.)) ;
#49727=CARTESIAN_POINT('Ctrl Pts',(-18.7209801146579,0.654482919550263,
-338.)) ;
#49728=CARTESIAN_POINT('Ctrl Pts',(-18.6893065939024,1.05199317238646,-338.)) ;
#49729=CARTESIAN_POINT('Ctrl Pts',(-18.6576201367373,1.44966578025454,-338.)) ;
#49730=CARTESIAN_POINT('Ctrl Pts',(-18.6132461326084,1.84642532793274,-338.)) ;
#49731=CARTESIAN_POINT('Ctrl Pts',(-18.5562794787259,2.24166310101432,-338.)) ;
#49732=CARTESIAN_POINT('Ctrl Pts',(-18.5221279800155,2.47860807456891,-338.)) ;
#49733=CARTESIAN_POINT('Ctrl Pts',(-18.483449708919,2.71500591409569,-338.)) ;
#49734=CARTESIAN_POINT('Ctrl Pts',(-18.4402565595206,2.95072268342921,-338.)) ;
#49735=CARTESIAN_POINT('Ctrl Pts',(-18.429993187445,3.00673269755961,-338.)) ;
#49736=CARTESIAN_POINT('Ctrl Pts',(-18.4194744473254,3.06270643984912,-338.)) ;
#49737=CARTESIAN_POINT('Ctrl Pts',(-18.4087018356681,3.11863490845468,-338.)) ;
#49738=CARTESIAN_POINT('Ctrl Pts',(-18.4018134016346,3.15439778368304,-338.)) ;
#49739=CARTESIAN_POINT('Ctrl Pts',(-18.3948215986383,3.19013989341542,-338.)) ;
#49740=CARTESIAN_POINT('Ctrl Pts',(-18.3877273514385,3.22585673647208,-338.)) ;
#49741=CARTESIAN_POINT('Ctrl Pts',(-18.3101159279799,3.61660080741016,-338.)) ;
#49742=CARTESIAN_POINT('Ctrl Pts',(-18.220212432157,4.00450434614193,-338.)) ;
#49743=CARTESIAN_POINT('Ctrl Pts',(-18.118173080588,4.38897607361206,-338.)) ;
#49744=CARTESIAN_POINT('Ctrl Pts',(-18.0163151528155,4.77276421852882,-338.)) ;
#49745=CARTESIAN_POINT('Ctrl Pts',(-17.9023643369644,5.15313328585193,-338.)) ;
#49746=CARTESIAN_POINT('Ctrl Pts',(-17.7764256451059,5.52948306809377,-338.)) ;
#49747=CARTESIAN_POINT('Ctrl Pts',(-17.651889804069,5.90164063114181,-338.)) ;
#49748=CARTESIAN_POINT('Ctrl Pts',(-17.5156314622654,6.26986843888553,-338.)) ;
#49749=CARTESIAN_POINT('Ctrl Pts',(-17.3677056193957,6.63356670882829,-338.)) ;
#49750=CARTESIAN_POINT('Ctrl Pts',(-17.2208939190367,6.99452568930165,-338.)) ;
#49751=CARTESIAN_POINT('Ctrl Pts',(-17.0625896473109,7.35102357559316,-338.)) ;
#49752=CARTESIAN_POINT('Ctrl Pts',(-16.8928031616867,7.70244771115104,-338.)) ;
#49753=CARTESIAN_POINT('',(-15.1169529804711,-10.7789097737449,-318.249803151889)) ;
#49754=CARTESIAN_POINT('Ctrl Pts',(-15.1172285295639,-10.7791107733297,
-318.25)) ;
#49755=CARTESIAN_POINT('Ctrl Pts',(-14.8934395929579,-11.1089469203127,
-318.25)) ;
#49756=CARTESIAN_POINT('Ctrl Pts',(-14.6593537074853,-11.431009438768,-318.25)) ;
#49757=CARTESIAN_POINT('Ctrl Pts',(-14.4152963237418,-11.7447716872223,
-318.25)) ;
#49758=CARTESIAN_POINT('Ctrl Pts',(-14.3474396575172,-11.8320087944987,
-318.25)) ;
#49759=CARTESIAN_POINT('Ctrl Pts',(-14.2788118621464,-11.918604159466,-318.25)) ;
#49760=CARTESIAN_POINT('Ctrl Pts',(-14.209419264857,-12.0045462090401,-318.25)) ;
#49761=CARTESIAN_POINT('Ctrl Pts',(-13.9621513090759,-12.3107851414901,
-318.25)) ;
#49762=CARTESIAN_POINT('Ctrl Pts',(-13.7051760626163,-12.6087308722331,
-318.25)) ;
#49763=CARTESIAN_POINT('Ctrl Pts',(-13.4390527258754,-12.8980992743919,
-318.25)) ;
#49764=CARTESIAN_POINT('Ctrl Pts',(-13.1707551578732,-13.1898318203108,
-318.25)) ;
#49765=CARTESIAN_POINT('Ctrl Pts',(-12.8931590317108,-13.4728466860606,
-318.25)) ;
#49766=CARTESIAN_POINT('Ctrl Pts',(-12.6067933865282,-13.7468220954629,
-318.25)) ;
#49767=CARTESIAN_POINT('Ctrl Pts',(-12.3195148583575,-14.0216708899748,
-318.25)) ;
#49768=CARTESIAN_POINT('Ctrl Pts',(-12.0234103896743,-14.2874228706985,
-318.25)) ;
#49769=CARTESIAN_POINT('Ctrl Pts',(-11.7189760896812,-14.5437169207685,
-318.25)) ;
#49770=CARTESIAN_POINT('Ctrl Pts',(-11.4152434420173,-14.7994202709167,
-318.25)) ;
#49771=CARTESIAN_POINT('Ctrl Pts',(-11.1032188665144,-15.0457095764132,
-318.25)) ;
#49772=CARTESIAN_POINT('Ctrl Pts',(-10.7833638518003,-15.2821849399938,
-318.25)) ;
#49773=CARTESIAN_POINT('Ctrl Pts',(-10.629871777717,-15.3956647741556,-318.25)) ;
#49774=CARTESIAN_POINT('Ctrl Pts',(-10.4745760517745,-15.5068839629755,
-318.25)) ;
#49775=CARTESIAN_POINT('Ctrl Pts',(-10.3175255756812,-15.615794572014,-318.25)) ;
#49776=CARTESIAN_POINT('Ctrl Pts',(-10.2483745954551,-15.6637490612928,
-318.25)) ;
#49777=CARTESIAN_POINT('Ctrl Pts',(-10.1788833998896,-15.7112559453889,
-318.25)) ;
#49778=CARTESIAN_POINT('Ctrl Pts',(-10.1090560916909,-15.7583109732571,
-318.25)) ;
#49779=CARTESIAN_POINT('Ctrl Pts',(-10.0638091334537,-15.7888018647969,
-318.25)) ;
#49780=CARTESIAN_POINT('Ctrl Pts',(-10.0184188268518,-15.8191044922151,
-318.25)) ;
#49781=CARTESIAN_POINT('Ctrl Pts',(-9.9728937426656,-15.8492127503619,-318.25)) ;
#49782=CARTESIAN_POINT('Ctrl Pts',(-9.92573156378842,-15.8804037098467,
-318.25)) ;
#49783=CARTESIAN_POINT('Ctrl Pts',(-9.87843774940729,-15.9113774836762,
-318.25)) ;
#49784=CARTESIAN_POINT('Ctrl Pts',(-9.8310174318769,-15.9421309678968,-318.25)) ;
#49785=CARTESIAN_POINT('Ctrl Pts',(-9.49504077518283,-16.1600218076937,
-318.25)) ;
#49786=CARTESIAN_POINT('Ctrl Pts',(-9.15264811101595,-16.3669028052293,
-318.25)) ;
#49787=CARTESIAN_POINT('Ctrl Pts',(-8.80438953721077,-16.5624759763278,
-318.25)) ;
#49788=CARTESIAN_POINT('Ctrl Pts',(-8.45495228619666,-16.7587110626145,
-318.25)) ;
#49789=CARTESIAN_POINT('Ctrl Pts',(-8.09960891386764,-16.9435620090313,
-318.25)) ;
#49790=CARTESIAN_POINT('Ctrl Pts',(-7.73887904347091,-17.1166898203253,
-318.25)) ;
#49791=CARTESIAN_POINT('Ctrl Pts',(-7.4327189837679,-17.2636275302069,-318.25)) ;
#49792=CARTESIAN_POINT('Ctrl Pts',(-7.12267810039724,-17.4021201630692,
-318.25)) ;
#49793=CARTESIAN_POINT('Ctrl Pts',(-6.80905734728888,-17.5319362137542,
-318.25)) ;
#49794=CARTESIAN_POINT('Ctrl Pts',(-6.44033603205845,-17.6845598665966,
-318.25)) ;
#49795=CARTESIAN_POINT('Ctrl Pts',(-6.0666666021044,-17.8251916385922,-318.25)) ;
#49796=CARTESIAN_POINT('Ctrl Pts',(-5.68866153394493,-17.9537870129653,
-318.25)) ;
#49797=CARTESIAN_POINT('Ctrl Pts',(-5.31000037174938,-18.0826055871452,
-318.25)) ;
#49798=CARTESIAN_POINT('Ctrl Pts',(-4.9269879640148,-18.1993460595037,-318.25)) ;
#49799=CARTESIAN_POINT('Ctrl Pts',(-4.54022430962917,-18.303913654081,-318.25)) ;
#49800=CARTESIAN_POINT('Ctrl Pts',(-4.25712592444706,-18.3804537240476,
-318.25)) ;
#49801=CARTESIAN_POINT('Ctrl Pts',(-3.97201735027695,-18.4504708252309,
-318.25)) ;
#49802=CARTESIAN_POINT('Ctrl Pts',(-3.68513114204395,-18.5139102951467,
-318.25)) ;
#49803=CARTESIAN_POINT('Ctrl Pts',(-3.60185362345996,-18.5323255465016,
-318.25)) ;
#49804=CARTESIAN_POINT('Ctrl Pts',(-3.51842630884418,-18.5501864512475,
-318.25)) ;
#49805=CARTESIAN_POINT('Ctrl Pts',(-3.43485487456654,-18.5674914340203,
-318.25)) ;
#49806=CARTESIAN_POINT('Ctrl Pts',(-3.37730934983001,-18.5794072797015,
-318.25)) ;
#49807=CARTESIAN_POINT('Ctrl Pts',(-3.31969462818924,-18.5910597081359,
-318.25)) ;
#49808=CARTESIAN_POINT('Ctrl Pts',(-3.26201522493554,-18.6024476502174,
-318.25)) ;
#49809=CARTESIAN_POINT('Ctrl Pts',(-3.21756770865879,-18.611223152606,-318.25)) ;
#49810=CARTESIAN_POINT('Ctrl Pts',(-3.17308968396432,-18.6198400188813,
-318.25)) ;
#49811=CARTESIAN_POINT('Ctrl Pts',(-3.12859179875859,-18.6282963987947,
-318.25)) ;
#49812=CARTESIAN_POINT('Ctrl Pts',(-2.73549464914775,-18.7030005970865,
-318.25)) ;
#49813=CARTESIAN_POINT('Ctrl Pts',(-2.34060402666148,-18.7652327176257,
-318.25)) ;
#49814=CARTESIAN_POINT('Ctrl Pts',(-1.94454526365388,-18.8150157087449,
-318.25)) ;
#49815=CARTESIAN_POINT('Ctrl Pts',(-1.54434519916198,-18.8653192447789,
-318.25)) ;
#49816=CARTESIAN_POINT('Ctrl Pts',(-1.14295191666762,-18.9029121077673,
-318.25)) ;
#49817=CARTESIAN_POINT('Ctrl Pts',(-0.740991016366364,-18.9277686014751,
-318.25)) ;
#49818=CARTESIAN_POINT('Ctrl Pts',(-0.338804046011407,-18.9526390749228,
-318.25)) ;
#49819=CARTESIAN_POINT('Ctrl Pts',(0.063951739996451,-18.9647589382012,
-318.25)) ;
#49820=CARTESIAN_POINT('Ctrl Pts',(0.466660972673863,-18.9640515178069,
-318.25)) ;
#49821=CARTESIAN_POINT('Ctrl Pts',(0.866538636378975,-18.9633490714969,
-318.25)) ;
#49822=CARTESIAN_POINT('Ctrl Pts',(1.26637094916322,-18.9499991231767,-318.25)) ;
#49823=CARTESIAN_POINT('Ctrl Pts',(1.66555826598646,-18.923875599887,-318.25)) ;
#49824=CARTESIAN_POINT('Ctrl Pts',(1.92227833398459,-18.907075385069,-318.25)) ;
#49825=CARTESIAN_POINT('Ctrl Pts',(2.17873167516151,-18.8849911641002,-318.25)) ;
#49826=CARTESIAN_POINT('Ctrl Pts',(2.43475782264655,-18.8575780223985,-318.25)) ;
#49827=CARTESIAN_POINT('Ctrl Pts',(2.83508915706831,-18.8147138864268,-318.25)) ;
#49828=CARTESIAN_POINT('Ctrl Pts',(3.23437686538619,-18.758823143256,-318.25)) ;
#49829=CARTESIAN_POINT('Ctrl Pts',(3.63204670084311,-18.6900943991976,-318.25)) ;
#49830=CARTESIAN_POINT('Ctrl Pts',(3.72453243208256,-18.6741102143672,-318.25)) ;
#49831=CARTESIAN_POINT('Ctrl Pts',(3.81693059106408,-18.6574314297529,-318.25)) ;
#49832=CARTESIAN_POINT('Ctrl Pts',(3.90923382524985,-18.6400600347302,-318.25)) ;
#49833=CARTESIAN_POINT('Ctrl Pts',(3.96405242176188,-18.6297432186077,-318.25)) ;
#49834=CARTESIAN_POINT('Ctrl Pts',(4.01883753596892,-18.6191821067855,-318.25)) ;
#49835=CARTESIAN_POINT('Ctrl Pts',(4.07358761785632,-18.6083770923689,-318.25)) ;
#49836=CARTESIAN_POINT('Ctrl Pts',(4.11408126063228,-18.6003856085411,-318.25)) ;
#49837=CARTESIAN_POINT('Ctrl Pts',(4.15454833823327,-18.5922621474935,-318.25)) ;
#49838=CARTESIAN_POINT('Ctrl Pts',(4.19498041797789,-18.5840086585812,-318.25)) ;
#49839=CARTESIAN_POINT('Ctrl Pts',(4.5873287012649,-18.5039177449713,-318.25)) ;
#49840=CARTESIAN_POINT('Ctrl Pts',(4.97661118933657,-18.41154179864,-318.25)) ;
#49841=CARTESIAN_POINT('Ctrl Pts',(5.36229079546034,-18.3072214478284,-318.25)) ;
#49842=CARTESIAN_POINT('Ctrl Pts',(5.75194592399491,-18.2018257798727,-318.25)) ;
#49843=CARTESIAN_POINT('Ctrl Pts',(6.13792402250833,-18.0842380932291,-318.25)) ;
#49844=CARTESIAN_POINT('Ctrl Pts',(6.51967037800299,-17.9547561950956,-318.25)) ;
#49845=CARTESIAN_POINT('Ctrl Pts',(6.90358541881112,-17.8245387156349,-318.25)) ;
#49846=CARTESIAN_POINT('Ctrl Pts',(7.28322103399168,-17.6822913566917,-318.25)) ;
#49847=CARTESIAN_POINT('Ctrl Pts',(7.65800424636563,-17.5282651576925,-318.25)) ;
#49848=CARTESIAN_POINT('Ctrl Pts',(8.03220348541031,-17.3744789566154,-318.25)) ;
#49849=CARTESIAN_POINT('Ctrl Pts',(8.40156595799478,-17.2089503963534,-318.25)) ;
#49850=CARTESIAN_POINT('Ctrl Pts',(8.76550470726295,-17.0318804289941,-318.25)) ;
#49851=CARTESIAN_POINT('Ctrl Pts',(9.12717779683322,-16.8559127907754,-318.25)) ;
#49852=CARTESIAN_POINT('Ctrl Pts',(9.48349498176718,-16.6685467769557,-318.25)) ;
#49853=CARTESIAN_POINT('Ctrl Pts',(9.83385611329522,-16.4699344361079,-318.25)) ;
#49854=CARTESIAN_POINT('Ctrl Pts',(10.0813465717466,-16.3296373116064,-318.25)) ;
#49855=CARTESIAN_POINT('Ctrl Pts',(10.3258645793787,-16.1837275282184,-318.25)) ;
#49856=CARTESIAN_POINT('Ctrl Pts',(10.5671892199504,-16.032245835092,-318.25)) ;
#49857=CARTESIAN_POINT('Ctrl Pts',(10.6765018800387,-15.963629274466,-318.25)) ;
#49858=CARTESIAN_POINT('Ctrl Pts',(10.7851592047769,-15.8938693215666,-318.25)) ;
#49859=CARTESIAN_POINT('Ctrl Pts',(10.8931400466771,-15.8229690739819,-318.25)) ;
#49860=CARTESIAN_POINT('Ctrl Pts',(10.9341643065962,-15.7960325347398,-318.25)) ;
#49861=CARTESIAN_POINT('Ctrl Pts',(10.9750910749037,-15.7689312332667,-318.25)) ;
#49862=CARTESIAN_POINT('Ctrl Pts',(11.0159020260381,-15.741676964968,-318.25)) ;
#49863=CARTESIAN_POINT('Ctrl Pts',(11.1048166349595,-15.6822982310779,-318.25)) ;
#49864=CARTESIAN_POINT('Ctrl Pts',(11.193201856226,-15.6221801352337,-318.25)) ;
#49865=CARTESIAN_POINT('Ctrl Pts',(11.2810474222442,-15.5613272740523,-318.25)) ;
#49866=CARTESIAN_POINT('Ctrl Pts',(11.6127958778286,-15.3315166685784,-318.25)) ;
#49867=CARTESIAN_POINT('Ctrl Pts',(11.93684968069,-15.0912306318534,-318.25)) ;
#49868=CARTESIAN_POINT('Ctrl Pts',(12.2528839901575,-14.8410069253261,-318.25)) ;
#49869=CARTESIAN_POINT('Ctrl Pts',(12.5712207270902,-14.5889602460483,-318.25)) ;
#49870=CARTESIAN_POINT('Ctrl Pts',(12.8814210852045,-14.326830220857,-318.25)) ;
#49871=CARTESIAN_POINT('Ctrl Pts',(13.1831255705581,-14.0551207702151,-318.25)) ;
#49872=CARTESIAN_POINT('Ctrl Pts',(13.4861015156718,-13.7822662665505,-318.25)) ;
#49873=CARTESIAN_POINT('Ctrl Pts',(13.7805102252478,-13.4997510463041,-318.25)) ;
#49874=CARTESIAN_POINT('Ctrl Pts',(14.0659540990013,-13.2080450727856,-318.25)) ;
#49875=CARTESIAN_POINT('Ctrl Pts',(14.2780380061313,-12.9913084450785,-318.25)) ;
#49876=CARTESIAN_POINT('Ctrl Pts',(14.4851722654754,-12.7694972480152,-318.25)) ;
#49877=CARTESIAN_POINT('Ctrl Pts',(14.687179910341,-12.5427918149033,-318.25)) ;
#49878=CARTESIAN_POINT('Ctrl Pts',(14.7184668118549,-12.5076797251448,-318.25)) ;
#49879=CARTESIAN_POINT('Ctrl Pts',(14.7496291449813,-12.4724519303098,-318.25)) ;
#49880=CARTESIAN_POINT('Ctrl Pts',(14.7806583427305,-12.4371182641492,-318.25)) ;
#49881=CARTESIAN_POINT('Ctrl Pts',(15.0525159971116,-12.1275476564679,-318.25)) ;
#49882=CARTESIAN_POINT('Ctrl Pts',(15.3143205432749,-11.8096706771766,-318.25)) ;
#49883=CARTESIAN_POINT('Ctrl Pts',(15.5657126298465,-11.4840113666617,-318.25)) ;
#49884=CARTESIAN_POINT('Ctrl Pts',(15.8161453061597,-11.1595948990998,-318.25)) ;
#49885=CARTESIAN_POINT('Ctrl Pts',(16.0562445808496,-10.8274556378891,-318.25)) ;
#49886=CARTESIAN_POINT('Ctrl Pts',(16.2856173638454,-10.4880756432578,-318.25)) ;
#49887=CARTESIAN_POINT('Ctrl Pts',(16.5163082412145,-10.1467453960488,-318.25)) ;
#49888=CARTESIAN_POINT('Ctrl Pts',(16.7361494174162,-9.79809056298881,-318.25)) ;
#49889=CARTESIAN_POINT('Ctrl Pts',(16.9446986253785,-9.44256919289982,-318.25)) ;
#49890=CARTESIAN_POINT('Ctrl Pts',(17.1532478333407,-9.08704782281084,-318.25)) ;
#49891=CARTESIAN_POINT('Ctrl Pts',(17.3505054705389,-8.72465948814614,-318.25)) ;
#49892=CARTESIAN_POINT('Ctrl Pts',(17.5359809117574,-8.35583619169791,-318.25)) ;
#49893=CARTESIAN_POINT('Ctrl Pts',(-15.1166752930756,-10.7787117730376,
-318.249803151889)) ;
#49894=CARTESIAN_POINT('Ctrl Pts',(-15.1223425749755,-10.7707636562237,
-318.249868767926)) ;
#49895=CARTESIAN_POINT('Ctrl Pts',(-15.1280035883766,-10.7628110697536,
-318.249934383963)) ;
#49896=CARTESIAN_POINT('Ctrl Pts',(-15.1336583262364,-10.7548540235205,
-318.25)) ;
#49897=CARTESIAN_POINT('Ctrl Pts',(-15.8220589029561,11.2756047307133,-317.75179962416)) ;
#49898=CARTESIAN_POINT('Ctrl Pts',(-13.9462169600666,13.9078331685254,-317.791516068309)) ;
#49899=CARTESIAN_POINT('Ctrl Pts',(-8.85808512633525,18.2140200078628,-317.870930498241)) ;
#49900=CARTESIAN_POINT('Ctrl Pts',(0.938245705209947,20.23155285505,-317.990042913955)) ;
#49901=CARTESIAN_POINT('Ctrl Pts',(10.502550121817,17.3171363004613,-318.1091368713)) ;
#49902=CARTESIAN_POINT('Ctrl Pts',(17.5078290499764,10.1819492314241,-318.228230828646)) ;
#49903=CARTESIAN_POINT('Ctrl Pts',(20.2452775605918,0.564912754706648,-318.347324785991)) ;
#49904=CARTESIAN_POINT('Ctrl Pts',(18.048297052031,-9.18978081702363,-318.466418743337)) ;
#49905=CARTESIAN_POINT('Ctrl Pts',(11.4520790521312,-16.7045512834906,-318.585512700682)) ;
#49906=CARTESIAN_POINT('Ctrl Pts',(2.06455022100158,-20.1477034639439,-318.704606658028)) ;
#49907=CARTESIAN_POINT('Ctrl Pts',(-7.82622053472994,-18.68000717547,-318.823700615374)) ;
#49908=CARTESIAN_POINT('Ctrl Pts',(-15.809397178503,-12.6591964182232,-318.942794572719)) ;
#49909=CARTESIAN_POINT('Ctrl Pts',(-19.9391565068373,-3.55280184418553,
-319.061888530065)) ;
#49910=CARTESIAN_POINT('Ctrl Pts',(-19.2088924586792,6.4195621534048,-319.18098248741)) ;
#49911=CARTESIAN_POINT('Ctrl Pts',(-13.7966053168245,14.8272055077051,-319.300076444756)) ;
#49912=CARTESIAN_POINT('Ctrl Pts',(-5.02149786345424,19.6208281495811,-319.419170402102)) ;
#49913=CARTESIAN_POINT('Ctrl Pts',(4.97756197041771,19.6320201345031,-319.538264359447)) ;
#49914=CARTESIAN_POINT('Ctrl Pts',(13.7633783186503,14.8580535757075,-319.657358316793)) ;
#49915=CARTESIAN_POINT('Ctrl Pts',(19.1944737272763,6.46254719947798,-319.776452274138)) ;
#49916=CARTESIAN_POINT('Ctrl Pts',(19.9470592755585,-3.50815687829998,-319.895546231484)) ;
#49917=CARTESIAN_POINT('Ctrl Pts',(15.8376977971645,-12.623773869973,-320.014640188829)) ;
#49918=CARTESIAN_POINT('Ctrl Pts',(7.86801554435696,-18.6624400785269,-320.133734146175)) ;
#49919=CARTESIAN_POINT('Ctrl Pts',(-2.01943685201295,-20.152275630516,-320.252828103521)) ;
#49920=CARTESIAN_POINT('Ctrl Pts',(-11.4146665670295,-16.7301442145837,
-320.371922060866)) ;
#49921=CARTESIAN_POINT('Ctrl Pts',(-18.0276563934026,-9.23016485487467,
-320.491016018212)) ;
#49922=CARTESIAN_POINT('Ctrl Pts',(-20.2465393536469,0.51959838559575,-320.610109975557)) ;
#49923=CARTESIAN_POINT('Ctrl Pts',(-17.5304792666225,10.1427133926868,-320.729203932903)) ;
#49924=CARTESIAN_POINT('Ctrl Pts',(-10.5414955324265,17.2936176152543,-320.848297890248)) ;
#49925=CARTESIAN_POINT('Ctrl Pts',(-0.983100839741991,20.2293314526664,
-320.967391847594)) ;
#49926=CARTESIAN_POINT('Ctrl Pts',(8.81491735450798,18.2342965402073,-321.086485804939)) ;
#49927=CARTESIAN_POINT('Ctrl Pts',(16.4643651509713,11.7947877665687,-321.205579762285)) ;
#49928=CARTESIAN_POINT('Ctrl Pts',(20.1007466691207,2.48038739450463,-321.324673719631)) ;
#49929=CARTESIAN_POINT('Ctrl Pts',(18.8377210198965,-7.43858891588363,-321.443767676976)) ;
#49930=CARTESIAN_POINT('Ctrl Pts',(12.9831412905652,-15.5444646261037,-321.562861634322)) ;
#49931=CARTESIAN_POINT('Ctrl Pts',(3.96401764945386,-19.861492953899,-321.681955591667)) ;
#49932=CARTESIAN_POINT('Ctrl Pts',(-6.02130574547807,-19.3374304239844,
-321.801049549013)) ;
#49933=CARTESIAN_POINT('Ctrl Pts',(-14.5389807484402,-14.1000133716053,
-321.920143506359)) ;
#49934=CARTESIAN_POINT('Ctrl Pts',(-19.5128875691681,-5.4258231629833,-322.039237463704)) ;
#49935=CARTESIAN_POINT('Ctrl Pts',(-19.7306734961704,4.57087099691963,-322.15833142105)) ;
#49936=CARTESIAN_POINT('Ctrl Pts',(-15.1392548331411,13.45344942311,-322.277425378395)) ;
#49937=CARTESIAN_POINT('Ctrl Pts',(-6.85775565424215,19.0568498359428,-322.396519335741)) ;
#49938=CARTESIAN_POINT('Ctrl Pts',(3.09527034689612,20.0152851531671,-322.515613293086)) ;
#49939=CARTESIAN_POINT('Ctrl Pts',(12.2938472734718,16.095143910494,-322.634707250432)) ;
#49940=CARTESIAN_POINT('Ctrl Pts',(18.4958905668593,8.25193131465147,-322.753801207777)) ;
#49941=CARTESIAN_POINT('Ctrl Pts',(20.189698405024,-1.60262802831304,-322.872895165123)) ;
#49942=CARTESIAN_POINT('Ctrl Pts',(16.9624177532472,-11.0665587355458,-322.991989122469)) ;
#49943=CARTESIAN_POINT('Ctrl Pts',(9.60067421388661,-17.8330982423632,-323.111083079814)) ;
#49944=CARTESIAN_POINT('Ctrl Pts',(-0.101162100603281,-20.2529529825249,
-323.23017703716)) ;
#49945=CARTESIAN_POINT('Ctrl Pts',(-9.7783409071448,-17.7363014009861,-323.349270994505)) ;
#49946=CARTESIAN_POINT('Ctrl Pts',(-17.0721220064229,-10.8965585613429,
-323.468364951851)) ;
#49947=CARTESIAN_POINT('Ctrl Pts',(-20.2047006241534,-1.40086079654568,
-323.587458909197)) ;
#49948=CARTESIAN_POINT('Ctrl Pts',(-18.4125340728579,8.43628634523557,-323.706552866542)) ;
#49949=CARTESIAN_POINT('Ctrl Pts',(-12.1324495904037,16.2171515753931,-323.825646823888)) ;
#49950=CARTESIAN_POINT('Ctrl Pts',(-2.89517095693271,20.0452069935208,-323.944740781233)) ;
#49951=CARTESIAN_POINT('Ctrl Pts',(7.04778401636063,18.9873926262059,-324.063834738579)) ;
#49952=CARTESIAN_POINT('Ctrl Pts',(15.2728941706411,13.3015428404137,-324.182928695924)) ;
#49953=CARTESIAN_POINT('Ctrl Pts',(19.7753502166989,4.37354113846764,-324.30202265327)) ;
#49954=CARTESIAN_POINT('Ctrl Pts',(19.4577120551217,-5.62047861511239,-324.421116610615)) ;
#49955=CARTESIAN_POINT('Ctrl Pts',(14.3974016200832,-14.2445486019387,-324.54021056796)) ;
#49956=CARTESIAN_POINT('Ctrl Pts',(5.8278318600006,-19.3966160475101,-324.659304525307)) ;
#49957=CARTESIAN_POINT('Ctrl Pts',(-4.16222847464273,-19.820902916059,-324.778398482652)) ;
#49958=CARTESIAN_POINT('Ctrl Pts',(-13.1377766443113,-15.4139924460587,
-324.897492439998)) ;
#49959=CARTESIAN_POINT('Ctrl Pts',(-18.9110896873939,-7.25003621496531,
-325.016586397343)) ;
#49960=CARTESIAN_POINT('Ctrl Pts',(-20.0749655845643,2.6810623009403,-325.135680354689)) ;
#49961=CARTESIAN_POINT('Ctrl Pts',(-16.345718261549,11.9586718659317,-325.254774312035)) ;
#49962=CARTESIAN_POINT('Ctrl Pts',(-8.63232395510391,18.3214443048877,-325.37386826938)) ;
#49963=CARTESIAN_POINT('Ctrl Pts',(1.18513496908386,20.2185012646342,-325.492962226726)) ;
#49964=CARTESIAN_POINT('Ctrl Pts',(10.7137260786869,17.1874492521093,-325.612056184072)) ;
#49965=CARTESIAN_POINT('Ctrl Pts',(17.6309263179295,9.96708460156269,-325.731150141417)) ;
#49966=CARTESIAN_POINT('Ctrl Pts',(20.2507196900847,0.31731737515523,-325.850244098763)) ;
#49967=CARTESIAN_POINT('Ctrl Pts',(17.9345510889248,-9.40979359612691,-325.969338056107)) ;
#49968=CARTESIAN_POINT('Ctrl Pts',(11.2469693460007,-16.8433375200132,-326.088432013454)) ;
#49969=CARTESIAN_POINT('Ctrl Pts',(1.81802266116369,-20.171443475529,-326.207525970799)) ;
#49970=CARTESIAN_POINT('Ctrl Pts',(-8.05405349558649,-18.5829104440933,
-326.326619928145)) ;
#49971=CARTESIAN_POINT('Ctrl Pts',(-15.9630141486082,-12.4649315110151,
-326.44571388549)) ;
#49972=CARTESIAN_POINT('Ctrl Pts',(-19.98110909301,-3.30871843712862,-326.564807842836)) ;
#49973=CARTESIAN_POINT('Ctrl Pts',(-19.1289576374257,6.65397009224849,-326.683901800182)) ;
#49974=CARTESIAN_POINT('Ctrl Pts',(-13.614265347121,14.9948030110817,-326.802995757527)) ;
#49975=CARTESIAN_POINT('Ctrl Pts',(-4.78119736072094,19.6807644689122,-326.922089714873)) ;
#49976=CARTESIAN_POINT('Ctrl Pts',(5.21725184277175,19.5696862900778,-327.041183672218)) ;
#49977=CARTESIAN_POINT('Ctrl Pts',(13.944034799571,14.6886429526801,-327.160277629564)) ;
#49978=CARTESIAN_POINT('Ctrl Pts',(19.2720632143789,6.22735238636345,-327.279371586909)) ;
#49979=CARTESIAN_POINT('Ctrl Pts',(19.9026698768091,-3.75180890474398,-327.398465544254)) ;
#49980=CARTESIAN_POINT('Ctrl Pts',(15.6821491135074,-12.8164947417256,-327.5175595016)) ;
#49981=CARTESIAN_POINT('Ctrl Pts',(7.639221400292,-18.7572555210053,-327.636653458946)) ;
#49982=CARTESIAN_POINT('Ctrl Pts',(-2.26570958562885,-20.1260750857328,
-327.755747416291)) ;
#49983=CARTESIAN_POINT('Ctrl Pts',(-11.6183907489069,-16.5893138703406,
-327.874841373638)) ;
#49984=CARTESIAN_POINT('Ctrl Pts',(-18.1391757719305,-9.00903105766491,
-327.993935330983)) ;
#49985=CARTESIAN_POINT('Ctrl Pts',(-20.2386719120029,0.76713592098574,-328.113029288328)) ;
#49986=CARTESIAN_POINT('Ctrl Pts',(-17.4051426348618,10.3563192372135,-328.232123245674)) ;
#49987=CARTESIAN_POINT('Ctrl Pts',(-10.3292395803644,17.4212269365392,-328.351217203019)) ;
#49988=CARTESIAN_POINT('Ctrl Pts',(-0.735661373466894,20.2398404298689,
-328.470311160365)) ;
#49989=CARTESIAN_POINT('Ctrl Pts',(9.03722880951048,18.1251436884654,-328.589405117711)) ;
#49990=CARTESIAN_POINT('Ctrl Pts',(16.6073618346899,11.5925782798587,-328.708499075056)) ;
#49991=CARTESIAN_POINT('Ctrl Pts',(20.1295742058069,2.23440832791899,-328.827593032402)) ;
#49992=CARTESIAN_POINT('Ctrl Pts',(18.7453529123693,-7.66838199841982,-328.946686989747)) ;
#49993=CARTESIAN_POINT('Ctrl Pts',(12.7920915765111,-15.702061373626,-329.065780947093)) ;
#49994=CARTESIAN_POINT('Ctrl Pts',(3.72085327256795,-19.9084803339427,-329.18487490444)) ;
#49995=CARTESIAN_POINT('Ctrl Pts',(-6.25731528090481,-19.2623556129129,
-329.303968861784)) ;
#49996=CARTESIAN_POINT('Ctrl Pts',(-14.7103098773889,-13.9211752950014,
-329.42306281913)) ;
#49997=CARTESIAN_POINT('Ctrl Pts',(-19.5777760935643,-5.1868122689399,-329.542156776475)) ;
#49998=CARTESIAN_POINT('Ctrl Pts',(-19.6733053218788,4.81179758459352,-329.661250733821)) ;
#49999=CARTESIAN_POINT('Ctrl Pts',(-14.9736130250163,13.6375676445628,-329.780344691166)) ;
#50000=CARTESIAN_POINT('Ctrl Pts',(-6.6242141683021,19.1392822471332,-329.899438648512)) ;
#50001=CARTESIAN_POINT('Ctrl Pts',(3.33978751429805,19.975939468328,-330.018532605858)) ;
#50002=CARTESIAN_POINT('Ctrl Pts',(12.4897408854399,15.9436103470178,-330.137626563203)) ;
#50003=CARTESIAN_POINT('Ctrl Pts',(18.5954130156895,8.02514504908728,-330.256720520549)) ;
#50004=CARTESIAN_POINT('Ctrl Pts',(20.1685918356652,-1.84938953422425,-330.375814477894)) ;
#50005=CARTESIAN_POINT('Ctrl Pts',(16.8258267346502,-11.2731492041263,-330.49490843524)) ;
#50006=CARTESIAN_POINT('Ctrl Pts',(9.38189178866938,-17.9491627868451,-330.614002392586)) ;
#50007=CARTESIAN_POINT('Ctrl Pts',(-0.348809347122767,-20.2502017353488,
-330.733096349931)) ;
#50008=CARTESIAN_POINT('Ctrl Pts',(-9.99449080461785,-17.6154049581431,
-330.852190307277)) ;
#50009=CARTESIAN_POINT('Ctrl Pts',(-17.2040896285461,-10.6869845296003,
-330.971284264622)) ;
#50010=CARTESIAN_POINT('Ctrl Pts',(-20.2203198467357,-1.15369128395224,
-331.090378221968)) ;
#50011=CARTESIAN_POINT('Ctrl Pts',(-18.3079978268224,8.66080561241441,-331.209472179313)) ;
#50012=CARTESIAN_POINT('Ctrl Pts',(-11.9332378064965,16.3642956993744,-331.328566136659)) ;
#50013=CARTESIAN_POINT('Ctrl Pts',(-2.64984002253427,20.0791106909131,-331.447660094004)) ;
#50014=CARTESIAN_POINT('Ctrl Pts',(7.27943651471512,18.8997921234915,-331.56675405135)) ;
#50015=CARTESIAN_POINT('Ctrl Pts',(15.4344046632414,13.1137901071458,-331.685848008696)) ;
#50016=CARTESIAN_POINT('Ctrl Pts',(19.8273517248913,4.13139950384977,-331.804941966041)) ;
#50017=CARTESIAN_POINT('Ctrl Pts',(19.3875295989093,-5.85798893259291,-331.924035923387)) ;
#50018=CARTESIAN_POINT('Ctrl Pts',(14.2221416500197,-14.4195362328246,-332.043129880732)) ;
#50019=CARTESIAN_POINT('Ctrl Pts',(5.59021268738151,-19.4664290611504,-332.162223838078)) ;
#50020=CARTESIAN_POINT('Ctrl Pts',(-4.4042889477316,-19.768524910773,-332.281317795423)) ;
#50021=CARTESIAN_POINT('Ctrl Pts',(-13.3252779819004,-15.2521901702032,
-332.400411752769)) ;
#50022=CARTESIAN_POINT('Ctrl Pts',(-18.998329836102,-7.01824776718787,-332.519505710115)) ;
#50023=CARTESIAN_POINT('Ctrl Pts',(-20.0406804084418,2.92634021427114,-332.63859966746)) ;
#50024=CARTESIAN_POINT('Ctrl Pts',(-16.1982645167102,12.1576545817708,-332.757693624806)) ;
#50025=CARTESIAN_POINT('Ctrl Pts',(-8.4076423927164,18.4256312694888,-332.876787582151)) ;
#50026=CARTESIAN_POINT('Ctrl Pts',(1.43227989298982,20.2024976819972,-332.995881539497)) ;
#50027=CARTESIAN_POINT('Ctrl Pts',(10.9230946311552,17.0551558762091,-333.114975496841)) ;
#50028=CARTESIAN_POINT('Ctrl Pts',(17.7514864749526,9.75074695664578,-333.234069454188)) ;
#50029=CARTESIAN_POINT('Ctrl Pts',(20.2530858120576,0.0696661495647872,
-333.353163411534)) ;
#50030=CARTESIAN_POINT('Ctrl Pts',(17.8181464512536,-9.62839526217338,-333.472257368879)) ;
#50031=CARTESIAN_POINT('Ctrl Pts',(11.0401667114247,-16.9796070998983,-333.591351326225)) ;
#50032=CARTESIAN_POINT('Ctrl Pts',(1.57122863033052,-20.1921662749243,-333.71044528357)) ;
#50033=CARTESIAN_POINT('Ctrl Pts',(-8.28068471729155,-18.4830354351167,
-333.829539240916)) ;
#50034=CARTESIAN_POINT('Ctrl Pts',(-16.1142428902293,-12.2688024826247,
-333.948633198262)) ;
#50035=CARTESIAN_POINT('Ctrl Pts',(-20.0200744760529,-3.06414037802701,
-334.067727155607)) ;
#50036=CARTESIAN_POINT('Ctrl Pts',(-19.0461621402262,6.88738310326793,-334.186821112953)) ;
#50037=CARTESIAN_POINT('Ctrl Pts',(-13.4298897549544,15.1601582924693,-334.305915070298)) ;
#50038=CARTESIAN_POINT('Ctrl Pts',(-4.54018184982169,19.7377579034077,-334.425009027644)) ;
#50039=CARTESIAN_POINT('Ctrl Pts',(5.45616153817922,19.5044261528559,-334.544102984989)) ;
#50040=CARTESIAN_POINT('Ctrl Pts',(14.1226062220899,14.5170359157374,-334.663196942335)) ;
#50041=CARTESIAN_POINT('Ctrl Pts',(19.3467709108636,5.99122638576585,-334.78229089968)) ;
#50042=CARTESIAN_POINT('Ctrl Pts',(19.8553044031172,-3.99489991643816,-334.901384857026)) ;
#50043=CARTESIAN_POINT('Ctrl Pts',(15.5242554507918,-13.0072991424903,-335.020478814372)) ;
#50044=CARTESIAN_POINT('Ctrl Pts',(7.40928495186548,-18.8492661603349,-335.139572771717)) ;
#50045=CARTESIAN_POINT('Ctrl Pts',(-2.51164352439901,-20.0968650563489,
-335.258666729063)) ;
#50046=CARTESIAN_POINT('Ctrl Pts',(-11.8203776137382,-16.4460028987553,
-335.377760686408)) ;
#50047=CARTESIAN_POINT('Ctrl Pts',(-18.2479827700008,-8.78655012580679,
-335.496854643754)) ;
#50048=CARTESIAN_POINT('Ctrl Pts',(-20.2277781489081,1.0145587461582,-335.6159486011)) ;
#50049=CARTESIAN_POINT('Ctrl Pts',(-17.277203383498,10.5683764826849,-335.735042558445)) ;
#50050=CARTESIAN_POINT('Ctrl Pts',(-10.115439080935,17.5462312370861,-335.854136515791)) ;
#50051=CARTESIAN_POINT('Ctrl Pts',(-0.488111901202637,20.2473229031516,
-335.973230473135)) ;
#50052=CARTESIAN_POINT('Ctrl Pts',(9.25818891017889,18.0132805702995,-336.092324430482)) ;
#50053=CARTESIAN_POINT('Ctrl Pts',(16.7478751983631,11.3886353032719,-336.211418387827)) ;
#50054=CARTESIAN_POINT('Ctrl Pts',(20.1553917224645,1.98809521454014,-336.330512345173)) ;
#50055=CARTESIAN_POINT('Ctrl Pts',(18.6501818066376,-7.89702855606564,-336.449606302519)) ;
#50056=CARTESIAN_POINT('Ctrl Pts',(12.5991289885161,-15.8573098746684,-336.568700259864)) ;
#50057=CARTESIAN_POINT('Ctrl Pts',(3.47713261749939,-19.9524913709672,-336.68779421721)) ;
#50058=CARTESIAN_POINT('Ctrl Pts',(-6.49238937166023,-19.1843992178428,
-336.806888174555)) ;
#50059=CARTESIAN_POINT('Ctrl Pts',(-14.8794388899768,-13.7402581581745,
-336.925982131901)) ;
#50060=CARTESIAN_POINT('Ctrl Pts',(-19.6397380740326,-4.94702040317705,
-337.045076089246)) ;
#50061=CARTESIAN_POINT('Ctrl Pts',(-19.6129933917417,5.05199350895541,-337.164170046592)) ;
#50062=CARTESIAN_POINT('Ctrl Pts',(-14.8057362800649,13.8196697192246,-337.283264003938)) ;
#50063=CARTESIAN_POINT('Ctrl Pts',(-6.38967367544487,19.2188048600104,-337.402357961283)) ;
#50064=CARTESIAN_POINT('Ctrl Pts',(3.58378767615178,19.933705979741,-337.521451918629)) ;
#50065=CARTESIAN_POINT('Ctrl Pts',(12.6838030107157,15.7894873221202,-337.640545875974)) ;
#50066=CARTESIAN_POINT('Ctrl Pts',(18.6920739072665,7.79758994659989,-337.75963983332)) ;
#50067=CARTESIAN_POINT('Ctrl Pts',(20.1448670002182,-2.09864690139803,-337.878756758576)) ;
#50068=CARTESIAN_POINT('Ctrl Pts',(17.8370731701076,-8.35261194983006,-337.958175698051)) ;
#50069=CARTESIAN_POINT('Ctrl Pts',(16.0042781108101,-11.015438797673,-337.997896651744)) ;
#50070=CARTESIAN_POINT('Ctrl Pts',(-15.5872995250709,11.1083032456097,-317.918234548891)) ;
#50071=CARTESIAN_POINT('Ctrl Pts',(-13.7392903370854,13.7014760640297,-317.957950993041)) ;
#50072=CARTESIAN_POINT('Ctrl Pts',(-8.72665352402181,17.943769970743,-318.037365422973)) ;
#50073=CARTESIAN_POINT('Ctrl Pts',(0.924324509529332,19.9313677280047,-318.156477838686)) ;
#50074=CARTESIAN_POINT('Ctrl Pts',(10.346718813899,17.0601937514806,-318.275571796032)) ;
#50075=CARTESIAN_POINT('Ctrl Pts',(17.2480571023999,10.0308748306847,-318.394665753377)) ;
#50076=CARTESIAN_POINT('Ctrl Pts',(19.9448887935932,0.556530876743228,-318.513759710723)) ;
#50077=CARTESIAN_POINT('Ctrl Pts',(17.7805059248579,-9.05342768872738,-318.632853668069)) ;
#50078=CARTESIAN_POINT('Ctrl Pts',(11.28215913398,-16.4566979483958,-318.751947625414)) ;
#50079=CARTESIAN_POINT('Ctrl Pts',(2.03391751204327,-19.8487624500075,-318.871041582759)) ;
#50080=CARTESIAN_POINT('Ctrl Pts',(-7.71009919583251,-18.4028430661526,
-318.990135540105)) ;
#50081=CARTESIAN_POINT('Ctrl Pts',(-15.5748256686173,-12.471365928279,-319.109229497451)) ;
#50082=CARTESIAN_POINT('Ctrl Pts',(-19.6433098028266,-3.50008724137647,
-319.228323454796)) ;
#50083=CARTESIAN_POINT('Ctrl Pts',(-18.9238810280478,6.32431207080355,-319.347417412142)) ;
#50084=CARTESIAN_POINT('Ctrl Pts',(-13.5918985526182,14.6072072405951,-319.466511369487)) ;
#50085=CARTESIAN_POINT('Ctrl Pts',(-4.94699152254709,19.3297046340993,-319.585605326833)) ;
#50086=CARTESIAN_POINT('Ctrl Pts',(4.90370752715424,19.3407305582428,-319.704699284178)) ;
#50087=CARTESIAN_POINT('Ctrl Pts',(13.5591645591451,14.6375976012094,-319.823793241524)) ;
#50088=CARTESIAN_POINT('Ctrl Pts',(18.9096762341886,6.36665932739958,-319.94288719887)) ;
#50089=CARTESIAN_POINT('Ctrl Pts',(19.6510953144271,-3.45610469398413,-320.061981156216)) ;
#50090=CARTESIAN_POINT('Ctrl Pts',(15.6027063776026,-12.4364689611457,-320.181075113561)) ;
#50091=CARTESIAN_POINT('Ctrl Pts',(7.75127407311647,-18.3855366205428,-320.300169070907)) ;
#50092=CARTESIAN_POINT('Ctrl Pts',(-1.9894735114664,-19.8532667771799,-320.419263028252)) ;
#50093=CARTESIAN_POINT('Ctrl Pts',(-11.2453017556306,-16.481911145055,-320.538356985598)) ;
#50094=CARTESIAN_POINT('Ctrl Pts',(-17.7601715214524,-9.09321252949154,
-320.657450942943)) ;
#50095=CARTESIAN_POINT('Ctrl Pts',(-19.9461318648274,0.511888858378053,
-320.776544900289)) ;
#50096=CARTESIAN_POINT('Ctrl Pts',(-17.2703712470592,9.99222115266052,-320.895638857634)) ;
#50097=CARTESIAN_POINT('Ctrl Pts',(-10.3850863730149,17.0370240241393,-321.01473281498)) ;
#50098=CARTESIAN_POINT('Ctrl Pts',(-0.968514107196489,19.9291792856197,
-321.133826772326)) ;
#50099=CARTESIAN_POINT('Ctrl Pts',(8.68412625286022,17.9637456505785,-321.252920729671)) ;
#50100=CARTESIAN_POINT('Ctrl Pts',(16.2200755712257,11.6197829169879,-321.372014687017)) ;
#50101=CARTESIAN_POINT('Ctrl Pts',(19.8025023753778,2.44358471255154,-321.491108644362)) ;
#50102=CARTESIAN_POINT('Ctrl Pts',(18.5582168356097,-7.32821905081441,-321.610202601708)) ;
#50103=CARTESIAN_POINT('Ctrl Pts',(12.790504277199,-15.3138240459134,-321.729296559053)) ;
#50104=CARTESIAN_POINT('Ctrl Pts',(3.9052016430782,-19.5667985807883,-321.848390516399)) ;
#50105=CARTESIAN_POINT('Ctrl Pts',(-5.93196478173024,-19.0505118147137,
-321.967484473744)) ;
#50106=CARTESIAN_POINT('Ctrl Pts',(-14.3232590085248,-13.890804798461,-322.08657843109)) ;
#50107=CARTESIAN_POINT('Ctrl Pts',(-19.2233656191755,-5.34531765620506,
-322.205672388436)) ;
#50108=CARTESIAN_POINT('Ctrl Pts',(-19.4379201532821,4.50305082015176,-322.324766345781)) ;
#50109=CARTESIAN_POINT('Ctrl Pts',(-14.9146265424696,13.253834225344,-322.443860303127)) ;
#50110=CARTESIAN_POINT('Ctrl Pts',(-6.75600388723424,18.7740943336799,-322.562954260472)) ;
#50111=CARTESIAN_POINT('Ctrl Pts',(3.04934435550142,19.7183088923925,-322.682048217818)) ;
#50112=CARTESIAN_POINT('Ctrl Pts',(12.1114376417395,15.8563326410773,-322.801142175163)) ;
#50113=CARTESIAN_POINT('Ctrl Pts',(18.2214582828222,8.12949350338674,-322.920236132509)) ;
#50114=CARTESIAN_POINT('Ctrl Pts',(19.890134292267,-1.57884907759523,-323.039330089855)) ;
#50115=CARTESIAN_POINT('Ctrl Pts',(16.7107383312702,-10.902358964832,-323.1584240472)) ;
#50116=CARTESIAN_POINT('Ctrl Pts',(9.45822446574986,-17.5685001218012,-323.277518004546)) ;
#50117=CARTESIAN_POINT('Ctrl Pts',(-0.0996611106279288,-19.9524503316576,
-323.396611961891)) ;
#50118=CARTESIAN_POINT('Ctrl Pts',(-9.63325503417527,-17.473139500982,-323.515705919237)) ;
#50119=CARTESIAN_POINT('Ctrl Pts',(-16.8188148505092,-10.7348811636893,
-323.634799876582)) ;
#50120=CARTESIAN_POINT('Ctrl Pts',(-19.9049139163692,-1.38007556175934,
-323.753893833928)) ;
#50121=CARTESIAN_POINT('Ctrl Pts',(-18.1393385885821,8.31111317111102,-323.872987791274)) ;
#50122=CARTESIAN_POINT('Ctrl Pts',(-11.9524346924985,15.9765300204956,-323.992081748619)) ;
#50123=CARTESIAN_POINT('Ctrl Pts',(-2.85221393491113,19.7477867682365,-324.111175705965)) ;
#50124=CARTESIAN_POINT('Ctrl Pts',(6.94321270858724,18.7056676934439,-324.23026966331)) ;
#50125=CARTESIAN_POINT('Ctrl Pts',(15.046283009856,13.1041815525256,-324.349363620656)) ;
#50126=CARTESIAN_POINT('Ctrl Pts',(19.4819339841588,4.30864883822279,-324.468457578002)) ;
#50127=CARTESIAN_POINT('Ctrl Pts',(19.1690087703503,-5.53708491324378,-324.587551535347)) ;
#50128=CARTESIAN_POINT('Ctrl Pts',(14.1837805567168,-14.033195491161,-324.706645492693)) ;
#50129=CARTESIAN_POINT('Ctrl Pts',(5.74136155987941,-19.1088192731257,-324.825739450038)) ;
#50130=CARTESIAN_POINT('Ctrl Pts',(-4.10047152042356,-19.5268107965543,
-324.944833407384)) ;
#50131=CARTESIAN_POINT('Ctrl Pts',(-12.9428452329993,-15.1852877433674,
-325.06392736473)) ;
#50132=CARTESIAN_POINT('Ctrl Pts',(-18.6304968974559,-7.14246399557781,
-325.183021322075)) ;
#50133=CARTESIAN_POINT('Ctrl Pts',(-19.7771038169774,2.64128211040375,-325.30211527942)) ;
#50134=CARTESIAN_POINT('Ctrl Pts',(-16.1031891018673,11.7812353903884,-325.421209236766)) ;
#50135=CARTESIAN_POINT('Ctrl Pts',(-8.50424207816021,18.0496003626199,-325.540303194112)) ;
#50136=CARTESIAN_POINT('Ctrl Pts',(1.1675505605212,19.9185097902143,-325.659397151457)) ;
#50137=CARTESIAN_POINT('Ctrl Pts',(10.554761453129,16.9324309312569,-325.778491108803)) ;
#50138=CARTESIAN_POINT('Ctrl Pts',(17.3693279179155,9.81919824905043,-325.897585066149)) ;
#50139=CARTESIAN_POINT('Ctrl Pts',(19.9502501756347,0.312609187046404,-326.016679023494)) ;
#50140=CARTESIAN_POINT('Ctrl Pts',(17.668447664452,-9.27017603407612,-326.13577298084)) ;
#50141=CARTESIAN_POINT('Ctrl Pts',(11.0800927376556,-16.5934249478277,-326.254866938185)) ;
#50142=CARTESIAN_POINT('Ctrl Pts',(1.7910477983134,-19.8721502198024,-326.373960895531)) ;
#50143=CARTESIAN_POINT('Ctrl Pts',(-7.93455169119587,-18.3071870049437,
-326.493054852876)) ;
#50144=CARTESIAN_POINT('Ctrl Pts',(-15.726163351017,-12.2799834214614,-326.612148810222)) ;
#50145=CARTESIAN_POINT('Ctrl Pts',(-19.6846399186186,-3.25962541537577,
-326.731242767567)) ;
#50146=CARTESIAN_POINT('Ctrl Pts',(-18.8451322375774,6.55524198809318,-326.850336724913)) ;
#50147=CARTESIAN_POINT('Ctrl Pts',(-13.4122640473623,14.7723180204756,-326.969430682259)) ;
#50148=CARTESIAN_POINT('Ctrl Pts',(-4.71025647212775,19.3887516498875,-327.088524639604)) ;
#50149=CARTESIAN_POINT('Ctrl Pts',(5.13984100740629,19.2793215905752,-327.20761859695)) ;
#50150=CARTESIAN_POINT('Ctrl Pts',(13.7371405543381,14.4707006037923,-327.326712554295)) ;
#50151=CARTESIAN_POINT('Ctrl Pts',(18.9861144893412,6.13495421106516,-327.445806511641)) ;
#50152=CARTESIAN_POINT('Ctrl Pts',(19.6073645422006,-3.69614153997029,-327.564900468986)) ;
#50153=CARTESIAN_POINT('Ctrl Pts',(15.4494656433997,-12.6263303420928,-327.683994426332)) ;
#50154=CARTESIAN_POINT('Ctrl Pts',(7.52587465607497,-18.4789452414169,-327.803088383677)) ;
#50155=CARTESIAN_POINT('Ctrl Pts',(-2.23209217995158,-19.8274549822824,
-327.922182341023)) ;
#50156=CARTESIAN_POINT('Ctrl Pts',(-11.4460031853812,-16.3431703672965,
-328.041276298369)) ;
#50157=CARTESIAN_POINT('Ctrl Pts',(-17.8700362341696,-8.87535979911265,
-328.160370255714)) ;
#50158=CARTESIAN_POINT('Ctrl Pts',(-19.9383811561395,0.755753562174654,
-328.27946421306)) ;
#50159=CARTESIAN_POINT('Ctrl Pts',(-17.1468942942365,10.2026576261539,-328.398558170406)) ;
#50160=CARTESIAN_POINT('Ctrl Pts',(-10.1759797629925,17.1627399455159,-328.517652127751)) ;
#50161=CARTESIAN_POINT('Ctrl Pts',(-0.724746017416909,19.9395323361526,
-328.636746085097)) ;
#50162=CARTESIAN_POINT('Ctrl Pts',(8.9031391675657,17.8562123513694,-328.755840042442)) ;
#50163=CARTESIAN_POINT('Ctrl Pts',(16.3609505454551,11.4205737081554,-328.874933999788)) ;
#50164=CARTESIAN_POINT('Ctrl Pts',(19.8309021842556,2.20125535381989,-328.994027957133)) ;
#50165=CARTESIAN_POINT('Ctrl Pts',(18.4672192374198,-7.55460258460419,-329.113121914479)) ;
#50166=CARTESIAN_POINT('Ctrl Pts',(12.6022892581927,-15.4690824558886,-329.232215871825)) ;
#50167=CARTESIAN_POINT('Ctrl Pts',(3.66564521116278,-19.613088786831,-329.35130982917)) ;
#50168=CARTESIAN_POINT('Ctrl Pts',(-6.16447253195624,-18.9765509241537,
-329.470403786516)) ;
#50169=CARTESIAN_POINT('Ctrl Pts',(-14.4920460460825,-13.7146202270592,
-329.589497743861)) ;
#50170=CARTESIAN_POINT('Ctrl Pts',(-19.2872913618179,-5.10985307994102,
-329.708591701207)) ;
#50171=CARTESIAN_POINT('Ctrl Pts',(-19.3814031777496,4.74040266599305,-329.827685658552)) ;
#50172=CARTESIAN_POINT('Ctrl Pts',(-14.7514424402645,13.435220597586,-329.946779615898)) ;
#50173=CARTESIAN_POINT('Ctrl Pts',(-6.52592756687639,18.8553036561632,-330.065873573244)) ;
#50174=CARTESIAN_POINT('Ctrl Pts',(3.29023350593959,19.6795469981051,-330.184967530589)) ;
#50175=CARTESIAN_POINT('Ctrl Pts',(12.3044246874535,15.7070474528163,-330.304061487935)) ;
#50176=CARTESIAN_POINT('Ctrl Pts',(18.3195040699664,7.90607217300219,-330.42315544528)) ;
#50177=CARTESIAN_POINT('Ctrl Pts',(19.8693408910694,-1.82194926622977,-330.542249402626)) ;
#50178=CARTESIAN_POINT('Ctrl Pts',(16.5761739782765,-11.1058841528331,-330.661343359971)) ;
#50179=CARTESIAN_POINT('Ctrl Pts',(9.24268821894413,-17.6828425616933,-330.780437317317)) ;
#50180=CARTESIAN_POINT('Ctrl Pts',(-0.343633897718047,-19.9497399060383,
-330.899531274662)) ;
#50181=CARTESIAN_POINT('Ctrl Pts',(-9.84619781329718,-17.3540368558921,
-331.018625232008)) ;
#50182=CARTESIAN_POINT('Ctrl Pts',(-16.9488244065513,-10.5284166810652,
-331.137719189353)) ;
#50183=CARTESIAN_POINT('Ctrl Pts',(-19.9203013891524,-1.13657342023086,
-331.256813146699)) ;
#50184=CARTESIAN_POINT('Ctrl Pts',(-18.0363533963149,8.53230113963843,-331.375907104045)) ;
#50185=CARTESIAN_POINT('Ctrl Pts',(-11.7561787081332,16.1214908974534,-331.49500106139)) ;
#50186=CARTESIAN_POINT('Ctrl Pts',(-2.61052309172258,19.7811874204209,-331.614095018736)) ;
#50187=CARTESIAN_POINT('Ctrl Pts',(7.17142806916257,18.6193669608572,-331.733188976082)) ;
#50188=CARTESIAN_POINT('Ctrl Pts',(15.205397094821,12.9192145954406,-331.852282933427)) ;
#50189=CARTESIAN_POINT('Ctrl Pts',(19.5331639213574,4.07009997366421,-331.971376890773)) ;
#50190=CARTESIAN_POINT('Ctrl Pts',(19.099867644464,-5.77107117770977,-332.090470848118)) ;
#50191=CARTESIAN_POINT('Ctrl Pts',(14.0111210017947,-14.2055867477309,-332.209564805464)) ;
#50192=CARTESIAN_POINT('Ctrl Pts',(5.50726805541008,-19.1775964380341,-332.328658762809)) ;
#50193=CARTESIAN_POINT('Ctrl Pts',(-4.33894042768517,-19.4752099485278,
-332.447752720155)) ;
#50194=CARTESIAN_POINT('Ctrl Pts',(-13.1275645244822,-15.0258862044737,
-332.5668466775)) ;
#50195=CARTESIAN_POINT('Ctrl Pts',(-18.7164426227795,-6.91411470272545,
-332.685940634846)) ;
#50196=CARTESIAN_POINT('Ctrl Pts',(-19.7433273462431,2.88292071922338,-332.805034592191)) ;
#50197=CARTESIAN_POINT('Ctrl Pts',(-15.9579231980432,11.9772657054768,-332.924128549537)) ;
#50198=CARTESIAN_POINT('Ctrl Pts',(-8.28289422247497,18.1522414559064,-333.043222506883)) ;
#50199=CARTESIAN_POINT('Ctrl Pts',(1.41102847819622,19.9027436603086,-333.162316464228)) ;
#50200=CARTESIAN_POINT('Ctrl Pts',(10.7610235052721,16.8021004548008,-333.281410421574)) ;
#50201=CARTESIAN_POINT('Ctrl Pts',(17.4880992668176,9.60607050818238,-333.40050437892)) ;
#50202=CARTESIAN_POINT('Ctrl Pts',(19.9525811903357,0.0686324799246863,
-333.519598336265)) ;
#50203=CARTESIAN_POINT('Ctrl Pts',(17.5537701774943,-9.4855342037205,-333.638692293611)) ;
#50204=CARTESIAN_POINT('Ctrl Pts',(10.8763585316662,-16.7276726314479,-333.757786250956)) ;
#50205=CARTESIAN_POINT('Ctrl Pts',(1.54791556734456,-19.8925655452134,-333.876880208302)) ;
#50206=CARTESIAN_POINT('Ctrl Pts',(-8.15782027818043,-18.2087938887545,
-333.995974165647)) ;
#50207=CARTESIAN_POINT('Ctrl Pts',(-15.8751482402092,-12.0867644523099,
-334.115068122993)) ;
#50208=CARTESIAN_POINT('Ctrl Pts',(-19.7230271538277,-3.01867627671687,
-334.234162080338)) ;
#50209=CARTESIAN_POINT('Ctrl Pts',(-18.7635652163641,6.78519173977364,-334.353256037684)) ;
#50210=CARTESIAN_POINT('Ctrl Pts',(-13.2306241231376,14.9352198472764,-334.472349995029)) ;
#50211=CARTESIAN_POINT('Ctrl Pts',(-4.47281702245709,19.4448994458156,-334.591443952375)) ;
#50212=CARTESIAN_POINT('Ctrl Pts',(5.37520588656649,19.2150297489026,-334.710537909721)) ;
#50213=CARTESIAN_POINT('Ctrl Pts',(13.913062428128,14.3016397816933,-334.829631867067)) ;
#50214=CARTESIAN_POINT('Ctrl Pts',(19.0597137123676,5.9023317237172,-334.948725824412)) ;
#50215=CARTESIAN_POINT('Ctrl Pts',(19.5607018524639,-3.93562569524808,-335.067819781758)) ;
#50216=CARTESIAN_POINT('Ctrl Pts',(15.2939147237023,-12.8143036876392,-335.186913739103)) ;
#50217=CARTESIAN_POINT('Ctrl Pts',(7.29934988358244,-18.5695906753343,-335.306007696449)) ;
#50218=CARTESIAN_POINT('Ctrl Pts',(-2.4743770804505,-19.7986783559321,-335.425101653794)) ;
#50219=CARTESIAN_POINT('Ctrl Pts',(-11.6449930754812,-16.201985768438,-335.54419561114)) ;
#50220=CARTESIAN_POINT('Ctrl Pts',(-17.9772288113016,-8.65617992215987,
-335.663289568485)) ;
#50221=CARTESIAN_POINT('Ctrl Pts',(-19.9276490289647,0.999505257763509,
-335.782383525831)) ;
#50222=CARTESIAN_POINT('Ctrl Pts',(-17.0208533381099,10.4115684778892,-335.901477483176)) ;
#50223=CARTESIAN_POINT('Ctrl Pts',(-9.96535152278336,17.2858894980803,-336.020571440522)) ;
#50224=CARTESIAN_POINT('Ctrl Pts',(-0.480869553859103,19.9469037884372,
-336.139665397868)) ;
#50225=CARTESIAN_POINT('Ctrl Pts',(9.12082077862105,17.7460089992421,-336.258759355213)) ;
#50226=CARTESIAN_POINT('Ctrl Pts',(16.4993790458345,11.2196567300561,-336.377853312559)) ;
#50227=CARTESIAN_POINT('Ctrl Pts',(19.8563366341969,1.95859690470542,-336.496947269905)) ;
#50228=CARTESIAN_POINT('Ctrl Pts',(18.3734602304366,-7.77985660503612,-336.61604122725)) ;
#50229=CARTESIAN_POINT('Ctrl Pts',(12.4121897474615,-15.6220274614286,-336.735135184596)) ;
#50230=CARTESIAN_POINT('Ctrl Pts',(3.42554075482743,-19.6564468112649,-336.854229141941)) ;
#50231=CARTESIAN_POINT('Ctrl Pts',(-6.39605871714633,-18.8997512050206,
-336.973323099287)) ;
#50232=CARTESIAN_POINT('Ctrl Pts',(-14.6586656114475,-13.536387443435,-337.092417056632)) ;
#50233=CARTESIAN_POINT('Ctrl Pts',(-19.3483339830501,-4.87361911960462,
-337.211511013978)) ;
#50234=CARTESIAN_POINT('Ctrl Pts',(-19.3219861242708,4.97703468971977,-337.330604971323)) ;
#50235=CARTESIAN_POINT('Ctrl Pts',(-14.5860565620484,13.6146207375616,-337.449698928669)) ;
#50236=CARTESIAN_POINT('Ctrl Pts',(-6.29486706233985,18.9336463543882,-337.568792886015)) ;
#50237=CARTESIAN_POINT('Ctrl Pts',(3.53061332188562,19.637940147781,-337.68788684336)) ;
#50238=CARTESIAN_POINT('Ctrl Pts',(12.4956074211102,15.5552112241988,-337.806980800706)) ;
#50239=CARTESIAN_POINT('Ctrl Pts',(18.4147307581373,7.68189341329181,-337.926074758051)) ;
#50240=CARTESIAN_POINT('Ctrl Pts',(19.8459680722369,-2.06750828385183,-338.045191683308)) ;
#50241=CARTESIAN_POINT('Ctrl Pts',(17.572416071661,-8.22868029232043,-338.124610622782)) ;
#50242=CARTESIAN_POINT('Ctrl Pts',(15.7668150602779,-10.8519975176768,-338.164331576474)) ;
#50243=CARTESIAN_POINT('Ctrl Pts',(-15.3525401471856,10.941001760506,-318.084669473621)) ;
#50244=CARTESIAN_POINT('Ctrl Pts',(-13.5323637141043,13.495118959534,-318.124385917771)) ;
#50245=CARTESIAN_POINT('Ctrl Pts',(-8.59522192170838,17.6735199336233,-318.203800347703)) ;
#50246=CARTESIAN_POINT('Ctrl Pts',(0.910403313848723,19.6311826009593,-318.322912763417)) ;
#50247=CARTESIAN_POINT('Ctrl Pts',(10.1908875059808,16.8032512024997,-318.442006720762)) ;
#50248=CARTESIAN_POINT('Ctrl Pts',(16.9882851548233,9.87980042994526,-318.561100678108)) ;
#50249=CARTESIAN_POINT('Ctrl Pts',(19.6445000265946,0.54814899877979,-318.680194635453)) ;
#50250=CARTESIAN_POINT('Ctrl Pts',(17.5127147976847,-8.91707456043111,-318.799288592799)) ;
#50251=CARTESIAN_POINT('Ctrl Pts',(11.1122392158291,-16.2088446133011,-318.918382550144)) ;
#50252=CARTESIAN_POINT('Ctrl Pts',(2.00328480308495,-19.5498214360711,-319.037476507491)) ;
#50253=CARTESIAN_POINT('Ctrl Pts',(-7.59397785693506,-18.1256789568353,
-319.156570464836)) ;
#50254=CARTESIAN_POINT('Ctrl Pts',(-15.3402541587318,-12.2835354383347,
-319.275664422181)) ;
#50255=CARTESIAN_POINT('Ctrl Pts',(-19.347463098816,-3.44737263856742,-319.394758379528)) ;
#50256=CARTESIAN_POINT('Ctrl Pts',(-18.6388695974165,6.22906198820229,-319.513852336872)) ;
#50257=CARTESIAN_POINT('Ctrl Pts',(-13.3871917884119,14.3872089734848,-319.632946294218)) ;
#50258=CARTESIAN_POINT('Ctrl Pts',(-4.8724851816399,19.0385811186175,-319.752040251563)) ;
#50259=CARTESIAN_POINT('Ctrl Pts',(4.82985308389071,19.0494409819826,-319.871134208909)) ;
#50260=CARTESIAN_POINT('Ctrl Pts',(13.35495079964,14.4171416267112,-319.990228166255)) ;
#50261=CARTESIAN_POINT('Ctrl Pts',(18.6248787411007,6.27077145532118,-320.109322123601)) ;
#50262=CARTESIAN_POINT('Ctrl Pts',(19.3551313532961,-3.40405250966826,-320.228416080946)) ;
#50263=CARTESIAN_POINT('Ctrl Pts',(15.3677149580408,-12.2491640523184,-320.347510038291)) ;
#50264=CARTESIAN_POINT('Ctrl Pts',(7.63453260187597,-18.1086331625589,-320.466603995637)) ;
#50265=CARTESIAN_POINT('Ctrl Pts',(-1.95951017091986,-19.5542579238435,
-320.585697952983)) ;
#50266=CARTESIAN_POINT('Ctrl Pts',(-11.0759369442315,-16.2336780755262,
-320.704791910328)) ;
#50267=CARTESIAN_POINT('Ctrl Pts',(-17.4926866495024,-8.95626020410841,
-320.823885867674)) ;
#50268=CARTESIAN_POINT('Ctrl Pts',(-19.6457243760081,0.50417933116037,-320.94297982502)) ;
#50269=CARTESIAN_POINT('Ctrl Pts',(-17.0102632274958,9.84172891263414,-321.062073782365)) ;
#50270=CARTESIAN_POINT('Ctrl Pts',(-10.2286772136034,16.7804304330243,-321.18116773971)) ;
#50271=CARTESIAN_POINT('Ctrl Pts',(-0.953927374650981,19.629027118573,-321.300261697056)) ;
#50272=CARTESIAN_POINT('Ctrl Pts',(8.55333515121244,17.6931947609498,-321.419355654403)) ;
#50273=CARTESIAN_POINT('Ctrl Pts',(15.9757859914798,11.4447780674072,-321.538449611747)) ;
#50274=CARTESIAN_POINT('Ctrl Pts',(19.5042580816349,2.40678203059845,-321.657543569093)) ;
#50275=CARTESIAN_POINT('Ctrl Pts',(18.2787126513231,-7.21784918574521,-321.776637526438)) ;
#50276=CARTESIAN_POINT('Ctrl Pts',(12.5978672638328,-15.0831834657231,-321.895731483785)) ;
#50277=CARTESIAN_POINT('Ctrl Pts',(3.84638563670257,-19.2721042076775,-322.01482544113)) ;
#50278=CARTESIAN_POINT('Ctrl Pts',(-5.84262381798243,-18.7635932054432,
-322.133919398475)) ;
#50279=CARTESIAN_POINT('Ctrl Pts',(-14.1075372686095,-13.6815962253168,
-322.253013355821)) ;
#50280=CARTESIAN_POINT('Ctrl Pts',(-18.9338436691828,-5.26481214942683,
-322.372107313166)) ;
#50281=CARTESIAN_POINT('Ctrl Pts',(-19.1451668103936,4.4352306433839,-322.491201270511)) ;
#50282=CARTESIAN_POINT('Ctrl Pts',(-14.6899982517982,13.054219027578,-322.610295227857)) ;
#50283=CARTESIAN_POINT('Ctrl Pts',(-6.65425212022631,18.4913388314171,-322.729389185204)) ;
#50284=CARTESIAN_POINT('Ctrl Pts',(3.00341836410673,19.4213326316182,-322.848483142548)) ;
#50285=CARTESIAN_POINT('Ctrl Pts',(11.9290280100071,15.6175213716606,-322.967577099894)) ;
#50286=CARTESIAN_POINT('Ctrl Pts',(17.947025998785,8.00705569212202,-323.08667105724)) ;
#50287=CARTESIAN_POINT('Ctrl Pts',(19.5905701795099,-1.5550701268774,-323.205765014586)) ;
#50288=CARTESIAN_POINT('Ctrl Pts',(16.4590589092933,-10.7381591941182,-323.324858971931)) ;
#50289=CARTESIAN_POINT('Ctrl Pts',(9.3157747176131,-17.3039020012393,-323.443952929276)) ;
#50290=CARTESIAN_POINT('Ctrl Pts',(-0.0981601206525683,-19.6519476807905,
-323.563046886622)) ;
#50291=CARTESIAN_POINT('Ctrl Pts',(-9.48816916120576,-17.2099776009777,
-323.682140843967)) ;
#50292=CARTESIAN_POINT('Ctrl Pts',(-16.5655076945953,-10.5732037660358,
-323.801234801313)) ;
#50293=CARTESIAN_POINT('Ctrl Pts',(-19.6051272085852,-1.359290326973,-323.920328758658)) ;
#50294=CARTESIAN_POINT('Ctrl Pts',(-17.8661431043062,8.18593999698645,-324.039422716004)) ;
#50295=CARTESIAN_POINT('Ctrl Pts',(-11.7724197945931,15.7359084655981,-324.158516673351)) ;
#50296=CARTESIAN_POINT('Ctrl Pts',(-2.80925691288954,19.4503665429521,-324.277610630695)) ;
#50297=CARTESIAN_POINT('Ctrl Pts',(6.83864140081385,18.423942760682,-324.396704588041)) ;
#50298=CARTESIAN_POINT('Ctrl Pts',(14.8196718490712,12.9068202646376,-324.515798545386)) ;
#50299=CARTESIAN_POINT('Ctrl Pts',(19.1885177516185,4.24375653797794,-324.634892502732)) ;
#50300=CARTESIAN_POINT('Ctrl Pts',(18.8803054855788,-5.45369121137518,-324.753986460077)) ;
#50301=CARTESIAN_POINT('Ctrl Pts',(13.9701594933504,-13.8218423803834,-324.873080417423)) ;
#50302=CARTESIAN_POINT('Ctrl Pts',(5.65489125975822,-18.8210224987411,-324.992174374769)) ;
#50303=CARTESIAN_POINT('Ctrl Pts',(-4.03871456620437,-19.2327186770497,
-325.111268332114)) ;
#50304=CARTESIAN_POINT('Ctrl Pts',(-12.7479138216875,-14.9565830406762,
-325.23036228946)) ;
#50305=CARTESIAN_POINT('Ctrl Pts',(-18.3499041075179,-7.03489177619029,
-325.349456246805)) ;
#50306=CARTESIAN_POINT('Ctrl Pts',(-19.4792420493903,2.60150191986722,-325.468550204151)) ;
#50307=CARTESIAN_POINT('Ctrl Pts',(-15.8606599421856,11.6037989148451,-325.587644161497)) ;
#50308=CARTESIAN_POINT('Ctrl Pts',(-8.37616020121653,17.7777564203519,-325.706738118843)) ;
#50309=CARTESIAN_POINT('Ctrl Pts',(1.14996615195856,19.6185183157945,-325.825832076188)) ;
#50310=CARTESIAN_POINT('Ctrl Pts',(10.3957968275708,16.6774126104045,-325.944926033533)) ;
#50311=CARTESIAN_POINT('Ctrl Pts',(17.1077295179018,9.67131189653814,-326.064019990879)) ;
#50312=CARTESIAN_POINT('Ctrl Pts',(19.6497806611846,0.307900998937585,-326.183113948225)) ;
#50313=CARTESIAN_POINT('Ctrl Pts',(17.4023442399792,-9.13055847202533,-326.30220790557)) ;
#50314=CARTESIAN_POINT('Ctrl Pts',(10.9132161293105,-16.3435123756421,-326.421301862916)) ;
#50315=CARTESIAN_POINT('Ctrl Pts',(1.76407293546312,-19.572856964076,-326.540395820261)) ;
#50316=CARTESIAN_POINT('Ctrl Pts',(-7.81504988680526,-18.0314635657939,
-326.659489777608)) ;
#50317=CARTESIAN_POINT('Ctrl Pts',(-15.4893125534258,-12.0950353319077,
-326.778583734953)) ;
#50318=CARTESIAN_POINT('Ctrl Pts',(-19.3881707442273,-3.21053239362289,
-326.897677692298)) ;
#50319=CARTESIAN_POINT('Ctrl Pts',(-18.561306837729,6.45651388393782,-327.016771649644)) ;
#50320=CARTESIAN_POINT('Ctrl Pts',(-13.2102627476037,14.5498330298696,-327.135865606989)) ;
#50321=CARTESIAN_POINT('Ctrl Pts',(-4.63931558353454,19.0967388308628,-327.254959564336)) ;
#50322=CARTESIAN_POINT('Ctrl Pts',(5.06243017204084,18.9889568910727,-327.37405352168)) ;
#50323=CARTESIAN_POINT('Ctrl Pts',(13.5302463091053,14.2527582549047,-327.493147479025)) ;
#50324=CARTESIAN_POINT('Ctrl Pts',(18.7001657643034,6.04255603576688,-327.612241436371)) ;
#50325=CARTESIAN_POINT('Ctrl Pts',(19.3120592075919,-3.64047417519661,-327.731335393717)) ;
#50326=CARTESIAN_POINT('Ctrl Pts',(15.2167821732917,-12.4361659424599,-327.850429351062)) ;
#50327=CARTESIAN_POINT('Ctrl Pts',(7.41252791185793,-18.2006349618286,-327.969523308408)) ;
#50328=CARTESIAN_POINT('Ctrl Pts',(-2.19847477427431,-19.5288348788321,
-328.088617265753)) ;
#50329=CARTESIAN_POINT('Ctrl Pts',(-11.2736156218556,-16.0970268642526,
-328.2077112231)) ;
#50330=CARTESIAN_POINT('Ctrl Pts',(-17.6008966964085,-8.74168854056036,
-328.326805180445)) ;
#50331=CARTESIAN_POINT('Ctrl Pts',(-19.638090400276,0.744371203363559,-328.44589913779)) ;
#50332=CARTESIAN_POINT('Ctrl Pts',(-16.8886459536112,10.0489960150942,-328.564993095137)) ;
#50333=CARTESIAN_POINT('Ctrl Pts',(-10.0227199456207,16.9042529544926,-328.684087052482)) ;
#50334=CARTESIAN_POINT('Ctrl Pts',(-0.713830661366919,19.6392242424365,
-328.803181009827)) ;
#50335=CARTESIAN_POINT('Ctrl Pts',(8.76904952562091,17.5872810142733,-328.922274967172)) ;
#50336=CARTESIAN_POINT('Ctrl Pts',(16.1145392562203,11.2485691364523,-329.041368924519)) ;
#50337=CARTESIAN_POINT('Ctrl Pts',(19.5322301627044,2.1681023797208,-329.160462881865)) ;
#50338=CARTESIAN_POINT('Ctrl Pts',(18.1890855624703,-7.44082317078855,-329.27955683921)) ;
#50339=CARTESIAN_POINT('Ctrl Pts',(12.4124869398741,-15.2361035381512,-329.398650796555)) ;
#50340=CARTESIAN_POINT('Ctrl Pts',(3.6104371497576,-19.3176972397194,-329.517744753901)) ;
#50341=CARTESIAN_POINT('Ctrl Pts',(-6.07162978300767,-18.6907462353942,
-329.636838711246)) ;
#50342=CARTESIAN_POINT('Ctrl Pts',(-14.2737822147762,-13.5080651591169,
-329.755932668592)) ;
#50343=CARTESIAN_POINT('Ctrl Pts',(-18.9968066300715,-5.03289389094214,
-329.875026625937)) ;
#50344=CARTESIAN_POINT('Ctrl Pts',(-19.0895010336205,4.66900774739259,-329.994120583283)) ;
#50345=CARTESIAN_POINT('Ctrl Pts',(-14.5292718555126,13.2328735506094,-330.113214540628)) ;
#50346=CARTESIAN_POINT('Ctrl Pts',(-6.42764096545065,18.5713250651932,-330.232308497974)) ;
#50347=CARTESIAN_POINT('Ctrl Pts',(3.24067949758114,19.3831545278824,-330.351402455319)) ;
#50348=CARTESIAN_POINT('Ctrl Pts',(12.119108489467,15.4704845586147,-330.470496412665)) ;
#50349=CARTESIAN_POINT('Ctrl Pts',(18.0435951242435,7.78699929691711,-330.58959037001)) ;
#50350=CARTESIAN_POINT('Ctrl Pts',(19.5700899464735,-1.79450899823529,-330.708684327357)) ;
#50351=CARTESIAN_POINT('Ctrl Pts',(16.3265212219027,-10.9386191015399,-330.827778284703)) ;
#50352=CARTESIAN_POINT('Ctrl Pts',(9.10348464921888,-17.4165223365414,-330.946872242047)) ;
#50353=CARTESIAN_POINT('Ctrl Pts',(-0.338458448313333,-19.6492780767278,
-331.065966199393)) ;
#50354=CARTESIAN_POINT('Ctrl Pts',(-9.69790482197649,-17.092668753641,-331.185060156739)) ;
#50355=CARTESIAN_POINT('Ctrl Pts',(-16.6935591845564,-10.3698488325299,
-331.304154114084)) ;
#50356=CARTESIAN_POINT('Ctrl Pts',(-19.6202829315688,-1.11945555650946,
-331.42324807143)) ;
#50357=CARTESIAN_POINT('Ctrl Pts',(-17.7647089658075,8.40379666686245,-331.542342028775)) ;
#50358=CARTESIAN_POINT('Ctrl Pts',(-11.5791196097698,15.8786860955325,-331.661435986121)) ;
#50359=CARTESIAN_POINT('Ctrl Pts',(-2.5712061609109,19.4832641499289,-331.780529943466)) ;
#50360=CARTESIAN_POINT('Ctrl Pts',(7.06341962361002,18.3389417982231,-331.899623900812)) ;
#50361=CARTESIAN_POINT('Ctrl Pts',(14.9763895264006,12.7246390837355,-332.018717858158)) ;
#50362=CARTESIAN_POINT('Ctrl Pts',(19.2389761178233,4.00880044347866,-332.137811815503)) ;
#50363=CARTESIAN_POINT('Ctrl Pts',(18.812205690019,-5.68415342282663,-332.256905772849)) ;
#50364=CARTESIAN_POINT('Ctrl Pts',(13.8001003535698,-13.9916372626369,-332.375999730194)) ;
#50365=CARTESIAN_POINT('Ctrl Pts',(5.42432342343864,-18.8887638149177,-332.49509368754)) ;
#50366=CARTESIAN_POINT('Ctrl Pts',(-4.27359190763872,-19.1818949862827,
-332.614187644887)) ;
#50367=CARTESIAN_POINT('Ctrl Pts',(-12.9298510670639,-14.7995822387444,
-332.73328160223)) ;
#50368=CARTESIAN_POINT('Ctrl Pts',(-18.4345554094567,-6.80998163826303,
-332.852375559577)) ;
#50369=CARTESIAN_POINT('Ctrl Pts',(-19.4459742840444,2.8395012241756,-332.971469516922)) ;
#50370=CARTESIAN_POINT('Ctrl Pts',(-15.7175818793762,11.796876829183,-333.090563474269)) ;
#50371=CARTESIAN_POINT('Ctrl Pts',(-8.15814605223354,17.8788516423241,-333.209657431613)) ;
#50372=CARTESIAN_POINT('Ctrl Pts',(1.38977706340263,19.6029896386202,-333.328751388959)) ;
#50373=CARTESIAN_POINT('Ctrl Pts',(10.598952379389,16.5490450333925,-333.447845346304)) ;
#50374=CARTESIAN_POINT('Ctrl Pts',(17.2247120586825,9.46139405971896,-333.56693930365)) ;
#50375=CARTESIAN_POINT('Ctrl Pts',(19.6520765686137,0.0675988102845867,
-333.686033260995)) ;
#50376=CARTESIAN_POINT('Ctrl Pts',(17.289393903735,-9.34267314526759,-333.805127218341)) ;
#50377=CARTESIAN_POINT('Ctrl Pts',(10.7125503519078,-16.4757381629974,-333.924221175687)) ;
#50378=CARTESIAN_POINT('Ctrl Pts',(1.5246025043586,-19.5929648155023,-334.043315133034)) ;
#50379=CARTESIAN_POINT('Ctrl Pts',(-8.03495583906933,-17.9345523423925,
-334.162409090378)) ;
#50380=CARTESIAN_POINT('Ctrl Pts',(-15.6360535901888,-11.9047264219953,
-334.281503047724)) ;
#50381=CARTESIAN_POINT('Ctrl Pts',(-19.4259798316024,-2.97321217540674,
-334.40059700507)) ;
#50382=CARTESIAN_POINT('Ctrl Pts',(-18.4809682925019,6.68300037627936,-334.519690962415)) ;
#50383=CARTESIAN_POINT('Ctrl Pts',(-13.0313584913207,14.7102814020834,-334.63878491976)) ;
#50384=CARTESIAN_POINT('Ctrl Pts',(-4.40545219509248,19.1520409882234,-334.757878877106)) ;
#50385=CARTESIAN_POINT('Ctrl Pts',(5.29425023495375,18.9256333449493,-334.876972834452)) ;
#50386=CARTESIAN_POINT('Ctrl Pts',(13.703518634166,14.086243647649,-334.996066791797)) ;
#50387=CARTESIAN_POINT('Ctrl Pts',(18.7726565138715,5.81343706166854,-335.115160749142)) ;
#50388=CARTESIAN_POINT('Ctrl Pts',(19.2660993018105,-3.876351474058,-335.234254706488)) ;
#50389=CARTESIAN_POINT('Ctrl Pts',(15.0635739966129,-12.621308232788,-335.353348663833)) ;
#50390=CARTESIAN_POINT('Ctrl Pts',(7.1894148152994,-18.2899151903336,-335.472442621179)) ;
#50391=CARTESIAN_POINT('Ctrl Pts',(-2.43711063650199,-19.5004916555153,
-335.591536578526)) ;
#50392=CARTESIAN_POINT('Ctrl Pts',(-11.4696085372243,-15.9579686381207,
-335.71063053587)) ;
#50393=CARTESIAN_POINT('Ctrl Pts',(-17.7064748526026,-8.52580971851293,
-335.829724493216)) ;
#50394=CARTESIAN_POINT('Ctrl Pts',(-19.6275199090212,0.984451769368805,
-335.948818450561)) ;
#50395=CARTESIAN_POINT('Ctrl Pts',(-16.7645032927217,10.2547604730937,-336.067912407907)) ;
#50396=CARTESIAN_POINT('Ctrl Pts',(-9.81526396463168,17.0255477590744,-336.187006365253)) ;
#50397=CARTESIAN_POINT('Ctrl Pts',(-0.473627206515563,19.6464846737229,
-336.306100322598)) ;
#50398=CARTESIAN_POINT('Ctrl Pts',(8.98345264706321,17.4787374281848,-336.425194279944)) ;
#50399=CARTESIAN_POINT('Ctrl Pts',(16.2508828933058,11.0506781568403,-336.544288237289)) ;
#50400=CARTESIAN_POINT('Ctrl Pts',(19.5572815459293,1.92909859487072,-336.663382194636)) ;
#50401=CARTESIAN_POINT('Ctrl Pts',(18.0967386542354,-7.66268465400661,-336.78247615198)) ;
#50402=CARTESIAN_POINT('Ctrl Pts',(12.2252505064069,-15.3867450481888,-336.901570109326)) ;
#50403=CARTESIAN_POINT('Ctrl Pts',(3.37394889215548,-19.3604022515627,-337.020664066672)) ;
#50404=CARTESIAN_POINT('Ctrl Pts',(-6.29972806263244,-18.6151031921984,
-337.139758024018)) ;
#50405=CARTESIAN_POINT('Ctrl Pts',(-14.437892332918,-13.3325167286957,-337.258851981363)) ;
#50406=CARTESIAN_POINT('Ctrl Pts',(-19.0569298920675,-4.80021783603219,
-337.377945938708)) ;
#50407=CARTESIAN_POINT('Ctrl Pts',(-19.0309788568,4.90207587048415,-337.497039896054)) ;
#50408=CARTESIAN_POINT('Ctrl Pts',(-14.366376844032,13.4095717558985,-337.616133853399)) ;
#50409=CARTESIAN_POINT('Ctrl Pts',(-6.20006044923484,18.648487848766,-337.735227810745)) ;
#50410=CARTESIAN_POINT('Ctrl Pts',(3.47743896761947,19.3421743158212,-337.85432176809)) ;
#50411=CARTESIAN_POINT('Ctrl Pts',(12.3074118315047,15.3209351262774,-337.973415725436)) ;
#50412=CARTESIAN_POINT('Ctrl Pts',(18.137387609008,7.56619687998373,-338.092509682783)) ;
#50413=CARTESIAN_POINT('Ctrl Pts',(19.5470691442554,-2.03636966630564,-338.211626608038)) ;
#50414=CARTESIAN_POINT('Ctrl Pts',(17.3077589732144,-8.1047486348108,-338.291045547513)) ;
#50415=CARTESIAN_POINT('Ctrl Pts',(15.5293520097458,-10.6885562376806,-338.330766501206)) ;
#50416=CARTESIAN_POINT('Ctrl Pts',(-15.1177807693004,10.7737002754024,-318.251104398353)) ;
#50417=CARTESIAN_POINT('Ctrl Pts',(-13.325437091123,13.2887618550384,-318.290820842503)) ;
#50418=CARTESIAN_POINT('Ctrl Pts',(-8.46379031939493,17.4032698965035,-318.370235272435)) ;
#50419=CARTESIAN_POINT('Ctrl Pts',(0.89648211816811,19.3309974739139,-318.489347688148)) ;
#50420=CARTESIAN_POINT('Ctrl Pts',(10.0350561980626,16.546308653519,-318.608441645494)) ;
#50421=CARTESIAN_POINT('Ctrl Pts',(16.7285132072465,9.72872602920581,-318.727535602839)) ;
#50422=CARTESIAN_POINT('Ctrl Pts',(19.344111259596,0.539767120816376,-318.846629560185)) ;
#50423=CARTESIAN_POINT('Ctrl Pts',(17.2449236705115,-8.78072143213488,-318.96572351753)) ;
#50424=CARTESIAN_POINT('Ctrl Pts',(10.942319297678,-15.9609912782063,-319.084817474876)) ;
#50425=CARTESIAN_POINT('Ctrl Pts',(1.97265209412664,-19.2508804221347,-319.203911432221)) ;
#50426=CARTESIAN_POINT('Ctrl Pts',(-7.47785651803763,-17.8485148475178,
-319.323005389567)) ;
#50427=CARTESIAN_POINT('Ctrl Pts',(-15.1056826488461,-12.0957049483905,
-319.442099346912)) ;
#50428=CARTESIAN_POINT('Ctrl Pts',(-19.0516163948054,-3.39465803575837,
-319.561193304259)) ;
#50429=CARTESIAN_POINT('Ctrl Pts',(-18.3538581667854,6.13381190560104,-319.680287261603)) ;
#50430=CARTESIAN_POINT('Ctrl Pts',(-13.1824850242055,14.1672107063747,-319.79938121895)) ;
#50431=CARTESIAN_POINT('Ctrl Pts',(-4.79797884073275,18.7474576031358,-319.918475176295)) ;
#50432=CARTESIAN_POINT('Ctrl Pts',(4.75599864062722,18.7581514057224,-320.037569133641)) ;
#50433=CARTESIAN_POINT('Ctrl Pts',(13.1507370401348,14.1966856522131,-320.156663090986)) ;
#50434=CARTESIAN_POINT('Ctrl Pts',(18.3400812480129,6.17488358324277,-320.275757048331)) ;
#50435=CARTESIAN_POINT('Ctrl Pts',(19.0591673921649,-3.3520003253524,-320.394851005677)) ;
#50436=CARTESIAN_POINT('Ctrl Pts',(15.132723538479,-12.0618591434911,-320.513944963023)) ;
#50437=CARTESIAN_POINT('Ctrl Pts',(7.51779113063549,-17.8317297045749,-320.633038920368)) ;
#50438=CARTESIAN_POINT('Ctrl Pts',(-1.92954683037332,-19.2552490705074,
-320.752132877714)) ;
#50439=CARTESIAN_POINT('Ctrl Pts',(-10.9065721328326,-15.9854450059974,
-320.87122683506)) ;
#50440=CARTESIAN_POINT('Ctrl Pts',(-17.2252017775524,-8.81930787872528,
-320.990320792405)) ;
#50441=CARTESIAN_POINT('Ctrl Pts',(-19.3453168871886,0.496469803942675,
-321.109414749751)) ;
#50442=CARTESIAN_POINT('Ctrl Pts',(-16.7501552079325,9.69123667260777,-321.228508707096)) ;
#50443=CARTESIAN_POINT('Ctrl Pts',(-10.0722680541918,16.5238368419094,-321.347602664442)) ;
#50444=CARTESIAN_POINT('Ctrl Pts',(-0.939340642105482,19.3288749515264,
-321.466696621787)) ;
#50445=CARTESIAN_POINT('Ctrl Pts',(8.42254404956468,17.422643871321,-321.585790579133)) ;
#50446=CARTESIAN_POINT('Ctrl Pts',(15.7314964117339,11.2697732178267,-321.704884536478)) ;
#50447=CARTESIAN_POINT('Ctrl Pts',(19.2060137878919,2.36997934864535,-321.823978493824)) ;
#50448=CARTESIAN_POINT('Ctrl Pts',(17.9992084670363,-7.10747932067599,-321.94307245117)) ;
#50449=CARTESIAN_POINT('Ctrl Pts',(12.4052302504666,-14.8525428855328,-322.062166408515)) ;
#50450=CARTESIAN_POINT('Ctrl Pts',(3.7875696303269,-18.9774098345666,-322.181260365861)) ;
#50451=CARTESIAN_POINT('Ctrl Pts',(-5.75328285423461,-18.4766745961726,
-322.300354323206)) ;
#50452=CARTESIAN_POINT('Ctrl Pts',(-13.8918155286942,-13.4723876521726,
-322.419448280552)) ;
#50453=CARTESIAN_POINT('Ctrl Pts',(-18.6443217191903,-5.1843066426486,-322.538542237898)) ;
#50454=CARTESIAN_POINT('Ctrl Pts',(-18.8524134675053,4.36741046661603,-322.657636195243)) ;
#50455=CARTESIAN_POINT('Ctrl Pts',(-14.4653699611266,12.8546038298119,-322.776730152589)) ;
#50456=CARTESIAN_POINT('Ctrl Pts',(-6.55250035321841,18.2085833291542,-322.895824109934)) ;
#50457=CARTESIAN_POINT('Ctrl Pts',(2.95749237271203,19.1243563708438,-323.01491806728)) ;
#50458=CARTESIAN_POINT('Ctrl Pts',(11.7466183782748,15.3787101022439,-323.134012024625)) ;
#50459=CARTESIAN_POINT('Ctrl Pts',(17.6725937147479,7.8846178808573,-323.253105981971)) ;
#50460=CARTESIAN_POINT('Ctrl Pts',(19.2910060667529,-1.53129117615959,-323.372199939316)) ;
#50461=CARTESIAN_POINT('Ctrl Pts',(16.2073794873162,-10.5739594234043,-323.491293896662)) ;
#50462=CARTESIAN_POINT('Ctrl Pts',(9.17332496947635,-17.0393038806773,-323.610387854007)) ;
#50463=CARTESIAN_POINT('Ctrl Pts',(-0.0966591306772172,-19.3514450299231,
-323.729481811354)) ;
#50464=CARTESIAN_POINT('Ctrl Pts',(-9.34308328823623,-16.9468157009735,
-323.848575768699)) ;
#50465=CARTESIAN_POINT('Ctrl Pts',(-16.3122005386815,-10.4115263683823,
-323.967669726045)) ;
#50466=CARTESIAN_POINT('Ctrl Pts',(-19.3053405008011,-1.33850509218666,
-324.08676368339)) ;
#50467=CARTESIAN_POINT('Ctrl Pts',(-17.5929476200303,8.06076682286189,-324.205857640736)) ;
#50468=CARTESIAN_POINT('Ctrl Pts',(-11.5924048966878,15.4952869107006,-324.324951598081)) ;
#50469=CARTESIAN_POINT('Ctrl Pts',(-2.76629989086795,19.1529463176678,-324.444045555427)) ;
#50470=CARTESIAN_POINT('Ctrl Pts',(6.73407009304045,18.14221782792,-324.563139512772)) ;
#50471=CARTESIAN_POINT('Ctrl Pts',(14.5930606882862,12.7094589767493,-324.682233470118)) ;
#50472=CARTESIAN_POINT('Ctrl Pts',(18.8951015190783,4.17886423773308,-324.801327427463)) ;
#50473=CARTESIAN_POINT('Ctrl Pts',(18.5916022008074,-5.37029750950658,-324.920421384809)) ;
#50474=CARTESIAN_POINT('Ctrl Pts',(13.756538429984,-13.6104892696057,-325.039515342155)) ;
#50475=CARTESIAN_POINT('Ctrl Pts',(5.56842095963703,-18.5332257243567,-325.1586092995)) ;
#50476=CARTESIAN_POINT('Ctrl Pts',(-3.9769576119852,-18.9386265575451,-325.277703256846)) ;
#50477=CARTESIAN_POINT('Ctrl Pts',(-12.5529824103755,-14.7278783379849,
-325.396797214191)) ;
#50478=CARTESIAN_POINT('Ctrl Pts',(-18.0693113175798,-6.92731955680278,
-325.515891171537)) ;
#50479=CARTESIAN_POINT('Ctrl Pts',(-19.1813802818034,2.56172172933069,-325.634985128882)) ;
#50480=CARTESIAN_POINT('Ctrl Pts',(-15.6181307825039,11.4263624393018,-325.754079086228)) ;
#50481=CARTESIAN_POINT('Ctrl Pts',(-8.24807832427286,17.5059124780841,-325.873173043573)) ;
#50482=CARTESIAN_POINT('Ctrl Pts',(1.13238174339593,19.3185268413744,-325.992267000919)) ;
#50483=CARTESIAN_POINT('Ctrl Pts',(10.2368322020129,16.4223942895521,-326.111360958265)) ;
#50484=CARTESIAN_POINT('Ctrl Pts',(16.8461311178881,9.52342554402588,-326.23045491561)) ;
#50485=CARTESIAN_POINT('Ctrl Pts',(19.3493111467344,0.303192810828759,-326.349548872956)) ;
#50486=CARTESIAN_POINT('Ctrl Pts',(17.1362408155064,-8.99094090997454,-326.468642830301)) ;
#50487=CARTESIAN_POINT('Ctrl Pts',(10.7463395209654,-16.0935998034566,-326.587736787647)) ;
#50488=CARTESIAN_POINT('Ctrl Pts',(1.73709807261283,-19.2735637083494,-326.706830744992)) ;
#50489=CARTESIAN_POINT('Ctrl Pts',(-7.69554808241464,-17.7557401266443,
-326.825924702338)) ;
#50490=CARTESIAN_POINT('Ctrl Pts',(-15.2524617558346,-11.9100872423539,
-326.945018659683)) ;
#50491=CARTESIAN_POINT('Ctrl Pts',(-19.0917015698358,-3.16143937187002,
-327.064112617029)) ;
#50492=CARTESIAN_POINT('Ctrl Pts',(-18.2774814378808,6.35778577978252,-327.183206574375)) ;
#50493=CARTESIAN_POINT('Ctrl Pts',(-13.0082614478451,14.3273480392636,-327.302300531721)) ;
#50494=CARTESIAN_POINT('Ctrl Pts',(-4.56837469494134,18.8047260118381,-327.421394489066)) ;
#50495=CARTESIAN_POINT('Ctrl Pts',(4.98501933667539,18.6985921915703,-327.540488446412)) ;
#50496=CARTESIAN_POINT('Ctrl Pts',(13.3233520638725,14.0348159060169,-327.659582403757)) ;
#50497=CARTESIAN_POINT('Ctrl Pts',(18.4142170392658,5.95015786046861,-327.778676361102)) ;
#50498=CARTESIAN_POINT('Ctrl Pts',(19.0167538729834,-3.58480681042292,-327.897770318448)) ;
#50499=CARTESIAN_POINT('Ctrl Pts',(14.984098703184,-12.246001542827,-328.016864275794)) ;
#50500=CARTESIAN_POINT('Ctrl Pts',(7.29918116764088,-17.9223246822402,-328.13595823314)) ;
#50501=CARTESIAN_POINT('Ctrl Pts',(-2.16485736859702,-19.2302147753817,
-328.255052190485)) ;
#50502=CARTESIAN_POINT('Ctrl Pts',(-11.1012280583299,-15.8508833612084,
-328.374146147831)) ;
#50503=CARTESIAN_POINT('Ctrl Pts',(-17.3317571586476,-8.60801728200809,
-328.493240105176)) ;
#50504=CARTESIAN_POINT('Ctrl Pts',(-19.3377996444125,0.732988844552469,
-328.612334062522)) ;
#50505=CARTESIAN_POINT('Ctrl Pts',(-16.6303976129859,9.89533440403462,-328.731428019867)) ;
#50506=CARTESIAN_POINT('Ctrl Pts',(-9.86946012824876,16.6457659634692,-328.850521977213)) ;
#50507=CARTESIAN_POINT('Ctrl Pts',(-0.702915305316933,19.3389161487203,
-328.969615934558)) ;
#50508=CARTESIAN_POINT('Ctrl Pts',(8.63495988367612,17.3183496771772,-329.088709891904)) ;
#50509=CARTESIAN_POINT('Ctrl Pts',(15.8681279669855,11.076564564749,-329.20780384925)) ;
#50510=CARTESIAN_POINT('Ctrl Pts',(19.2335581411531,2.13494940562169,-329.326897806595)) ;
#50511=CARTESIAN_POINT('Ctrl Pts',(17.9109518875208,-7.32704375697291,-329.445991763941)) ;
#50512=CARTESIAN_POINT('Ctrl Pts',(12.2226846215556,-15.0031246204138,-329.565085721286)) ;
#50513=CARTESIAN_POINT('Ctrl Pts',(3.55522908835243,-19.0223056926077,-329.684179678632)) ;
#50514=CARTESIAN_POINT('Ctrl Pts',(-5.97878703405911,-18.4049415466349,
-329.803273635977)) ;
#50515=CARTESIAN_POINT('Ctrl Pts',(-14.0555183834698,-13.3015100911747,
-329.922367593323)) ;
#50516=CARTESIAN_POINT('Ctrl Pts',(-18.706321898325,-4.95593470194325,-330.041461550668)) ;
#50517=CARTESIAN_POINT('Ctrl Pts',(-18.7975988894914,4.59761282879211,-330.160555508015)) ;
#50518=CARTESIAN_POINT('Ctrl Pts',(-14.3071012707609,13.0305265036326,-330.279649465359)) ;
#50519=CARTESIAN_POINT('Ctrl Pts',(-6.3293543640249,18.2873464742231,-330.398743422706)) ;
#50520=CARTESIAN_POINT('Ctrl Pts',(3.19112548922268,19.0867620576596,-330.517837380051)) ;
#50521=CARTESIAN_POINT('Ctrl Pts',(11.9337922914806,15.2339216644132,-330.636931337396)) ;
#50522=CARTESIAN_POINT('Ctrl Pts',(17.7676861785204,7.667926420832,-330.756025294742)) ;
#50523=CARTESIAN_POINT('Ctrl Pts',(19.2708390018775,-1.76706873024081,-330.875119252087)) ;
#50524=CARTESIAN_POINT('Ctrl Pts',(16.0768684655289,-10.7713540502466,-330.994213209433)) ;
#50525=CARTESIAN_POINT('Ctrl Pts',(8.96428107949361,-17.1502021113896,-331.113307166779)) ;
#50526=CARTESIAN_POINT('Ctrl Pts',(-0.333282998908613,-19.3488162474173,
-331.232401124124)) ;
#50527=CARTESIAN_POINT('Ctrl Pts',(-9.54961183065582,-16.8313006513899,
-331.35149508147)) ;
#50528=CARTESIAN_POINT('Ctrl Pts',(-16.4382939625616,-10.2112809839948,
-331.470589038815)) ;
#50529=CARTESIAN_POINT('Ctrl Pts',(-19.3202644739853,-1.10233769278807,
-331.589682996161)) ;
#50530=CARTESIAN_POINT('Ctrl Pts',(-17.4930645353,8.27529219408646,-331.708776953506)) ;
#50531=CARTESIAN_POINT('Ctrl Pts',(-11.4020605114064,15.6358812936114,-331.827870910852)) ;
#50532=CARTESIAN_POINT('Ctrl Pts',(-2.53188923009922,19.1853408794367,-331.946964868198)) ;
#50533=CARTESIAN_POINT('Ctrl Pts',(6.95541117805748,18.0585166355887,-332.066058825544)) ;
#50534=CARTESIAN_POINT('Ctrl Pts',(14.7473819579802,12.5300635720304,-332.185152782889)) ;
#50535=CARTESIAN_POINT('Ctrl Pts',(18.9447883142893,3.9475009132931,-332.304246740235)) ;
#50536=CARTESIAN_POINT('Ctrl Pts',(18.5245437355737,-5.59723566794349,-332.42334069758)) ;
#50537=CARTESIAN_POINT('Ctrl Pts',(13.589079705345,-13.7776877775432,-332.542434654926)) ;
#50538=CARTESIAN_POINT('Ctrl Pts',(5.3413787914672,-18.5999311918014,-332.661528612271)) ;
#50539=CARTESIAN_POINT('Ctrl Pts',(-4.20824338759227,-18.8885800240374,
-332.780622569617)) ;
#50540=CARTESIAN_POINT('Ctrl Pts',(-12.7321376096457,-14.5732782730149,
-332.899716526962)) ;
#50541=CARTESIAN_POINT('Ctrl Pts',(-18.152668196134,-6.70584857380063,-333.018810484308)) ;
#50542=CARTESIAN_POINT('Ctrl Pts',(-19.1486212218456,2.79608172912783,-333.137904441654)) ;
#50543=CARTESIAN_POINT('Ctrl Pts',(-15.4772405607092,11.6164879528891,-333.256998398999)) ;
#50544=CARTESIAN_POINT('Ctrl Pts',(-8.03339788199212,17.6054618287418,-333.376092356345)) ;
#50545=CARTESIAN_POINT('Ctrl Pts',(1.36852564860903,19.3032356169317,-333.49518631369)) ;
#50546=CARTESIAN_POINT('Ctrl Pts',(10.4368812535058,16.2959896119843,-333.614280271036)) ;
#50547=CARTESIAN_POINT('Ctrl Pts',(16.9613248505475,9.31671761125554,-333.733374228381)) ;
#50548=CARTESIAN_POINT('Ctrl Pts',(19.3515719468919,0.066565140644495,-333.852468185727)) ;
#50549=CARTESIAN_POINT('Ctrl Pts',(17.0250176299756,-9.19981208681469,-333.971562143072)) ;
#50550=CARTESIAN_POINT('Ctrl Pts',(10.5487421721494,-16.223803694547,-334.090656100418)) ;
#50551=CARTESIAN_POINT('Ctrl Pts',(1.50128944137264,-19.2933640857914,-334.209750057763)) ;
#50552=CARTESIAN_POINT('Ctrl Pts',(-7.91209139995821,-17.6603107960304,
-334.32884401511)) ;
#50553=CARTESIAN_POINT('Ctrl Pts',(-15.3969589401686,-11.7226883916804,
-334.447937972455)) ;
#50554=CARTESIAN_POINT('Ctrl Pts',(-19.1289325093771,-2.92774807409659,
-334.5670319298)) ;
#50555=CARTESIAN_POINT('Ctrl Pts',(-18.1983713686398,6.58080901278506,-334.686125887146)) ;
#50556=CARTESIAN_POINT('Ctrl Pts',(-12.832092859504,14.4853429568906,-334.805219844492)) ;
#50557=CARTESIAN_POINT('Ctrl Pts',(-4.33808736772787,18.8591825306311,-334.924313801837)) ;
#50558=CARTESIAN_POINT('Ctrl Pts',(5.21329458334102,18.6362369409961,-335.043407759183)) ;
#50559=CARTESIAN_POINT('Ctrl Pts',(13.4939748402039,13.8708475136049,-335.162501716528)) ;
#50560=CARTESIAN_POINT('Ctrl Pts',(18.4855993153755,5.72454239961989,-335.281595673874)) ;
#50561=CARTESIAN_POINT('Ctrl Pts',(18.9714967511573,-3.81707725286791,-335.400689631219)) ;
#50562=CARTESIAN_POINT('Ctrl Pts',(14.8332332695234,-12.4283127779369,-335.519783588565)) ;
#50563=CARTESIAN_POINT('Ctrl Pts',(7.07947974701638,-18.010239705333,-335.63887754591)) ;
#50564=CARTESIAN_POINT('Ctrl Pts',(-2.39984419255349,-19.2023049550986,
-335.757971503256)) ;
#50565=CARTESIAN_POINT('Ctrl Pts',(-11.2942239989673,-15.7139515078035,
-335.877065460602)) ;
#50566=CARTESIAN_POINT('Ctrl Pts',(-17.4357208939035,-8.39543951486601,
-335.996159417947)) ;
#50567=CARTESIAN_POINT('Ctrl Pts',(-19.3273907890776,0.969398280974121,
-336.115253375293)) ;
#50568=CARTESIAN_POINT('Ctrl Pts',(-16.5081532473335,10.097952468298,-336.234347332638)) ;
#50569=CARTESIAN_POINT('Ctrl Pts',(-9.66517640648003,16.7652060200686,-336.353441289984)) ;
#50570=CARTESIAN_POINT('Ctrl Pts',(-0.466384859172032,19.3460655590084,
-336.472535247329)) ;
#50571=CARTESIAN_POINT('Ctrl Pts',(8.84608451550538,17.2114658571273,-336.591629204675)) ;
#50572=CARTESIAN_POINT('Ctrl Pts',(16.0023867407771,10.8816995836245,-336.71072316202)) ;
#50573=CARTESIAN_POINT('Ctrl Pts',(19.2582264576617,1.89960028503601,-336.829817119367)) ;
#50574=CARTESIAN_POINT('Ctrl Pts',(17.8200170780343,-7.54551270297707,-336.948911076712)) ;
#50575=CARTESIAN_POINT('Ctrl Pts',(12.0383112653523,-15.151462634949,-337.068005034058)) ;
#50576=CARTESIAN_POINT('Ctrl Pts',(3.32235702948351,-19.0643576918605,-337.187098991403)) ;
#50577=CARTESIAN_POINT('Ctrl Pts',(-6.20339740811853,-18.3304551793761,
-337.306192948749)) ;
#50578=CARTESIAN_POINT('Ctrl Pts',(-14.2171190543885,-13.1286460139561,
-337.425286906094)) ;
#50579=CARTESIAN_POINT('Ctrl Pts',(-18.7655258010849,-4.72681655245975,
-337.54438086344)) ;
#50580=CARTESIAN_POINT('Ctrl Pts',(-18.7399715893291,4.82711705124851,-337.663474820785)) ;
#50581=CARTESIAN_POINT('Ctrl Pts',(-14.1466971260155,13.2045227742355,-337.782568778131)) ;
#50582=CARTESIAN_POINT('Ctrl Pts',(-6.10525383612982,18.3633293431438,-337.901662735476)) ;
#50583=CARTESIAN_POINT('Ctrl Pts',(3.42426461335331,19.0464084838613,-338.020756692822)) ;
#50584=CARTESIAN_POINT('Ctrl Pts',(12.1192162418993,15.086659028356,-338.139850650167)) ;
#50585=CARTESIAN_POINT('Ctrl Pts',(17.8600444598788,7.45050034667566,-338.258944607513)) ;
#50586=CARTESIAN_POINT('Ctrl Pts',(19.2481702162741,-2.00523104875944,-338.37806153277)) ;
#50587=CARTESIAN_POINT('Ctrl Pts',(17.0431018747678,-7.98081697730116,-338.457480472244)) ;
#50588=CARTESIAN_POINT('Ctrl Pts',(15.2918889592135,-10.5251149576845,-338.497201425936)) ;
#50589=CARTESIAN_POINT('',(1.77633320448849,18.481120189533,-338.000196845114)) ;
#50590=CARTESIAN_POINT('Ctrl Pts',(1.77636947923266,18.4814593181941,-338.)) ;
#50591=CARTESIAN_POINT('Ctrl Pts',(2.17391040292432,18.45257048948,-338.)) ;
#50592=CARTESIAN_POINT('Ctrl Pts',(2.56986764189956,18.4108774285079,-338.)) ;
#50593=CARTESIAN_POINT('Ctrl Pts',(2.96362238619549,18.3563986629109,-338.)) ;
#50594=CARTESIAN_POINT('Ctrl Pts',(3.07310029706004,18.3412516163535,-338.)) ;
#50595=CARTESIAN_POINT('Ctrl Pts',(3.18240800731617,18.3251158806936,-338.)) ;
#50596=CARTESIAN_POINT('Ctrl Pts',(3.29153233075946,18.3079911489261,-338.)) ;
#50597=CARTESIAN_POINT('Ctrl Pts',(3.67850503528529,18.2472640483377,-338.)) ;
#50598=CARTESIAN_POINT('Ctrl Pts',(4.06317162667884,18.1741041213075,-338.)) ;
#50599=CARTESIAN_POINT('Ctrl Pts',(4.44501400222461,18.0888487936864,-338.)) ;
#50600=CARTESIAN_POINT('Ctrl Pts',(4.8320753856327,18.0024281993121,-338.)) ;
#50601=CARTESIAN_POINT('Ctrl Pts',(5.21623533761152,17.9035792153684,-338.)) ;
#50602=CARTESIAN_POINT('Ctrl Pts',(5.59694970980476,17.7925998953498,-338.)) ;
#50603=CARTESIAN_POINT('Ctrl Pts',(5.97863845099117,17.6813365440043,-338.)) ;
#50604=CARTESIAN_POINT('Ctrl Pts',(6.35686448045023,17.557880499624,-338.)) ;
#50605=CARTESIAN_POINT('Ctrl Pts',(6.7310670982975,17.4224810427333,-338.)) ;
#50606=CARTESIAN_POINT('Ctrl Pts',(7.07320197655524,17.2986848037707,-338.)) ;
#50607=CARTESIAN_POINT('Ctrl Pts',(7.4119736372984,17.1649037532658,-338.)) ;
#50608=CARTESIAN_POINT('Ctrl Pts',(7.74693884571632,17.0212932123994,-338.)) ;
#50609=CARTESIAN_POINT('Ctrl Pts',(7.91442144992528,16.9494879419662,-338.)) ;
#50610=CARTESIAN_POINT('Ctrl Pts',(8.08095218795725,16.875224786464,-338.)) ;
#50611=CARTESIAN_POINT('Ctrl Pts',(8.24647391943457,16.7985201662949,-338.)) ;
#50612=CARTESIAN_POINT('Ctrl Pts',(8.34874712530054,16.7511256197335,-338.)) ;
#50613=CARTESIAN_POINT('Ctrl Pts',(8.45063508783765,16.7027989309844,-338.)) ;
#50614=CARTESIAN_POINT('Ctrl Pts',(8.5521240703735,16.653543605919,-338.)) ;
#50615=CARTESIAN_POINT('Ctrl Pts',(8.61488761099822,16.6230827763937,-338.)) ;
#50616=CARTESIAN_POINT('Ctrl Pts',(8.67750192033957,16.5922650996453,-338.)) ;
#50617=CARTESIAN_POINT('Ctrl Pts',(8.73995271599396,16.5610968510217,-338.)) ;
#50618=CARTESIAN_POINT('Ctrl Pts',(8.75802449680454,16.5520774982421,-338.)) ;
#50619=CARTESIAN_POINT('Ctrl Pts',(8.77608157694232,16.5430292933114,-338.)) ;
#50620=CARTESIAN_POINT('Ctrl Pts',(8.79412176922075,16.5339533427775,-338.)) ;
#50621=CARTESIAN_POINT('Ctrl Pts',(9.15176790784609,16.3540229621748,-338.)) ;
#50622=CARTESIAN_POINT('Ctrl Pts',(9.50314107696398,16.163010215128,-338.)) ;
#50623=CARTESIAN_POINT('Ctrl Pts',(9.8477099058203,15.9612466705402,-338.)) ;
#50624=CARTESIAN_POINT('Ctrl Pts',(10.1936378838504,15.7586872711566,-338.)) ;
#50625=CARTESIAN_POINT('Ctrl Pts',(10.5327082667092,15.5452918979248,-338.)) ;
#50626=CARTESIAN_POINT('Ctrl Pts',(10.8643692312143,15.3213455170803,-338.)) ;
#50627=CARTESIAN_POINT('Ctrl Pts',(11.1757947544843,15.1110626490227,-338.)) ;
#50628=CARTESIAN_POINT('Ctrl Pts',(11.4806876427794,14.891476392563,-338.)) ;
#50629=CARTESIAN_POINT('Ctrl Pts',(11.7785734771352,14.662784696522,-338.)) ;
#50630=CARTESIAN_POINT('Ctrl Pts',(12.0947284400047,14.4200674997583,-338.)) ;
#50631=CARTESIAN_POINT('Ctrl Pts',(12.4029912449325,14.167093939552,-338.)) ;
#50632=CARTESIAN_POINT('Ctrl Pts',(12.70301836703,13.9043703660326,-338.)) ;
#50633=CARTESIAN_POINT('Ctrl Pts',(13.0148096585189,13.6313453084328,-338.)) ;
#50634=CARTESIAN_POINT('Ctrl Pts',(13.3177074184112,13.3477904382868,-338.)) ;
#50635=CARTESIAN_POINT('Ctrl Pts',(13.6112858760549,13.0542304304932,-338.)) ;
#50636=CARTESIAN_POINT('Ctrl Pts',(13.9048643336986,12.7606704226996,-338.)) ;
#50637=CARTESIAN_POINT('Ctrl Pts',(14.189123933801,12.4571047703764,-338.)) ;
#50638=CARTESIAN_POINT('Ctrl Pts',(14.4635914006402,12.1440212322596,-338.)) ;
#50639=CARTESIAN_POINT('Ctrl Pts',(14.4888948053455,12.1151577769191,-338.)) ;
#50640=CARTESIAN_POINT('Ctrl Pts',(14.5141145397938,12.0862138269971,-338.)) ;
#50641=CARTESIAN_POINT('Ctrl Pts',(14.5392407487137,12.0572008275875,-338.)) ;
#50642=CARTESIAN_POINT('Ctrl Pts',(14.8011157482534,11.754816204771,-338.)) ;
#50643=CARTESIAN_POINT('Ctrl Pts',(15.0531043329262,11.4446271310053,-338.)) ;
#50644=CARTESIAN_POINT('Ctrl Pts',(15.294915138725,11.1271876030117,-338.)) ;
#50645=CARTESIAN_POINT('Ctrl Pts',(15.539325453578,10.8063355437855,-338.)) ;
#50646=CARTESIAN_POINT('Ctrl Pts',(15.7733383878772,10.4780759367288,-338.)) ;
#50647=CARTESIAN_POINT('Ctrl Pts',(15.9966203086589,10.1429389926428,-338.)) ;
#50648=CARTESIAN_POINT('Ctrl Pts',(16.2200615880048,9.80756285793146,-338.)) ;
#50649=CARTESIAN_POINT('Ctrl Pts',(16.4327568885147,9.46529912697264,-338.)) ;
#50650=CARTESIAN_POINT('Ctrl Pts',(16.6343335873533,9.11664365354599,-338.)) ;
#50651=CARTESIAN_POINT('Ctrl Pts',(16.8345187990813,8.77039495431535,-338.)) ;
#50652=CARTESIAN_POINT('Ctrl Pts',(17.0237386859317,8.41784199162096,-338.)) ;
#50653=CARTESIAN_POINT('Ctrl Pts',(17.2015857010701,8.05944220770482,-338.)) ;
#50654=CARTESIAN_POINT('Ctrl Pts',(17.3225387132176,7.81569601166157,-338.)) ;
#50655=CARTESIAN_POINT('Ctrl Pts',(17.4382305466854,7.56924490433029,-338.)) ;
#50656=CARTESIAN_POINT('Ctrl Pts',(17.54852052106,7.32022687050523,-338.)) ;
#50657=CARTESIAN_POINT('Ctrl Pts',(17.7115647639123,6.95209770000015,-338.)) ;
#50658=CARTESIAN_POINT('Ctrl Pts',(17.8628058244222,6.57835903075512,-338.)) ;
#50659=CARTESIAN_POINT('Ctrl Pts',(18.0021199161755,6.19960247884217,-338.)) ;
#50660=CARTESIAN_POINT('Ctrl Pts',(18.0345200794339,6.11151538038197,-338.)) ;
#50661=CARTESIAN_POINT('Ctrl Pts',(18.0662749154496,6.02315682168231,-338.)) ;
#50662=CARTESIAN_POINT('Ctrl Pts',(18.0973824707912,5.93453416492661,-338.)) ;
#50663=CARTESIAN_POINT('Ctrl Pts',(18.1158571451719,5.8819014617672,-338.)) ;
#50664=CARTESIAN_POINT('Ctrl Pts',(18.1341035121823,5.82917560727256,-338.)) ;
#50665=CARTESIAN_POINT('Ctrl Pts',(18.1521211372521,5.77635814034836,-338.)) ;
#50666=CARTESIAN_POINT('Ctrl Pts',(18.1654471331487,5.73729387162396,-338.)) ;
#50667=CARTESIAN_POINT('Ctrl Pts',(18.1786455508356,5.69818662038403,-338.)) ;
#50668=CARTESIAN_POINT('Ctrl Pts',(18.1917138621592,5.65904466423081,-338.)) ;
#50669=CARTESIAN_POINT('Ctrl Pts',(18.3184406876075,5.27947490021735,-338.)) ;
#50670=CARTESIAN_POINT('Ctrl Pts',(18.4330120738589,4.89642243179216,-338.)) ;
#50671=CARTESIAN_POINT('Ctrl Pts',(18.5354544304136,4.51052141368157,-338.)) ;
#50672=CARTESIAN_POINT('Ctrl Pts',(18.6389760269065,4.12055489176024,-338.)) ;
#50673=CARTESIAN_POINT('Ctrl Pts',(18.7301118538657,3.72767899305814,-338.)) ;
#50674=CARTESIAN_POINT('Ctrl Pts',(18.8088425322345,3.33252217319263,-338.)) ;
#50675=CARTESIAN_POINT('Ctrl Pts',(18.8882582346412,2.93392715203159,-338.)) ;
#50676=CARTESIAN_POINT('Ctrl Pts',(18.9550521478952,2.53301081531028,-338.)) ;
#50677=CARTESIAN_POINT('Ctrl Pts',(19.0091546529916,2.13039965164354,-338.)) ;
#50678=CARTESIAN_POINT('Ctrl Pts',(19.0630644990411,1.72922218652565,-338.)) ;
#50679=CARTESIAN_POINT('Ctrl Pts',(19.1043732401407,1.32636138246208,-338.)) ;
#50680=CARTESIAN_POINT('Ctrl Pts',(19.1329611487376,0.922426999182332,-338.)) ;
#50681=CARTESIAN_POINT('Ctrl Pts',(19.1617023053855,0.516327289371959,-338.)) ;
#50682=CARTESIAN_POINT('Ctrl Pts',(19.1775860460932,0.109141896139547,-338.)) ;
#50683=CARTESIAN_POINT('Ctrl Pts',(19.1804373013571,-0.298511319337705,
-338.)) ;
#50684=CARTESIAN_POINT('Ctrl Pts',(19.1832885566211,-0.706164534814958,
-338.)) ;
#50685=CARTESIAN_POINT('Ctrl Pts',(19.1731074546459,-1.11428614840787,-338.)) ;
#50686=CARTESIAN_POINT('Ctrl Pts',(19.1496635348269,-1.52225148885922,-338.)) ;
#50687=CARTESIAN_POINT('Ctrl Pts',(19.1471568248662,-1.56587264054497,-338.)) ;
#50688=CARTESIAN_POINT('Ctrl Pts',(19.144498328436,-1.60949310274768,-338.)) ;
#50689=CARTESIAN_POINT('Ctrl Pts',(19.1416889329332,-1.65309486766109,-338.)) ;
#50690=CARTESIAN_POINT('Ctrl Pts',(19.1344676969147,-1.76516831369235,-338.)) ;
#50691=CARTESIAN_POINT('Ctrl Pts',(19.1262480834202,-1.87714443349572,-338.)) ;
#50692=CARTESIAN_POINT('Ctrl Pts',(19.1170287633827,-1.98901025853755,-338.)) ;
#50693=CARTESIAN_POINT('Ctrl Pts',(19.0838939307125,-2.39106327103881,-338.)) ;
#50694=CARTESIAN_POINT('Ctrl Pts',(19.0378497220312,-2.79169132925915,-338.)) ;
#50695=CARTESIAN_POINT('Ctrl Pts',(18.9791990932023,-3.19034486804637,-338.)) ;
#50696=CARTESIAN_POINT('Ctrl Pts',(18.9201130494373,-3.59195796086731,-338.)) ;
#50697=CARTESIAN_POINT('Ctrl Pts',(18.8482326076527,-3.99156762017486,-338.)) ;
#50698=CARTESIAN_POINT('Ctrl Pts',(18.7638142657312,-4.38861097663487,-338.)) ;
#50699=CARTESIAN_POINT('Ctrl Pts',(18.6790169160031,-4.78743691408631,-338.)) ;
#50700=CARTESIAN_POINT('Ctrl Pts',(18.5815687026665,-5.18367398668219,-338.)) ;
#50701=CARTESIAN_POINT('Ctrl Pts',(18.4716778745572,-5.57674284347594,-338.)) ;
#50702=CARTESIAN_POINT('Ctrl Pts',(18.4042537522977,-5.81791240341871,-338.)) ;
#50703=CARTESIAN_POINT('Ctrl Pts',(18.3321446001537,-6.057889081464,-338.)) ;
#50704=CARTESIAN_POINT('Ctrl Pts',(18.2553892686054,-6.29653609375471,-338.)) ;
#50705=CARTESIAN_POINT('Ctrl Pts',(18.2347050437555,-6.36084730657091,-338.)) ;
#50706=CARTESIAN_POINT('Ctrl Pts',(18.2136824989532,-6.42506454969312,-338.)) ;
#50707=CARTESIAN_POINT('Ctrl Pts',(18.1923252042675,-6.48917644953959,-338.)) ;
#50708=CARTESIAN_POINT('Ctrl Pts',(18.1821231319009,-6.51980178160615,-338.)) ;
#50709=CARTESIAN_POINT('Ctrl Pts',(18.1718451611425,-6.55040161889664,-338.)) ;
#50710=CARTESIAN_POINT('Ctrl Pts',(18.1614925996888,-6.58097220724148,-338.)) ;
#50711=CARTESIAN_POINT('Ctrl Pts',(18.1587181966591,-6.58916487852408,-338.)) ;
#50712=CARTESIAN_POINT('Ctrl Pts',(18.1559384069493,-6.59735553787596,-338.)) ;
#50713=CARTESIAN_POINT('Ctrl Pts',(18.153153236177,-6.60554417179179,-338.)) ;
#50714=CARTESIAN_POINT('Ctrl Pts',(18.0211106344472,-6.99376041246909,-338.)) ;
#50715=CARTESIAN_POINT('Ctrl Pts',(17.8769670753422,-7.37745629177543,-338.)) ;
#50716=CARTESIAN_POINT('Ctrl Pts',(17.7209928606868,-7.75606376024863,-338.)) ;
#50717=CARTESIAN_POINT('Ctrl Pts',(17.5648885109938,-8.1349871148908,-338.)) ;
#50718=CARTESIAN_POINT('Ctrl Pts',(17.3969335821973,-8.50881409698665,-338.)) ;
#50719=CARTESIAN_POINT('Ctrl Pts',(17.2173482215894,-8.87696303044654,-338.)) ;
#50720=CARTESIAN_POINT('Ctrl Pts',(17.0381291457527,-9.24436108227884,-338.)) ;
#50721=CARTESIAN_POINT('Ctrl Pts',(16.8473268445395,-9.60610474835268,-338.)) ;
#50722=CARTESIAN_POINT('Ctrl Pts',(16.6451122658087,-9.96159584933572,-338.)) ;
#50723=CARTESIAN_POINT('Ctrl Pts',(16.442897687078,-10.3170869503188,-338.)) ;
#50724=CARTESIAN_POINT('Ctrl Pts',(16.2292706658994,-10.6663260229615,-338.)) ;
#50725=CARTESIAN_POINT('Ctrl Pts',(16.0043568677508,-11.0086868540113,-338.)) ;
#50726=CARTESIAN_POINT('Ctrl Pts',(1.74714810520642,18.4835595300519,-338.)) ;
#50727=CARTESIAN_POINT('Ctrl Pts',(1.75686632367078,18.4826409208983,-338.000065615038)) ;
#50728=CARTESIAN_POINT('Ctrl Pts',(1.76658381766053,18.4817146473289,-338.000131230076)) ;
#50729=CARTESIAN_POINT('Ctrl Pts',(1.77630057508728,18.4807807104961,-338.000196845114)) ;
#50730=CARTESIAN_POINT('Ctrl Pts',(17.5364361419604,8.35653984306081,-318.25)) ;
#50731=CARTESIAN_POINT('Ctrl Pts',(17.3525924946923,8.7230155740616,-318.25)) ;
#50732=CARTESIAN_POINT('Ctrl Pts',(17.1574041217987,9.08303922266712,-318.25)) ;
#50733=CARTESIAN_POINT('Ctrl Pts',(16.9510889781351,9.43604656513547,-318.25)) ;
#50734=CARTESIAN_POINT('Ctrl Pts',(16.8896859298515,9.54110781516859,-318.25)) ;
#50735=CARTESIAN_POINT('Ctrl Pts',(16.8272969806292,9.64554747471652,-318.25)) ;
#50736=CARTESIAN_POINT('Ctrl Pts',(16.7639270427763,9.74935035327283,-318.25)) ;
#50737=CARTESIAN_POINT('Ctrl Pts',(16.5527990036617,10.0951878110104,-318.25)) ;
#50738=CARTESIAN_POINT('Ctrl Pts',(16.330785425417,10.4339589343761,-318.25)) ;
#50739=CARTESIAN_POINT('Ctrl Pts',(16.098381788604,10.765286099281,-318.25)) ;
#50740=CARTESIAN_POINT('Ctrl Pts',(15.8636872847762,11.0998792478148,-318.25)) ;
#50741=CARTESIAN_POINT('Ctrl Pts',(15.6183965352335,11.4268813867568,-318.25)) ;
#50742=CARTESIAN_POINT('Ctrl Pts',(15.3629759208164,11.74587376911,-318.25)) ;
#50743=CARTESIAN_POINT('Ctrl Pts',(15.1075497328084,12.0648731122681,-318.25)) ;
#50744=CARTESIAN_POINT('Ctrl Pts',(14.841992826869,12.3758627364995,-318.25)) ;
#50745=CARTESIAN_POINT('Ctrl Pts',(14.5667337092679,12.6783881128115,-318.25)) ;
#50746=CARTESIAN_POINT('Ctrl Pts',(14.2937526021076,12.9784098264952,-318.25)) ;
#50747=CARTESIAN_POINT('Ctrl Pts',(14.0112287706723,13.2701071365275,-318.25)) ;
#50748=CARTESIAN_POINT('Ctrl Pts',(13.7195492816368,13.5529963066618,-318.25)) ;
#50749=CARTESIAN_POINT('Ctrl Pts',(13.4708564703982,13.7941942846968,-318.25)) ;
#50750=CARTESIAN_POINT('Ctrl Pts',(13.2155071586103,14.0289885024467,-318.25)) ;
#50751=CARTESIAN_POINT('Ctrl Pts',(12.9537267975706,14.2570528823813,-318.25)) ;
#50752=CARTESIAN_POINT('Ctrl Pts',(12.9229309771306,14.2838823575389,-318.25)) ;
#50753=CARTESIAN_POINT('Ctrl Pts',(12.8920519586899,14.3106135816842,-318.25)) ;
#50754=CARTESIAN_POINT('Ctrl Pts',(12.8610956304185,14.337241494279,-318.25)) ;
#50755=CARTESIAN_POINT('Ctrl Pts',(12.5522537735751,14.6029000664955,-318.25)) ;
#50756=CARTESIAN_POINT('Ctrl Pts',(12.2355521289726,14.8584249449322,-318.25)) ;
#50757=CARTESIAN_POINT('Ctrl Pts',(11.9114691856933,15.1034336822037,-318.25)) ;
#50758=CARTESIAN_POINT('Ctrl Pts',(11.5875586146252,15.3483121050028,-318.25)) ;
#50759=CARTESIAN_POINT('Ctrl Pts',(11.2562741718227,15.5826859352766,-318.25)) ;
#50760=CARTESIAN_POINT('Ctrl Pts',(10.9180574167217,15.8061361585003,-318.25)) ;
#50761=CARTESIAN_POINT('Ctrl Pts',(10.6011819128877,16.015486821937,-318.25)) ;
#50762=CARTESIAN_POINT('Ctrl Pts',(10.2782207486639,16.2152488449875,-318.25)) ;
#50763=CARTESIAN_POINT('Ctrl Pts',(9.94951312127901,16.4050437026364,-318.25)) ;
#50764=CARTESIAN_POINT('Ctrl Pts',(9.5981567850144,16.6079158609612,-318.25)) ;
#50765=CARTESIAN_POINT('Ctrl Pts',(9.24023458672591,16.7994006724583,-318.25)) ;
#50766=CARTESIAN_POINT('Ctrl Pts',(8.87634769728984,16.9793380940572,-318.25)) ;
#50767=CARTESIAN_POINT('Ctrl Pts',(8.498588126862,17.1661353793137,-318.25)) ;
#50768=CARTESIAN_POINT('Ctrl Pts',(8.11439989269635,17.3404885525691,-318.25)) ;
#50769=CARTESIAN_POINT('Ctrl Pts',(7.72443780478856,17.5021619857,-318.25)) ;
#50770=CARTESIAN_POINT('Ctrl Pts',(7.33447571688085,17.6638354188309,-318.25)) ;
#50771=CARTESIAN_POINT('Ctrl Pts',(6.93873911864697,17.8128293033643,-318.25)) ;
#50772=CARTESIAN_POINT('Ctrl Pts',(6.53787445191548,17.9488476178146,-318.25)) ;
#50773=CARTESIAN_POINT('Ctrl Pts',(6.50295674792525,17.9606956244746,-318.25)) ;
#50774=CARTESIAN_POINT('Ctrl Pts',(6.46800115095872,17.9724447698048,-318.25)) ;
#50775=CARTESIAN_POINT('Ctrl Pts',(6.43302014559825,17.984090917627,-318.25)) ;
#50776=CARTESIAN_POINT('Ctrl Pts',(6.05072538567341,18.1113674564188,-318.25)) ;
#50777=CARTESIAN_POINT('Ctrl Pts',(5.66501511560512,18.2264768395085,-318.25)) ;
#50778=CARTESIAN_POINT('Ctrl Pts',(5.27649729541834,18.3293332926791,-318.25)) ;
#50779=CARTESIAN_POINT('Ctrl Pts',(4.88547792735887,18.432852007214,-318.25)) ;
#50780=CARTESIAN_POINT('Ctrl Pts',(4.49161421006131,18.5239596743265,-318.25)) ;
#50781=CARTESIAN_POINT('Ctrl Pts',(4.09550603735771,18.6025201392987,-318.25)) ;
#50782=CARTESIAN_POINT('Ctrl Pts',(3.70013762588986,18.6809338868067,-318.25)) ;
#50783=CARTESIAN_POINT('Ctrl Pts',(3.302532587526,18.7468473697804,-318.25)) ;
#50784=CARTESIAN_POINT('Ctrl Pts',(2.90327583137912,18.8000747289629,-318.25)) ;
#50785=CARTESIAN_POINT('Ctrl Pts',(2.50813492818765,18.852753378624,-318.25)) ;
#50786=CARTESIAN_POINT('Ctrl Pts',(2.11137566179237,18.8930061594508,-318.25)) ;
#50787=CARTESIAN_POINT('Ctrl Pts',(1.71356161645191,18.9206023316054,-318.25)) ;
#50788=CARTESIAN_POINT('Ctrl Pts',(1.43581579041974,18.9398694281802,-318.25)) ;
#50789=CARTESIAN_POINT('Ctrl Pts',(1.15755572908782,18.9529659484427,-318.25)) ;
#50790=CARTESIAN_POINT('Ctrl Pts',(0.878974271023465,18.9597982921062,-318.25)) ;
#50791=CARTESIAN_POINT('Ctrl Pts',(0.475814698531161,18.969685973683,-318.25)) ;
#50792=CARTESIAN_POINT('Ctrl Pts',(0.0719811820807826,18.9664562374422,
-318.25)) ;
#50793=CARTESIAN_POINT('Ctrl Pts',(-0.33191013715013,18.9501896976789,-318.25)) ;
#50794=CARTESIAN_POINT('Ctrl Pts',(-0.481432201224366,18.9441677643396,
-318.25)) ;
#50795=CARTESIAN_POINT('Ctrl Pts',(-0.630962043592318,18.9363586349412,
-318.25)) ;
#50796=CARTESIAN_POINT('Ctrl Pts',(-0.780467810007441,18.9267646830662,
-318.25)) ;
#50797=CARTESIAN_POINT('Ctrl Pts',(-0.819481615977578,18.9242611235988,
-318.25)) ;
#50798=CARTESIAN_POINT('Ctrl Pts',(-0.858484587804893,18.9216366023749,
-318.25)) ;
#50799=CARTESIAN_POINT('Ctrl Pts',(-0.897472407300964,18.9188916105698,
-318.25)) ;
#50800=CARTESIAN_POINT('Ctrl Pts',(-1.29519018423448,18.8908897358177,-318.25)) ;
#50801=CARTESIAN_POINT('Ctrl Pts',(-1.69145771369441,18.8503477102804,-318.25)) ;
#50802=CARTESIAN_POINT('Ctrl Pts',(-2.08569795887412,18.79750147337,-318.25)) ;
#50803=CARTESIAN_POINT('Ctrl Pts',(-2.48308103887955,18.7442339527479,-318.25)) ;
#50804=CARTESIAN_POINT('Ctrl Pts',(-2.87840492618743,18.6784651799139,-318.25)) ;
#50805=CARTESIAN_POINT('Ctrl Pts',(-3.27107831682424,18.6003836668584,-318.25)) ;
#50806=CARTESIAN_POINT('Ctrl Pts',(-3.66482131669959,18.5220894663388,-318.25)) ;
#50807=CARTESIAN_POINT('Ctrl Pts',(-4.05589991391592,18.4314152331644,-318.25)) ;
#50808=CARTESIAN_POINT('Ctrl Pts',(-4.44370933874037,18.3284994600864,-318.25)) ;
#50809=CARTESIAN_POINT('Ctrl Pts',(-4.82917214527218,18.2262064259627,-318.25)) ;
#50810=CARTESIAN_POINT('Ctrl Pts',(-5.21140574505791,18.1118193654387,-318.25)) ;
#50811=CARTESIAN_POINT('Ctrl Pts',(-5.58979976385578,17.9854258122364,-318.25)) ;
#50812=CARTESIAN_POINT('Ctrl Pts',(-5.96503249356178,17.8600882127258,-318.25)) ;
#50813=CARTESIAN_POINT('Ctrl Pts',(-6.33649001753982,17.7229437130915,-318.25)) ;
#50814=CARTESIAN_POINT('Ctrl Pts',(-6.70355335341107,17.574032647774,-318.25)) ;
#50815=CARTESIAN_POINT('Ctrl Pts',(-6.95903479026918,17.4703883738477,-318.25)) ;
#50816=CARTESIAN_POINT('Ctrl Pts',(-7.21238703652132,17.3610430147345,-318.25)) ;
#50817=CARTESIAN_POINT('Ctrl Pts',(-7.46339259575838,17.2459978119553,-318.25)) ;
#50818=CARTESIAN_POINT('Ctrl Pts',(-7.54473144738717,17.2087171847536,-318.25)) ;
#50819=CARTESIAN_POINT('Ctrl Pts',(-7.62582381093297,17.1708379407375,-318.25)) ;
#50820=CARTESIAN_POINT('Ctrl Pts',(-7.70666209599477,17.132359899455,-318.25)) ;
#50821=CARTESIAN_POINT('Ctrl Pts',(-7.75575752701837,17.1089910709319,-318.25)) ;
#50822=CARTESIAN_POINT('Ctrl Pts',(-7.80476131161023,17.0854003626289,-318.25)) ;
#50823=CARTESIAN_POINT('Ctrl Pts',(-7.85366455439646,17.0615912195305,-318.25)) ;
#50824=CARTESIAN_POINT('Ctrl Pts',(-7.90459638592846,17.0367944331392,-318.25)) ;
#50825=CARTESIAN_POINT('Ctrl Pts',(-7.95540854768636,17.011765894505,-318.25)) ;
#50826=CARTESIAN_POINT('Ctrl Pts',(-8.00609533409681,16.9865079891405,-318.25)) ;
#50827=CARTESIAN_POINT('Ctrl Pts',(-8.07389495885023,16.9527225269511,-318.25)) ;
#50828=CARTESIAN_POINT('Ctrl Pts',(-8.14147310723852,16.9185252869047,-318.25)) ;
#50829=CARTESIAN_POINT('Ctrl Pts',(-8.20882574575339,16.8839172080118,-318.25)) ;
#50830=CARTESIAN_POINT('Ctrl Pts',(-8.56205988198051,16.7024134818954,-318.25)) ;
#50831=CARTESIAN_POINT('Ctrl Pts',(-8.90909315514637,16.5096133834362,-318.25)) ;
#50832=CARTESIAN_POINT('Ctrl Pts',(-9.24951326696572,16.305980925201,-318.25)) ;
#50833=CARTESIAN_POINT('Ctrl Pts',(-9.59174277293422,16.1012661238089,-318.25)) ;
#50834=CARTESIAN_POINT('Ctrl Pts',(-9.92728906249252,15.8856031573382,-318.25)) ;
#50835=CARTESIAN_POINT('Ctrl Pts',(-10.2557062508469,15.6594179589091,-318.25)) ;
#50836=CARTESIAN_POINT('Ctrl Pts',(-10.5842576024294,15.433140360516,-318.25)) ;
#50837=CARTESIAN_POINT('Ctrl Pts',(-10.9056744444572,15.1963315518295,-318.25)) ;
#50838=CARTESIAN_POINT('Ctrl Pts',(-11.2194770645759,14.9493780742992,-318.25)) ;
#50839=CARTESIAN_POINT('Ctrl Pts',(-11.4076016762541,14.8013295110163,-318.25)) ;
#50840=CARTESIAN_POINT('Ctrl Pts',(-11.5929890692767,14.6496342143967,-318.25)) ;
#50841=CARTESIAN_POINT('Ctrl Pts',(-11.7755291988218,14.4943694532838,-318.25)) ;
#50842=CARTESIAN_POINT('Ctrl Pts',(-11.8551661029436,14.4266319923482,-318.25)) ;
#50843=CARTESIAN_POINT('Ctrl Pts',(-11.9342712318962,14.3582058144664,-318.25)) ;
#50844=CARTESIAN_POINT('Ctrl Pts',(-12.0127749516453,14.2891508895264,-318.25)) ;
#50845=CARTESIAN_POINT('Ctrl Pts',(-12.1830299567138,14.1393879657664,-318.25)) ;
#50846=CARTESIAN_POINT('Ctrl Pts',(-12.3504882754301,13.9866429757157,-318.25)) ;
#50847=CARTESIAN_POINT('Ctrl Pts',(-12.5150767471472,13.8309917767329,-318.25)) ;
#50848=CARTESIAN_POINT('Ctrl Pts',(-12.8040613656493,13.5576992314641,-318.25)) ;
#50849=CARTESIAN_POINT('Ctrl Pts',(-13.0841952993138,13.2754541823834,-318.25)) ;
#50850=CARTESIAN_POINT('Ctrl Pts',(-13.3550247088023,12.9846635634382,-318.25)) ;
#50851=CARTESIAN_POINT('Ctrl Pts',(-13.6247425545384,12.6950664349349,-318.25)) ;
#50852=CARTESIAN_POINT('Ctrl Pts',(-13.8852324722817,12.3969933377131,-318.25)) ;
#50853=CARTESIAN_POINT('Ctrl Pts',(-14.1360073231497,12.0908124329483,-318.25)) ;
#50854=CARTESIAN_POINT('Ctrl Pts',(-14.3837323667058,11.7883551582001,-318.25)) ;
#50855=CARTESIAN_POINT('Ctrl Pts',(-14.6219775075002,11.4779856734317,-318.25)) ;
#50856=CARTESIAN_POINT('Ctrl Pts',(-14.850230230253,11.1600319202285,-318.25)) ;
#50857=CARTESIAN_POINT('Ctrl Pts',(-14.94070771286,11.033997694532,-318.25)) ;
#50858=CARTESIAN_POINT('Ctrl Pts',(-15.0296146205133,10.9067715134026,-318.25)) ;
#50859=CARTESIAN_POINT('Ctrl Pts',(-15.1169169700217,10.7783728235744,-318.25)) ;
#50860=CARTESIAN_POINT('Origin',(0.,17.5,-338.)) ;
#50861=CARTESIAN_POINT('Ctrl Pts',(18.2156409023172,-9.03480205490196,1.0374236006889)) ;
#50862=CARTESIAN_POINT('Ctrl Pts',(16.7221931315368,-12.045882967535,0.953894028032912)) ;
#50863=CARTESIAN_POINT('Ctrl Pts',(12.216439346858,-17.3085987169493,0.786888023505637)) ;
#50864=CARTESIAN_POINT('Ctrl Pts',(2.51163677899751,-21.0350137533098,0.536405587107078)) ;
#50865=CARTESIAN_POINT('Ctrl Pts',(-7.79288106850021,-19.6988587020956,
0.285976291493228)) ;
#50866=CARTESIAN_POINT('Ctrl Pts',(-16.2235226537376,-13.6228781814821,
0.0355469958793765)) ;
#50867=CARTESIAN_POINT('Ctrl Pts',(-20.7497884505389,-4.26885360646641,
-0.214882299734473)) ;
#50868=CARTESIAN_POINT('Ctrl Pts',(-20.2835223316277,6.11231092290265,-0.465311595348325)) ;
#50869=CARTESIAN_POINT('Ctrl Pts',(-14.9364280746688,15.0227392151939,-0.715740890962176)) ;
#50870=CARTESIAN_POINT('Ctrl Pts',(-5.99538406350538,20.3183546957665,-0.966170186576025)) ;
#50871=CARTESIAN_POINT('Ctrl Pts',(4.38832445956057,20.7249313061308,-1.21659948218988)) ;
#50872=CARTESIAN_POINT('Ctrl Pts',(13.7160834985439,16.1446296976496,-1.46702877780373)) ;
#50873=CARTESIAN_POINT('Ctrl Pts',(19.7434615051254,7.67957554311442,-1.71745807341758)) ;
#50874=CARTESIAN_POINT('Ctrl Pts',(21.0201216199593,-2.63335454319917,-1.96788736903143)) ;
#50875=CARTESIAN_POINT('Ctrl Pts',(17.2388798197488,-12.3126410962928,-2.21831666464528)) ;
#50876=CARTESIAN_POINT('Ctrl Pts',(9.30958190986166,-19.0292348637601,-2.46874596025913)) ;
#50877=CARTESIAN_POINT('Ctrl Pts',(-0.859805955447589,-21.1669749936797,
-2.71917525587298)) ;
#50878=CARTESIAN_POINT('Ctrl Pts',(-10.8223059286107,-18.2114742094664,
-2.96960455148683)) ;
#50879=CARTESIAN_POINT('Ctrl Pts',(-18.1807202456265,-10.8738911034878,
-3.22003384710069)) ;
#50880=CARTESIAN_POINT('Ctrl Pts',(-21.1644524458383,-0.919810017240595,
-3.47046314271453)) ;
#50881=CARTESIAN_POINT('Ctrl Pts',(-19.0555506147577,9.25559764924098,-3.72089243832839)) ;
#50882=CARTESIAN_POINT('Ctrl Pts',(-12.3614631148788,17.2039044119632,-3.97132173394223)) ;
#50883=CARTESIAN_POINT('Ctrl Pts',(-2.69293497920678,21.0125723910915,-4.22175102955609)) ;
#50884=CARTESIAN_POINT('Ctrl Pts',(7.62357269090942,19.7651520789397,-4.47218032516994)) ;
#50885=CARTESIAN_POINT('Ctrl Pts',(16.1056806585396,13.7618003122057,-4.72260962078379)) ;
#50886=CARTESIAN_POINT('Ctrl Pts',(20.7124066925322,4.44705591235964,-4.97303891639765)) ;
#50887=CARTESIAN_POINT('Ctrl Pts',(20.3352709233352,-5.93774820719521,-5.22346821201149)) ;
#50888=CARTESIAN_POINT('Ctrl Pts',(15.0650205323582,-14.8937991678264,-5.47389750762534)) ;
#50889=CARTESIAN_POINT('Ctrl Pts',(6.16979398488841,-20.26607360782,-5.72432680323919)) ;
#50890=CARTESIAN_POINT('Ctrl Pts',(-4.21002105290652,-20.7618838265611,
-5.97475609885304)) ;
#50891=CARTESIAN_POINT('Ctrl Pts',(-13.5768121851455,-16.2619269516994,
-6.22518539446689)) ;
#50892=CARTESIAN_POINT('Ctrl Pts',(-19.6767229072805,-7.84899184122399,
-6.47561469008074)) ;
#50893=CARTESIAN_POINT('Ctrl Pts',(-21.041980183154,2.45258379368018,-6.7260439856946)) ;
#50894=CARTESIAN_POINT('Ctrl Pts',(-17.3440730053068,12.1640136829898,-6.97647328130845)) ;
#50895=CARTESIAN_POINT('Ctrl Pts',(-9.47279938765414,18.9485136370798,-7.2269025769223)) ;
#50896=CARTESIAN_POINT('Ctrl Pts',(0.677838658600559,21.1735833539401,-7.47733187253615)) ;
#50897=CARTESIAN_POINT('Ctrl Pts',(10.6653737757727,18.3038219920433,-7.72776116814999)) ;
#50898=CARTESIAN_POINT('Ctrl Pts',(18.0865847676868,11.0297574195729,-7.97819046376386)) ;
#50899=CARTESIAN_POINT('Ctrl Pts',(21.1557646157634,1.10168998169065,-8.22861975937769)) ;
#50900=CARTESIAN_POINT('Ctrl Pts',(19.1344009664301,-9.09146836045887,-8.47904905499156)) ;
#50901=CARTESIAN_POINT('Ctrl Pts',(12.5088784892037,-17.0970189283302,-8.7294783506054)) ;
#50902=CARTESIAN_POINT('Ctrl Pts',(2.87344399935931,-20.9886497154031,-8.97990764621926)) ;
#50903=CARTESIAN_POINT('Ctrl Pts',(-7.45340448245264,-19.8299485353416,
-9.2303369418331)) ;
#50904=CARTESIAN_POINT('Ctrl Pts',(-15.9867994819242,-13.8997244439627,
-9.48076623744696)) ;
#50905=CARTESIAN_POINT('Ctrl Pts',(-20.6734179821683,-4.62492013205691,
-9.7311955330608)) ;
#50906=CARTESIAN_POINT('Ctrl Pts',(-20.3855562218433,5.76274195322095,-9.98162482867465)) ;
#50907=CARTESIAN_POINT('Ctrl Pts',(-15.1924800884643,14.7637612434962,-10.2320541242885)) ;
#50908=CARTESIAN_POINT('Ctrl Pts',(-6.34375821840344,20.2122940053766,-10.4824834199024)) ;
#50909=CARTESIAN_POINT('Ctrl Pts',(4.0314117727417,20.7973031042956,-10.7329127155162)) ;
#50910=CARTESIAN_POINT('Ctrl Pts',(13.4365351899228,16.3780224503238,-10.9833420111301)) ;
#50911=CARTESIAN_POINT('Ctrl Pts',(19.6085319354347,8.0178284236062,-11.2337713067439)) ;
#50912=CARTESIAN_POINT('Ctrl Pts',(21.0622834862866,-2.27163193247568,-11.4842006023578)) ;
#50913=CARTESIAN_POINT('Ctrl Pts',(17.4479851609442,-12.0144875511529,-11.7346298979716)) ;
#50914=CARTESIAN_POINT('Ctrl Pts',(9.63531683966331,-18.86639251931,-11.9850591935855)) ;
#50915=CARTESIAN_POINT('Ctrl Pts',(-0.495821193039116,-21.1786274021194,
-12.2354884891993)) ;
#50916=CARTESIAN_POINT('Ctrl Pts',(-10.5076537127573,-18.3948174969548,
-12.4859177848132)) ;
#50917=CARTESIAN_POINT('Ctrl Pts',(-17.9911130324473,-11.1848088560703,
-12.736347080427)) ;
#50918=CARTESIAN_POINT('Ctrl Pts',(-21.1455138131668,-1.28348855495878,
-12.9867763760408)) ;
#50919=CARTESIAN_POINT('Ctrl Pts',(-19.2118376656181,8.92666739626179,-13.2372056716547)) ;
#50920=CARTESIAN_POINT('Ctrl Pts',(-12.6553697127338,16.9888703192985,-13.4876349672685)) ;
#50921=CARTESIAN_POINT('Ctrl Pts',(-3.05374072833861,20.963176402005,-13.7380642628824)) ;
#50922=CARTESIAN_POINT('Ctrl Pts',(7.28268561683616,19.8932799580872,-13.9884935584963)) ;
#50923=CARTESIAN_POINT('Ctrl Pts',(15.8667372036925,14.0366216667987,-14.2389228541101)) ;
#50924=CARTESIAN_POINT('Ctrl Pts',(20.6329019226472,4.80244266260591,-14.489352149724)) ;
#50925=CARTESIAN_POINT('Ctrl Pts',(20.4343354393096,-5.5873099472703,-14.7397814453378)) ;
#50926=CARTESIAN_POINT('Ctrl Pts',(15.3188172257628,-14.6326325779113,-14.9902107409517)) ;
#50927=CARTESIAN_POINT('Ctrl Pts',(6.51725377771559,-20.1570211160549,-15.2406400365655)) ;
#50928=CARTESIAN_POINT('Ctrl Pts',(-3.85250465566884,-20.8311858922631,
-15.4910693321794)) ;
#50929=CARTESIAN_POINT('Ctrl Pts',(-13.2952654995439,-16.4929079205848,
-15.7414986277932)) ;
#50930=CARTESIAN_POINT('Ctrl Pts',(-19.5388923004895,-8.18607269478913,
-15.9919279234071)) ;
#50931=CARTESIAN_POINT('Ctrl Pts',(-21.0810306877392,2.09051233114877,-16.2423572190209)) ;
#50932=CARTESIAN_POINT('Ctrl Pts',(-17.5506083086661,11.8640736188016,-16.4927865146348)) ;
#50933=CARTESIAN_POINT('Ctrl Pts',(-9.79712234498845,18.7828778935281,-16.7432158102486)) ;
#50934=CARTESIAN_POINT('Ctrl Pts',(0.313766917516524,21.1821061131688,-16.9936451058625)) ;
#50935=CARTESIAN_POINT('Ctrl Pts',(10.3491576970094,18.4844552986881,-17.2440744014763)) ;
#50936=CARTESIAN_POINT('Ctrl Pts',(17.8943114275467,11.3390314025154,-17.4945036970902)) ;
#50937=CARTESIAN_POINT('Ctrl Pts',(21.1337021366055,1.46519732713946,-17.744932992704)) ;
#50938=CARTESIAN_POINT('Ctrl Pts',(19.2878523405992,-8.76121679329746,-17.9953622883179)) ;
#50939=CARTESIAN_POINT('Ctrl Pts',(12.8009311760093,-16.879447212055,-18.2457915839317)) ;
#50940=CARTESIAN_POINT('Ctrl Pts',(3.2338016054572,-20.9361923513427,-18.4962208795456)) ;
#50941=CARTESIAN_POINT('Ctrl Pts',(-7.11140859808664,-19.9550670158388,
-18.7466501751594)) ;
#50942=CARTESIAN_POINT('Ctrl Pts',(-15.7455421785189,-14.1726285052673,
-18.9970794707733)) ;
#50943=CARTESIAN_POINT('Ctrl Pts',(-20.590783964988,-4.97932176306281,-19.2475087663871)) ;
#50944=CARTESIAN_POINT('Ctrl Pts',(-20.4817574082174,5.41089053506673,-19.497938062001)) ;
#50945=CARTESIAN_POINT('Ctrl Pts',(-15.4429055813031,14.5031102705227,-19.7484078957157)) ;
#50946=CARTESIAN_POINT('Ctrl Pts',(-9.60564812754564,18.2335667456015,-19.9154012975592)) ;
#50947=CARTESIAN_POINT('Ctrl Pts',(-6.41678291451902,19.2940954441978,-19.9989182675314)) ;
#50948=CARTESIAN_POINT('Ctrl Pts',(18.753381758839,-9.30151691942753,0.690868146532775)) ;
#50949=CARTESIAN_POINT('Ctrl Pts',(17.2158461688193,-12.4014874427912,0.607338573876783)) ;
#50950=CARTESIAN_POINT('Ctrl Pts',(12.5770787881632,-17.8195629344126,0.440332569349508)) ;
#50951=CARTESIAN_POINT('Ctrl Pts',(2.58578238386823,-21.6559848392743,0.18985013295095)) ;
#50952=CARTESIAN_POINT('Ctrl Pts',(-8.0229333934785,-20.2803853806118,-0.0605791626629008)) ;
#50953=CARTESIAN_POINT('Ctrl Pts',(-16.7024545241233,-14.0250368659274,
-0.311008458276752)) ;
#50954=CARTESIAN_POINT('Ctrl Pts',(-21.3623394485453,-4.39487371232039,
-0.561437753890603)) ;
#50955=CARTESIAN_POINT('Ctrl Pts',(-20.8823087663395,6.29275142063949,-0.811867049504453)) ;
#50956=CARTESIAN_POINT('Ctrl Pts',(-15.3773638435128,15.4662229606302,-1.0622963451183)) ;
#50957=CARTESIAN_POINT('Ctrl Pts',(-6.17237278318731,20.9181694108132,-1.31272564073215)) ;
#50958=CARTESIAN_POINT('Ctrl Pts',(4.51787144427738,21.3367485005781,-1.563154936346)) ;
#50959=CARTESIAN_POINT('Ctrl Pts',(14.1209936814018,16.621232582412,-1.81358423195985)) ;
#50960=CARTESIAN_POINT('Ctrl Pts',(20.3263048954516,7.90628299482715,-2.0640135275737)) ;
#50961=CARTESIAN_POINT('Ctrl Pts',(21.6406530777721,-2.71109335761582,-2.31444282318755)) ;
#50962=CARTESIAN_POINT('Ctrl Pts',(17.7477858774307,-12.6761204931842,-2.5648721188014)) ;
#50963=CARTESIAN_POINT('Ctrl Pts',(9.58440850404605,-19.5909936901154,-2.81530141441525)) ;
#50964=CARTESIAN_POINT('Ctrl Pts',(-0.885188141745862,-21.7918416851191,
-3.0657307100291)) ;
#50965=CARTESIAN_POINT('Ctrl Pts',(-11.1417893928927,-18.7490920617528,
-3.31616000564295)) ;
#50966=CARTESIAN_POINT('Ctrl Pts',(-18.7174302153441,-11.1948974049994,
-3.56658930125681)) ;
#50967=CARTESIAN_POINT('Ctrl Pts',(-21.789244669569,-0.946963573305998,
-3.81701859687065)) ;
#50968=CARTESIAN_POINT('Ctrl Pts',(-19.6180863039507,9.52883058319122,-4.0674478924845)) ;
#50969=CARTESIAN_POINT('Ctrl Pts',(-12.7263837783299,17.7117779665431,-4.31787718809835)) ;
#50970=CARTESIAN_POINT('Ctrl Pts',(-2.77243265760535,21.6328809893946,-4.5683064837122)) ;
#50971=CARTESIAN_POINT('Ctrl Pts',(7.84862689188701,20.3486357930296,-4.81873577932606)) ;
#50972=CARTESIAN_POINT('Ctrl Pts',(16.5811337353011,14.1680600933934,-5.06916507493991)) ;
#50973=CARTESIAN_POINT('Ctrl Pts',(21.3238541499783,4.57833669836856,-5.31959437055376)) ;
#50974=CARTESIAN_POINT('Ctrl Pts',(20.9355850194769,-6.11303546850379,-5.57002366616761)) ;
#50975=CARTESIAN_POINT('Ctrl Pts',(15.5097524574127,-15.333476495916,-5.82045296178146)) ;
#50976=CARTESIAN_POINT('Ctrl Pts',(6.35193143038317,-20.8643449417053,-6.07088225739531)) ;
#50977=CARTESIAN_POINT('Ctrl Pts',(-4.33430437288991,-21.3747918901187,
-6.32131155300916)) ;
#50978=CARTESIAN_POINT('Ctrl Pts',(-13.9776109630983,-16.7419925488747,
-6.57174084862301)) ;
#50979=CARTESIAN_POINT('Ctrl Pts',(-20.2575961187389,-8.08070060284082,
-6.82217014423686)) ;
#50980=CARTESIAN_POINT('Ctrl Pts',(-21.6631569239166,2.52498610535163,-7.07259943985072)) ;
#50981=CARTESIAN_POINT('Ctrl Pts',(-17.8560844532414,12.5231054751321,-7.32302873546457)) ;
#50982=CARTESIAN_POINT('Ctrl Pts',(-9.75244429741565,19.5078895057446,-7.57345803107841)) ;
#50983=CARTESIAN_POINT('Ctrl Pts',(0.697849019082179,21.7986451296659,-7.82388732669226)) ;
#50984=CARTESIAN_POINT('Ctrl Pts',(10.9802244724935,18.8441660276118,-8.07431662230612)) ;
#50985=CARTESIAN_POINT('Ctrl Pts',(18.6205157798695,11.3553650242592,-8.32474591791996)) ;
#50986=CARTESIAN_POINT('Ctrl Pts',(21.7803003675309,1.13421278544775,-8.57517521353382)) ;
#50987=CARTESIAN_POINT('Ctrl Pts',(19.6992643835285,-9.35985606141382,-8.82560450914767)) ;
#50988=CARTESIAN_POINT('Ctrl Pts',(12.8781509770061,-17.6017371346119,-9.07603380476152)) ;
#50989=CARTESIAN_POINT('Ctrl Pts',(2.95827045403466,-21.6082520964405,-9.32646310037537)) ;
#50990=CARTESIAN_POINT('Ctrl Pts',(-7.67343517650784,-20.4153450946701,
-9.57689239598922)) ;
#50991=CARTESIAN_POINT('Ctrl Pts',(-16.4587430875625,-14.310055860134,-9.82732169160307)) ;
#50992=CARTESIAN_POINT('Ctrl Pts',(-21.283714460485,-4.76145161763541,-10.077750987217)) ;
#50993=CARTESIAN_POINT('Ctrl Pts',(-20.9873547817838,5.93286288448311,-10.3281802828308)) ;
#50994=CARTESIAN_POINT('Ctrl Pts',(-15.6409747255331,15.1995997439989,-10.5786095784447)) ;
#50995=CARTESIAN_POINT('Ctrl Pts',(-6.53103123263476,20.8089777207072,-10.8290388740585)) ;
#50996=CARTESIAN_POINT('Ctrl Pts',(4.15042239835139,21.4112567743653,-11.0794681696724)) ;
#50997=CARTESIAN_POINT('Ctrl Pts',(13.8331928744073,16.8615152830932,-11.3298974652862)) ;
#50998=CARTESIAN_POINT('Ctrl Pts',(20.187392092738,8.2545213814371,-11.5803267609001)) ;
#50999=CARTESIAN_POINT('Ctrl Pts',(21.6840595974296,-2.33869239483448,-11.8307560565139)) ;
#51000=CARTESIAN_POINT('Ctrl Pts',(17.9630641820635,-12.3691652076281,-12.0811853521278)) ;
#51001=CARTESIAN_POINT('Ctrl Pts',(9.91975939965916,-19.423344104336,-12.3316146477416)) ;
#51002=CARTESIAN_POINT('Ctrl Pts',(-0.510458246681989,-21.8038380823388,
-12.5820439433555)) ;
#51003=CARTESIAN_POINT('Ctrl Pts',(-10.8178483821533,-18.937847795445,-12.8324732389693)) ;
#51004=CARTESIAN_POINT('Ctrl Pts',(-18.5222256396692,-11.5149937080088,
-13.0829025345832)) ;
#51005=CARTESIAN_POINT('Ctrl Pts',(-21.7697469527232,-1.32137820367226,
-13.333331830197)) ;
#51006=CARTESIAN_POINT('Ctrl Pts',(-19.778987078426,9.19019003580505,-13.5837611258109)) ;
#51007=CARTESIAN_POINT('Ctrl Pts',(-13.028966743188,17.4903958887708,-13.8341904214247)) ;
#51008=CARTESIAN_POINT('Ctrl Pts',(-3.14388969227891,21.5820267896627,-14.0846197170386)) ;
#51009=CARTESIAN_POINT('Ctrl Pts',(7.49767654811204,20.4805461136431,-14.3350490126524)) ;
#51010=CARTESIAN_POINT('Ctrl Pts',(16.3351364711065,14.4509944027488,-14.5854783082663)) ;
#51011=CARTESIAN_POINT('Ctrl Pts',(21.2420023332181,4.94421476080632,-14.8359076038801)) ;
#51012=CARTESIAN_POINT('Ctrl Pts',(21.037574002285,-5.75225197993385,-15.086336899494)) ;
#51013=CARTESIAN_POINT('Ctrl Pts',(15.7710414401101,-15.0646000512388,-15.3367661951078)) ;
#51014=CARTESIAN_POINT('Ctrl Pts',(6.70964852503154,-20.7520731297612,-15.5871954907217)) ;
#51015=CARTESIAN_POINT('Ctrl Pts',(-3.96623379451182,-21.4461398103899,
-15.8376247863355)) ;
#51016=CARTESIAN_POINT('Ctrl Pts',(-13.6877527853741,-16.9797922679054,
-16.0880540819494)) ;
#51017=CARTESIAN_POINT('Ctrl Pts',(-20.1156966378992,-8.4277323633153,-16.3384833775632)) ;
#51018=CARTESIAN_POINT('Ctrl Pts',(-21.703360231848,2.15222599236713,-16.5889126731771)) ;
#51019=CARTESIAN_POINT('Ctrl Pts',(-18.0687168503854,12.2143109310008,-16.8393419687909)) ;
#51020=CARTESIAN_POINT('Ctrl Pts',(-10.0863415379608,19.3373640574009,-17.0897712644048)) ;
#51021=CARTESIAN_POINT('Ctrl Pts',(0.323029577659986,21.8074194878293,-17.3402005600186)) ;
#51022=CARTESIAN_POINT('Ctrl Pts',(10.6546734323115,19.030131779574,-17.5906298556325)) ;
#51023=CARTESIAN_POINT('Ctrl Pts',(18.4225663709505,11.6737690321829,-17.8410591512463)) ;
#51024=CARTESIAN_POINT('Ctrl Pts',(21.7575865856544,1.50845116980659,-18.0914884468602)) ;
#51025=CARTESIAN_POINT('Ctrl Pts',(19.8572457697802,-9.01985519355281,-18.341917742474)) ;
#51026=CARTESIAN_POINT('Ctrl Pts',(13.1788253018201,-17.3777425204716,-18.5923470380879)) ;
#51027=CARTESIAN_POINT('Ctrl Pts',(3.32926611611954,-21.5542461474013,-18.8427763337017)) ;
#51028=CARTESIAN_POINT('Ctrl Pts',(-7.32134328943889,-20.5441571766842,
-19.0932056293156)) ;
#51029=CARTESIAN_POINT('Ctrl Pts',(-16.2103636680775,-14.5910162761098,
-19.3436349249294)) ;
#51030=CARTESIAN_POINT('Ctrl Pts',(-21.1986410184491,-5.12631547929417,
-19.5940642205433)) ;
#51031=CARTESIAN_POINT('Ctrl Pts',(-21.0863959071223,5.57062452007862,-19.8444935161572)) ;
#51032=CARTESIAN_POINT('Ctrl Pts',(-15.8987929870226,14.9312541377039,-20.0949633498719)) ;
#51033=CARTESIAN_POINT('Ctrl Pts',(-9.88921484250523,18.7718367879134,-20.2619567517154)) ;
#51034=CARTESIAN_POINT('Ctrl Pts',(-6.60621167846272,19.863673174985,-20.3454737216875)) ;
#51035=CARTESIAN_POINT('Ctrl Pts',(19.2911226153608,-9.5682317839531,0.344312692376646)) ;
#51036=CARTESIAN_POINT('Ctrl Pts',(17.7094992061018,-12.7570919180474,0.260783119720654)) ;
#51037=CARTESIAN_POINT('Ctrl Pts',(12.9377182294684,-18.330527151876,0.0937771151933803)) ;
#51038=CARTESIAN_POINT('Ctrl Pts',(2.65992798873894,-22.276955925239,-0.156705321205179)) ;
#51039=CARTESIAN_POINT('Ctrl Pts',(-8.2529857184568,-20.8619120591279,-0.407134616819029)) ;
#51040=CARTESIAN_POINT('Ctrl Pts',(-17.181386394509,-14.4271955503726,-0.65756391243288)) ;
#51041=CARTESIAN_POINT('Ctrl Pts',(-21.9748904465517,-4.52089381817433,
-0.907993208046731)) ;
#51042=CARTESIAN_POINT('Ctrl Pts',(-21.4810952010514,6.47319191837629,-1.15842250366058)) ;
#51043=CARTESIAN_POINT('Ctrl Pts',(-15.8182996123569,15.9097067060664,-1.40885179927444)) ;
#51044=CARTESIAN_POINT('Ctrl Pts',(-6.34936150286924,21.5179841258598,-1.65928109488828)) ;
#51045=CARTESIAN_POINT('Ctrl Pts',(4.64741842899419,21.9485656950253,-1.90971039050214)) ;
#51046=CARTESIAN_POINT('Ctrl Pts',(14.5259038642597,17.0978354671745,-2.16013968611599)) ;
#51047=CARTESIAN_POINT('Ctrl Pts',(20.9091482857778,8.13299044653988,-2.41056898172984)) ;
#51048=CARTESIAN_POINT('Ctrl Pts',(22.261184535585,-2.78883217203244,-2.66099827734369)) ;
#51049=CARTESIAN_POINT('Ctrl Pts',(18.2566919351126,-13.0395998900757,-2.91142757295754)) ;
#51050=CARTESIAN_POINT('Ctrl Pts',(9.85923509823043,-20.1527525164705,-3.16185686857139)) ;
#51051=CARTESIAN_POINT('Ctrl Pts',(-0.91057032804412,-22.4167083765583,
-3.41228616418524)) ;
#51052=CARTESIAN_POINT('Ctrl Pts',(-11.461272857175,-19.2867099140392,-3.6627154597991)) ;
#51053=CARTESIAN_POINT('Ctrl Pts',(-19.2541401850614,-11.5159037065109,
-3.91314475541294)) ;
#51054=CARTESIAN_POINT('Ctrl Pts',(-22.4140368932999,-0.974117129371415,
-4.1635740510268)) ;
#51055=CARTESIAN_POINT('Ctrl Pts',(-20.1806219931435,9.80206351714144,-4.41400334664064)) ;
#51056=CARTESIAN_POINT('Ctrl Pts',(-13.0913044417807,18.2196515211228,-4.6644326422545)) ;
#51057=CARTESIAN_POINT('Ctrl Pts',(-2.85193033600393,22.253189587698,-4.91486193786834)) ;
#51058=CARTESIAN_POINT('Ctrl Pts',(8.07368109286461,20.9321195071196,-5.1652912334822)) ;
#51059=CARTESIAN_POINT('Ctrl Pts',(17.0565868120627,14.5743198745811,-5.41572052909605)) ;
#51060=CARTESIAN_POINT('Ctrl Pts',(21.9353016074241,4.70961748437752,-5.6661498247099)) ;
#51061=CARTESIAN_POINT('Ctrl Pts',(21.5358991156188,-6.28832272981237,-5.91657912032376)) ;
#51062=CARTESIAN_POINT('Ctrl Pts',(15.9544843824673,-15.7731538240056,-6.1670084159376)) ;
#51063=CARTESIAN_POINT('Ctrl Pts',(6.53406887587788,-21.4626162755904,-6.41743771155145)) ;
#51064=CARTESIAN_POINT('Ctrl Pts',(-4.45858769287325,-21.9876999536765,
-6.6678670071653)) ;
#51065=CARTESIAN_POINT('Ctrl Pts',(-14.3784097410511,-17.2220581460501,
-6.91829630277916)) ;
#51066=CARTESIAN_POINT('Ctrl Pts',(-20.8384693301974,-8.31240936445765,
-7.168725598393)) ;
#51067=CARTESIAN_POINT('Ctrl Pts',(-22.2843336646794,2.59738841702309,-7.41915489400686)) ;
#51068=CARTESIAN_POINT('Ctrl Pts',(-18.3680959011759,12.8821972672744,-7.6695841896207)) ;
#51069=CARTESIAN_POINT('Ctrl Pts',(-10.0320892071771,20.0672653744092,-7.92001348523456)) ;
#51070=CARTESIAN_POINT('Ctrl Pts',(0.717859379563796,22.4237069053915,-8.17044278084841)) ;
#51071=CARTESIAN_POINT('Ctrl Pts',(11.2950751692142,19.3845100631803,-8.42087207646225)) ;
#51072=CARTESIAN_POINT('Ctrl Pts',(19.1544467920521,11.6809726289455,-8.67130137207612)) ;
#51073=CARTESIAN_POINT('Ctrl Pts',(22.4048361192983,1.16673558920485,-8.92173066768995)) ;
#51074=CARTESIAN_POINT('Ctrl Pts',(20.2641278006269,-9.62824376236878,-9.17215996330381)) ;
#51075=CARTESIAN_POINT('Ctrl Pts',(13.2474234648083,-18.1064553408938,-9.42258925891765)) ;
#51076=CARTESIAN_POINT('Ctrl Pts',(3.04309690871005,-22.2278544774778,-9.67301855453152)) ;
#51077=CARTESIAN_POINT('Ctrl Pts',(-7.89346587056307,-21.0007416539985,
-9.92344785014535)) ;
#51078=CARTESIAN_POINT('Ctrl Pts',(-16.9306866932007,-14.7203872763052,
-10.1738771457592)) ;
#51079=CARTESIAN_POINT('Ctrl Pts',(-21.8940109388016,-4.89798310321389,
-10.424306441373)) ;
#51080=CARTESIAN_POINT('Ctrl Pts',(-21.5891533417242,6.10298381574526,-10.6747357369869)) ;
#51081=CARTESIAN_POINT('Ctrl Pts',(-16.0894693626021,15.6354382445016,-10.9251650326007)) ;
#51082=CARTESIAN_POINT('Ctrl Pts',(-6.71830424686603,21.4056614360378,-11.1755943282146)) ;
#51083=CARTESIAN_POINT('Ctrl Pts',(4.26943302396105,22.0252104444349,-11.4260236238284)) ;
#51084=CARTESIAN_POINT('Ctrl Pts',(14.2298505588917,17.3450081158625,-11.6764529194423)) ;
#51085=CARTESIAN_POINT('Ctrl Pts',(20.7662522500413,8.49121433926803,-11.9268822150561)) ;
#51086=CARTESIAN_POINT('Ctrl Pts',(22.3058357085726,-2.40575285719332,-12.17731151067)) ;
#51087=CARTESIAN_POINT('Ctrl Pts',(18.4781432031829,-12.7238428641032,-12.4277408062838)) ;
#51088=CARTESIAN_POINT('Ctrl Pts',(10.204201959655,-19.980295689362,-12.6781701018977)) ;
#51089=CARTESIAN_POINT('Ctrl Pts',(-0.525095300324845,-22.4290487625584,
-12.9285993975115)) ;
#51090=CARTESIAN_POINT('Ctrl Pts',(-11.1280430515494,-19.4808780939352,
-13.1790286931254)) ;
#51091=CARTESIAN_POINT('Ctrl Pts',(-19.0533382468912,-11.8451785599472,
-13.4294579887392)) ;
#51092=CARTESIAN_POINT('Ctrl Pts',(-22.3939800922797,-1.35926785238574,
-13.6798872843531)) ;
#51093=CARTESIAN_POINT('Ctrl Pts',(-20.3461364912338,9.45371267534834,-13.9303165799669)) ;
#51094=CARTESIAN_POINT('Ctrl Pts',(-13.4025637736422,17.991921458243,-14.1807458755808)) ;
#51095=CARTESIAN_POINT('Ctrl Pts',(-3.23403865621921,22.2008771773204,-14.4311751711946)) ;
#51096=CARTESIAN_POINT('Ctrl Pts',(7.71266747938792,21.067812269199,-14.6816044668085)) ;
#51097=CARTESIAN_POINT('Ctrl Pts',(16.8035357385204,14.8653671386988,-14.9320337624223)) ;
#51098=CARTESIAN_POINT('Ctrl Pts',(21.8511027437891,5.08598685900673,-15.1824630580362)) ;
#51099=CARTESIAN_POINT('Ctrl Pts',(21.6408125652603,-5.91719401259742,-15.43289235365)) ;
#51100=CARTESIAN_POINT('Ctrl Pts',(16.2232656544574,-15.4965675245663,-15.6833216492639)) ;
#51101=CARTESIAN_POINT('Ctrl Pts',(6.90204327234747,-21.3471251434677,-15.9337509448777)) ;
#51102=CARTESIAN_POINT('Ctrl Pts',(-4.0799629333548,-22.0610937285166,-16.1841802404916)) ;
#51103=CARTESIAN_POINT('Ctrl Pts',(-14.0802400712044,-17.4666766152259,
-16.4346095361054)) ;
#51104=CARTESIAN_POINT('Ctrl Pts',(-20.6925009753088,-8.6693920318415,-16.6850388317193)) ;
#51105=CARTESIAN_POINT('Ctrl Pts',(-22.3256897759567,2.21393965358552,-16.9354681273331)) ;
#51106=CARTESIAN_POINT('Ctrl Pts',(-18.5868253921046,12.5645482431999,-17.185897422947)) ;
#51107=CARTESIAN_POINT('Ctrl Pts',(-10.3755607309332,19.8918502212737,-17.4363267185608)) ;
#51108=CARTESIAN_POINT('Ctrl Pts',(0.332292237803433,22.4327328624897,-17.6867560141747)) ;
#51109=CARTESIAN_POINT('Ctrl Pts',(10.9601891676135,19.5758082604597,-17.9371853097885)) ;
#51110=CARTESIAN_POINT('Ctrl Pts',(18.9508213143542,12.0085066618505,-18.1876146054024)) ;
#51111=CARTESIAN_POINT('Ctrl Pts',(22.3814710347033,1.5517050124737,-18.4380439010162)) ;
#51112=CARTESIAN_POINT('Ctrl Pts',(20.4266391989612,-9.27849359380813,-18.6884731966301)) ;
#51113=CARTESIAN_POINT('Ctrl Pts',(13.5567194276309,-17.8760378288881,-18.9389024922439)) ;
#51114=CARTESIAN_POINT('Ctrl Pts',(3.42473062678186,-22.1722999434598,-19.1893317878578)) ;
#51115=CARTESIAN_POINT('Ctrl Pts',(-7.53127798079115,-21.1332473375296,
-19.4397610834716)) ;
#51116=CARTESIAN_POINT('Ctrl Pts',(-16.675185157636,-15.0094040469524,-19.6901903790855)) ;
#51117=CARTESIAN_POINT('Ctrl Pts',(-21.8064980719103,-5.27330919552554,
-19.9406196746993)) ;
#51118=CARTESIAN_POINT('Ctrl Pts',(-21.6910344060272,5.73035850509048,-20.1910489703132)) ;
#51119=CARTESIAN_POINT('Ctrl Pts',(-16.3546803927421,15.3593980048849,-20.4415188040279)) ;
#51120=CARTESIAN_POINT('Ctrl Pts',(-10.1727815574648,19.3101068302253,-20.6085122058714)) ;
#51121=CARTESIAN_POINT('Ctrl Pts',(-6.79564044240643,20.4332509057722,-20.6920291758436)) ;
#51122=CARTESIAN_POINT('Ctrl Pts',(19.8288634718826,-9.83494664847866,-0.00224276177948207)) ;
#51123=CARTESIAN_POINT('Ctrl Pts',(18.2031522433843,-13.1126963933035,-0.0857723344354735)) ;
#51124=CARTESIAN_POINT('Ctrl Pts',(13.2983576707735,-18.8414913693392,-0.252778338962747)) ;
#51125=CARTESIAN_POINT('Ctrl Pts',(2.73407359360966,-22.8979270112036,-0.503260775361306)) ;
#51126=CARTESIAN_POINT('Ctrl Pts',(-8.48303804343507,-21.443438737644,-0.753690070975157)) ;
#51127=CARTESIAN_POINT('Ctrl Pts',(-17.6603182648948,-14.8293542348178,
-1.004119366589)) ;
#51128=CARTESIAN_POINT('Ctrl Pts',(-22.5874414445579,-4.64691392402828,
-1.25454866220285)) ;
#51129=CARTESIAN_POINT('Ctrl Pts',(-22.0798816357632,6.6536324161131,-1.5049779578167)) ;
#51130=CARTESIAN_POINT('Ctrl Pts',(-16.2592353812007,16.3531904515028,-1.75540725343056)) ;
#51131=CARTESIAN_POINT('Ctrl Pts',(-6.52635022255116,22.1177988409065,-2.0058365490444)) ;
#51132=CARTESIAN_POINT('Ctrl Pts',(4.77696541371103,22.5603828894726,-2.25626584465826)) ;
#51133=CARTESIAN_POINT('Ctrl Pts',(14.9308140471177,17.5744383519371,-2.5066951402721)) ;
#51134=CARTESIAN_POINT('Ctrl Pts',(21.491991676104,8.35969789825263,-2.75712443588596)) ;
#51135=CARTESIAN_POINT('Ctrl Pts',(22.8817159933979,-2.86657098644908,-3.0075537314998)) ;
#51136=CARTESIAN_POINT('Ctrl Pts',(18.7655979927946,-13.4030792869672,-3.25798302711366)) ;
#51137=CARTESIAN_POINT('Ctrl Pts',(10.1340616924148,-20.7145113428256,-3.5084123227275)) ;
#51138=CARTESIAN_POINT('Ctrl Pts',(-0.935952514342351,-23.0415750679976,
-3.75884161834136)) ;
#51139=CARTESIAN_POINT('Ctrl Pts',(-11.7807563214571,-19.8243277663255,
-4.0092709139552)) ;
#51140=CARTESIAN_POINT('Ctrl Pts',(-19.7908501547789,-11.8369100080224,
-4.25970020956907)) ;
#51141=CARTESIAN_POINT('Ctrl Pts',(-23.0388291170308,-1.00127068543683,
-4.51012950518291)) ;
#51142=CARTESIAN_POINT('Ctrl Pts',(-20.7431576823363,10.0752964510917,-4.76055880079676)) ;
#51143=CARTESIAN_POINT('Ctrl Pts',(-13.4562251052316,18.7275250757026,-5.01098809641061)) ;
#51144=CARTESIAN_POINT('Ctrl Pts',(-2.93142801440251,22.8734981860013,-5.26141739202447)) ;
#51145=CARTESIAN_POINT('Ctrl Pts',(8.29873529384221,21.5156032212096,-5.51184668763831)) ;
#51146=CARTESIAN_POINT('Ctrl Pts',(17.5320398888242,14.9805796557688,-5.76227598325218)) ;
#51147=CARTESIAN_POINT('Ctrl Pts',(22.5467490648702,4.84089827038645,-6.01270527886601)) ;
#51148=CARTESIAN_POINT('Ctrl Pts',(22.1362132117605,-6.46360999112095,-6.26313457447988)) ;
#51149=CARTESIAN_POINT('Ctrl Pts',(16.3992163075217,-16.2128311520952,-6.51356387009371)) ;
#51150=CARTESIAN_POINT('Ctrl Pts',(6.71620632137261,-22.0608876094757,-6.76399316570757)) ;
#51151=CARTESIAN_POINT('Ctrl Pts',(-4.58287101285661,-22.6006080172341,
-7.01442246132142)) ;
#51152=CARTESIAN_POINT('Ctrl Pts',(-14.779208519004,-17.7021237432253,-7.26485175693527)) ;
#51153=CARTESIAN_POINT('Ctrl Pts',(-21.4193425416559,-8.54411812607449,
-7.51528105254913)) ;
#51154=CARTESIAN_POINT('Ctrl Pts',(-22.905510405442,2.66979072869455,-7.76571034816297)) ;
#51155=CARTESIAN_POINT('Ctrl Pts',(-18.8801073491104,13.2412890594167,-8.01613964377683)) ;
#51156=CARTESIAN_POINT('Ctrl Pts',(-10.3117341169386,20.626641243074,-8.26656893939068)) ;
#51157=CARTESIAN_POINT('Ctrl Pts',(0.737869740045429,23.0487686811173,-8.51699823500452)) ;
#51158=CARTESIAN_POINT('Ctrl Pts',(11.6099258659349,19.9248540987488,-8.76742753061838)) ;
#51159=CARTESIAN_POINT('Ctrl Pts',(19.6883778042348,12.0065802336318,-9.01785682623222)) ;
#51160=CARTESIAN_POINT('Ctrl Pts',(23.0293718710659,1.19925839296196,-9.26828612184608)) ;
#51161=CARTESIAN_POINT('Ctrl Pts',(20.8289912177253,-9.89663146332373,-9.51871541745992)) ;
#51162=CARTESIAN_POINT('Ctrl Pts',(13.6166959526106,-18.6111735471754,-9.76914471307378)) ;
#51163=CARTESIAN_POINT('Ctrl Pts',(3.12792336338541,-22.8474568585153,-10.0195740086876)) ;
#51164=CARTESIAN_POINT('Ctrl Pts',(-8.11349656461829,-21.5861382133269,
-10.2700033043015)) ;
#51165=CARTESIAN_POINT('Ctrl Pts',(-17.4026302988391,-15.1307186924764,
-10.5204325999153)) ;
#51166=CARTESIAN_POINT('Ctrl Pts',(-22.5043074171183,-5.03451458879237,
-10.7708618955292)) ;
#51167=CARTESIAN_POINT('Ctrl Pts',(-22.1909519016647,6.27310474700741,-11.021291191143)) ;
#51168=CARTESIAN_POINT('Ctrl Pts',(-16.5379639996709,16.0712767450043,-11.2717204867569)) ;
#51169=CARTESIAN_POINT('Ctrl Pts',(-6.90557726109732,22.0023451513683,-11.5221497823707)) ;
#51170=CARTESIAN_POINT('Ctrl Pts',(4.38844364957074,22.6391641145045,-11.7725790779846)) ;
#51171=CARTESIAN_POINT('Ctrl Pts',(14.6265082433763,17.8285009486319,-12.0230083735984)) ;
#51172=CARTESIAN_POINT('Ctrl Pts',(21.3451124073446,8.72790729709893,-12.2734376692123)) ;
#51173=CARTESIAN_POINT('Ctrl Pts',(22.9276118197158,-2.47281331955212,-12.5238669648261)) ;
#51174=CARTESIAN_POINT('Ctrl Pts',(18.9932222243021,-13.0785205205784,-12.77429626044)) ;
#51175=CARTESIAN_POINT('Ctrl Pts',(10.4886445196508,-20.537247274388,-13.0247255560538)) ;
#51176=CARTESIAN_POINT('Ctrl Pts',(-0.539732353967712,-23.054259442778,
-13.2751548516677)) ;
#51177=CARTESIAN_POINT('Ctrl Pts',(-11.4382377209455,-20.0239083924253,
-13.5255841472815)) ;
#51178=CARTESIAN_POINT('Ctrl Pts',(-19.5844508541132,-12.1753634118858,
-13.7760134428954)) ;
#51179=CARTESIAN_POINT('Ctrl Pts',(-23.018213231836,-1.39715750109922,-14.0264427385092)) ;
#51180=CARTESIAN_POINT('Ctrl Pts',(-20.9132859040416,9.7172353148916,-14.2768720341231)) ;
#51181=CARTESIAN_POINT('Ctrl Pts',(-13.7761608040964,18.4934470277153,-14.5273013297369)) ;
#51182=CARTESIAN_POINT('Ctrl Pts',(-3.32418762015953,22.8197275649781,-14.7777306253508)) ;
#51183=CARTESIAN_POINT('Ctrl Pts',(7.92765841066382,21.655078424755,-15.0281599209646)) ;
#51184=CARTESIAN_POINT('Ctrl Pts',(17.2719350059343,15.2797398746489,-15.2785892165785)) ;
#51185=CARTESIAN_POINT('Ctrl Pts',(22.4602031543601,5.22775895720716,-15.5290185121924)) ;
#51186=CARTESIAN_POINT('Ctrl Pts',(22.2440511282356,-6.08213604526099,-15.7794478078062)) ;
#51187=CARTESIAN_POINT('Ctrl Pts',(16.6754898688048,-15.9285349978939,-16.0298771034201)) ;
#51188=CARTESIAN_POINT('Ctrl Pts',(7.09443801966338,-21.942177157174,-16.2803063990339)) ;
#51189=CARTESIAN_POINT('Ctrl Pts',(-4.19369207219777,-22.6760476466434,
-16.5307356946477)) ;
#51190=CARTESIAN_POINT('Ctrl Pts',(-14.4727273570347,-17.9535609625466,
-16.7811649902616)) ;
#51191=CARTESIAN_POINT('Ctrl Pts',(-21.2693053127184,-8.91105170036767,
-17.0315942858754)) ;
#51192=CARTESIAN_POINT('Ctrl Pts',(-22.9480193200655,2.27565331480388,-17.2820235814893)) ;
#51193=CARTESIAN_POINT('Ctrl Pts',(-19.1049339338239,12.9147855553991,-17.5324528771031)) ;
#51194=CARTESIAN_POINT('Ctrl Pts',(-10.6647799239057,20.4463363851465,-17.782882172717)) ;
#51195=CARTESIAN_POINT('Ctrl Pts',(0.341554897946883,23.0580462371502,-18.0333114683308)) ;
#51196=CARTESIAN_POINT('Ctrl Pts',(11.2657049029156,20.1214847413455,-18.2837407639447)) ;
#51197=CARTESIAN_POINT('Ctrl Pts',(19.479076257758,12.343244291518,-18.5341700595585)) ;
#51198=CARTESIAN_POINT('Ctrl Pts',(23.0053554837523,1.59495885514083,-18.7845993551724)) ;
#51199=CARTESIAN_POINT('Ctrl Pts',(20.9960326281422,-9.53713199406347,-19.0350286507863)) ;
#51200=CARTESIAN_POINT('Ctrl Pts',(13.9346135534416,-18.3743331373046,-19.2854579464001)) ;
#51201=CARTESIAN_POINT('Ctrl Pts',(3.52019513744419,-22.7903537395183,-19.535887242014)) ;
#51202=CARTESIAN_POINT('Ctrl Pts',(-7.74121267214341,-21.722337498375,-19.7863165376278)) ;
#51203=CARTESIAN_POINT('Ctrl Pts',(-17.1400066471944,-15.4277918177948,
-20.0367458332417)) ;
#51204=CARTESIAN_POINT('Ctrl Pts',(-22.4143551253713,-5.42030291175687,
-20.2871751288555)) ;
#51205=CARTESIAN_POINT('Ctrl Pts',(-22.295672904932,5.89009249010236,-20.5376044244694)) ;
#51206=CARTESIAN_POINT('Ctrl Pts',(-16.8105677984616,15.7875418720662,-20.7880742581841)) ;
#51207=CARTESIAN_POINT('Ctrl Pts',(-10.4563482724244,19.8483768725371,-20.9550676600276)) ;
#51208=CARTESIAN_POINT('Ctrl Pts',(-6.98506920635011,21.0028286365594,-21.0385846299998)) ;
#51209=CARTESIAN_POINT('Ctrl Pts',(-15.4058029086567,-15.8881929686655,
-20.)) ;
#51210=CARTESIAN_POINT('Ctrl Pts',(-15.7163716256076,-15.5628634893299,
-20.)) ;
#51211=CARTESIAN_POINT('Ctrl Pts',(-16.0164501429934,-15.2285241822995,
-20.)) ;
#51212=CARTESIAN_POINT('Ctrl Pts',(-16.3055626420778,-14.8855558777442,
-20.)) ;
#51213=CARTESIAN_POINT('Ctrl Pts',(-16.3389516192681,-14.8459472100662,
-20.)) ;
#51214=CARTESIAN_POINT('Ctrl Pts',(-16.3721942998987,-14.8062234108858,
-20.)) ;
#51215=CARTESIAN_POINT('Ctrl Pts',(-16.4052899206017,-14.7663850339305,
-20.)) ;
#51216=CARTESIAN_POINT('Ctrl Pts',(-16.6898920554989,-14.4237993113638,
-20.)) ;
#51217=CARTESIAN_POINT('Ctrl Pts',(-16.9636224828775,-14.072743433732,-20.)) ;
#51218=CARTESIAN_POINT('Ctrl Pts',(-17.2262741595062,-13.7138211105957,
-20.)) ;
#51219=CARTESIAN_POINT('Ctrl Pts',(-17.5044211527437,-13.3337239177371,
-20.)) ;
#51220=CARTESIAN_POINT('Ctrl Pts',(-17.770144363433,-12.9448044622572,-20.)) ;
#51221=CARTESIAN_POINT('Ctrl Pts',(-18.0231465801008,-12.5477434530078,
-20.)) ;
#51222=CARTESIAN_POINT('Ctrl Pts',(-18.2640935768956,-12.1696018739219,
-20.)) ;
#51223=CARTESIAN_POINT('Ctrl Pts',(-18.4935028088626,-11.784075385089,-20.)) ;
#51224=CARTESIAN_POINT('Ctrl Pts',(-18.7110696989301,-11.3917284518891,
-20.)) ;
#51225=CARTESIAN_POINT('Ctrl Pts',(-18.9276966497186,-11.0010765481736,
-20.)) ;
#51226=CARTESIAN_POINT('Ctrl Pts',(-19.1325835442372,-10.6036625010867,
-20.)) ;
#51227=CARTESIAN_POINT('Ctrl Pts',(-19.325380463851,-10.2000284326727,-20.)) ;
#51228=CARTESIAN_POINT('Ctrl Pts',(-19.5159919112789,-9.80096980577254,
-20.)) ;
#51229=CARTESIAN_POINT('Ctrl Pts',(-19.694786044292,-9.39583089087994,-20.)) ;
#51230=CARTESIAN_POINT('Ctrl Pts',(-19.8613742887721,-8.98512816896795,
-20.)) ;
#51231=CARTESIAN_POINT('Ctrl Pts',(-19.8901475315712,-8.91419129600486,
-20.)) ;
#51232=CARTESIAN_POINT('Ctrl Pts',(-19.9185565173491,-8.84308843309169,
-20.)) ;
#51233=CARTESIAN_POINT('Ctrl Pts',(-19.9465990851001,-8.77182223500242,
-20.)) ;
#51234=CARTESIAN_POINT('Ctrl Pts',(-19.9623892760821,-8.73169371009773,
-20.)) ;
#51235=CARTESIAN_POINT('Ctrl Pts',(-19.9780637277542,-8.69151219088789,
-20.)) ;
#51236=CARTESIAN_POINT('Ctrl Pts',(-19.9936156884536,-8.65129482506473,
-20.)) ;
#51237=CARTESIAN_POINT('Ctrl Pts',(-20.1540466428267,-8.2364204239466,-20.)) ;
#51238=CARTESIAN_POINT('Ctrl Pts',(-20.3016056037318,-7.81733218163497,
-20.)) ;
#51239=CARTESIAN_POINT('Ctrl Pts',(-20.4360702560848,-7.39460598547406,
-19.9999999999999)) ;
#51240=CARTESIAN_POINT('Ctrl Pts',(-20.5702980837657,-6.97262431206373,
-19.9999999999999)) ;
#51241=CARTESIAN_POINT('Ctrl Pts',(-20.6914778674514,-6.54701698129526,
-20.)) ;
#51242=CARTESIAN_POINT('Ctrl Pts',(-20.7993404945017,-6.11833751408086,
-20.)) ;
#51243=CARTESIAN_POINT('Ctrl Pts',(-20.8854364080905,-5.77616570373388,
-20.)) ;
#51244=CARTESIAN_POINT('Ctrl Pts',(-20.963046773811,-5.43203610044039,-20.)) ;
#51245=CARTESIAN_POINT('Ctrl Pts',(-21.0320115546805,-5.08622456252226,
-20.)) ;
#51246=CARTESIAN_POINT('Ctrl Pts',(-21.1186694126574,-4.65169425934677,
-19.9999999999999)) ;
#51247=CARTESIAN_POINT('Ctrl Pts',(-21.191678125955,-4.21450807110328,-20.)) ;
#51248=CARTESIAN_POINT('Ctrl Pts',(-21.2510743901899,-3.77530376686837,
-20.)) ;
#51249=CARTESIAN_POINT('Ctrl Pts',(-21.3104617875586,-3.33616502847145,
-20.)) ;
#51250=CARTESIAN_POINT('Ctrl Pts',(-21.3562407539206,-2.89500822541275,
-19.9999999999999)) ;
#51251=CARTESIAN_POINT('Ctrl Pts',(-21.3883959838031,-2.4524733104577,-20.)) ;
#51252=CARTESIAN_POINT('Ctrl Pts',(-21.4203262144307,-2.01303493770006,
-20.)) ;
#51253=CARTESIAN_POINT('Ctrl Pts',(-21.4388226045321,-1.57223714600192,
-20.)) ;
#51254=CARTESIAN_POINT('Ctrl Pts',(-21.4438200461406,-1.13071700482763,
-20.)) ;
#51255=CARTESIAN_POINT('Ctrl Pts',(-21.4458766248401,-0.949019850796634,
-20.)) ;
#51256=CARTESIAN_POINT('Ctrl Pts',(-21.4456465214687,-0.767200531796367,
-20.)) ;
#51257=CARTESIAN_POINT('Ctrl Pts',(-21.4431227621937,-0.585304284853741,
-20.)) ;
#51258=CARTESIAN_POINT('Ctrl Pts',(-21.442338628647,-0.528789009941922,
-20.)) ;
#51259=CARTESIAN_POINT('Ctrl Pts',(-21.4413329023764,-0.472260605289573,
-20.)) ;
#51260=CARTESIAN_POINT('Ctrl Pts',(-21.4401061791021,-0.41575316401674,
-20.)) ;
#51261=CARTESIAN_POINT('Ctrl Pts',(-21.430594871128,0.0223730931662136,
-20.)) ;
#51262=CARTESIAN_POINT('Ctrl Pts',(-21.4078008345799,0.459551132058727,
-20.)) ;
#51263=CARTESIAN_POINT('Ctrl Pts',(-21.3718229821551,0.895170021038482,
-20.)) ;
#51264=CARTESIAN_POINT('Ctrl Pts',(-21.3356991982527,1.33255584450437,-20.)) ;
#51265=CARTESIAN_POINT('Ctrl Pts',(-21.2862843980238,1.76837038828578,-20.)) ;
#51266=CARTESIAN_POINT('Ctrl Pts',(-21.2236263779098,2.20199489548804,-20.)) ;
#51267=CARTESIAN_POINT('Ctrl Pts',(-21.1611418379815,2.6344188339529,-20.)) ;
#51268=CARTESIAN_POINT('Ctrl Pts',(-21.0854872263467,3.06466537747855,-20.)) ;
#51269=CARTESIAN_POINT('Ctrl Pts',(-20.9966589676707,3.49211247687234,-20.)) ;
#51270=CARTESIAN_POINT('Ctrl Pts',(-20.9087567138529,3.91510358335862,-20.)) ;
#51271=CARTESIAN_POINT('Ctrl Pts',(-20.8079539088575,4.33535379125912,-20.)) ;
#51272=CARTESIAN_POINT('Ctrl Pts',(-20.6941988108917,4.75224453494563,-20.)) ;
#51273=CARTESIAN_POINT('Ctrl Pts',(-20.6335152012047,4.97463839354549,-20.)) ;
#51274=CARTESIAN_POINT('Ctrl Pts',(-20.5691448457971,5.19607591101803,-20.)) ;
#51275=CARTESIAN_POINT('Ctrl Pts',(-20.5010743690551,5.41646059911979,-20.)) ;
#51276=CARTESIAN_POINT('Ctrl Pts',(-20.3720176703124,5.83429402208323,-20.)) ;
#51277=CARTESIAN_POINT('Ctrl Pts',(-20.2296631034003,6.2483448872045,-20.)) ;
#51278=CARTESIAN_POINT('Ctrl Pts',(-20.0742865758653,6.6580351300983,-20.)) ;
#51279=CARTESIAN_POINT('Ctrl Pts',(-19.974727149743,6.92054920553505,-20.)) ;
#51280=CARTESIAN_POINT('Ctrl Pts',(-19.8698203408578,7.18127234357877,-20.)) ;
#51281=CARTESIAN_POINT('Ctrl Pts',(-19.7596300991819,7.44004522863576,-20.)) ;
#51282=CARTESIAN_POINT('Ctrl Pts',(-19.743426557129,7.47809793876163,-20.)) ;
#51283=CARTESIAN_POINT('Ctrl Pts',(-19.7271080968926,7.51610998653188,-20.)) ;
#51284=CARTESIAN_POINT('Ctrl Pts',(-19.7106769746549,7.55407608714222,-20.)) ;
#51285=CARTESIAN_POINT('Ctrl Pts',(-19.5393337799005,7.94998531822446,-20.)) ;
#51286=CARTESIAN_POINT('Ctrl Pts',(-19.356105481169,8.34006611847233,-20.)) ;
#51287=CARTESIAN_POINT('Ctrl Pts',(-19.1613930760502,8.72383375706302,-20.)) ;
#51288=CARTESIAN_POINT('Ctrl Pts',(-18.9653863811575,9.11015237092336,-20.)) ;
#51289=CARTESIAN_POINT('Ctrl Pts',(-18.7577421300927,9.4900740890982,-20.)) ;
#51290=CARTESIAN_POINT('Ctrl Pts',(-18.5388203966269,9.86308441658966,-20.)) ;
#51291=CARTESIAN_POINT('Ctrl Pts',(-18.319565318918,10.2366627134797,-20.)) ;
#51292=CARTESIAN_POINT('Ctrl Pts',(-18.088998084385,10.6033090194613,-20.)) ;
#51293=CARTESIAN_POINT('Ctrl Pts',(-17.8474358298871,10.9624794239074,-20.)) ;
#51294=CARTESIAN_POINT('Ctrl Pts',(-17.6075749157737,11.3191201652846,-20.)) ;
#51295=CARTESIAN_POINT('Ctrl Pts',(-17.3568729675726,11.668390348116,-20.)) ;
#51296=CARTESIAN_POINT('Ctrl Pts',(-17.0956014939349,12.0097243781994,-20.)) ;
#51297=CARTESIAN_POINT('Ctrl Pts',(-16.8365444490206,12.3481654025138,-20.)) ;
#51298=CARTESIAN_POINT('Ctrl Pts',(-16.5670959558664,12.678804607708,-20.)) ;
#51299=CARTESIAN_POINT('Ctrl Pts',(-16.2874872516987,13.0010522033732,-20.)) ;
#51300=CARTESIAN_POINT('Ctrl Pts',(-16.0124316447049,13.3180523779271,-20.)) ;
#51301=CARTESIAN_POINT('Ctrl Pts',(-15.7275436921894,13.6269323033859,-20.)) ;
#51302=CARTESIAN_POINT('Ctrl Pts',(-15.4330159894672,13.927088326476,-20.)) ;
#51303=CARTESIAN_POINT('Ctrl Pts',(-15.3371463552999,14.0247899954897,-20.)) ;
#51304=CARTESIAN_POINT('Ctrl Pts',(-15.240255169351,14.1215669921431,-20.)) ;
#51305=CARTESIAN_POINT('Ctrl Pts',(-15.1423485188742,14.2173974310379,-20.)) ;
#51306=CARTESIAN_POINT('Ctrl Pts',(-15.0615994091814,14.2964341725109,-20.)) ;
#51307=CARTESIAN_POINT('Ctrl Pts',(-14.980206607069,14.3747808968213,-20.)) ;
#51308=CARTESIAN_POINT('Ctrl Pts',(-14.8981884568382,14.4524259180576,-20.)) ;
#51309=CARTESIAN_POINT('Ctrl Pts',(-14.5873267664777,14.7467127616609,-20.)) ;
#51310=CARTESIAN_POINT('Ctrl Pts',(-14.2674495159252,15.0309567608575,-20.)) ;
#51311=CARTESIAN_POINT('Ctrl Pts',(-13.9391293443686,15.3048916258252,-20.)) ;
#51312=CARTESIAN_POINT('Ctrl Pts',(-13.6095969492685,15.5798379129394,-20.)) ;
#51313=CARTESIAN_POINT('Ctrl Pts',(-13.2715586942242,15.8443990772164,-20.)) ;
#51314=CARTESIAN_POINT('Ctrl Pts',(-12.9255620668213,16.0982636774071,-20.)) ;
#51315=CARTESIAN_POINT('Ctrl Pts',(-12.5802282517134,16.3516419590474,-20.)) ;
#51316=CARTESIAN_POINT('Ctrl Pts',(-12.226966029585,16.5943648615532,-20.)) ;
#51317=CARTESIAN_POINT('Ctrl Pts',(-11.8662957588071,16.8260769315832,-20.)) ;
#51318=CARTESIAN_POINT('Ctrl Pts',(-11.6413560918667,16.9705890804392,-20.)) ;
#51319=CARTESIAN_POINT('Ctrl Pts',(-11.413534500183,17.1108174721437,-20.)) ;
#51320=CARTESIAN_POINT('Ctrl Pts',(-11.1829537686147,17.2466661897157,-20.)) ;
#51321=CARTESIAN_POINT('Ctrl Pts',(-11.1400129309677,17.2719651714915,-20.)) ;
#51322=CARTESIAN_POINT('Ctrl Pts',(-11.0969743505193,17.2971134233324,-20.)) ;
#51323=CARTESIAN_POINT('Ctrl Pts',(-11.0538454480649,17.3221064554476,-20.)) ;
#51324=CARTESIAN_POINT('Ctrl Pts',(-10.6847916114131,17.5359717259913,-20.)) ;
#51325=CARTESIAN_POINT('Ctrl Pts',(-10.3095060771257,17.7382566945241,-20.)) ;
#51326=CARTESIAN_POINT('Ctrl Pts',(-9.92853192271807,17.9286680256626,-20.)) ;
#51327=CARTESIAN_POINT('Ctrl Pts',(-9.54864671752116,18.1185350987029,-20.)) ;
#51328=CARTESIAN_POINT('Ctrl Pts',(-9.16310486846575,18.2965965356029,-20.)) ;
#51329=CARTESIAN_POINT('Ctrl Pts',(-8.77242344642078,18.4625145294738,-20.)) ;
#51330=CARTESIAN_POINT('Ctrl Pts',(-8.38645555043553,18.6264307419858,-20.)) ;
#51331=CARTESIAN_POINT('Ctrl Pts',(-7.99547086428503,18.7784949003803,-20.)) ;
#51332=CARTESIAN_POINT('Ctrl Pts',(-7.59995442243829,18.9183328108531,-20.)) ;
#51333=CARTESIAN_POINT('Ctrl Pts',(-7.21155076956793,19.0556559395297,-20.)) ;
#51334=CARTESIAN_POINT('Ctrl Pts',(-6.81877645105338,19.181188684393,-20.)) ;
#51335=CARTESIAN_POINT('Ctrl Pts',(-6.42208446149232,19.2945281628512,-20.)) ;
#51336=CARTESIAN_POINT('Ctrl Pts',(-17.8811317021246,13.0451252434097,1.03858668902498)) ;
#51337=CARTESIAN_POINT('Ctrl Pts',(-15.7250931322991,16.0004653153199,0.955069732687912)) ;
#51338=CARTESIAN_POINT('Ctrl Pts',(-9.92321314561447,20.8175865914447,0.788076344479562)) ;
#51339=CARTESIAN_POINT('Ctrl Pts',(1.17400689041209,23.0306757905423,0.537606524399929)) ;
#51340=CARTESIAN_POINT('Ctrl Pts',(11.9841056083277,19.7018876770169,0.287177228786078)) ;
#51341=CARTESIAN_POINT('Ctrl Pts',(19.9119536450833,11.6323207154006,0.0367479331722268)) ;
#51342=CARTESIAN_POINT('Ctrl Pts',(23.0478433418594,0.763795191132392,-0.213681362441623)) ;
#51343=CARTESIAN_POINT('Ctrl Pts',(20.6382716461964,-10.2885336600105,-0.464110658055474)) ;
#51344=CARTESIAN_POINT('Ctrl Pts',(13.2624942528171,-18.8652055910463,-0.714539953669324)) ;
#51345=CARTESIAN_POINT('Ctrl Pts',(2.69556125327808,-22.9024975410042,-0.964969249283176)) ;
#51346=CARTESIAN_POINT('Ctrl Pts',(-8.5200306184055,-21.4289412372532,-1.21539854489703)) ;
#51347=CARTESIAN_POINT('Ctrl Pts',(-17.6854910820251,-14.799110286703,-1.46582784051088)) ;
#51348=CARTESIAN_POINT('Ctrl Pts',(-22.5954447001295,-4.60828645213766,
-1.71625713612473)) ;
#51349=CARTESIAN_POINT('Ctrl Pts',(-22.0684297685877,6.6913924216612,-1.96668643173858)) ;
#51350=CARTESIAN_POINT('Ctrl Pts',(-16.2312671764708,16.3809748738999,-2.21711572735243)) ;
#51351=CARTESIAN_POINT('Ctrl Pts',(-6.48850213627474,22.1289334562072,-2.46754502296629)) ;
#51352=CARTESIAN_POINT('Ctrl Pts',(4.81553877248335,22.5521826978432,-2.71797431858013)) ;
#51353=CARTESIAN_POINT('Ctrl Pts',(14.9608552830364,17.5488794369338,-2.96840361419398)) ;
#51354=CARTESIAN_POINT('Ctrl Pts',(21.5062598770076,8.32292880280115,-3.21883290980783)) ;
#51355=CARTESIAN_POINT('Ctrl Pts',(22.8767841945832,-2.90570204539006,-3.46926220542169)) ;
#51356=CARTESIAN_POINT('Ctrl Pts',(18.742649695744,-13.4351569016615,-3.71969150103554)) ;
#51357=CARTESIAN_POINT('Ctrl Pts',(10.0986203923039,-20.7318167341985,-3.97012079664939)) ;
#51358=CARTESIAN_POINT('Ctrl Pts',(-0.975359688754453,-23.0399442779018,
-4.22055009226323)) ;
#51359=CARTESIAN_POINT('Ctrl Pts',(-11.8146467124566,-19.804153147564,-4.47097938787709)) ;
#51360=CARTESIAN_POINT('Ctrl Pts',(-19.8110692021406,-11.8030460448693,
-4.72140868349093)) ;
#51361=CARTESIAN_POINT('Ctrl Pts',(-23.040511562476,-0.961865780905311,
-4.97183797910479)) ;
#51362=CARTESIAN_POINT('Ctrl Pts',(-20.7258987482158,10.1107606012354,-5.22226727471864)) ;
#51363=CARTESIAN_POINT('Ctrl Pts',(-13.4241776432584,18.7505150183207,-5.4726965703325)) ;
#51364=CARTESIAN_POINT('Ctrl Pts',(-2.89230336512565,22.8784820321647,-5.72312586594633)) ;
#51365=CARTESIAN_POINT('Ctrl Pts',(8.33552288439842,21.5013817485216,-5.9735551615602)) ;
#51366=CARTESIAN_POINT('Ctrl Pts',(17.5576385113683,14.9505748637168,-6.22398445717404)) ;
#51367=CARTESIAN_POINT('Ctrl Pts',(22.5549991282262,4.80232997384176,-6.47441375278789)) ;
#51368=CARTESIAN_POINT('Ctrl Pts',(22.1251295677783,-6.50146140961283,-6.72484304840174)) ;
#51369=CARTESIAN_POINT('Ctrl Pts',(16.3714659258583,-16.2408578064785,-6.9752723440156)) ;
#51370=CARTESIAN_POINT('Ctrl Pts',(6.67846655556003,-22.0723456686872,-7.22570163962945)) ;
#51371=CARTESIAN_POINT('Ctrl Pts',(-4.62151914279075,-22.5927404195368,
-7.4761309352433)) ;
#51372=CARTESIAN_POINT('Ctrl Pts',(-14.8094654207873,-17.6768236061309,
-7.72656023085714)) ;
#51373=CARTESIAN_POINT('Ctrl Pts',(-21.4339277374552,-8.50747322048703,
-7.97698952647101)) ;
#51374=CARTESIAN_POINT('Ctrl Pts',(-22.9009143755295,2.70896283038824,-8.22741882208484)) ;
#51375=CARTESIAN_POINT('Ctrl Pts',(-18.8574359996269,13.2735626857198,-8.47784811769871)) ;
#51376=CARTESIAN_POINT('Ctrl Pts',(-10.2764426745271,20.6442506477933,-8.72827741331255)) ;
#51377=CARTESIAN_POINT('Ctrl Pts',(0.777289376089591,23.0474766531517,-8.9787067089264)) ;
#51378=CARTESIAN_POINT('Ctrl Pts',(11.6439884618892,19.9049715285189,-9.22913600454027)) ;
#51379=CARTESIAN_POINT('Ctrl Pts',(19.7088871483584,11.9728913059891,-9.47956530015409)) ;
#51380=CARTESIAN_POINT('Ctrl Pts',(23.0313929628866,1.15986940681171,-9.72999459576797)) ;
#51381=CARTESIAN_POINT('Ctrl Pts',(20.8120377379817,-9.93224264930053,-9.98042389138181)) ;
#51382=CARTESIAN_POINT('Ctrl Pts',(13.5848472823902,-18.6344380963283,-10.2308531869956)) ;
#51383=CARTESIAN_POINT('Ctrl Pts',(3.08884299507603,-22.8527768072837,-10.4812824826094)) ;
#51384=CARTESIAN_POINT('Ctrl Pts',(-8.15040503259386,-21.5722334647209,
-10.7317117782233)) ;
#51385=CARTESIAN_POINT('Ctrl Pts',(-17.4284858751735,-15.1009350356404,
-10.9821410738372)) ;
#51386=CARTESIAN_POINT('Ctrl Pts',(-22.5128886799735,-4.9960186283562,-11.232570369451)) ;
#51387=CARTESIAN_POINT('Ctrl Pts',(-22.180194009962,6.3110500340433,-11.4829996650648)) ;
#51388=CARTESIAN_POINT('Ctrl Pts',(-16.5104555393895,16.0995408858014,-11.7334289606787)) ;
#51389=CARTESIAN_POINT('Ctrl Pts',(-6.86793737440163,22.014127170367,-11.9838582562926)) ;
#51390=CARTESIAN_POINT('Ctrl Pts',(4.42715797589815,22.6316289981103,-12.2342875519064)) ;
#51391=CARTESIAN_POINT('Ctrl Pts',(14.6569814886892,17.803461812023,-12.4847168475202)) ;
#51392=CARTESIAN_POINT('Ctrl Pts',(21.3600120368117,8.69138910869525,-12.7351461431341)) ;
#51393=CARTESIAN_POINT('Ctrl Pts',(22.9233526539321,-2.51202347828334,-12.985575438748)) ;
#51394=CARTESIAN_POINT('Ctrl Pts',(18.9708291124514,-13.1109878208384,-13.2360047343618)) ;
#51395=CARTESIAN_POINT('Ctrl Pts',(10.4535057383161,-20.5551593676385,-13.4864340299757)) ;
#51396=CARTESIAN_POINT('Ctrl Pts',(-0.579161639218072,-23.0533062846188,
-13.7368633255895)) ;
#51397=CARTESIAN_POINT('Ctrl Pts',(-11.4724699543666,-20.0043193332644,
-13.9872926212034)) ;
#51398=CARTESIAN_POINT('Ctrl Pts',(-19.6052490058639,-12.14185201225,-14.2377219168172)) ;
#51399=CARTESIAN_POINT('Ctrl Pts',(-23.0205728071453,-1.35778734095291,
-14.488151212431)) ;
#51400=CARTESIAN_POINT('Ctrl Pts',(-20.8966391386554,9.75299090331169,-14.7385805080449)) ;
#51401=CARTESIAN_POINT('Ctrl Pts',(-13.7445132737265,18.5169844682281,-14.9890098036587)) ;
#51402=CARTESIAN_POINT('Ctrl Pts',(-3.28515442466593,22.8253832168429,-15.2394390992726)) ;
#51403=CARTESIAN_POINT('Ctrl Pts',(7.96468503575488,21.6414914399017,-15.4898683948864)) ;
#51404=CARTESIAN_POINT('Ctrl Pts',(17.2980456144141,15.2501795292886,-15.7402976905003)) ;
#51405=CARTESIAN_POINT('Ctrl Pts',(22.4691150045175,5.18933822426017,-15.9907269861142)) ;
#51406=CARTESIAN_POINT('Ctrl Pts',(22.2336197411977,-6.12017249021728,-16.241156281728)) ;
#51407=CARTESIAN_POINT('Ctrl Pts',(16.6482254452527,-15.9570343549712,-16.4915855773418)) ;
#51408=CARTESIAN_POINT('Ctrl Pts',(7.05690063010837,-21.9542826225338,-16.7420148729558)) ;
#51409=CARTESIAN_POINT('Ctrl Pts',(-4.23246941534568,-22.6688448677897,
-16.9924441685695)) ;
#51410=CARTESIAN_POINT('Ctrl Pts',(-14.5034153210617,-17.928786050549,-17.2428734641834)) ;
#51411=CARTESIAN_POINT('Ctrl Pts',(-21.2845170458594,-8.87466023095568,
-17.4933027597973)) ;
#51412=CARTESIAN_POINT('Ctrl Pts',(-22.9440997446774,2.31489334409071,-17.7437320554111)) ;
#51413=CARTESIAN_POINT('Ctrl Pts',(-19.0828159826577,12.9474545088177,-17.994161351025)) ;
#51414=CARTESIAN_POINT('Ctrl Pts',(-10.6298056821963,20.4645294829176,-18.2445906466388)) ;
#51415=CARTESIAN_POINT('Ctrl Pts',(0.381009130946933,23.0574719658833,-18.4950199422527)) ;
#51416=CARTESIAN_POINT('Ctrl Pts',(11.3000685139548,20.1021122617704,-18.7454492378665)) ;
#51417=CARTESIAN_POINT('Ctrl Pts',(19.5002317951268,12.3100667393077,-18.9958785334804)) ;
#51418=CARTESIAN_POINT('Ctrl Pts',(23.0079156563239,1.55530782188901,-19.2463078290942)) ;
#51419=CARTESIAN_POINT('Ctrl Pts',(20.9799656776099,-9.57242705452063,-19.4967371247081)) ;
#51420=CARTESIAN_POINT('Ctrl Pts',(13.9010937855928,-18.4013181476927,-19.7472203327695)) ;
#51421=CARTESIAN_POINT('Ctrl Pts',(6.95138205173184,-21.3301728280204,-19.9142271089598)) ;
#51422=CARTESIAN_POINT('Ctrl Pts',(3.33433033300097,-21.8813254712477,-19.9977574532787)) ;
#51423=CARTESIAN_POINT('Ctrl Pts',(-17.3962108599074,12.6913527179767,0.692030669808437)) ;
#51424=CARTESIAN_POINT('Ctrl Pts',(-15.2986421932486,15.5665465205911,0.60851371347137)) ;
#51425=CARTESIAN_POINT('Ctrl Pts',(-9.65410417889847,20.2530316297668,0.441520325263021)) ;
#51426=CARTESIAN_POINT('Ctrl Pts',(1.14216883790227,22.4061037619246,0.191050505183387)) ;
#51427=CARTESIAN_POINT('Ctrl Pts',(11.6591070186625,19.167589505919,-0.0593787904304645)) ;
#51428=CARTESIAN_POINT('Ctrl Pts',(19.3719586664313,11.3168622280845,-0.309808086044315)) ;
#51429=CARTESIAN_POINT('Ctrl Pts',(22.4228057440828,0.743081725478456,-0.560237381658167)) ;
#51430=CARTESIAN_POINT('Ctrl Pts',(20.0785795509029,-10.009517516586,-0.810666677272016)) ;
#51431=CARTESIAN_POINT('Ctrl Pts',(12.9028268676587,-18.3535975152151,-1.06109597288587)) ;
#51432=CARTESIAN_POINT('Ctrl Pts',(2.62245996109128,-22.281401595766,-1.31152526849971)) ;
#51433=CARTESIAN_POINT('Ctrl Pts',(-8.28897474945834,-20.8478068657999,
-1.56195456411357)) ;
#51434=CARTESIAN_POINT('Ctrl Pts',(-17.2058758443889,-14.3977712023632,
-1.81238385972742)) ;
#51435=CARTESIAN_POINT('Ctrl Pts',(-21.9826757626381,-4.48331370517877,
-2.06281315534127)) ;
#51436=CARTESIAN_POINT('Ctrl Pts',(-21.4699530206913,6.50992764064117,-2.31324245095512)) ;
#51437=CARTESIAN_POINT('Ctrl Pts',(-15.7910892346836,15.936736988708,-2.56367174656897)) ;
#51438=CARTESIAN_POINT('Ctrl Pts',(-6.31253956449433,21.5288159005788,-2.81410104218282)) ;
#51439=CARTESIAN_POINT('Ctrl Pts',(4.68494552166555,21.9405869884746,-3.06453033779668)) ;
#51440=CARTESIAN_POINT('Ctrl Pts',(14.5551298141459,17.0729689890782,-3.31495963341052)) ;
#51441=CARTESIAN_POINT('Ctrl Pts',(20.9230286908485,8.09721816479448,-3.56538892902439)) ;
#51442=CARTESIAN_POINT('Ctrl Pts',(22.2563855730833,-2.82690191648573,-3.81581822463822)) ;
#51443=CARTESIAN_POINT('Ctrl Pts',(18.2343652299033,-13.0708070546494,-4.06624752025209)) ;
#51444=CARTESIAN_POINT('Ctrl Pts',(9.82475453261194,-20.1695877769427,-4.31667681586593)) ;
#51445=CARTESIAN_POINT('Ctrl Pts',(-0.948908776719674,-22.4151208959148,
-4.56710611147979)) ;
#51446=CARTESIAN_POINT('Ctrl Pts',(-11.4942437016324,-19.2670816252636,
-4.81753540709363)) ;
#51447=CARTESIAN_POINT('Ctrl Pts',(-19.2738101224156,-11.4829576341271,
-5.06796470270747)) ;
#51448=CARTESIAN_POINT('Ctrl Pts',(-22.4156727962215,-0.93578081199245,
-5.31839399832132)) ;
#51449=CARTESIAN_POINT('Ctrl Pts',(-20.1638302816266,9.83656550956651,-5.56882329393518)) ;
#51450=CARTESIAN_POINT('Ctrl Pts',(-13.0601255442479,18.2420172517274,-5.81925258954903)) ;
#51451=CARTESIAN_POINT('Ctrl Pts',(-2.81386659685344,22.2580373667766,-6.06968188516289)) ;
#51452=CARTESIAN_POINT('Ctrl Pts',(8.10947070578031,20.9182828529922,-6.32011118077673)) ;
#51453=CARTESIAN_POINT('Ctrl Pts',(17.081490524982,14.5451281909156,-6.57054047639058)) ;
#51454=CARTESIAN_POINT('Ctrl Pts',(21.9433270396991,4.67209493423049,-6.82096977200444)) ;
#51455=CARTESIAN_POINT('Ctrl Pts',(21.5251151703174,-6.32514739353649,-7.07139906761828)) ;
#51456=CARTESIAN_POINT('Ctrl Pts',(15.9274859151215,-15.8004197750919,-7.32182836323213)) ;
#51457=CARTESIAN_POINT('Ctrl Pts',(6.49735231286047,-21.4737627249635,-7.572257658846)) ;
#51458=CARTESIAN_POINT('Ctrl Pts',(-4.49618753669457,-21.9800448197985,
-7.82268695445983)) ;
#51459=CARTESIAN_POINT('Ctrl Pts',(-14.407845514158,-17.197443422952,-8.07311625007371)) ;
#51460=CARTESIAN_POINT('Ctrl Pts',(-20.8526581364247,-8.27675789732166,
-8.32354554568752)) ;
#51461=CARTESIAN_POINT('Ctrl Pts',(-22.2798613643712,2.63549809900938,-8.5739748413014)) ;
#51462=CARTESIAN_POINT('Ctrl Pts',(-18.3460386284019,12.9135951342243,-8.82440413691524)) ;
#51463=CARTESIAN_POINT('Ctrl Pts',(-9.99775442818221,20.0843964071426,-9.07483343252909)) ;
#51464=CARTESIAN_POINT('Ctrl Pts',(0.756209959798816,22.4224489996561,-9.32526272814294)) ;
#51465=CARTESIAN_POINT('Ctrl Pts',(11.3282135553694,19.3651658988355,-9.57569202375679)) ;
#51466=CARTESIAN_POINT('Ctrl Pts',(19.1743991576454,11.6481968385139,-9.82612131937065)) ;
#51467=CARTESIAN_POINT('Ctrl Pts',(22.4068014851743,1.12841475064213,-10.0765506149845)) ;
#51468=CARTESIAN_POINT('Ctrl Pts',(20.2476332564153,-9.66288881024618,-10.3269799105984)) ;
#51469=CARTESIAN_POINT('Ctrl Pts',(13.2164379615872,-18.1290882355676,-10.5774092062123)) ;
#51470=CARTESIAN_POINT('Ctrl Pts',(3.00507624185253,-22.2330292453847,-10.8278385018261)) ;
#51471=CARTESIAN_POINT('Ctrl Pts',(-7.92937309017233,-20.9872131318651,
-11.07826779744)) ;
#51472=CARTESIAN_POINT('Ctrl Pts',(-16.955840396691,-14.69141072489,-11.3286970930538)) ;
#51473=CARTESIAN_POINT('Ctrl Pts',(-21.902358590419,-4.8605309197842,-11.5791263886677)) ;
#51474=CARTESIAN_POINT('Ctrl Pts',(-21.5786863124056,6.13989980995436,-11.8295556842815)) ;
#51475=CARTESIAN_POINT('Ctrl Pts',(-16.0627062504226,15.6629352472039,-12.0799849798954)) ;
#51476=CARTESIAN_POINT('Ctrl Pts',(-6.68168484680049,21.4171230620162,-12.3304142755092)) ;
#51477=CARTESIAN_POINT('Ctrl Pts',(4.30709727671738,22.0178787737213,-12.5808435711231)) ;
#51478=CARTESIAN_POINT('Ctrl Pts',(14.2594968145501,17.3206473101176,-12.8312728667369)) ;
#51479=CARTESIAN_POINT('Ctrl Pts',(20.7807469657185,8.45568614554753,-13.0817021623508)) ;
#51480=CARTESIAN_POINT('Ctrl Pts',(22.3016911360505,-2.44389957197528,-13.3321314579646)) ;
#51481=CARTESIAN_POINT('Ctrl Pts',(18.4563566179797,-12.7554291592116,-13.5825607535785)) ;
#51482=CARTESIAN_POINT('Ctrl Pts',(10.1700156946661,-19.9977212055294,-13.8329900491923)) ;
#51483=CARTESIAN_POINT('Ctrl Pts',(-0.563455275966131,-22.4281205365546,
-14.0834193448062)) ;
#51484=CARTESIAN_POINT('Ctrl Pts',(-11.1613464815765,-19.4618194769542,
-14.33384864042)) ;
#51485=CARTESIAN_POINT('Ctrl Pts',(-19.0735715920305,-11.8125754764054,
-14.5842779360339)) ;
#51486=CARTESIAN_POINT('Ctrl Pts',(-22.3962747627081,-1.32096532141325,
-14.8347072316477)) ;
#51487=CARTESIAN_POINT('Ctrl Pts',(-20.3299403401995,9.4884982167326,-15.0851365272616)) ;
#51488=CARTESIAN_POINT('Ctrl Pts',(-13.3717739491923,18.0148198483798,-15.3355658228754)) ;
#51489=CARTESIAN_POINT('Ctrl Pts',(-3.19606387508772,22.2063785454482,-15.5859951184893)) ;
#51490=CARTESIAN_POINT('Ctrl Pts',(7.74868965918299,21.0545928905987,-15.8364244141031)) ;
#51491=CARTESIAN_POINT('Ctrl Pts',(16.8289375631012,14.8366078368198,-16.086853709717)) ;
#51492=CARTESIAN_POINT('Ctrl Pts',(21.8597720192203,5.04860785527804,-16.3372830053308)) ;
#51493=CARTESIAN_POINT('Ctrl Pts',(21.6306631839706,-5.95419870019608,-16.5877123009447)) ;
#51494=CARTESIAN_POINT('Ctrl Pts',(16.1967399554739,-15.5242933703622,-16.8381415965585)) ;
#51495=CARTESIAN_POINT('Ctrl Pts',(6.86552358227933,-21.3589014466138,-17.0885708921724)) ;
#51496=CARTESIAN_POINT('Ctrl Pts',(-4.11768850171349,-22.0540853811699,
-17.3390001877862)) ;
#51497=CARTESIAN_POINT('Ctrl Pts',(-14.1100952287054,-17.4425728635766,
-17.5894294834001)) ;
#51498=CARTESIAN_POINT('Ctrl Pts',(-20.7072993336923,-8.63398711332103,
-17.8398587790139)) ;
#51499=CARTESIAN_POINT('Ctrl Pts',(-22.3218755836205,2.25211543669878,-18.0902880746278)) ;
#51500=CARTESIAN_POINT('Ctrl Pts',(-18.5653065010242,12.5963307293179,-18.3407173702416)) ;
#51501=CARTESIAN_POINT('Ctrl Pts',(-10.3415345363939,19.9095491249766,-18.5911466658555)) ;
#51502=CARTESIAN_POINT('Ctrl Pts',(0.370676492512795,22.4321732481425,-18.8415759614693)) ;
#51503=CARTESIAN_POINT('Ctrl Pts',(10.9936204192713,19.5569603457334,-19.0920052570832)) ;
#51504=CARTESIAN_POINT('Ctrl Pts',(18.9714023573123,11.9762283654051,-19.342434552697)) ;
#51505=CARTESIAN_POINT('Ctrl Pts',(22.3839608628809,1.51312921756678,-19.5928638483109)) ;
#51506=CARTESIAN_POINT('Ctrl Pts',(20.4110071354131,-9.31283110351108,-19.8432931439247)) ;
#51507=CARTESIAN_POINT('Ctrl Pts',(13.5241081328644,-17.9022902985201,-20.0937763519862)) ;
#51508=CARTESIAN_POINT('Ctrl Pts',(6.76286657657885,-20.7517169704882,-20.2607831281764)) ;
#51509=CARTESIAN_POINT('Ctrl Pts',(3.24390617527739,-21.2879228302346,-20.3443134724953)) ;
#51510=CARTESIAN_POINT('Ctrl Pts',(-16.9112900176904,12.3375801925435,0.345474650591894)) ;
#51511=CARTESIAN_POINT('Ctrl Pts',(-14.872191254198,15.1326277258625,0.261957694254827)) ;
#51512=CARTESIAN_POINT('Ctrl Pts',(-9.38499521218246,19.6884766680889,0.0949643060464787)) ;
#51513=CARTESIAN_POINT('Ctrl Pts',(1.11033078539246,21.7815317333067,-0.155505514033156)) ;
#51514=CARTESIAN_POINT('Ctrl Pts',(11.3341084289973,18.6332913348211,-0.405934809647006)) ;
#51515=CARTESIAN_POINT('Ctrl Pts',(18.8319636877793,11.0014037407683,-0.656364105260858)) ;
#51516=CARTESIAN_POINT('Ctrl Pts',(21.7977681463063,0.722368259824523,-0.906793400874708)) ;
#51517=CARTESIAN_POINT('Ctrl Pts',(19.5188874556096,-9.73050137316158,-1.15722269648855)) ;
#51518=CARTESIAN_POINT('Ctrl Pts',(12.5431594825004,-17.8419894393837,-1.4076519921024)) ;
#51519=CARTESIAN_POINT('Ctrl Pts',(2.54935866890447,-21.6603056505278,-1.65808128771625)) ;
#51520=CARTESIAN_POINT('Ctrl Pts',(-8.0579188805112,-20.2666724943465,-1.90851058333011)) ;
#51521=CARTESIAN_POINT('Ctrl Pts',(-16.7262606067527,-13.9964321180233,
-2.15893987894396)) ;
#51522=CARTESIAN_POINT('Ctrl Pts',(-21.3699068251464,-4.35834095821984,
-2.40936917455781)) ;
#51523=CARTESIAN_POINT('Ctrl Pts',(-20.8714762727951,6.32846285962108,-2.65979847017166)) ;
#51524=CARTESIAN_POINT('Ctrl Pts',(-15.3509112928965,15.4924991035161,-2.91022776578551)) ;
#51525=CARTESIAN_POINT('Ctrl Pts',(-6.13657699271392,20.9286983449502,-3.16065706139936)) ;
#51526=CARTESIAN_POINT('Ctrl Pts',(4.55435227084776,21.3289912791062,-3.41108635701321)) ;
#51527=CARTESIAN_POINT('Ctrl Pts',(14.1494043452553,16.5970585412225,-3.66151565262706)) ;
#51528=CARTESIAN_POINT('Ctrl Pts',(20.3397975046893,7.87150752678782,-3.91194494824091)) ;
#51529=CARTESIAN_POINT('Ctrl Pts',(21.6359869515834,-2.74810178758143,-4.16237424385476)) ;
#51530=CARTESIAN_POINT('Ctrl Pts',(17.7260807640627,-12.7064572076373,-4.41280353946861)) ;
#51531=CARTESIAN_POINT('Ctrl Pts',(9.55088867291999,-19.607358819687,-4.66323283508247)) ;
#51532=CARTESIAN_POINT('Ctrl Pts',(-0.922457864684889,-21.7902975139278,
-4.9136621306963)) ;
#51533=CARTESIAN_POINT('Ctrl Pts',(-11.1738406908084,-18.7300101029632,
-5.16409142631018)) ;
#51534=CARTESIAN_POINT('Ctrl Pts',(-18.7365510426908,-11.1628692233849,
-5.414520721924)) ;
#51535=CARTESIAN_POINT('Ctrl Pts',(-21.790834029967,-0.90969584307959,-5.66495001753788)) ;
#51536=CARTESIAN_POINT('Ctrl Pts',(-19.6017618150375,9.56237041789767,-5.91537931315171)) ;
#51537=CARTESIAN_POINT('Ctrl Pts',(-12.6960734452374,17.7335194851344,-6.16580860876558)) ;
#51538=CARTESIAN_POINT('Ctrl Pts',(-2.73542982858124,21.6375927013884,-6.41623790437941)) ;
#51539=CARTESIAN_POINT('Ctrl Pts',(7.88341852716223,20.3351839574628,-6.66666719999328)) ;
#51540=CARTESIAN_POINT('Ctrl Pts',(16.6053425385957,14.1396815181147,-6.91709649560712)) ;
#51541=CARTESIAN_POINT('Ctrl Pts',(21.331654951172,4.54185989461926,-7.16752579122098)) ;
#51542=CARTESIAN_POINT('Ctrl Pts',(20.9251007728565,-6.14883337746017,-7.41795508683483)) ;
#51543=CARTESIAN_POINT('Ctrl Pts',(15.4835059043847,-15.3599817437055,-7.66838438244868)) ;
#51544=CARTESIAN_POINT('Ctrl Pts',(6.31623807016093,-20.87517978124,-7.91881367806253)) ;
#51545=CARTESIAN_POINT('Ctrl Pts',(-4.37085593059841,-21.36734922006,-8.16924297367638)) ;
#51546=CARTESIAN_POINT('Ctrl Pts',(-14.0062256075287,-16.7180632397733,
-8.41967226929022)) ;
#51547=CARTESIAN_POINT('Ctrl Pts',(-20.2713885353943,-8.04604257415629,
-8.67010156490409)) ;
#51548=CARTESIAN_POINT('Ctrl Pts',(-21.6588083532127,2.56203336763053,-8.92053086051792)) ;
#51549=CARTESIAN_POINT('Ctrl Pts',(-17.8346412571768,12.5536275827289,-9.17096015613178)) ;
#51550=CARTESIAN_POINT('Ctrl Pts',(-9.71906618183729,19.5245421664919,-9.42138945174563)) ;
#51551=CARTESIAN_POINT('Ctrl Pts',(0.735130543508015,21.7974213461604,-9.67181874735948)) ;
#51552=CARTESIAN_POINT('Ctrl Pts',(11.0124386488497,18.8253602691521,-9.92224804297333)) ;
#51553=CARTESIAN_POINT('Ctrl Pts',(18.6399111669323,11.3235023710388,-10.1726773385872)) ;
#51554=CARTESIAN_POINT('Ctrl Pts',(21.7822100074621,1.09696009447255,-10.423106634201)) ;
#51555=CARTESIAN_POINT('Ctrl Pts',(19.6832287748491,-9.39353497119186,-10.6735359298149)) ;
#51556=CARTESIAN_POINT('Ctrl Pts',(12.8480286407844,-17.6237383748068,-10.9239652254287)) ;
#51557=CARTESIAN_POINT('Ctrl Pts',(2.92130948862902,-21.6132816834856,-11.1743945210426)) ;
#51558=CARTESIAN_POINT('Ctrl Pts',(-7.7083411477508,-20.4021927990092,-11.4248238166564)) ;
#51559=CARTESIAN_POINT('Ctrl Pts',(-16.4831949182086,-14.2818864141397,
-11.6752531122703)) ;
#51560=CARTESIAN_POINT('Ctrl Pts',(-21.2918285008646,-4.72504321121219,
-11.9256824078841)) ;
#51561=CARTESIAN_POINT('Ctrl Pts',(-20.9771786148489,5.96874958586541,-12.176111703498)) ;
#51562=CARTESIAN_POINT('Ctrl Pts',(-15.6149569614558,15.2263296086064,-12.4265409991118)) ;
#51563=CARTESIAN_POINT('Ctrl Pts',(-6.49543231919935,20.8201189536655,-12.6769702947257)) ;
#51564=CARTESIAN_POINT('Ctrl Pts',(4.1870365775366,21.4041285493321,-12.9273995903395)) ;
#51565=CARTESIAN_POINT('Ctrl Pts',(13.8620121404112,16.8378328082122,-13.1778288859534)) ;
#51566=CARTESIAN_POINT('Ctrl Pts',(20.2014818946252,8.2199831823998,-13.4282581815672)) ;
#51567=CARTESIAN_POINT('Ctrl Pts',(21.6800296181687,-2.37577566566717,-13.6786874771811)) ;
#51568=CARTESIAN_POINT('Ctrl Pts',(17.9418841235082,-12.3998704975848,-13.9291167727949)) ;
#51569=CARTESIAN_POINT('Ctrl Pts',(9.88652565101624,-19.4402830434204,-14.1795460684088)) ;
#51570=CARTESIAN_POINT('Ctrl Pts',(-0.547748912714191,-21.8029347884905,
-14.4299753640226)) ;
#51571=CARTESIAN_POINT('Ctrl Pts',(-10.8502230087865,-18.919319620644,-14.6804046596365)) ;
#51572=CARTESIAN_POINT('Ctrl Pts',(-18.5418941781971,-11.483298940561,-14.9308339552503)) ;
#51573=CARTESIAN_POINT('Ctrl Pts',(-21.7719767182707,-1.28414330187359,
-15.1812632508642)) ;
#51574=CARTESIAN_POINT('Ctrl Pts',(-19.7632415417438,9.22400553015349,-15.431692546478)) ;
#51575=CARTESIAN_POINT('Ctrl Pts',(-12.9990346246578,17.5126552285315,-15.6821218420919)) ;
#51576=CARTESIAN_POINT('Ctrl Pts',(-3.10697332550952,21.5873738740534,-15.9325511377058)) ;
#51577=CARTESIAN_POINT('Ctrl Pts',(7.53269428261108,20.4676943412959,-16.1829804333196)) ;
#51578=CARTESIAN_POINT('Ctrl Pts',(16.3598295117884,14.423036144351,-16.4334097289334)) ;
#51579=CARTESIAN_POINT('Ctrl Pts',(21.2504290339233,4.90787748629594,-16.6838390245473)) ;
#51580=CARTESIAN_POINT('Ctrl Pts',(21.0277066267436,-5.78822491017488,-16.9342683201612)) ;
#51581=CARTESIAN_POINT('Ctrl Pts',(15.7452544656953,-15.0915523857532,-17.184697615775)) ;
#51582=CARTESIAN_POINT('Ctrl Pts',(6.6741465344503,-20.7635202706937,-17.4351269113889)) ;
#51583=CARTESIAN_POINT('Ctrl Pts',(-4.00290758808131,-21.4393258945502,
-17.6855562070027)) ;
#51584=CARTESIAN_POINT('Ctrl Pts',(-13.7167751363492,-16.9563596766042,
-17.9359855026166)) ;
#51585=CARTESIAN_POINT('Ctrl Pts',(-20.1300816215249,-8.39331399568637,
-18.1864147982304)) ;
#51586=CARTESIAN_POINT('Ctrl Pts',(-21.6996514225636,2.18933752930682,-18.4368440938443)) ;
#51587=CARTESIAN_POINT('Ctrl Pts',(-18.0477970193908,12.2452069498181,-18.6872733894581)) ;
#51588=CARTESIAN_POINT('Ctrl Pts',(-10.0532633905914,19.3545687670357,-18.937702685072)) ;
#51589=CARTESIAN_POINT('Ctrl Pts',(0.36034385407868,21.8068745304016,-19.1881319806858)) ;
#51590=CARTESIAN_POINT('Ctrl Pts',(10.687172324588,19.0118084296965,-19.4385612762997)) ;
#51591=CARTESIAN_POINT('Ctrl Pts',(18.4425729194978,11.6423899915026,-19.6889905719135)) ;
#51592=CARTESIAN_POINT('Ctrl Pts',(21.7600060694379,1.47095061324456,-19.9394198675273)) ;
#51593=CARTESIAN_POINT('Ctrl Pts',(19.842048593216,-9.05323515250154,-20.1898491631412)) ;
#51594=CARTESIAN_POINT('Ctrl Pts',(13.1471224801359,-17.4032624493475,-20.4403323712028)) ;
#51595=CARTESIAN_POINT('Ctrl Pts',(6.57435110142589,-20.1732611129558,-20.6073391473929)) ;
#51596=CARTESIAN_POINT('Ctrl Pts',(3.1534820175538,-20.6945201892214,-20.6908694917118)) ;
#51597=CARTESIAN_POINT('Ctrl Pts',(-16.4263691754732,11.9838076671105,-0.00108136862464728)) ;
#51598=CARTESIAN_POINT('Ctrl Pts',(-14.4457403151475,14.6987089311338,-0.084598324961714)) ;
#51599=CARTESIAN_POINT('Ctrl Pts',(-9.11588624546646,19.123921706411,-0.251591713170063)) ;
#51600=CARTESIAN_POINT('Ctrl Pts',(1.07849273288265,21.1569597046888,-0.502061533249697)) ;
#51601=CARTESIAN_POINT('Ctrl Pts',(11.0091098393319,18.0989931637232,-0.752490828863548)) ;
#51602=CARTESIAN_POINT('Ctrl Pts',(18.2919687091274,10.6859452534523,-1.0029201244774)) ;
#51603=CARTESIAN_POINT('Ctrl Pts',(21.1727305485295,0.701654794170591,-1.25334942009125)) ;
#51604=CARTESIAN_POINT('Ctrl Pts',(18.9591953603162,-9.45148522973715,-1.5037787157051)) ;
#51605=CARTESIAN_POINT('Ctrl Pts',(12.183492097342,-17.3303813635526,-1.75420801131895)) ;
#51606=CARTESIAN_POINT('Ctrl Pts',(2.47625737671769,-21.0392097052897,-2.0046373069328)) ;
#51607=CARTESIAN_POINT('Ctrl Pts',(-7.82686301156406,-19.685538122893,-2.25506660254666)) ;
#51608=CARTESIAN_POINT('Ctrl Pts',(-16.2466453691165,-13.5950930336833,
-2.50549589816051)) ;
#51609=CARTESIAN_POINT('Ctrl Pts',(-20.7571378876549,-4.23336821126094,
-2.75592519377435)) ;
#51610=CARTESIAN_POINT('Ctrl Pts',(-20.2729995248988,6.14699807860102,-3.00635448938821)) ;
#51611=CARTESIAN_POINT('Ctrl Pts',(-14.9107333511094,15.0482612183243,-3.25678378500206)) ;
#51612=CARTESIAN_POINT('Ctrl Pts',(-5.96061442093349,20.3285807893217,-3.50721308061591)) ;
#51613=CARTESIAN_POINT('Ctrl Pts',(4.42375902002995,20.7173955697377,-3.75764237622976)) ;
#51614=CARTESIAN_POINT('Ctrl Pts',(13.7436788763648,16.1211480933668,-4.0080716718436)) ;
#51615=CARTESIAN_POINT('Ctrl Pts',(19.75656631853,7.64579688878116,-4.25850096745746)) ;
#51616=CARTESIAN_POINT('Ctrl Pts',(21.0155883300835,-2.66930165867712,-4.50893026307131)) ;
#51617=CARTESIAN_POINT('Ctrl Pts',(17.217796298222,-12.3421073606251,-4.75935955868516)) ;
#51618=CARTESIAN_POINT('Ctrl Pts',(9.27702281322807,-19.0451298624311,-5.00978885429902)) ;
#51619=CARTESIAN_POINT('Ctrl Pts',(-0.896006952650112,-21.1654741319408,
-5.26021814991286)) ;
#51620=CARTESIAN_POINT('Ctrl Pts',(-10.8534376799843,-18.1929385806628,
-5.51064744552672)) ;
#51621=CARTESIAN_POINT('Ctrl Pts',(-18.1992919629658,-10.8427808126426,
-5.76107674114056)) ;
#51622=CARTESIAN_POINT('Ctrl Pts',(-21.1659952637126,-0.883610874166736,
-6.01150603675442)) ;
#51623=CARTESIAN_POINT('Ctrl Pts',(-19.0396933484483,9.28817532622884,-6.26193533236826)) ;
#51624=CARTESIAN_POINT('Ctrl Pts',(-12.3320213462269,17.2250217185411,-6.51236462798212)) ;
#51625=CARTESIAN_POINT('Ctrl Pts',(-2.65699306030903,21.0171480360003,-6.76279392359596)) ;
#51626=CARTESIAN_POINT('Ctrl Pts',(7.65736634854412,19.7520850619333,-7.01322321920982)) ;
#51627=CARTESIAN_POINT('Ctrl Pts',(16.1291945522093,13.7342348453136,-7.26365251482367)) ;
#51628=CARTESIAN_POINT('Ctrl Pts',(20.719982862645,4.41162485500801,-7.51408181043751)) ;
#51629=CARTESIAN_POINT('Ctrl Pts',(20.3250863753955,-5.97251936138383,-7.76451110605137)) ;
#51630=CARTESIAN_POINT('Ctrl Pts',(15.0395258936478,-14.919543712319,-8.01494040166522)) ;
#51631=CARTESIAN_POINT('Ctrl Pts',(6.13512382746137,-20.2765968375164,-8.26536969727907)) ;
#51632=CARTESIAN_POINT('Ctrl Pts',(-4.24552432450223,-20.7546536203216,
-8.51579899289292)) ;
#51633=CARTESIAN_POINT('Ctrl Pts',(-13.6046057008994,-16.2386830565945,
-8.76622828850679)) ;
#51634=CARTESIAN_POINT('Ctrl Pts',(-19.6901189343637,-7.81532725099089,
-9.01665758412061)) ;
#51635=CARTESIAN_POINT('Ctrl Pts',(-21.0377553420544,2.48856863625166,-9.26708687973448)) ;
#51636=CARTESIAN_POINT('Ctrl Pts',(-17.3232438859519,12.1936600312335,-9.51751617534832)) ;
#51637=CARTESIAN_POINT('Ctrl Pts',(-9.44037793549236,18.964687925841,-9.76794547096218)) ;
#51638=CARTESIAN_POINT('Ctrl Pts',(0.714051127217217,21.1723936926648,-10.018374766576)) ;
#51639=CARTESIAN_POINT('Ctrl Pts',(10.6966637423299,18.2855546394686,-10.2688040621899)) ;
#51640=CARTESIAN_POINT('Ctrl Pts',(18.1054231762193,10.9988079035636,-10.5192333578037)) ;
#51641=CARTESIAN_POINT('Ctrl Pts',(21.1576185297499,1.06550543830298,-10.7696626534176)) ;
#51642=CARTESIAN_POINT('Ctrl Pts',(19.1188242932827,-9.12418113213751,-11.0200919490314)) ;
#51643=CARTESIAN_POINT('Ctrl Pts',(12.4796193199814,-17.1183885140459,-11.2705212446453)) ;
#51644=CARTESIAN_POINT('Ctrl Pts',(2.83754273540551,-20.9935341215866,-11.5209505402591)) ;
#51645=CARTESIAN_POINT('Ctrl Pts',(-7.48730920532926,-19.8171724661533,
-11.771379835873)) ;
#51646=CARTESIAN_POINT('Ctrl Pts',(-16.0105494397262,-13.8723621033893,
-12.0218091314868)) ;
#51647=CARTESIAN_POINT('Ctrl Pts',(-20.6812984113101,-4.58955550264018,
-12.2722384271007)) ;
#51648=CARTESIAN_POINT('Ctrl Pts',(-20.3756709172924,5.79759936177647,-12.5226677227145)) ;
#51649=CARTESIAN_POINT('Ctrl Pts',(-15.1672076724889,14.789723970009,-12.7730970183284)) ;
#51650=CARTESIAN_POINT('Ctrl Pts',(-6.30917979159822,20.2231148453148,-13.0235263139422)) ;
#51651=CARTESIAN_POINT('Ctrl Pts',(4.06697587835583,20.7903783249431,-13.2739556095561)) ;
#51652=CARTESIAN_POINT('Ctrl Pts',(13.4645274662721,16.3550183063067,-13.5243849051699)) ;
#51653=CARTESIAN_POINT('Ctrl Pts',(19.622216823532,7.9842802192521,-13.7748142007838)) ;
#51654=CARTESIAN_POINT('Ctrl Pts',(21.0583681002872,-2.30765175935909,-14.0252434963976)) ;
#51655=CARTESIAN_POINT('Ctrl Pts',(17.4274116290366,-12.0443118359581,-14.2756727920115)) ;
#51656=CARTESIAN_POINT('Ctrl Pts',(9.60303560736628,-18.8828448813113,-14.5261020876253)) ;
#51657=CARTESIAN_POINT('Ctrl Pts',(-0.532042549462259,-21.1777490404263,
-14.7765313832392)) ;
#51658=CARTESIAN_POINT('Ctrl Pts',(-10.5390995359964,-18.3768197643338,
-15.026960678853)) ;
#51659=CARTESIAN_POINT('Ctrl Pts',(-18.0102167643638,-11.1540224047163,
-15.2773899744669)) ;
#51660=CARTESIAN_POINT('Ctrl Pts',(-21.1476786738334,-1.24732128233393,
-15.5278192700807)) ;
#51661=CARTESIAN_POINT('Ctrl Pts',(-19.1965427432879,8.95951284357439,-15.7782485656946)) ;
#51662=CARTESIAN_POINT('Ctrl Pts',(-12.6262953001234,17.0104906086833,-16.0286778613084)) ;
#51663=CARTESIAN_POINT('Ctrl Pts',(-3.01788277593133,20.9683692026586,-16.2791071569223)) ;
#51664=CARTESIAN_POINT('Ctrl Pts',(7.31669890603918,19.8807957919929,-16.5295364525362)) ;
#51665=CARTESIAN_POINT('Ctrl Pts',(15.8907214604756,14.0094644518822,-16.77996574815)) ;
#51666=CARTESIAN_POINT('Ctrl Pts',(20.6410860486261,4.76714711731379,-17.0303950437638)) ;
#51667=CARTESIAN_POINT('Ctrl Pts',(20.4247500695165,-5.62225112015366,-17.2808243393777)) ;
#51668=CARTESIAN_POINT('Ctrl Pts',(15.2937689759164,-14.6588114011443,-17.5312536349915)) ;
#51669=CARTESIAN_POINT('Ctrl Pts',(6.48276948662126,-20.1681390947737,-17.7816829306054)) ;
#51670=CARTESIAN_POINT('Ctrl Pts',(-3.88812667444911,-20.8245664079305,
-18.0321122262192)) ;
#51671=CARTESIAN_POINT('Ctrl Pts',(-13.3234550439929,-16.4701464896319,
-18.2825415218331)) ;
#51672=CARTESIAN_POINT('Ctrl Pts',(-19.5528639093576,-8.15264087805174,
-18.5329708174469)) ;
#51673=CARTESIAN_POINT('Ctrl Pts',(-21.0774272615067,2.12655962191487,-18.7834001130608)) ;
#51674=CARTESIAN_POINT('Ctrl Pts',(-17.5302875377575,11.8940831703183,-19.0338294086746)) ;
#51675=CARTESIAN_POINT('Ctrl Pts',(-9.76499224478906,18.7995884090949,-19.2842587042885)) ;
#51676=CARTESIAN_POINT('Ctrl Pts',(0.350011215644548,21.1815758126608,-19.5346879999023)) ;
#51677=CARTESIAN_POINT('Ctrl Pts',(10.3807242299048,18.4666565136597,-19.7851172955162)) ;
#51678=CARTESIAN_POINT('Ctrl Pts',(17.9137434816832,11.3085516176001,-20.03554659113)) ;
#51679=CARTESIAN_POINT('Ctrl Pts',(21.1360512759951,1.42877200892233,-20.2859758867439)) ;
#51680=CARTESIAN_POINT('Ctrl Pts',(19.273090051019,-8.793639201492,-20.5364051823577)) ;
#51681=CARTESIAN_POINT('Ctrl Pts',(12.7701368274074,-16.9042346001747,-20.7868883904192)) ;
#51682=CARTESIAN_POINT('Ctrl Pts',(6.3858356262729,-19.5948052554236,-20.9538951666095)) ;
#51683=CARTESIAN_POINT('Ctrl Pts',(3.06305785983022,-20.1011175482083,-21.0374255109284)) ;
#51684=CARTESIAN_POINT('',(16.4193236035816,11.9978307730923,-20.0002857096829)) ;
#51685=CARTESIAN_POINT('Ctrl Pts',(16.4197292796609,11.9981151325406,-19.9999999999999)) ;
#51686=CARTESIAN_POINT('Ctrl Pts',(16.6862133039597,11.6651737505463,-20.)) ;
#51687=CARTESIAN_POINT('Ctrl Pts',(16.9417323578455,11.3243161017761,-20.)) ;
#51688=CARTESIAN_POINT('Ctrl Pts',(17.1858733884563,10.9760266131827,-20.)) ;
#51689=CARTESIAN_POINT('Ctrl Pts',(17.2064494004021,10.9466730520056,-20.)) ;
#51690=CARTESIAN_POINT('Ctrl Pts',(17.2269445780442,10.9172666767459,-20.)) ;
#51691=CARTESIAN_POINT('Ctrl Pts',(17.247358664803,10.8878077633562,-20.)) ;
#51692=CARTESIAN_POINT('Ctrl Pts',(17.4900365983564,10.5376070264538,-20.)) ;
#51693=CARTESIAN_POINT('Ctrl Pts',(17.7212580268335,10.1799851561655,-20.)) ;
#51694=CARTESIAN_POINT('Ctrl Pts',(17.9409219607083,9.81560429891178,-20.)) ;
#51695=CARTESIAN_POINT('Ctrl Pts',(18.1595616319545,9.45292249934163,-20.)) ;
#51696=CARTESIAN_POINT('Ctrl Pts',(18.3667515113989,9.08354407349083,-20.)) ;
#51697=CARTESIAN_POINT('Ctrl Pts',(18.5623524443059,8.70808474634139,-20.)) ;
#51698=CARTESIAN_POINT('Ctrl Pts',(18.7589822028964,8.33065057074363,-20.)) ;
#51699=CARTESIAN_POINT('Ctrl Pts',(18.9439010327212,7.94707088429373,-20.)) ;
#51700=CARTESIAN_POINT('Ctrl Pts',(19.1169242226168,7.55794089715604,-20.)) ;
#51701=CARTESIAN_POINT('Ctrl Pts',(19.2899858008947,7.16872457436191,-20.)) ;
#51702=CARTESIAN_POINT('Ctrl Pts',(19.451146684296,6.77395498478179,-20.)) ;
#51703=CARTESIAN_POINT('Ctrl Pts',(19.6001752754721,6.37420488768944,-20.)) ;
#51704=CARTESIAN_POINT('Ctrl Pts',(19.7492082704025,5.9744429780903,-20.)) ;
#51705=CARTESIAN_POINT('Ctrl Pts',(19.8861084889852,5.56969975867407,-20.)) ;
#51706=CARTESIAN_POINT('Ctrl Pts',(20.010594127929,5.16053277403186,-20.)) ;
#51707=CARTESIAN_POINT('Ctrl Pts',(20.029874433682,5.09716109007805,-20.)) ;
#51708=CARTESIAN_POINT('Ctrl Pts',(20.0488574581927,5.03368115903446,-20.)) ;
#51709=CARTESIAN_POINT('Ctrl Pts',(20.0675400518462,4.97010181780182,-20.)) ;
#51710=CARTESIAN_POINT('Ctrl Pts',(20.0825290409452,4.91909230218903,-20.)) ;
#51711=CARTESIAN_POINT('Ctrl Pts',(20.0973224475511,4.86802621134112,-20.)) ;
#51712=CARTESIAN_POINT('Ctrl Pts',(20.1119161689802,4.81691812032873,-20.)) ;
#51713=CARTESIAN_POINT('Ctrl Pts',(20.2302152409695,4.40262764841097,-20.)) ;
#51714=CARTESIAN_POINT('Ctrl Pts',(20.3354841370377,3.98528158528001,-20.)) ;
#51715=CARTESIAN_POINT('Ctrl Pts',(20.427602726343,3.56551255586273,-20.)) ;
#51716=CARTESIAN_POINT('Ctrl Pts',(20.5202217737677,3.14346302236244,-20.)) ;
#51717=CARTESIAN_POINT('Ctrl Pts',(20.5995474842104,2.71896362856786,-20.)) ;
#51718=CARTESIAN_POINT('Ctrl Pts',(20.6654124192146,2.29263066822524,-20.)) ;
#51719=CARTESIAN_POINT('Ctrl Pts',(20.7109932711171,1.99759326288532,-20.)) ;
#51720=CARTESIAN_POINT('Ctrl Pts',(20.7501266438824,1.70167717908982,-20.)) ;
#51721=CARTESIAN_POINT('Ctrl Pts',(20.7827435110061,1.40508115597038,-20.)) ;
#51722=CARTESIAN_POINT('Ctrl Pts',(20.8295945595039,0.979048986458191,-20.)) ;
#51723=CARTESIAN_POINT('Ctrl Pts',(20.8630027249507,0.551614161017511,-20.)) ;
#51724=CARTESIAN_POINT('Ctrl Pts',(20.8831226202743,0.123380410496852,-20.)) ;
#51725=CARTESIAN_POINT('Ctrl Pts',(20.9033298789958,-0.306712790829077,
-20.)) ;
#51726=CARTESIAN_POINT('Ctrl Pts',(20.9101332115589,-0.737612398604347,
-20.)) ;
#51727=CARTESIAN_POINT('Ctrl Pts',(20.9036368555828,-1.16871241502824,-20.)) ;
#51728=CARTESIAN_POINT('Ctrl Pts',(20.8971421869036,-1.59970046194614,-20.)) ;
#51729=CARTESIAN_POINT('Ctrl Pts',(20.8773546977867,-2.03088935474534,-20.)) ;
#51730=CARTESIAN_POINT('Ctrl Pts',(20.8443266935953,-2.4616711459039,-20.)) ;
#51731=CARTESIAN_POINT('Ctrl Pts',(20.8299804328112,-2.64878835350629,-20.)) ;
#51732=CARTESIAN_POINT('Ctrl Pts',(20.8131353688933,-2.83582867226119,-20.)) ;
#51733=CARTESIAN_POINT('Ctrl Pts',(20.7937927667325,-3.02274173750564,-20.)) ;
#51734=CARTESIAN_POINT('Ctrl Pts',(20.7887912971327,-3.07107236054491,-20.)) ;
#51735=CARTESIAN_POINT('Ctrl Pts',(20.7836229540371,-3.11939285262655,-20.)) ;
#51736=CARTESIAN_POINT('Ctrl Pts',(20.7782901354159,-3.16768221580796,-20.)) ;
#51737=CARTESIAN_POINT('Ctrl Pts',(20.7307766888087,-3.59792262753397,-20.)) ;
#51738=CARTESIAN_POINT('Ctrl Pts',(20.670167860427,-4.02611636531182,-20.)) ;
#51739=CARTESIAN_POINT('Ctrl Pts',(20.5966777225206,-4.45165660389502,-20.)) ;
#51740=CARTESIAN_POINT('Ctrl Pts',(20.5223305323676,-4.88215955214073,-20.)) ;
#51741=CARTESIAN_POINT('Ctrl Pts',(20.4347998671604,-5.30994727220065,-20.)) ;
#51742=CARTESIAN_POINT('Ctrl Pts',(20.3342547042927,-5.73439911854882,-20.)) ;
#51743=CARTESIAN_POINT('Ctrl Pts',(20.2335254061709,-6.15962829268022,-20.)) ;
#51744=CARTESIAN_POINT('Ctrl Pts',(20.1197338520914,-6.58150991347884,-20.)) ;
#51745=CARTESIAN_POINT('Ctrl Pts',(19.9929976115934,-6.99941944689774,-20.)) ;
#51746=CARTESIAN_POINT('Ctrl Pts',(19.8668278005729,-7.41546119350469,-20.)) ;
#51747=CARTESIAN_POINT('Ctrl Pts',(19.7278286613732,-7.82756681794848,-20.)) ;
#51748=CARTESIAN_POINT('Ctrl Pts',(19.5760654853802,-8.23511151272187,-20.)) ;
#51749=CARTESIAN_POINT('Ctrl Pts',(19.5021725166428,-8.43354362375884,-20.)) ;
#51750=CARTESIAN_POINT('Ctrl Pts',(19.4252528423934,-8.63089430266909,-20.)) ;
#51751=CARTESIAN_POINT('Ctrl Pts',(19.3453097129688,-8.82709009854958,-20.)) ;
#51752=CARTESIAN_POINT('Ctrl Pts',(19.180732696096,-9.2309937115481,-20.)) ;
#51753=CARTESIAN_POINT('Ctrl Pts',(19.0033447592909,-9.6300043076582,-20.)) ;
#51754=CARTESIAN_POINT('Ctrl Pts',(18.8135117710249,-10.023630445027,-20.)) ;
#51755=CARTESIAN_POINT('Ctrl Pts',(18.6803892841659,-10.2996651362462,-20.)) ;
#51756=CARTESIAN_POINT('Ctrl Pts',(18.5411457110759,-10.5730515120463,-20.0000000000001)) ;
#51757=CARTESIAN_POINT('Ctrl Pts',(18.3958940868607,-10.843612277219,-20.)) ;
#51758=CARTESIAN_POINT('Ctrl Pts',(18.376401160023,-10.8799218278293,-20.)) ;
#51759=CARTESIAN_POINT('Ctrl Pts',(18.3567991230378,-10.9161820673089,-20.)) ;
#51760=CARTESIAN_POINT('Ctrl Pts',(18.3370964703204,-10.9523775690894,-20.)) ;
#51761=CARTESIAN_POINT('Ctrl Pts',(18.1288264545511,-11.3349878619637,-20.)) ;
#51762=CARTESIAN_POINT('Ctrl Pts',(17.9091288638351,-11.7107205413323,-20.)) ;
#51763=CARTESIAN_POINT('Ctrl Pts',(17.6785011392334,-12.0791488707737,-20.)) ;
#51764=CARTESIAN_POINT('Ctrl Pts',(17.4454005262735,-12.4515276451508,-20.)) ;
#51765=CARTESIAN_POINT('Ctrl Pts',(17.2011339150899,-12.8164450377157,-20.)) ;
#51766=CARTESIAN_POINT('Ctrl Pts',(16.9461630841213,-13.1734471994973,-20.)) ;
#51767=CARTESIAN_POINT('Ctrl Pts',(16.6895009605379,-13.5328174561601,-20.)) ;
#51768=CARTESIAN_POINT('Ctrl Pts',(16.4219918820727,-13.8841675923275,-20.)) ;
#51769=CARTESIAN_POINT('Ctrl Pts',(16.1440582308894,-14.227014410769,-20.)) ;
#51770=CARTESIAN_POINT('Ctrl Pts',(15.8659290427536,-14.5701024350588,-20.)) ;
#51771=CARTESIAN_POINT('Ctrl Pts',(15.5773603059104,-14.9046756305149,-20.)) ;
#51772=CARTESIAN_POINT('Ctrl Pts',(15.2787310149449,-15.2302226371145,-20.)) ;
#51773=CARTESIAN_POINT('Ctrl Pts',(14.9815081945709,-15.5542363972954,-20.)) ;
#51774=CARTESIAN_POINT('Ctrl Pts',(14.6743190319459,-15.8693092199902,-20.)) ;
#51775=CARTESIAN_POINT('Ctrl Pts',(14.3574981339932,-16.1749034673177,-20.)) ;
#51776=CARTESIAN_POINT('Ctrl Pts',(14.0446734403697,-16.4766431171044,-20.)) ;
#51777=CARTESIAN_POINT('Ctrl Pts',(13.722458104397,-16.7691421598843,-20.)) ;
#51778=CARTESIAN_POINT('Ctrl Pts',(13.3911412031311,-17.051844554609,-20.)) ;
#51779=CARTESIAN_POINT('Ctrl Pts',(13.2887762376605,-17.1391893920256,-20.)) ;
#51780=CARTESIAN_POINT('Ctrl Pts',(13.1855422289172,-17.2255987530988,-20.)) ;
#51781=CARTESIAN_POINT('Ctrl Pts',(13.0814471333101,-17.3110553987592,-20.)) ;
#51782=CARTESIAN_POINT('Ctrl Pts',(13.048030312067,-17.3384888665457,-20.)) ;
#51783=CARTESIAN_POINT('Ctrl Pts',(13.0145317665027,-17.3658183827095,-20.)) ;
#51784=CARTESIAN_POINT('Ctrl Pts',(12.9809537152124,-17.3930425047458,-20.)) ;
#51785=CARTESIAN_POINT('Ctrl Pts',(12.6331656762335,-17.6750190832576,-20.)) ;
#51786=CARTESIAN_POINT('Ctrl Pts',(12.2767956567509,-17.9457381705363,-20.)) ;
#51787=CARTESIAN_POINT('Ctrl Pts',(11.9125033775857,-18.2050396015228,-20.)) ;
#51788=CARTESIAN_POINT('Ctrl Pts',(11.5503007497329,-18.4628536291067,-20.)) ;
#51789=CARTESIAN_POINT('Ctrl Pts',(11.1802659791631,-18.7093808135623,-20.)) ;
#51790=CARTESIAN_POINT('Ctrl Pts',(10.8030080891504,-18.9444265203506,-20.)) ;
#51791=CARTESIAN_POINT('Ctrl Pts',(10.4239904271859,-19.1805686305624,-20.)) ;
#51792=CARTESIAN_POINT('Ctrl Pts',(10.037681655143,-19.4051221766271,-20.)) ;
#51793=CARTESIAN_POINT('Ctrl Pts',(9.64466654416206,-19.6178484363144,-20.)) ;
#51794=CARTESIAN_POINT('Ctrl Pts',(9.39842589258477,-19.75113046881,-20.)) ;
#51795=CARTESIAN_POINT('Ctrl Pts',(9.14955200279447,-19.8797687995387,-20.)) ;
#51796=CARTESIAN_POINT('Ctrl Pts',(8.89818338640667,-20.0036957576717,-19.9999999999999)) ;
#51797=CARTESIAN_POINT('Ctrl Pts',(8.81183420772632,-20.0462666688893,-19.9999999999999)) ;
#51798=CARTESIAN_POINT('Ctrl Pts',(8.72519061167969,-20.088281560275,-19.9999999999999)) ;
#51799=CARTESIAN_POINT('Ctrl Pts',(8.63825811992194,-20.1297374908914,-20.)) ;
#51800=CARTESIAN_POINT('Ctrl Pts',(8.56437314507967,-20.1649713870874,-20.)) ;
#51801=CARTESIAN_POINT('Ctrl Pts',(8.49027196637771,-20.1998049273805,-20.)) ;
#51802=CARTESIAN_POINT('Ctrl Pts',(8.41599661777268,-20.2342185484354,-20.)) ;
#51803=CARTESIAN_POINT('Ctrl Pts',(8.00723515078845,-20.4236079285037,-20.)) ;
#51804=CARTESIAN_POINT('Ctrl Pts',(7.59304737752386,-20.600359290717,-20.)) ;
#51805=CARTESIAN_POINT('Ctrl Pts',(7.17405350980231,-20.7642755093381,-20.)) ;
#51806=CARTESIAN_POINT('Ctrl Pts',(6.7543491679915,-20.9284696752876,-20.)) ;
#51807=CARTESIAN_POINT('Ctrl Pts',(6.32982193923238,-21.0797853877173,-20.)) ;
#51808=CARTESIAN_POINT('Ctrl Pts',(5.90106642836833,-21.2179806890933,-20.)) ;
#51809=CARTESIAN_POINT('Ctrl Pts',(5.4746446821956,-21.355423777829,-20.)) ;
#51810=CARTESIAN_POINT('Ctrl Pts',(5.04404006112706,-21.4798891022081,-20.)) ;
#51811=CARTESIAN_POINT('Ctrl Pts',(4.6098164331882,-21.591091970763,-20.)) ;
#51812=CARTESIAN_POINT('Ctrl Pts',(4.18999697364085,-21.6986059915877,-20.)) ;
#51813=CARTESIAN_POINT('Ctrl Pts',(3.76679413188183,-21.7937228229268,-20.)) ;
#51814=CARTESIAN_POINT('Ctrl Pts',(3.34070509846234,-21.8761405304411,-20.)) ;
#51815=CARTESIAN_POINT('Ctrl Pts',(16.4056275812262,12.0157134421436,-20.)) ;
#51816=CARTESIAN_POINT('Ctrl Pts',(16.4100629678363,12.0096575969161,-20.000095236561)) ;
#51817=CARTESIAN_POINT('Ctrl Pts',(16.414495001335,12.0035992958223,-20.0001904731219)) ;
#51818=CARTESIAN_POINT('Ctrl Pts',(16.4189236790046,11.9975385425771,-20.0002857096829)) ;
#51819=CARTESIAN_POINT('Origin',(0.,20.065,-20.)) ;
#51820=CARTESIAN_POINT('',(-2.45725380248917E-15,-20.065,-20.)) ;
#51821=CARTESIAN_POINT('Origin',(0.,0.,-20.)) ;
#51822=CARTESIAN_POINT('Origin',(5.00000000000251,14.8,-258.5)) ;
#51823=CARTESIAN_POINT('',(5.00000000000251,14.8,-303.5)) ;
#51824=CARTESIAN_POINT('',(5.00000000000251,14.8,-303.5)) ;
#51825=CARTESIAN_POINT('',(5.00000000000251,14.8,-258.5)) ;
#51826=CARTESIAN_POINT('',(5.00000000000251,14.8,-258.5)) ;
#51827=CARTESIAN_POINT('',(5.00000000000251,14.8,-258.5)) ;
#51828=CARTESIAN_POINT('Origin',(0.,14.8,-258.5)) ;
#51829=CARTESIAN_POINT('',(-5.00000000000251,14.8,-258.5)) ;
#51830=CARTESIAN_POINT('Origin',(0.,14.8,-258.5)) ;
#51831=CARTESIAN_POINT('',(-5.00000000000251,14.8,-258.5)) ;
#51832=CARTESIAN_POINT('Origin',(-5.00000000000251,14.8,-303.5)) ;
#51833=CARTESIAN_POINT('',(-5.00000000000251,14.8,-303.5)) ;
#51834=CARTESIAN_POINT('',(-5.00000000000251,14.8,-303.5)) ;
#51835=CARTESIAN_POINT('',(-5.00000000000251,14.8,-303.5)) ;
#51836=CARTESIAN_POINT('Origin',(0.,14.8,-303.5)) ;
#51837=CARTESIAN_POINT('Origin',(0.,14.8,-303.5)) ;
#51838=CARTESIAN_POINT('Origin',(0.,14.8,-281.)) ;
#51839=CARTESIAN_POINT('Origin',(0.,0.,-22.)) ;
#51840=CARTESIAN_POINT('',(-2.45725380248917E-15,-20.065,-24.)) ;
#51841=CARTESIAN_POINT('Origin',(0.,0.,-24.)) ;
#51842=CARTESIAN_POINT('',(-2.45725380248916E-15,-20.065,-22.)) ;
#51843=CARTESIAN_POINT('Origin',(0.,23.,-24.)) ;
#51844=CARTESIAN_POINT('',(-2.81668763803891E-15,-23.,-24.)) ;
#51845=CARTESIAN_POINT('Origin',(0.,0.,-24.)) ;
#51846=CARTESIAN_POINT('Origin',(0.,0.,-29.)) ;
#51847=CARTESIAN_POINT('',(-2.81668763803891E-15,-23.,-29.)) ;
#51848=CARTESIAN_POINT('Origin',(0.,0.,-42.87)) ;
#51849=CARTESIAN_POINT('',(-2.45725380248916E-15,-20.065,-42.87)) ;
#51850=CARTESIAN_POINT('Origin',(0.,0.,-72.)) ;
#51851=CARTESIAN_POINT('',(-2.75545529808154E-15,-22.5,-88.)) ;
#51852=CARTESIAN_POINT('Origin',(0.,0.,-88.)) ;
#51853=CARTESIAN_POINT('',(-2.75545529808154E-15,-22.5,-72.)) ;
#51854=CARTESIAN_POINT('Origin',(0.,22.25,-88.)) ;
#51855=CARTESIAN_POINT('',(-2.72483912810286E-15,-22.25,-88.)) ;
#51856=CARTESIAN_POINT('Origin',(0.,0.,-88.)) ;
#51857=CARTESIAN_POINT('Origin',(0.,0.,-146.)) ;
#51858=CARTESIAN_POINT('',(-2.72483912810286E-15,-22.25,-204.)) ;
#51859=CARTESIAN_POINT('Origin',(0.,0.,-204.)) ;
#51860=CARTESIAN_POINT('',(-2.72483912810286E-15,-22.25,-146.)) ;
#51861=CARTESIAN_POINT('Origin',(0.,22.5,-204.)) ;
#51862=CARTESIAN_POINT('Origin',(0.,0.,-317.125)) ;
#51863=CARTESIAN_POINT('',(-2.20436423846523E-15,-18.,-318.25)) ;
#51864=CARTESIAN_POINT('Origin',(0.,0.,-318.25)) ;
#51865=CARTESIAN_POINT('',(-2.20436423846524E-15,-18.,-317.125)) ;
#51866=CARTESIAN_POINT('Origin',(0.,19.5,-318.25)) ;
#63797=UNCERTAINTY_MEASURE_WITH_UNIT(LENGTH_MEASURE(0.01),#63825,
'DISTANCE_ACCURACY_VALUE',
'Maximum model space distance between geometric entities at asserted c
onnectivities') ;
#63807=UNCERTAINTY_MEASURE_WITH_UNIT(LENGTH_MEASURE(0.01),#63825,
'DISTANCE_ACCURACY_VALUE',
'Maximum model space distance between geometric entities at asserted c
onnectivities') ;
#63814=(
GEOMETRIC_REPRESENTATION_CONTEXT(3)
GLOBAL_UNCERTAINTY_ASSIGNED_CONTEXT((#63797))
GLOBAL_UNIT_ASSIGNED_CONTEXT((#63825,#63827,#63828))
REPRESENTATION_CONTEXT('','3D')
) ;
#63824=(
GEOMETRIC_REPRESENTATION_CONTEXT(3)
GLOBAL_UNCERTAINTY_ASSIGNED_CONTEXT((#63807))
GLOBAL_UNIT_ASSIGNED_CONTEXT((#63825,#63827,#63828))
REPRESENTATION_CONTEXT('','3D')
) ;
#63825=(
LENGTH_UNIT()
NAMED_UNIT(*)
SI_UNIT(.MILLI.,.METRE.)
) ;
#63827=(
NAMED_UNIT(*)
PLANE_ANGLE_UNIT()
SI_UNIT($,.RADIAN.)
) ;
#63828=(
NAMED_UNIT(*)
SI_UNIT($,.STERADIAN.)
SOLID_ANGLE_UNIT()
) ;
#63835=SHAPE_DEFINITION_REPRESENTATION(#63851,#63884) ;
#63851=PRODUCT_DEFINITION_SHAPE('',$,#63901) ;
#63884=SHAPE_REPRESENTATION('',(#16025),#63814) ;
#63894=PRODUCT_DEFINITION_CONTEXT('part definition',#63944,'design') ;
#63901=PRODUCT_DEFINITION('Spindle','Spindle',#63917,#63894) ;
#63917=PRODUCT_DEFINITION_FORMATION('',$,#63952) ;
#63944=APPLICATION_CONTEXT(
'Core Data for Automotive Mechanical Design Process') ;
#63945=PRODUCT_CONTEXT('part definition',#63944,'mechanical') ;
#63952=PRODUCT('Spindle','Spindle',$,(#63945)) ;
#63964=PRESENTATION_STYLE_ASSIGNMENT((#63969)) ;
#63969=SURFACE_STYLE_USAGE(.BOTH.,#63974) ;
#63974=SURFACE_SIDE_STYLE('',(#63979)) ;
#63979=SURFACE_STYLE_FILL_AREA(#63984) ;
#63984=FILL_AREA_STYLE('Opaque(203,203,203)',(#63989)) ;
#63989=FILL_AREA_STYLE_COLOUR('Opaque(203,203,203)',#63994) ;
#63994=COLOUR_RGB('Opaque(203,203,203)', 0.08235294, 0.09019608, 0.10196078) ;
ENDSEC;
END-ISO-10303-21;
